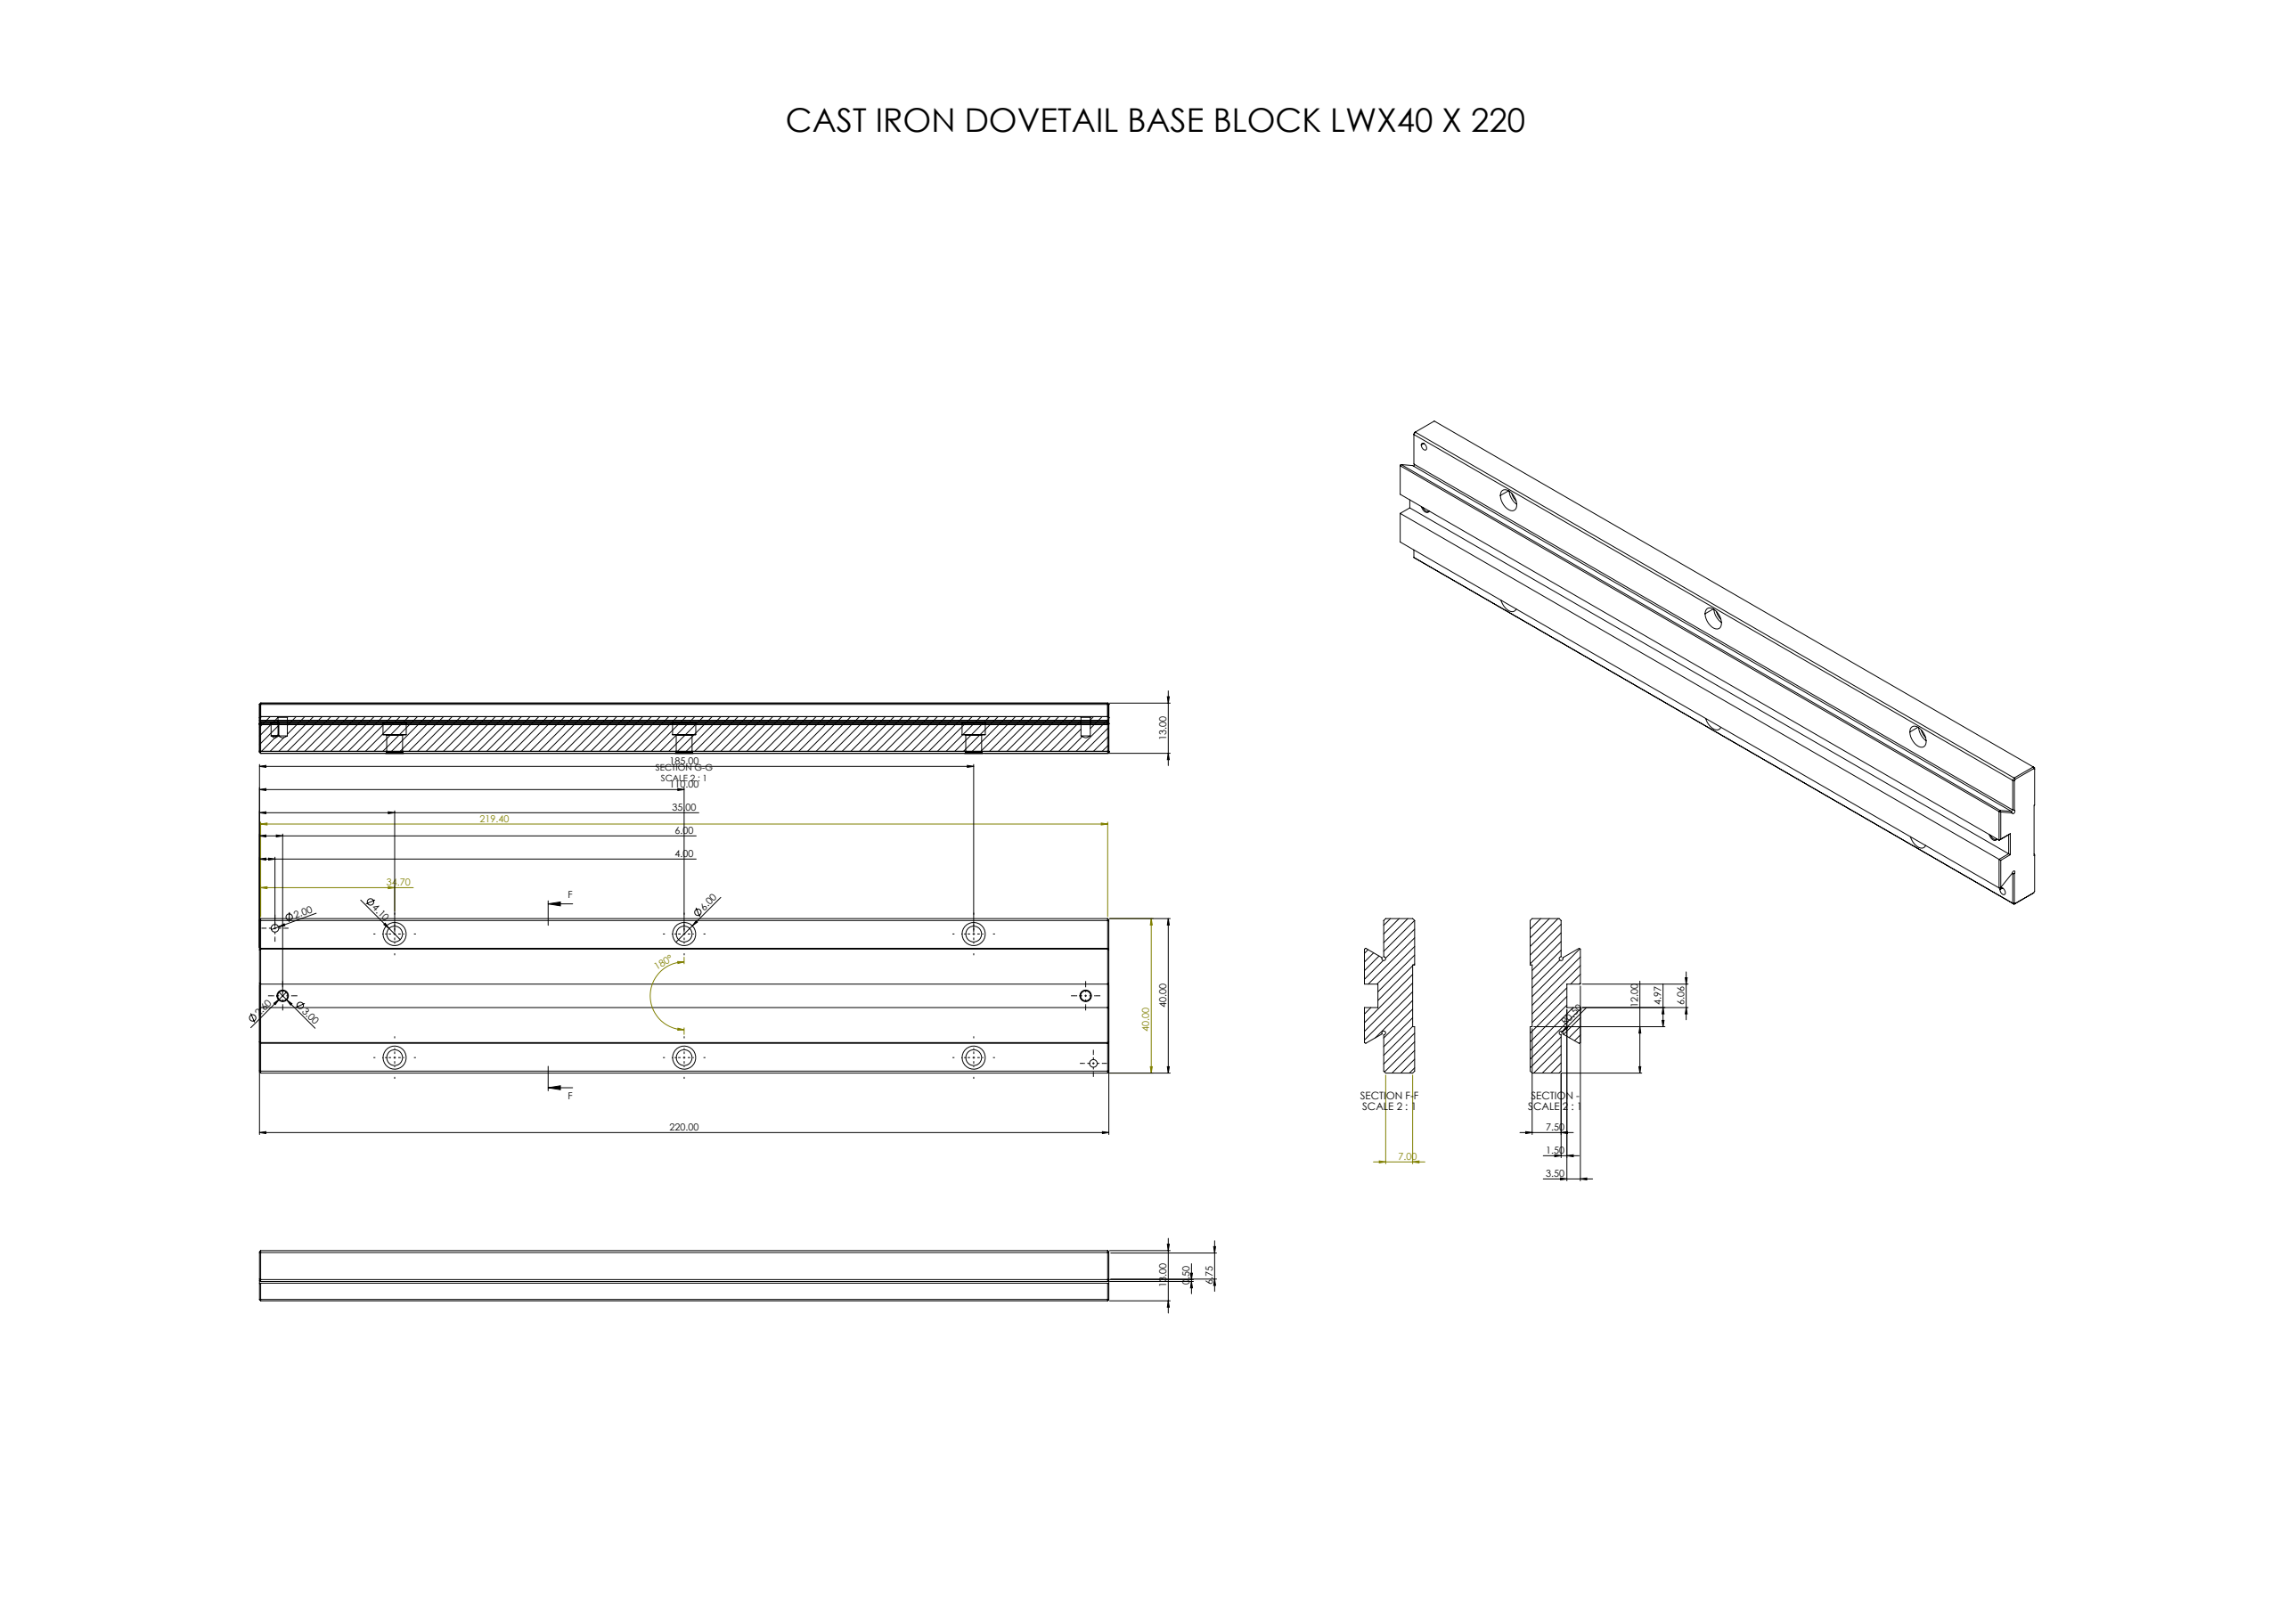
ISO-10303-21;
HEADER;
/* Generated by software containing ST-Developer
 * from STEP Tools, Inc. (www.steptools.com) 
 */

FILE_DESCRIPTION(
/* description */ (''),
/* implementation_level */ '2;1');

FILE_NAME(
/* name */ 'Cast Iron Dovetail Base Block LWX40 x 220.step',
/* time_stamp */ '2026-10-05T09:57:53+05:00',
/* author */ (''),
/* organization */ (''),
/* preprocessor_version */ 'ST-DEVELOPER v20.2',
/* originating_system */ 'Autodesk Translation Framework v15.15.0.0',
/* authorisation */ '');

FILE_SCHEMA (('AUTOMOTIVE_DESIGN { 1 0 10303 214 3 1 1 }'));
ENDSEC;

DATA;
#10=MECHANICAL_DESIGN_GEOMETRIC_PRESENTATION_REPRESENTATION('',(#551),#113984);
#515=SHAPE_REPRESENTATION_RELATIONSHIP('SRR','None',#114052,#533);
#533=ADVANCED_BREP_SHAPE_REPRESENTATION('',(#569),#113966);
#551=STYLED_ITEM('',(#114289),#569);
#569=MANIFOLD_SOLID_BREP('Cast Iron Dovetail Base Block LWX40 x 220',#60392);
#587=ELLIPSE('',#61749,0.707106781186562,0.499999999999998);
#588=ELLIPSE('',#61756,0.70710678118656,0.5);
#589=ELLIPSE('',#61760,0.707106781186549,0.499999999999998);
#590=ELLIPSE('',#61761,0.707106781186545,0.499999999999998);
#591=ELLIPSE('',#61762,0.707106781186558,0.499999999999998);
#592=ELLIPSE('',#61770,0.707106781186561,0.5);
#593=ELLIPSE('',#61787,0.707106781186547,0.5);
#594=ELLIPSE('',#61805,0.707106781186548,0.5);
#603=CYLINDRICAL_SURFACE('',#61679,1.);
#604=CYLINDRICAL_SURFACE('',#61681,1.00000000000001);
#605=CYLINDRICAL_SURFACE('',#61686,1.29999999999999);
#606=CYLINDRICAL_SURFACE('',#61693,1.3);
#607=CYLINDRICAL_SURFACE('',#61696,3.00000000000001);
#608=CYLINDRICAL_SURFACE('',#61701,3.);
#609=CYLINDRICAL_SURFACE('',#61706,3.);
#610=CYLINDRICAL_SURFACE('',#61711,3.00000000000001);
#611=CYLINDRICAL_SURFACE('',#61716,3.00000000000001);
#612=CYLINDRICAL_SURFACE('',#61721,3.00000000000001);
#613=CYLINDRICAL_SURFACE('',#61732,2.04999999999998);
#614=CYLINDRICAL_SURFACE('',#61735,2.05);
#615=CYLINDRICAL_SURFACE('',#61738,2.05);
#616=CYLINDRICAL_SURFACE('',#61741,2.05);
#617=CYLINDRICAL_SURFACE('',#61744,2.05);
#618=CYLINDRICAL_SURFACE('',#61747,2.04999999999998);
#619=CYLINDRICAL_SURFACE('',#61759,0.499999999999998);
#620=CYLINDRICAL_SURFACE('',#61809,0.5);
#875=CONICAL_SURFACE('',#61675,0.999999999999979,1.02974425867664);
#876=CONICAL_SURFACE('',#61677,1.,1.02974425867665);
#877=CONICAL_SURFACE('',#61683,1.39999999999999,0.785398163397437);
#878=CONICAL_SURFACE('',#61690,1.30000000000003,1.02974425867666);
#879=CONICAL_SURFACE('',#61691,1.4,0.785398163397448);
#880=CONICAL_SURFACE('',#61695,1.3,1.02974425867665);
#881=CONICAL_SURFACE('',#61726,2.19999999999999,0.785398163397467);
#882=CONICAL_SURFACE('',#61733,2.2,0.785398163397438);
#883=CONICAL_SURFACE('',#61736,2.2,0.785398163397438);
#884=CONICAL_SURFACE('',#61739,2.2,0.785398163397445);
#885=CONICAL_SURFACE('',#61742,2.2,0.785398163397445);
#886=CONICAL_SURFACE('',#61745,2.19999999999999,0.785398163397467);
#957=CIRCLE('',#61666,0.499999999999998);
#958=CIRCLE('',#61667,0.5);
#959=CIRCLE('',#61672,2.34999999999999);
#960=CIRCLE('',#61673,2.35);
#961=CIRCLE('',#61674,2.34999999999999);
#962=CIRCLE('',#61676,1.00000000000001);
#963=CIRCLE('',#61678,1.);
#964=CIRCLE('',#61680,1.);
#965=CIRCLE('',#61682,1.00000000000001);
#966=CIRCLE('',#61684,1.49999999999999);
#967=CIRCLE('',#61685,1.29999999999999);
#968=CIRCLE('',#61687,1.29999999999999);
#969=CIRCLE('',#61689,1.5);
#970=CIRCLE('',#61692,1.3);
#971=CIRCLE('',#61694,1.3);
#972=CIRCLE('',#61697,3.00000000000001);
#973=CIRCLE('',#61698,3.00000000000001);
#974=CIRCLE('',#61700,2.04999999999998);
#975=CIRCLE('',#61702,3.);
#976=CIRCLE('',#61703,3.);
#977=CIRCLE('',#61705,2.05);
#978=CIRCLE('',#61707,3.);
#979=CIRCLE('',#61708,3.);
#980=CIRCLE('',#61710,2.05);
#981=CIRCLE('',#61712,3.00000000000001);
#982=CIRCLE('',#61713,3.00000000000001);
#983=CIRCLE('',#61715,2.05);
#984=CIRCLE('',#61717,3.00000000000001);
#985=CIRCLE('',#61718,3.00000000000001);
#986=CIRCLE('',#61720,2.05);
#987=CIRCLE('',#61722,3.00000000000001);
#988=CIRCLE('',#61723,3.00000000000001);
#989=CIRCLE('',#61725,2.04999999999998);
#990=CIRCLE('',#61727,2.04999999999998);
#991=CIRCLE('',#61729,2.34999999999999);
#992=CIRCLE('',#61730,2.35);
#993=CIRCLE('',#61731,2.34999999999999);
#994=CIRCLE('',#61734,2.05);
#995=CIRCLE('',#61737,2.05);
#996=CIRCLE('',#61740,2.05);
#997=CIRCLE('',#61743,2.05);
#998=CIRCLE('',#61746,2.04999999999998);
#999=CIRCLE('',#61763,0.499999999999998);
#1000=CIRCLE('',#61807,0.5);
#1542=FACE_BOUND('',#7313,.T.);
#1543=FACE_BOUND('',#7345,.T.);
#1544=FACE_BOUND('',#7369,.T.);
#1545=FACE_BOUND('',#7404,.T.);
#1546=FACE_BOUND('',#7405,.T.);
#1547=FACE_BOUND('',#7430,.T.);
#1548=FACE_BOUND('',#7465,.T.);
#1549=FACE_BOUND('',#7495,.T.);
#1550=FACE_BOUND('',#7519,.T.);
#1551=FACE_BOUND('',#7565,.T.);
#1552=FACE_BOUND('',#7581,.T.);
#1553=FACE_BOUND('',#7605,.T.);
#1554=FACE_BOUND('',#7659,.T.);
#1555=FACE_BOUND('',#7705,.T.);
#1556=FACE_BOUND('',#7738,.T.);
#1557=FACE_BOUND('',#7761,.T.);
#1558=FACE_BOUND('',#7794,.T.);
#1559=FACE_BOUND('',#7840,.T.);
#1560=FACE_BOUND('',#7894,.T.);
#1561=FACE_BOUND('',#7910,.T.);
#1562=FACE_BOUND('',#7934,.T.);
#1563=FACE_BOUND('',#7980,.T.);
#1564=FACE_BOUND('',#8010,.T.);
#1565=FACE_BOUND('',#8034,.T.);
#1566=FACE_BOUND('',#8069,.T.);
#1567=FACE_BOUND('',#8104,.T.);
#1568=FACE_BOUND('',#8105,.T.);
#1569=FACE_BOUND('',#8130,.T.);
#1570=FACE_BOUND('',#8162,.T.);
#1571=FACE_BOUND('',#9078,.T.);
#1572=FACE_BOUND('',#9079,.T.);
#1573=FACE_BOUND('',#9080,.T.);
#1574=FACE_BOUND('',#9088,.T.);
#1575=FACE_BOUND('',#9089,.T.);
#1576=FACE_BOUND('',#9096,.T.);
#1577=FACE_BOUND('',#9099,.T.);
#1578=FACE_BOUND('',#9102,.T.);
#1579=FACE_BOUND('',#9105,.T.);
#1580=FACE_BOUND('',#9108,.T.);
#1581=FACE_BOUND('',#9111,.T.);
#1582=FACE_BOUND('',#9114,.T.);
#1583=FACE_BOUND('',#9115,.T.);
#1584=FACE_BOUND('',#9116,.T.);
#1585=FACE_BOUND('',#9152,.T.);
#1586=FACE_BOUND('',#9153,.T.);
#1587=FACE_BOUND('',#9154,.T.);
#1588=FACE_BOUND('',#9155,.T.);
#1589=FACE_BOUND('',#9161,.T.);
#1590=FACE_BOUND('',#9162,.T.);
#1591=FACE_BOUND('',#9163,.T.);
#1592=FACE_BOUND('',#9164,.T.);
#1593=FACE_BOUND('',#9165,.T.);
#1594=FACE_BOUND('',#9166,.T.);
#1595=FACE_BOUND('',#9167,.T.);
#1596=FACE_BOUND('',#9168,.T.);
#1597=FACE_BOUND('',#9169,.T.);
#1598=FACE_BOUND('',#9170,.T.);
#1599=FACE_BOUND('',#9171,.T.);
#1600=FACE_BOUND('',#9172,.T.);
#1601=FACE_BOUND('',#9173,.T.);
#1602=FACE_BOUND('',#9174,.T.);
#1603=FACE_BOUND('',#9175,.T.);
#1604=FACE_BOUND('',#9176,.T.);
#1605=FACE_BOUND('',#9177,.T.);
#1606=FACE_BOUND('',#9178,.T.);
#1607=FACE_BOUND('',#9179,.T.);
#1608=FACE_BOUND('',#9180,.T.);
#1609=FACE_BOUND('',#9181,.T.);
#1610=FACE_BOUND('',#9182,.T.);
#1611=FACE_BOUND('',#9183,.T.);
#1612=FACE_BOUND('',#9184,.T.);
#1613=FACE_BOUND('',#9185,.T.);
#1614=FACE_BOUND('',#9186,.T.);
#1615=FACE_BOUND('',#9187,.T.);
#1616=FACE_BOUND('',#9188,.T.);
#1617=FACE_BOUND('',#9189,.T.);
#1618=FACE_BOUND('',#9190,.T.);
#1619=FACE_BOUND('',#9191,.T.);
#1620=FACE_BOUND('',#9192,.T.);
#1621=FACE_BOUND('',#9193,.T.);
#1622=FACE_BOUND('',#9194,.T.);
#1623=FACE_BOUND('',#9195,.T.);
#1624=FACE_BOUND('',#9196,.T.);
#1625=FACE_BOUND('',#9197,.T.);
#1626=FACE_BOUND('',#9198,.T.);
#1627=FACE_BOUND('',#9199,.T.);
#1628=FACE_BOUND('',#9200,.T.);
#1629=FACE_BOUND('',#9201,.T.);
#1630=FACE_BOUND('',#9202,.T.);
#1631=FACE_BOUND('',#9203,.T.);
#1632=FACE_BOUND('',#9204,.T.);
#1633=FACE_BOUND('',#9205,.T.);
#1634=FACE_BOUND('',#9206,.T.);
#1635=FACE_BOUND('',#9207,.T.);
#1636=FACE_BOUND('',#9208,.T.);
#1637=FACE_BOUND('',#9209,.T.);
#1638=FACE_BOUND('',#9210,.T.);
#1639=FACE_BOUND('',#9211,.T.);
#1640=FACE_BOUND('',#9212,.T.);
#1641=FACE_BOUND('',#9213,.T.);
#1642=FACE_BOUND('',#9214,.T.);
#1643=FACE_BOUND('',#9215,.T.);
#1644=FACE_BOUND('',#9216,.T.);
#1645=FACE_BOUND('',#9217,.T.);
#1646=FACE_BOUND('',#9218,.T.);
#1647=FACE_BOUND('',#9219,.T.);
#1648=FACE_BOUND('',#9220,.T.);
#1649=FACE_BOUND('',#9221,.T.);
#1650=FACE_BOUND('',#9222,.T.);
#1651=FACE_BOUND('',#9223,.T.);
#1652=FACE_BOUND('',#9224,.T.);
#1653=FACE_BOUND('',#9225,.T.);
#1654=FACE_BOUND('',#9226,.T.);
#1655=FACE_BOUND('',#9227,.T.);
#1656=FACE_BOUND('',#9228,.T.);
#1657=FACE_BOUND('',#9229,.T.);
#1658=FACE_BOUND('',#9230,.T.);
#1659=FACE_BOUND('',#9231,.T.);
#1660=FACE_BOUND('',#9232,.T.);
#1661=FACE_BOUND('',#9233,.T.);
#1662=FACE_BOUND('',#9234,.T.);
#1663=FACE_BOUND('',#9235,.T.);
#1664=FACE_BOUND('',#9236,.T.);
#1665=FACE_BOUND('',#9237,.T.);
#1666=FACE_BOUND('',#9238,.T.);
#1667=FACE_BOUND('',#9239,.T.);
#1668=FACE_BOUND('',#9240,.T.);
#1669=FACE_BOUND('',#9241,.T.);
#1670=FACE_BOUND('',#9242,.T.);
#1671=FACE_BOUND('',#9243,.T.);
#1672=FACE_BOUND('',#9244,.T.);
#1673=FACE_BOUND('',#9245,.T.);
#1674=FACE_BOUND('',#9246,.T.);
#1675=FACE_BOUND('',#9247,.T.);
#1676=FACE_BOUND('',#9248,.T.);
#1677=FACE_BOUND('',#9249,.T.);
#1678=FACE_BOUND('',#9250,.T.);
#1679=FACE_BOUND('',#9251,.T.);
#1680=FACE_BOUND('',#9252,.T.);
#1681=FACE_BOUND('',#9253,.T.);
#1682=FACE_BOUND('',#9254,.T.);
#1683=FACE_BOUND('',#9255,.T.);
#1684=FACE_BOUND('',#9256,.T.);
#1685=FACE_BOUND('',#9257,.T.);
#1686=FACE_BOUND('',#9258,.T.);
#1687=FACE_BOUND('',#9259,.T.);
#1688=FACE_BOUND('',#9260,.T.);
#1689=FACE_BOUND('',#9261,.T.);
#1690=FACE_BOUND('',#9262,.T.);
#1691=FACE_BOUND('',#9263,.T.);
#1692=FACE_BOUND('',#9264,.T.);
#1693=FACE_BOUND('',#9265,.T.);
#1694=FACE_BOUND('',#9266,.T.);
#1695=FACE_BOUND('',#9267,.T.);
#1696=FACE_BOUND('',#9268,.T.);
#1697=FACE_BOUND('',#9269,.T.);
#1698=FACE_BOUND('',#9270,.T.);
#1699=FACE_BOUND('',#9271,.T.);
#1700=FACE_BOUND('',#9272,.T.);
#1701=FACE_BOUND('',#9273,.T.);
#1702=FACE_BOUND('',#9274,.T.);
#1703=FACE_BOUND('',#9275,.T.);
#1704=FACE_BOUND('',#9276,.T.);
#1705=FACE_BOUND('',#9277,.T.);
#1706=FACE_BOUND('',#9278,.T.);
#1707=FACE_BOUND('',#9279,.T.);
#1708=FACE_BOUND('',#9280,.T.);
#1709=FACE_BOUND('',#9281,.T.);
#1710=FACE_BOUND('',#9282,.T.);
#1711=FACE_BOUND('',#9283,.T.);
#1712=FACE_BOUND('',#9284,.T.);
#1713=FACE_BOUND('',#9285,.T.);
#1714=FACE_BOUND('',#9286,.T.);
#1715=FACE_BOUND('',#9287,.T.);
#1716=FACE_BOUND('',#9288,.T.);
#1717=FACE_BOUND('',#9289,.T.);
#1718=FACE_BOUND('',#9290,.T.);
#1719=FACE_BOUND('',#9291,.T.);
#1720=FACE_BOUND('',#9292,.T.);
#1721=FACE_BOUND('',#9293,.T.);
#1722=FACE_BOUND('',#9294,.T.);
#1723=FACE_BOUND('',#9295,.T.);
#1724=FACE_BOUND('',#9296,.T.);
#1725=FACE_BOUND('',#9297,.T.);
#1726=FACE_BOUND('',#9298,.T.);
#1727=FACE_BOUND('',#9299,.T.);
#1728=FACE_BOUND('',#9300,.T.);
#1729=FACE_BOUND('',#9301,.T.);
#1730=FACE_BOUND('',#9302,.T.);
#1731=FACE_BOUND('',#9303,.T.);
#1732=FACE_BOUND('',#9304,.T.);
#1733=FACE_BOUND('',#9305,.T.);
#1734=FACE_BOUND('',#9306,.T.);
#1735=FACE_BOUND('',#9307,.T.);
#1736=FACE_BOUND('',#9308,.T.);
#1737=FACE_BOUND('',#9309,.T.);
#1738=FACE_BOUND('',#9310,.T.);
#1739=FACE_BOUND('',#9311,.T.);
#1740=FACE_BOUND('',#9312,.T.);
#1741=FACE_BOUND('',#9313,.T.);
#1742=FACE_BOUND('',#9314,.T.);
#1743=FACE_BOUND('',#9315,.T.);
#1744=FACE_BOUND('',#9316,.T.);
#1745=FACE_BOUND('',#9317,.T.);
#1746=FACE_BOUND('',#9318,.T.);
#1747=FACE_BOUND('',#9319,.T.);
#1748=FACE_BOUND('',#9320,.T.);
#1749=FACE_BOUND('',#9321,.T.);
#1750=FACE_BOUND('',#9322,.T.);
#1751=FACE_BOUND('',#9323,.T.);
#1752=FACE_BOUND('',#9324,.T.);
#1753=FACE_BOUND('',#9325,.T.);
#1754=FACE_BOUND('',#9326,.T.);
#1755=FACE_BOUND('',#9327,.T.);
#1756=FACE_BOUND('',#9328,.T.);
#1757=FACE_BOUND('',#9329,.T.);
#1758=FACE_BOUND('',#9330,.T.);
#1759=FACE_BOUND('',#9331,.T.);
#1760=FACE_BOUND('',#9332,.T.);
#1761=FACE_BOUND('',#9333,.T.);
#1762=FACE_BOUND('',#9334,.T.);
#1763=FACE_BOUND('',#9335,.T.);
#1764=FACE_BOUND('',#9336,.T.);
#1765=FACE_BOUND('',#9337,.T.);
#1766=FACE_BOUND('',#9338,.T.);
#1767=FACE_BOUND('',#9339,.T.);
#1768=FACE_BOUND('',#9340,.T.);
#1769=FACE_BOUND('',#9341,.T.);
#1770=FACE_BOUND('',#9342,.T.);
#1771=FACE_BOUND('',#9343,.T.);
#1772=FACE_BOUND('',#9344,.T.);
#1773=FACE_BOUND('',#9345,.T.);
#1774=FACE_BOUND('',#9346,.T.);
#1775=FACE_BOUND('',#9347,.T.);
#1776=FACE_BOUND('',#9348,.T.);
#1777=FACE_BOUND('',#9349,.T.);
#1778=FACE_BOUND('',#9350,.T.);
#1779=FACE_BOUND('',#9351,.T.);
#1780=FACE_BOUND('',#9352,.T.);
#1781=FACE_BOUND('',#9353,.T.);
#1782=FACE_BOUND('',#9354,.T.);
#1783=FACE_BOUND('',#9355,.T.);
#1784=FACE_BOUND('',#9356,.T.);
#1785=FACE_BOUND('',#9357,.T.);
#1786=FACE_BOUND('',#9358,.T.);
#1787=FACE_BOUND('',#9359,.T.);
#1788=FACE_BOUND('',#9360,.T.);
#1789=FACE_BOUND('',#9361,.T.);
#1790=FACE_BOUND('',#9362,.T.);
#1791=FACE_BOUND('',#9363,.T.);
#1792=FACE_BOUND('',#9364,.T.);
#1793=FACE_BOUND('',#9365,.T.);
#1794=FACE_BOUND('',#9366,.T.);
#1795=FACE_BOUND('',#9367,.T.);
#1796=FACE_BOUND('',#9368,.T.);
#1797=FACE_BOUND('',#9369,.T.);
#1798=FACE_BOUND('',#9370,.T.);
#1799=FACE_BOUND('',#9371,.T.);
#1800=FACE_BOUND('',#9372,.T.);
#1801=FACE_BOUND('',#9373,.T.);
#1802=FACE_BOUND('',#9374,.T.);
#1803=FACE_BOUND('',#9375,.T.);
#1804=FACE_BOUND('',#9376,.T.);
#1805=FACE_BOUND('',#9377,.T.);
#1806=FACE_BOUND('',#9378,.T.);
#1807=FACE_BOUND('',#9381,.T.);
#1808=FACE_BOUND('',#9382,.T.);
#1809=FACE_BOUND('',#9383,.T.);
#1810=FACE_BOUND('',#9384,.T.);
#1859=PLANE('',#60611);
#1860=PLANE('',#60612);
#1861=PLANE('',#60613);
#1862=PLANE('',#60614);
#1863=PLANE('',#60615);
#1864=PLANE('',#60616);
#1865=PLANE('',#60617);
#1866=PLANE('',#60618);
#1867=PLANE('',#60619);
#1868=PLANE('',#60620);
#1869=PLANE('',#60621);
#1870=PLANE('',#60622);
#1871=PLANE('',#60623);
#1872=PLANE('',#60624);
#1873=PLANE('',#60625);
#1874=PLANE('',#60626);
#1875=PLANE('',#60627);
#1876=PLANE('',#60628);
#1877=PLANE('',#60629);
#1878=PLANE('',#60630);
#1879=PLANE('',#60631);
#1880=PLANE('',#60632);
#1881=PLANE('',#60633);
#1882=PLANE('',#60634);
#1883=PLANE('',#60635);
#1884=PLANE('',#60636);
#1885=PLANE('',#60637);
#1886=PLANE('',#60638);
#1887=PLANE('',#60639);
#1888=PLANE('',#60640);
#1889=PLANE('',#60641);
#1890=PLANE('',#60642);
#1891=PLANE('',#60643);
#1892=PLANE('',#60644);
#1893=PLANE('',#60645);
#1894=PLANE('',#60646);
#1895=PLANE('',#60647);
#1896=PLANE('',#60648);
#1897=PLANE('',#60649);
#1898=PLANE('',#60650);
#1899=PLANE('',#60651);
#1900=PLANE('',#60652);
#1901=PLANE('',#60653);
#1902=PLANE('',#60654);
#1903=PLANE('',#60655);
#1904=PLANE('',#60656);
#1905=PLANE('',#60657);
#1906=PLANE('',#60658);
#1907=PLANE('',#60659);
#1908=PLANE('',#60660);
#1909=PLANE('',#60661);
#1910=PLANE('',#60662);
#1911=PLANE('',#60663);
#1912=PLANE('',#60664);
#1913=PLANE('',#60665);
#1914=PLANE('',#60666);
#1915=PLANE('',#60667);
#1916=PLANE('',#60668);
#1917=PLANE('',#60669);
#1918=PLANE('',#60670);
#1919=PLANE('',#60671);
#1920=PLANE('',#60672);
#1921=PLANE('',#60673);
#1922=PLANE('',#60674);
#1923=PLANE('',#60675);
#1924=PLANE('',#60676);
#1925=PLANE('',#60677);
#1926=PLANE('',#60678);
#1927=PLANE('',#60679);
#1928=PLANE('',#60680);
#1929=PLANE('',#60681);
#1930=PLANE('',#60682);
#1931=PLANE('',#60683);
#1932=PLANE('',#60684);
#1933=PLANE('',#60685);
#1934=PLANE('',#60686);
#1935=PLANE('',#60687);
#1936=PLANE('',#60688);
#1937=PLANE('',#60689);
#1938=PLANE('',#60690);
#1939=PLANE('',#60691);
#1940=PLANE('',#60692);
#1941=PLANE('',#60693);
#1942=PLANE('',#60694);
#1943=PLANE('',#60695);
#1944=PLANE('',#60696);
#1945=PLANE('',#60697);
#1946=PLANE('',#60698);
#1947=PLANE('',#60699);
#1948=PLANE('',#60700);
#1949=PLANE('',#60701);
#1950=PLANE('',#60702);
#1951=PLANE('',#60703);
#1952=PLANE('',#60704);
#1953=PLANE('',#60705);
#1954=PLANE('',#60706);
#1955=PLANE('',#60707);
#1956=PLANE('',#60708);
#1957=PLANE('',#60709);
#1958=PLANE('',#60710);
#1959=PLANE('',#60711);
#1960=PLANE('',#60712);
#1961=PLANE('',#60713);
#1962=PLANE('',#60714);
#1963=PLANE('',#60715);
#1964=PLANE('',#60716);
#1965=PLANE('',#60717);
#1966=PLANE('',#60718);
#1967=PLANE('',#60719);
#1968=PLANE('',#60720);
#1969=PLANE('',#60721);
#1970=PLANE('',#60722);
#1971=PLANE('',#60723);
#1972=PLANE('',#60724);
#1973=PLANE('',#60725);
#1974=PLANE('',#60726);
#1975=PLANE('',#60727);
#1976=PLANE('',#60728);
#1977=PLANE('',#60729);
#1978=PLANE('',#60730);
#1979=PLANE('',#60731);
#1980=PLANE('',#60732);
#1981=PLANE('',#60733);
#1982=PLANE('',#60734);
#1983=PLANE('',#60735);
#1984=PLANE('',#60736);
#1985=PLANE('',#60737);
#1986=PLANE('',#60738);
#1987=PLANE('',#60739);
#1988=PLANE('',#60740);
#1989=PLANE('',#60741);
#1990=PLANE('',#60742);
#1991=PLANE('',#60743);
#1992=PLANE('',#60744);
#1993=PLANE('',#60745);
#1994=PLANE('',#60746);
#1995=PLANE('',#60747);
#1996=PLANE('',#60748);
#1997=PLANE('',#60749);
#1998=PLANE('',#60750);
#1999=PLANE('',#60751);
#2000=PLANE('',#60752);
#2001=PLANE('',#60753);
#2002=PLANE('',#60754);
#2003=PLANE('',#60755);
#2004=PLANE('',#60756);
#2005=PLANE('',#60757);
#2006=PLANE('',#60758);
#2007=PLANE('',#60759);
#2008=PLANE('',#60760);
#2009=PLANE('',#60761);
#2010=PLANE('',#60762);
#2011=PLANE('',#60763);
#2012=PLANE('',#60764);
#2013=PLANE('',#60765);
#2014=PLANE('',#60766);
#2015=PLANE('',#60767);
#2016=PLANE('',#60768);
#2017=PLANE('',#60769);
#2018=PLANE('',#60770);
#2019=PLANE('',#60771);
#2020=PLANE('',#60772);
#2021=PLANE('',#60773);
#2022=PLANE('',#60774);
#2023=PLANE('',#60775);
#2024=PLANE('',#60776);
#2025=PLANE('',#60777);
#2026=PLANE('',#60778);
#2027=PLANE('',#60779);
#2028=PLANE('',#60780);
#2029=PLANE('',#60781);
#2030=PLANE('',#60782);
#2031=PLANE('',#60783);
#2032=PLANE('',#60784);
#2033=PLANE('',#60785);
#2034=PLANE('',#60786);
#2035=PLANE('',#60787);
#2036=PLANE('',#60788);
#2037=PLANE('',#60789);
#2038=PLANE('',#60790);
#2039=PLANE('',#60791);
#2040=PLANE('',#60792);
#2041=PLANE('',#60793);
#2042=PLANE('',#60794);
#2043=PLANE('',#60795);
#2044=PLANE('',#60796);
#2045=PLANE('',#60797);
#2046=PLANE('',#60798);
#2047=PLANE('',#60799);
#2048=PLANE('',#60800);
#2049=PLANE('',#60801);
#2050=PLANE('',#60802);
#2051=PLANE('',#60803);
#2052=PLANE('',#60804);
#2053=PLANE('',#60805);
#2054=PLANE('',#60806);
#2055=PLANE('',#60807);
#2056=PLANE('',#60808);
#2057=PLANE('',#60809);
#2058=PLANE('',#60810);
#2059=PLANE('',#60811);
#2060=PLANE('',#60812);
#2061=PLANE('',#60813);
#2062=PLANE('',#60814);
#2063=PLANE('',#60815);
#2064=PLANE('',#60816);
#2065=PLANE('',#60817);
#2066=PLANE('',#60818);
#2067=PLANE('',#60819);
#2068=PLANE('',#60820);
#2069=PLANE('',#60821);
#2070=PLANE('',#60822);
#2071=PLANE('',#60823);
#2072=PLANE('',#60824);
#2073=PLANE('',#60825);
#2074=PLANE('',#60826);
#2075=PLANE('',#60827);
#2076=PLANE('',#60828);
#2077=PLANE('',#60829);
#2078=PLANE('',#60830);
#2079=PLANE('',#60831);
#2080=PLANE('',#60832);
#2081=PLANE('',#60833);
#2082=PLANE('',#60834);
#2083=PLANE('',#60835);
#2084=PLANE('',#60836);
#2085=PLANE('',#60837);
#2086=PLANE('',#60838);
#2087=PLANE('',#60839);
#2088=PLANE('',#60840);
#2089=PLANE('',#60841);
#2090=PLANE('',#60842);
#2091=PLANE('',#60843);
#2092=PLANE('',#60844);
#2093=PLANE('',#60845);
#2094=PLANE('',#60846);
#2095=PLANE('',#60847);
#2096=PLANE('',#60848);
#2097=PLANE('',#60849);
#2098=PLANE('',#60850);
#2099=PLANE('',#60851);
#2100=PLANE('',#60852);
#2101=PLANE('',#60853);
#2102=PLANE('',#60854);
#2103=PLANE('',#60855);
#2104=PLANE('',#60856);
#2105=PLANE('',#60857);
#2106=PLANE('',#60858);
#2107=PLANE('',#60859);
#2108=PLANE('',#60860);
#2109=PLANE('',#60861);
#2110=PLANE('',#60862);
#2111=PLANE('',#60863);
#2112=PLANE('',#60864);
#2113=PLANE('',#60865);
#2114=PLANE('',#60866);
#2115=PLANE('',#60867);
#2116=PLANE('',#60868);
#2117=PLANE('',#60869);
#2118=PLANE('',#60870);
#2119=PLANE('',#60871);
#2120=PLANE('',#60872);
#2121=PLANE('',#60873);
#2122=PLANE('',#60874);
#2123=PLANE('',#60875);
#2124=PLANE('',#60876);
#2125=PLANE('',#60877);
#2126=PLANE('',#60878);
#2127=PLANE('',#60879);
#2128=PLANE('',#60880);
#2129=PLANE('',#60881);
#2130=PLANE('',#60882);
#2131=PLANE('',#60883);
#2132=PLANE('',#60884);
#2133=PLANE('',#60885);
#2134=PLANE('',#60886);
#2135=PLANE('',#60887);
#2136=PLANE('',#60888);
#2137=PLANE('',#60889);
#2138=PLANE('',#60890);
#2139=PLANE('',#60891);
#2140=PLANE('',#60892);
#2141=PLANE('',#60893);
#2142=PLANE('',#60894);
#2143=PLANE('',#60895);
#2144=PLANE('',#60896);
#2145=PLANE('',#60897);
#2146=PLANE('',#60898);
#2147=PLANE('',#60899);
#2148=PLANE('',#60900);
#2149=PLANE('',#60901);
#2150=PLANE('',#60902);
#2151=PLANE('',#60903);
#2152=PLANE('',#60904);
#2153=PLANE('',#60905);
#2154=PLANE('',#60906);
#2155=PLANE('',#60907);
#2156=PLANE('',#60908);
#2157=PLANE('',#60909);
#2158=PLANE('',#60910);
#2159=PLANE('',#60911);
#2160=PLANE('',#60912);
#2161=PLANE('',#60913);
#2162=PLANE('',#60914);
#2163=PLANE('',#60915);
#2164=PLANE('',#60916);
#2165=PLANE('',#60917);
#2166=PLANE('',#60918);
#2167=PLANE('',#60919);
#2168=PLANE('',#60920);
#2169=PLANE('',#60921);
#2170=PLANE('',#60922);
#2171=PLANE('',#60923);
#2172=PLANE('',#60924);
#2173=PLANE('',#60925);
#2174=PLANE('',#60926);
#2175=PLANE('',#60927);
#2176=PLANE('',#60928);
#2177=PLANE('',#60929);
#2178=PLANE('',#60930);
#2179=PLANE('',#60931);
#2180=PLANE('',#60932);
#2181=PLANE('',#60933);
#2182=PLANE('',#60934);
#2183=PLANE('',#60935);
#2184=PLANE('',#60936);
#2185=PLANE('',#60937);
#2186=PLANE('',#60938);
#2187=PLANE('',#60939);
#2188=PLANE('',#60940);
#2189=PLANE('',#60941);
#2190=PLANE('',#60942);
#2191=PLANE('',#60943);
#2192=PLANE('',#60944);
#2193=PLANE('',#60945);
#2194=PLANE('',#60946);
#2195=PLANE('',#60947);
#2196=PLANE('',#60948);
#2197=PLANE('',#60949);
#2198=PLANE('',#60950);
#2199=PLANE('',#60951);
#2200=PLANE('',#60952);
#2201=PLANE('',#60953);
#2202=PLANE('',#60954);
#2203=PLANE('',#60955);
#2204=PLANE('',#60956);
#2205=PLANE('',#60957);
#2206=PLANE('',#60958);
#2207=PLANE('',#60959);
#2208=PLANE('',#60960);
#2209=PLANE('',#60961);
#2210=PLANE('',#60962);
#2211=PLANE('',#60963);
#2212=PLANE('',#60964);
#2213=PLANE('',#60965);
#2214=PLANE('',#60966);
#2215=PLANE('',#60967);
#2216=PLANE('',#60968);
#2217=PLANE('',#60969);
#2218=PLANE('',#60970);
#2219=PLANE('',#60971);
#2220=PLANE('',#60972);
#2221=PLANE('',#60973);
#2222=PLANE('',#60974);
#2223=PLANE('',#60975);
#2224=PLANE('',#60976);
#2225=PLANE('',#60977);
#2226=PLANE('',#60978);
#2227=PLANE('',#60979);
#2228=PLANE('',#60980);
#2229=PLANE('',#60981);
#2230=PLANE('',#60982);
#2231=PLANE('',#60983);
#2232=PLANE('',#60984);
#2233=PLANE('',#60985);
#2234=PLANE('',#60986);
#2235=PLANE('',#60987);
#2236=PLANE('',#60988);
#2237=PLANE('',#60989);
#2238=PLANE('',#60990);
#2239=PLANE('',#60991);
#2240=PLANE('',#60992);
#2241=PLANE('',#60993);
#2242=PLANE('',#60994);
#2243=PLANE('',#60995);
#2244=PLANE('',#60996);
#2245=PLANE('',#60997);
#2246=PLANE('',#60998);
#2247=PLANE('',#60999);
#2248=PLANE('',#61000);
#2249=PLANE('',#61001);
#2250=PLANE('',#61002);
#2251=PLANE('',#61003);
#2252=PLANE('',#61004);
#2253=PLANE('',#61005);
#2254=PLANE('',#61006);
#2255=PLANE('',#61007);
#2256=PLANE('',#61008);
#2257=PLANE('',#61009);
#2258=PLANE('',#61010);
#2259=PLANE('',#61011);
#2260=PLANE('',#61012);
#2261=PLANE('',#61013);
#2262=PLANE('',#61014);
#2263=PLANE('',#61015);
#2264=PLANE('',#61016);
#2265=PLANE('',#61017);
#2266=PLANE('',#61018);
#2267=PLANE('',#61019);
#2268=PLANE('',#61020);
#2269=PLANE('',#61021);
#2270=PLANE('',#61022);
#2271=PLANE('',#61023);
#2272=PLANE('',#61024);
#2273=PLANE('',#61025);
#2274=PLANE('',#61026);
#2275=PLANE('',#61027);
#2276=PLANE('',#61028);
#2277=PLANE('',#61029);
#2278=PLANE('',#61030);
#2279=PLANE('',#61031);
#2280=PLANE('',#61032);
#2281=PLANE('',#61033);
#2282=PLANE('',#61034);
#2283=PLANE('',#61035);
#2284=PLANE('',#61036);
#2285=PLANE('',#61037);
#2286=PLANE('',#61038);
#2287=PLANE('',#61039);
#2288=PLANE('',#61040);
#2289=PLANE('',#61041);
#2290=PLANE('',#61042);
#2291=PLANE('',#61043);
#2292=PLANE('',#61044);
#2293=PLANE('',#61045);
#2294=PLANE('',#61046);
#2295=PLANE('',#61047);
#2296=PLANE('',#61048);
#2297=PLANE('',#61049);
#2298=PLANE('',#61050);
#2299=PLANE('',#61051);
#2300=PLANE('',#61052);
#2301=PLANE('',#61053);
#2302=PLANE('',#61054);
#2303=PLANE('',#61055);
#2304=PLANE('',#61056);
#2305=PLANE('',#61057);
#2306=PLANE('',#61058);
#2307=PLANE('',#61059);
#2308=PLANE('',#61060);
#2309=PLANE('',#61061);
#2310=PLANE('',#61062);
#2311=PLANE('',#61063);
#2312=PLANE('',#61064);
#2313=PLANE('',#61065);
#2314=PLANE('',#61066);
#2315=PLANE('',#61067);
#2316=PLANE('',#61068);
#2317=PLANE('',#61069);
#2318=PLANE('',#61070);
#2319=PLANE('',#61071);
#2320=PLANE('',#61072);
#2321=PLANE('',#61073);
#2322=PLANE('',#61074);
#2323=PLANE('',#61075);
#2324=PLANE('',#61076);
#2325=PLANE('',#61077);
#2326=PLANE('',#61078);
#2327=PLANE('',#61079);
#2328=PLANE('',#61080);
#2329=PLANE('',#61081);
#2330=PLANE('',#61082);
#2331=PLANE('',#61083);
#2332=PLANE('',#61084);
#2333=PLANE('',#61085);
#2334=PLANE('',#61086);
#2335=PLANE('',#61087);
#2336=PLANE('',#61088);
#2337=PLANE('',#61089);
#2338=PLANE('',#61090);
#2339=PLANE('',#61091);
#2340=PLANE('',#61092);
#2341=PLANE('',#61093);
#2342=PLANE('',#61094);
#2343=PLANE('',#61095);
#2344=PLANE('',#61096);
#2345=PLANE('',#61097);
#2346=PLANE('',#61098);
#2347=PLANE('',#61099);
#2348=PLANE('',#61100);
#2349=PLANE('',#61101);
#2350=PLANE('',#61102);
#2351=PLANE('',#61103);
#2352=PLANE('',#61104);
#2353=PLANE('',#61105);
#2354=PLANE('',#61106);
#2355=PLANE('',#61107);
#2356=PLANE('',#61108);
#2357=PLANE('',#61109);
#2358=PLANE('',#61110);
#2359=PLANE('',#61111);
#2360=PLANE('',#61112);
#2361=PLANE('',#61113);
#2362=PLANE('',#61114);
#2363=PLANE('',#61115);
#2364=PLANE('',#61116);
#2365=PLANE('',#61117);
#2366=PLANE('',#61118);
#2367=PLANE('',#61119);
#2368=PLANE('',#61120);
#2369=PLANE('',#61121);
#2370=PLANE('',#61122);
#2371=PLANE('',#61123);
#2372=PLANE('',#61124);
#2373=PLANE('',#61125);
#2374=PLANE('',#61126);
#2375=PLANE('',#61127);
#2376=PLANE('',#61128);
#2377=PLANE('',#61129);
#2378=PLANE('',#61130);
#2379=PLANE('',#61131);
#2380=PLANE('',#61132);
#2381=PLANE('',#61133);
#2382=PLANE('',#61134);
#2383=PLANE('',#61135);
#2384=PLANE('',#61136);
#2385=PLANE('',#61137);
#2386=PLANE('',#61138);
#2387=PLANE('',#61139);
#2388=PLANE('',#61140);
#2389=PLANE('',#61141);
#2390=PLANE('',#61142);
#2391=PLANE('',#61143);
#2392=PLANE('',#61144);
#2393=PLANE('',#61145);
#2394=PLANE('',#61146);
#2395=PLANE('',#61147);
#2396=PLANE('',#61148);
#2397=PLANE('',#61149);
#2398=PLANE('',#61150);
#2399=PLANE('',#61151);
#2400=PLANE('',#61152);
#2401=PLANE('',#61153);
#2402=PLANE('',#61154);
#2403=PLANE('',#61155);
#2404=PLANE('',#61156);
#2405=PLANE('',#61157);
#2406=PLANE('',#61158);
#2407=PLANE('',#61159);
#2408=PLANE('',#61160);
#2409=PLANE('',#61161);
#2410=PLANE('',#61162);
#2411=PLANE('',#61163);
#2412=PLANE('',#61164);
#2413=PLANE('',#61165);
#2414=PLANE('',#61166);
#2415=PLANE('',#61167);
#2416=PLANE('',#61168);
#2417=PLANE('',#61169);
#2418=PLANE('',#61170);
#2419=PLANE('',#61171);
#2420=PLANE('',#61172);
#2421=PLANE('',#61173);
#2422=PLANE('',#61174);
#2423=PLANE('',#61175);
#2424=PLANE('',#61176);
#2425=PLANE('',#61177);
#2426=PLANE('',#61178);
#2427=PLANE('',#61179);
#2428=PLANE('',#61180);
#2429=PLANE('',#61181);
#2430=PLANE('',#61182);
#2431=PLANE('',#61183);
#2432=PLANE('',#61184);
#2433=PLANE('',#61185);
#2434=PLANE('',#61186);
#2435=PLANE('',#61187);
#2436=PLANE('',#61188);
#2437=PLANE('',#61189);
#2438=PLANE('',#61190);
#2439=PLANE('',#61191);
#2440=PLANE('',#61192);
#2441=PLANE('',#61193);
#2442=PLANE('',#61194);
#2443=PLANE('',#61195);
#2444=PLANE('',#61196);
#2445=PLANE('',#61197);
#2446=PLANE('',#61198);
#2447=PLANE('',#61199);
#2448=PLANE('',#61200);
#2449=PLANE('',#61201);
#2450=PLANE('',#61202);
#2451=PLANE('',#61203);
#2452=PLANE('',#61204);
#2453=PLANE('',#61205);
#2454=PLANE('',#61206);
#2455=PLANE('',#61207);
#2456=PLANE('',#61208);
#2457=PLANE('',#61209);
#2458=PLANE('',#61210);
#2459=PLANE('',#61211);
#2460=PLANE('',#61212);
#2461=PLANE('',#61213);
#2462=PLANE('',#61214);
#2463=PLANE('',#61215);
#2464=PLANE('',#61216);
#2465=PLANE('',#61217);
#2466=PLANE('',#61218);
#2467=PLANE('',#61219);
#2468=PLANE('',#61220);
#2469=PLANE('',#61221);
#2470=PLANE('',#61222);
#2471=PLANE('',#61223);
#2472=PLANE('',#61224);
#2473=PLANE('',#61225);
#2474=PLANE('',#61226);
#2475=PLANE('',#61227);
#2476=PLANE('',#61228);
#2477=PLANE('',#61229);
#2478=PLANE('',#61230);
#2479=PLANE('',#61231);
#2480=PLANE('',#61232);
#2481=PLANE('',#61233);
#2482=PLANE('',#61234);
#2483=PLANE('',#61235);
#2484=PLANE('',#61236);
#2485=PLANE('',#61237);
#2486=PLANE('',#61238);
#2487=PLANE('',#61239);
#2488=PLANE('',#61240);
#2489=PLANE('',#61241);
#2490=PLANE('',#61242);
#2491=PLANE('',#61243);
#2492=PLANE('',#61244);
#2493=PLANE('',#61245);
#2494=PLANE('',#61246);
#2495=PLANE('',#61247);
#2496=PLANE('',#61248);
#2497=PLANE('',#61249);
#2498=PLANE('',#61250);
#2499=PLANE('',#61251);
#2500=PLANE('',#61252);
#2501=PLANE('',#61253);
#2502=PLANE('',#61254);
#2503=PLANE('',#61255);
#2504=PLANE('',#61256);
#2505=PLANE('',#61257);
#2506=PLANE('',#61258);
#2507=PLANE('',#61259);
#2508=PLANE('',#61260);
#2509=PLANE('',#61261);
#2510=PLANE('',#61262);
#2511=PLANE('',#61263);
#2512=PLANE('',#61264);
#2513=PLANE('',#61265);
#2514=PLANE('',#61266);
#2515=PLANE('',#61267);
#2516=PLANE('',#61268);
#2517=PLANE('',#61269);
#2518=PLANE('',#61270);
#2519=PLANE('',#61271);
#2520=PLANE('',#61272);
#2521=PLANE('',#61273);
#2522=PLANE('',#61274);
#2523=PLANE('',#61275);
#2524=PLANE('',#61276);
#2525=PLANE('',#61277);
#2526=PLANE('',#61278);
#2527=PLANE('',#61279);
#2528=PLANE('',#61280);
#2529=PLANE('',#61281);
#2530=PLANE('',#61282);
#2531=PLANE('',#61283);
#2532=PLANE('',#61284);
#2533=PLANE('',#61285);
#2534=PLANE('',#61286);
#2535=PLANE('',#61287);
#2536=PLANE('',#61288);
#2537=PLANE('',#61289);
#2538=PLANE('',#61290);
#2539=PLANE('',#61291);
#2540=PLANE('',#61292);
#2541=PLANE('',#61293);
#2542=PLANE('',#61294);
#2543=PLANE('',#61295);
#2544=PLANE('',#61296);
#2545=PLANE('',#61297);
#2546=PLANE('',#61298);
#2547=PLANE('',#61299);
#2548=PLANE('',#61300);
#2549=PLANE('',#61301);
#2550=PLANE('',#61302);
#2551=PLANE('',#61303);
#2552=PLANE('',#61304);
#2553=PLANE('',#61305);
#2554=PLANE('',#61306);
#2555=PLANE('',#61307);
#2556=PLANE('',#61308);
#2557=PLANE('',#61309);
#2558=PLANE('',#61310);
#2559=PLANE('',#61311);
#2560=PLANE('',#61312);
#2561=PLANE('',#61313);
#2562=PLANE('',#61314);
#2563=PLANE('',#61315);
#2564=PLANE('',#61316);
#2565=PLANE('',#61317);
#2566=PLANE('',#61318);
#2567=PLANE('',#61319);
#2568=PLANE('',#61320);
#2569=PLANE('',#61321);
#2570=PLANE('',#61322);
#2571=PLANE('',#61323);
#2572=PLANE('',#61324);
#2573=PLANE('',#61325);
#2574=PLANE('',#61326);
#2575=PLANE('',#61327);
#2576=PLANE('',#61328);
#2577=PLANE('',#61329);
#2578=PLANE('',#61330);
#2579=PLANE('',#61331);
#2580=PLANE('',#61332);
#2581=PLANE('',#61333);
#2582=PLANE('',#61334);
#2583=PLANE('',#61335);
#2584=PLANE('',#61336);
#2585=PLANE('',#61337);
#2586=PLANE('',#61338);
#2587=PLANE('',#61339);
#2588=PLANE('',#61340);
#2589=PLANE('',#61341);
#2590=PLANE('',#61342);
#2591=PLANE('',#61343);
#2592=PLANE('',#61344);
#2593=PLANE('',#61345);
#2594=PLANE('',#61346);
#2595=PLANE('',#61347);
#2596=PLANE('',#61348);
#2597=PLANE('',#61349);
#2598=PLANE('',#61350);
#2599=PLANE('',#61351);
#2600=PLANE('',#61352);
#2601=PLANE('',#61353);
#2602=PLANE('',#61354);
#2603=PLANE('',#61355);
#2604=PLANE('',#61356);
#2605=PLANE('',#61357);
#2606=PLANE('',#61358);
#2607=PLANE('',#61359);
#2608=PLANE('',#61360);
#2609=PLANE('',#61361);
#2610=PLANE('',#61362);
#2611=PLANE('',#61363);
#2612=PLANE('',#61364);
#2613=PLANE('',#61365);
#2614=PLANE('',#61366);
#2615=PLANE('',#61367);
#2616=PLANE('',#61368);
#2617=PLANE('',#61369);
#2618=PLANE('',#61370);
#2619=PLANE('',#61371);
#2620=PLANE('',#61372);
#2621=PLANE('',#61373);
#2622=PLANE('',#61374);
#2623=PLANE('',#61375);
#2624=PLANE('',#61376);
#2625=PLANE('',#61377);
#2626=PLANE('',#61378);
#2627=PLANE('',#61379);
#2628=PLANE('',#61380);
#2629=PLANE('',#61381);
#2630=PLANE('',#61382);
#2631=PLANE('',#61383);
#2632=PLANE('',#61384);
#2633=PLANE('',#61385);
#2634=PLANE('',#61386);
#2635=PLANE('',#61387);
#2636=PLANE('',#61388);
#2637=PLANE('',#61389);
#2638=PLANE('',#61390);
#2639=PLANE('',#61391);
#2640=PLANE('',#61392);
#2641=PLANE('',#61393);
#2642=PLANE('',#61394);
#2643=PLANE('',#61395);
#2644=PLANE('',#61396);
#2645=PLANE('',#61397);
#2646=PLANE('',#61398);
#2647=PLANE('',#61399);
#2648=PLANE('',#61400);
#2649=PLANE('',#61401);
#2650=PLANE('',#61402);
#2651=PLANE('',#61403);
#2652=PLANE('',#61404);
#2653=PLANE('',#61405);
#2654=PLANE('',#61406);
#2655=PLANE('',#61407);
#2656=PLANE('',#61408);
#2657=PLANE('',#61409);
#2658=PLANE('',#61410);
#2659=PLANE('',#61411);
#2660=PLANE('',#61412);
#2661=PLANE('',#61413);
#2662=PLANE('',#61414);
#2663=PLANE('',#61415);
#2664=PLANE('',#61416);
#2665=PLANE('',#61417);
#2666=PLANE('',#61418);
#2667=PLANE('',#61419);
#2668=PLANE('',#61420);
#2669=PLANE('',#61421);
#2670=PLANE('',#61422);
#2671=PLANE('',#61423);
#2672=PLANE('',#61424);
#2673=PLANE('',#61425);
#2674=PLANE('',#61426);
#2675=PLANE('',#61427);
#2676=PLANE('',#61428);
#2677=PLANE('',#61429);
#2678=PLANE('',#61430);
#2679=PLANE('',#61431);
#2680=PLANE('',#61432);
#2681=PLANE('',#61433);
#2682=PLANE('',#61434);
#2683=PLANE('',#61435);
#2684=PLANE('',#61436);
#2685=PLANE('',#61437);
#2686=PLANE('',#61438);
#2687=PLANE('',#61439);
#2688=PLANE('',#61440);
#2689=PLANE('',#61441);
#2690=PLANE('',#61442);
#2691=PLANE('',#61443);
#2692=PLANE('',#61444);
#2693=PLANE('',#61445);
#2694=PLANE('',#61446);
#2695=PLANE('',#61447);
#2696=PLANE('',#61448);
#2697=PLANE('',#61449);
#2698=PLANE('',#61450);
#2699=PLANE('',#61451);
#2700=PLANE('',#61452);
#2701=PLANE('',#61453);
#2702=PLANE('',#61454);
#2703=PLANE('',#61455);
#2704=PLANE('',#61456);
#2705=PLANE('',#61457);
#2706=PLANE('',#61458);
#2707=PLANE('',#61459);
#2708=PLANE('',#61460);
#2709=PLANE('',#61461);
#2710=PLANE('',#61462);
#2711=PLANE('',#61463);
#2712=PLANE('',#61464);
#2713=PLANE('',#61465);
#2714=PLANE('',#61466);
#2715=PLANE('',#61467);
#2716=PLANE('',#61468);
#2717=PLANE('',#61469);
#2718=PLANE('',#61470);
#2719=PLANE('',#61471);
#2720=PLANE('',#61472);
#2721=PLANE('',#61473);
#2722=PLANE('',#61474);
#2723=PLANE('',#61475);
#2724=PLANE('',#61476);
#2725=PLANE('',#61477);
#2726=PLANE('',#61478);
#2727=PLANE('',#61479);
#2728=PLANE('',#61480);
#2729=PLANE('',#61481);
#2730=PLANE('',#61482);
#2731=PLANE('',#61483);
#2732=PLANE('',#61484);
#2733=PLANE('',#61485);
#2734=PLANE('',#61486);
#2735=PLANE('',#61487);
#2736=PLANE('',#61488);
#2737=PLANE('',#61489);
#2738=PLANE('',#61490);
#2739=PLANE('',#61491);
#2740=PLANE('',#61492);
#2741=PLANE('',#61493);
#2742=PLANE('',#61494);
#2743=PLANE('',#61495);
#2744=PLANE('',#61496);
#2745=PLANE('',#61497);
#2746=PLANE('',#61498);
#2747=PLANE('',#61499);
#2748=PLANE('',#61500);
#2749=PLANE('',#61501);
#2750=PLANE('',#61502);
#2751=PLANE('',#61503);
#2752=PLANE('',#61504);
#2753=PLANE('',#61505);
#2754=PLANE('',#61506);
#2755=PLANE('',#61507);
#2756=PLANE('',#61508);
#2757=PLANE('',#61509);
#2758=PLANE('',#61510);
#2759=PLANE('',#61511);
#2760=PLANE('',#61512);
#2761=PLANE('',#61513);
#2762=PLANE('',#61514);
#2763=PLANE('',#61515);
#2764=PLANE('',#61516);
#2765=PLANE('',#61517);
#2766=PLANE('',#61518);
#2767=PLANE('',#61519);
#2768=PLANE('',#61520);
#2769=PLANE('',#61521);
#2770=PLANE('',#61522);
#2771=PLANE('',#61523);
#2772=PLANE('',#61524);
#2773=PLANE('',#61525);
#2774=PLANE('',#61526);
#2775=PLANE('',#61527);
#2776=PLANE('',#61528);
#2777=PLANE('',#61529);
#2778=PLANE('',#61530);
#2779=PLANE('',#61531);
#2780=PLANE('',#61532);
#2781=PLANE('',#61533);
#2782=PLANE('',#61534);
#2783=PLANE('',#61535);
#2784=PLANE('',#61536);
#2785=PLANE('',#61537);
#2786=PLANE('',#61538);
#2787=PLANE('',#61539);
#2788=PLANE('',#61540);
#2789=PLANE('',#61541);
#2790=PLANE('',#61542);
#2791=PLANE('',#61543);
#2792=PLANE('',#61544);
#2793=PLANE('',#61545);
#2794=PLANE('',#61546);
#2795=PLANE('',#61547);
#2796=PLANE('',#61548);
#2797=PLANE('',#61549);
#2798=PLANE('',#61550);
#2799=PLANE('',#61551);
#2800=PLANE('',#61552);
#2801=PLANE('',#61553);
#2802=PLANE('',#61554);
#2803=PLANE('',#61555);
#2804=PLANE('',#61556);
#2805=PLANE('',#61557);
#2806=PLANE('',#61558);
#2807=PLANE('',#61559);
#2808=PLANE('',#61560);
#2809=PLANE('',#61561);
#2810=PLANE('',#61562);
#2811=PLANE('',#61563);
#2812=PLANE('',#61564);
#2813=PLANE('',#61565);
#2814=PLANE('',#61566);
#2815=PLANE('',#61567);
#2816=PLANE('',#61568);
#2817=PLANE('',#61569);
#2818=PLANE('',#61570);
#2819=PLANE('',#61571);
#2820=PLANE('',#61572);
#2821=PLANE('',#61573);
#2822=PLANE('',#61574);
#2823=PLANE('',#61575);
#2824=PLANE('',#61576);
#2825=PLANE('',#61577);
#2826=PLANE('',#61578);
#2827=PLANE('',#61579);
#2828=PLANE('',#61580);
#2829=PLANE('',#61581);
#2830=PLANE('',#61582);
#2831=PLANE('',#61583);
#2832=PLANE('',#61584);
#2833=PLANE('',#61585);
#2834=PLANE('',#61586);
#2835=PLANE('',#61587);
#2836=PLANE('',#61588);
#2837=PLANE('',#61589);
#2838=PLANE('',#61590);
#2839=PLANE('',#61591);
#2840=PLANE('',#61592);
#2841=PLANE('',#61593);
#2842=PLANE('',#61594);
#2843=PLANE('',#61595);
#2844=PLANE('',#61596);
#2845=PLANE('',#61597);
#2846=PLANE('',#61598);
#2847=PLANE('',#61599);
#2848=PLANE('',#61600);
#2849=PLANE('',#61601);
#2850=PLANE('',#61602);
#2851=PLANE('',#61603);
#2852=PLANE('',#61604);
#2853=PLANE('',#61605);
#2854=PLANE('',#61606);
#2855=PLANE('',#61607);
#2856=PLANE('',#61608);
#2857=PLANE('',#61609);
#2858=PLANE('',#61610);
#2859=PLANE('',#61611);
#2860=PLANE('',#61612);
#2861=PLANE('',#61613);
#2862=PLANE('',#61614);
#2863=PLANE('',#61615);
#2864=PLANE('',#61616);
#2865=PLANE('',#61617);
#2866=PLANE('',#61618);
#2867=PLANE('',#61619);
#2868=PLANE('',#61620);
#2869=PLANE('',#61621);
#2870=PLANE('',#61622);
#2871=PLANE('',#61623);
#2872=PLANE('',#61624);
#2873=PLANE('',#61625);
#2874=PLANE('',#61626);
#2875=PLANE('',#61627);
#2876=PLANE('',#61628);
#2877=PLANE('',#61629);
#2878=PLANE('',#61630);
#2879=PLANE('',#61631);
#2880=PLANE('',#61632);
#2881=PLANE('',#61633);
#2882=PLANE('',#61634);
#2883=PLANE('',#61635);
#2884=PLANE('',#61636);
#2885=PLANE('',#61637);
#2886=PLANE('',#61638);
#2887=PLANE('',#61639);
#2888=PLANE('',#61640);
#2889=PLANE('',#61641);
#2890=PLANE('',#61642);
#2891=PLANE('',#61643);
#2892=PLANE('',#61644);
#2893=PLANE('',#61645);
#2894=PLANE('',#61646);
#2895=PLANE('',#61647);
#2896=PLANE('',#61648);
#2897=PLANE('',#61649);
#2898=PLANE('',#61650);
#2899=PLANE('',#61651);
#2900=PLANE('',#61652);
#2901=PLANE('',#61653);
#2902=PLANE('',#61654);
#2903=PLANE('',#61655);
#2904=PLANE('',#61656);
#2905=PLANE('',#61657);
#2906=PLANE('',#61658);
#2907=PLANE('',#61659);
#2908=PLANE('',#61660);
#2909=PLANE('',#61661);
#2910=PLANE('',#61662);
#2911=PLANE('',#61663);
#2912=PLANE('',#61664);
#2913=PLANE('',#61665);
#2914=PLANE('',#61668);
#2915=PLANE('',#61669);
#2916=PLANE('',#61670);
#2917=PLANE('',#61671);
#2918=PLANE('',#61688);
#2919=PLANE('',#61699);
#2920=PLANE('',#61704);
#2921=PLANE('',#61709);
#2922=PLANE('',#61714);
#2923=PLANE('',#61719);
#2924=PLANE('',#61724);
#2925=PLANE('',#61728);
#2926=PLANE('',#61748);
#2927=PLANE('',#61750);
#2928=PLANE('',#61751);
#2929=PLANE('',#61752);
#2930=PLANE('',#61753);
#2931=PLANE('',#61754);
#2932=PLANE('',#61755);
#2933=PLANE('',#61757);
#2934=PLANE('',#61758);
#2935=PLANE('',#61764);
#2936=PLANE('',#61765);
#2937=PLANE('',#61766);
#2938=PLANE('',#61767);
#2939=PLANE('',#61768);
#2940=PLANE('',#61769);
#2941=PLANE('',#61771);
#2942=PLANE('',#61772);
#2943=PLANE('',#61773);
#2944=PLANE('',#61774);
#2945=PLANE('',#61775);
#2946=PLANE('',#61776);
#2947=PLANE('',#61777);
#2948=PLANE('',#61778);
#2949=PLANE('',#61779);
#2950=PLANE('',#61780);
#2951=PLANE('',#61781);
#2952=PLANE('',#61782);
#2953=PLANE('',#61783);
#2954=PLANE('',#61784);
#2955=PLANE('',#61785);
#2956=PLANE('',#61786);
#2957=PLANE('',#61788);
#2958=PLANE('',#61789);
#2959=PLANE('',#61790);
#2960=PLANE('',#61791);
#2961=PLANE('',#61792);
#2962=PLANE('',#61793);
#2963=PLANE('',#61794);
#2964=PLANE('',#61795);
#2965=PLANE('',#61796);
#2966=PLANE('',#61797);
#2967=PLANE('',#61798);
#2968=PLANE('',#61799);
#2969=PLANE('',#61800);
#2970=PLANE('',#61801);
#2971=PLANE('',#61802);
#2972=PLANE('',#61803);
#2973=PLANE('',#61804);
#2974=PLANE('',#61806);
#2975=PLANE('',#61808);
#2976=PLANE('',#61810);
#2977=PLANE('',#61811);
#4025=FACE_OUTER_BOUND('',#7292,.T.);
#4026=FACE_OUTER_BOUND('',#7293,.T.);
#4027=FACE_OUTER_BOUND('',#7294,.T.);
#4028=FACE_OUTER_BOUND('',#7295,.T.);
#4029=FACE_OUTER_BOUND('',#7296,.T.);
#4030=FACE_OUTER_BOUND('',#7297,.T.);
#4031=FACE_OUTER_BOUND('',#7298,.T.);
#4032=FACE_OUTER_BOUND('',#7299,.T.);
#4033=FACE_OUTER_BOUND('',#7300,.T.);
#4034=FACE_OUTER_BOUND('',#7301,.T.);
#4035=FACE_OUTER_BOUND('',#7302,.T.);
#4036=FACE_OUTER_BOUND('',#7303,.T.);
#4037=FACE_OUTER_BOUND('',#7304,.T.);
#4038=FACE_OUTER_BOUND('',#7305,.T.);
#4039=FACE_OUTER_BOUND('',#7306,.T.);
#4040=FACE_OUTER_BOUND('',#7307,.T.);
#4041=FACE_OUTER_BOUND('',#7308,.T.);
#4042=FACE_OUTER_BOUND('',#7309,.T.);
#4043=FACE_OUTER_BOUND('',#7310,.T.);
#4044=FACE_OUTER_BOUND('',#7311,.T.);
#4045=FACE_OUTER_BOUND('',#7312,.T.);
#4046=FACE_OUTER_BOUND('',#7314,.T.);
#4047=FACE_OUTER_BOUND('',#7315,.T.);
#4048=FACE_OUTER_BOUND('',#7316,.T.);
#4049=FACE_OUTER_BOUND('',#7317,.T.);
#4050=FACE_OUTER_BOUND('',#7318,.T.);
#4051=FACE_OUTER_BOUND('',#7319,.T.);
#4052=FACE_OUTER_BOUND('',#7320,.T.);
#4053=FACE_OUTER_BOUND('',#7321,.T.);
#4054=FACE_OUTER_BOUND('',#7322,.T.);
#4055=FACE_OUTER_BOUND('',#7323,.T.);
#4056=FACE_OUTER_BOUND('',#7324,.T.);
#4057=FACE_OUTER_BOUND('',#7325,.T.);
#4058=FACE_OUTER_BOUND('',#7326,.T.);
#4059=FACE_OUTER_BOUND('',#7327,.T.);
#4060=FACE_OUTER_BOUND('',#7328,.T.);
#4061=FACE_OUTER_BOUND('',#7329,.T.);
#4062=FACE_OUTER_BOUND('',#7330,.T.);
#4063=FACE_OUTER_BOUND('',#7331,.T.);
#4064=FACE_OUTER_BOUND('',#7332,.T.);
#4065=FACE_OUTER_BOUND('',#7333,.T.);
#4066=FACE_OUTER_BOUND('',#7334,.T.);
#4067=FACE_OUTER_BOUND('',#7335,.T.);
#4068=FACE_OUTER_BOUND('',#7336,.T.);
#4069=FACE_OUTER_BOUND('',#7337,.T.);
#4070=FACE_OUTER_BOUND('',#7338,.T.);
#4071=FACE_OUTER_BOUND('',#7339,.T.);
#4072=FACE_OUTER_BOUND('',#7340,.T.);
#4073=FACE_OUTER_BOUND('',#7341,.T.);
#4074=FACE_OUTER_BOUND('',#7342,.T.);
#4075=FACE_OUTER_BOUND('',#7343,.T.);
#4076=FACE_OUTER_BOUND('',#7344,.T.);
#4077=FACE_OUTER_BOUND('',#7346,.T.);
#4078=FACE_OUTER_BOUND('',#7347,.T.);
#4079=FACE_OUTER_BOUND('',#7348,.T.);
#4080=FACE_OUTER_BOUND('',#7349,.T.);
#4081=FACE_OUTER_BOUND('',#7350,.T.);
#4082=FACE_OUTER_BOUND('',#7351,.T.);
#4083=FACE_OUTER_BOUND('',#7352,.T.);
#4084=FACE_OUTER_BOUND('',#7353,.T.);
#4085=FACE_OUTER_BOUND('',#7354,.T.);
#4086=FACE_OUTER_BOUND('',#7355,.T.);
#4087=FACE_OUTER_BOUND('',#7356,.T.);
#4088=FACE_OUTER_BOUND('',#7357,.T.);
#4089=FACE_OUTER_BOUND('',#7358,.T.);
#4090=FACE_OUTER_BOUND('',#7359,.T.);
#4091=FACE_OUTER_BOUND('',#7360,.T.);
#4092=FACE_OUTER_BOUND('',#7361,.T.);
#4093=FACE_OUTER_BOUND('',#7362,.T.);
#4094=FACE_OUTER_BOUND('',#7363,.T.);
#4095=FACE_OUTER_BOUND('',#7364,.T.);
#4096=FACE_OUTER_BOUND('',#7365,.T.);
#4097=FACE_OUTER_BOUND('',#7366,.T.);
#4098=FACE_OUTER_BOUND('',#7367,.T.);
#4099=FACE_OUTER_BOUND('',#7368,.T.);
#4100=FACE_OUTER_BOUND('',#7370,.T.);
#4101=FACE_OUTER_BOUND('',#7371,.T.);
#4102=FACE_OUTER_BOUND('',#7372,.T.);
#4103=FACE_OUTER_BOUND('',#7373,.T.);
#4104=FACE_OUTER_BOUND('',#7374,.T.);
#4105=FACE_OUTER_BOUND('',#7375,.T.);
#4106=FACE_OUTER_BOUND('',#7376,.T.);
#4107=FACE_OUTER_BOUND('',#7377,.T.);
#4108=FACE_OUTER_BOUND('',#7378,.T.);
#4109=FACE_OUTER_BOUND('',#7379,.T.);
#4110=FACE_OUTER_BOUND('',#7380,.T.);
#4111=FACE_OUTER_BOUND('',#7381,.T.);
#4112=FACE_OUTER_BOUND('',#7382,.T.);
#4113=FACE_OUTER_BOUND('',#7383,.T.);
#4114=FACE_OUTER_BOUND('',#7384,.T.);
#4115=FACE_OUTER_BOUND('',#7385,.T.);
#4116=FACE_OUTER_BOUND('',#7386,.T.);
#4117=FACE_OUTER_BOUND('',#7387,.T.);
#4118=FACE_OUTER_BOUND('',#7388,.T.);
#4119=FACE_OUTER_BOUND('',#7389,.T.);
#4120=FACE_OUTER_BOUND('',#7390,.T.);
#4121=FACE_OUTER_BOUND('',#7391,.T.);
#4122=FACE_OUTER_BOUND('',#7392,.T.);
#4123=FACE_OUTER_BOUND('',#7393,.T.);
#4124=FACE_OUTER_BOUND('',#7394,.T.);
#4125=FACE_OUTER_BOUND('',#7395,.T.);
#4126=FACE_OUTER_BOUND('',#7396,.T.);
#4127=FACE_OUTER_BOUND('',#7397,.T.);
#4128=FACE_OUTER_BOUND('',#7398,.T.);
#4129=FACE_OUTER_BOUND('',#7399,.T.);
#4130=FACE_OUTER_BOUND('',#7400,.T.);
#4131=FACE_OUTER_BOUND('',#7401,.T.);
#4132=FACE_OUTER_BOUND('',#7402,.T.);
#4133=FACE_OUTER_BOUND('',#7403,.T.);
#4134=FACE_OUTER_BOUND('',#7406,.T.);
#4135=FACE_OUTER_BOUND('',#7407,.T.);
#4136=FACE_OUTER_BOUND('',#7408,.T.);
#4137=FACE_OUTER_BOUND('',#7409,.T.);
#4138=FACE_OUTER_BOUND('',#7410,.T.);
#4139=FACE_OUTER_BOUND('',#7411,.T.);
#4140=FACE_OUTER_BOUND('',#7412,.T.);
#4141=FACE_OUTER_BOUND('',#7413,.T.);
#4142=FACE_OUTER_BOUND('',#7414,.T.);
#4143=FACE_OUTER_BOUND('',#7415,.T.);
#4144=FACE_OUTER_BOUND('',#7416,.T.);
#4145=FACE_OUTER_BOUND('',#7417,.T.);
#4146=FACE_OUTER_BOUND('',#7418,.T.);
#4147=FACE_OUTER_BOUND('',#7419,.T.);
#4148=FACE_OUTER_BOUND('',#7420,.T.);
#4149=FACE_OUTER_BOUND('',#7421,.T.);
#4150=FACE_OUTER_BOUND('',#7422,.T.);
#4151=FACE_OUTER_BOUND('',#7423,.T.);
#4152=FACE_OUTER_BOUND('',#7424,.T.);
#4153=FACE_OUTER_BOUND('',#7425,.T.);
#4154=FACE_OUTER_BOUND('',#7426,.T.);
#4155=FACE_OUTER_BOUND('',#7427,.T.);
#4156=FACE_OUTER_BOUND('',#7428,.T.);
#4157=FACE_OUTER_BOUND('',#7429,.T.);
#4158=FACE_OUTER_BOUND('',#7431,.T.);
#4159=FACE_OUTER_BOUND('',#7432,.T.);
#4160=FACE_OUTER_BOUND('',#7433,.T.);
#4161=FACE_OUTER_BOUND('',#7434,.T.);
#4162=FACE_OUTER_BOUND('',#7435,.T.);
#4163=FACE_OUTER_BOUND('',#7436,.T.);
#4164=FACE_OUTER_BOUND('',#7437,.T.);
#4165=FACE_OUTER_BOUND('',#7438,.T.);
#4166=FACE_OUTER_BOUND('',#7439,.T.);
#4167=FACE_OUTER_BOUND('',#7440,.T.);
#4168=FACE_OUTER_BOUND('',#7441,.T.);
#4169=FACE_OUTER_BOUND('',#7442,.T.);
#4170=FACE_OUTER_BOUND('',#7443,.T.);
#4171=FACE_OUTER_BOUND('',#7444,.T.);
#4172=FACE_OUTER_BOUND('',#7445,.T.);
#4173=FACE_OUTER_BOUND('',#7446,.T.);
#4174=FACE_OUTER_BOUND('',#7447,.T.);
#4175=FACE_OUTER_BOUND('',#7448,.T.);
#4176=FACE_OUTER_BOUND('',#7449,.T.);
#4177=FACE_OUTER_BOUND('',#7450,.T.);
#4178=FACE_OUTER_BOUND('',#7451,.T.);
#4179=FACE_OUTER_BOUND('',#7452,.T.);
#4180=FACE_OUTER_BOUND('',#7453,.T.);
#4181=FACE_OUTER_BOUND('',#7454,.T.);
#4182=FACE_OUTER_BOUND('',#7455,.T.);
#4183=FACE_OUTER_BOUND('',#7456,.T.);
#4184=FACE_OUTER_BOUND('',#7457,.T.);
#4185=FACE_OUTER_BOUND('',#7458,.T.);
#4186=FACE_OUTER_BOUND('',#7459,.T.);
#4187=FACE_OUTER_BOUND('',#7460,.T.);
#4188=FACE_OUTER_BOUND('',#7461,.T.);
#4189=FACE_OUTER_BOUND('',#7462,.T.);
#4190=FACE_OUTER_BOUND('',#7463,.T.);
#4191=FACE_OUTER_BOUND('',#7464,.T.);
#4192=FACE_OUTER_BOUND('',#7466,.T.);
#4193=FACE_OUTER_BOUND('',#7467,.T.);
#4194=FACE_OUTER_BOUND('',#7468,.T.);
#4195=FACE_OUTER_BOUND('',#7469,.T.);
#4196=FACE_OUTER_BOUND('',#7470,.T.);
#4197=FACE_OUTER_BOUND('',#7471,.T.);
#4198=FACE_OUTER_BOUND('',#7472,.T.);
#4199=FACE_OUTER_BOUND('',#7473,.T.);
#4200=FACE_OUTER_BOUND('',#7474,.T.);
#4201=FACE_OUTER_BOUND('',#7475,.T.);
#4202=FACE_OUTER_BOUND('',#7476,.T.);
#4203=FACE_OUTER_BOUND('',#7477,.T.);
#4204=FACE_OUTER_BOUND('',#7478,.T.);
#4205=FACE_OUTER_BOUND('',#7479,.T.);
#4206=FACE_OUTER_BOUND('',#7480,.T.);
#4207=FACE_OUTER_BOUND('',#7481,.T.);
#4208=FACE_OUTER_BOUND('',#7482,.T.);
#4209=FACE_OUTER_BOUND('',#7483,.T.);
#4210=FACE_OUTER_BOUND('',#7484,.T.);
#4211=FACE_OUTER_BOUND('',#7485,.T.);
#4212=FACE_OUTER_BOUND('',#7486,.T.);
#4213=FACE_OUTER_BOUND('',#7487,.T.);
#4214=FACE_OUTER_BOUND('',#7488,.T.);
#4215=FACE_OUTER_BOUND('',#7489,.T.);
#4216=FACE_OUTER_BOUND('',#7490,.T.);
#4217=FACE_OUTER_BOUND('',#7491,.T.);
#4218=FACE_OUTER_BOUND('',#7492,.T.);
#4219=FACE_OUTER_BOUND('',#7493,.T.);
#4220=FACE_OUTER_BOUND('',#7494,.T.);
#4221=FACE_OUTER_BOUND('',#7496,.T.);
#4222=FACE_OUTER_BOUND('',#7497,.T.);
#4223=FACE_OUTER_BOUND('',#7498,.T.);
#4224=FACE_OUTER_BOUND('',#7499,.T.);
#4225=FACE_OUTER_BOUND('',#7500,.T.);
#4226=FACE_OUTER_BOUND('',#7501,.T.);
#4227=FACE_OUTER_BOUND('',#7502,.T.);
#4228=FACE_OUTER_BOUND('',#7503,.T.);
#4229=FACE_OUTER_BOUND('',#7504,.T.);
#4230=FACE_OUTER_BOUND('',#7505,.T.);
#4231=FACE_OUTER_BOUND('',#7506,.T.);
#4232=FACE_OUTER_BOUND('',#7507,.T.);
#4233=FACE_OUTER_BOUND('',#7508,.T.);
#4234=FACE_OUTER_BOUND('',#7509,.T.);
#4235=FACE_OUTER_BOUND('',#7510,.T.);
#4236=FACE_OUTER_BOUND('',#7511,.T.);
#4237=FACE_OUTER_BOUND('',#7512,.T.);
#4238=FACE_OUTER_BOUND('',#7513,.T.);
#4239=FACE_OUTER_BOUND('',#7514,.T.);
#4240=FACE_OUTER_BOUND('',#7515,.T.);
#4241=FACE_OUTER_BOUND('',#7516,.T.);
#4242=FACE_OUTER_BOUND('',#7517,.T.);
#4243=FACE_OUTER_BOUND('',#7518,.T.);
#4244=FACE_OUTER_BOUND('',#7520,.T.);
#4245=FACE_OUTER_BOUND('',#7521,.T.);
#4246=FACE_OUTER_BOUND('',#7522,.T.);
#4247=FACE_OUTER_BOUND('',#7523,.T.);
#4248=FACE_OUTER_BOUND('',#7524,.T.);
#4249=FACE_OUTER_BOUND('',#7525,.T.);
#4250=FACE_OUTER_BOUND('',#7526,.T.);
#4251=FACE_OUTER_BOUND('',#7527,.T.);
#4252=FACE_OUTER_BOUND('',#7528,.T.);
#4253=FACE_OUTER_BOUND('',#7529,.T.);
#4254=FACE_OUTER_BOUND('',#7530,.T.);
#4255=FACE_OUTER_BOUND('',#7531,.T.);
#4256=FACE_OUTER_BOUND('',#7532,.T.);
#4257=FACE_OUTER_BOUND('',#7533,.T.);
#4258=FACE_OUTER_BOUND('',#7534,.T.);
#4259=FACE_OUTER_BOUND('',#7535,.T.);
#4260=FACE_OUTER_BOUND('',#7536,.T.);
#4261=FACE_OUTER_BOUND('',#7537,.T.);
#4262=FACE_OUTER_BOUND('',#7538,.T.);
#4263=FACE_OUTER_BOUND('',#7539,.T.);
#4264=FACE_OUTER_BOUND('',#7540,.T.);
#4265=FACE_OUTER_BOUND('',#7541,.T.);
#4266=FACE_OUTER_BOUND('',#7542,.T.);
#4267=FACE_OUTER_BOUND('',#7543,.T.);
#4268=FACE_OUTER_BOUND('',#7544,.T.);
#4269=FACE_OUTER_BOUND('',#7545,.T.);
#4270=FACE_OUTER_BOUND('',#7546,.T.);
#4271=FACE_OUTER_BOUND('',#7547,.T.);
#4272=FACE_OUTER_BOUND('',#7548,.T.);
#4273=FACE_OUTER_BOUND('',#7549,.T.);
#4274=FACE_OUTER_BOUND('',#7550,.T.);
#4275=FACE_OUTER_BOUND('',#7551,.T.);
#4276=FACE_OUTER_BOUND('',#7552,.T.);
#4277=FACE_OUTER_BOUND('',#7553,.T.);
#4278=FACE_OUTER_BOUND('',#7554,.T.);
#4279=FACE_OUTER_BOUND('',#7555,.T.);
#4280=FACE_OUTER_BOUND('',#7556,.T.);
#4281=FACE_OUTER_BOUND('',#7557,.T.);
#4282=FACE_OUTER_BOUND('',#7558,.T.);
#4283=FACE_OUTER_BOUND('',#7559,.T.);
#4284=FACE_OUTER_BOUND('',#7560,.T.);
#4285=FACE_OUTER_BOUND('',#7561,.T.);
#4286=FACE_OUTER_BOUND('',#7562,.T.);
#4287=FACE_OUTER_BOUND('',#7563,.T.);
#4288=FACE_OUTER_BOUND('',#7564,.T.);
#4289=FACE_OUTER_BOUND('',#7566,.T.);
#4290=FACE_OUTER_BOUND('',#7567,.T.);
#4291=FACE_OUTER_BOUND('',#7568,.T.);
#4292=FACE_OUTER_BOUND('',#7569,.T.);
#4293=FACE_OUTER_BOUND('',#7570,.T.);
#4294=FACE_OUTER_BOUND('',#7571,.T.);
#4295=FACE_OUTER_BOUND('',#7572,.T.);
#4296=FACE_OUTER_BOUND('',#7573,.T.);
#4297=FACE_OUTER_BOUND('',#7574,.T.);
#4298=FACE_OUTER_BOUND('',#7575,.T.);
#4299=FACE_OUTER_BOUND('',#7576,.T.);
#4300=FACE_OUTER_BOUND('',#7577,.T.);
#4301=FACE_OUTER_BOUND('',#7578,.T.);
#4302=FACE_OUTER_BOUND('',#7579,.T.);
#4303=FACE_OUTER_BOUND('',#7580,.T.);
#4304=FACE_OUTER_BOUND('',#7582,.T.);
#4305=FACE_OUTER_BOUND('',#7583,.T.);
#4306=FACE_OUTER_BOUND('',#7584,.T.);
#4307=FACE_OUTER_BOUND('',#7585,.T.);
#4308=FACE_OUTER_BOUND('',#7586,.T.);
#4309=FACE_OUTER_BOUND('',#7587,.T.);
#4310=FACE_OUTER_BOUND('',#7588,.T.);
#4311=FACE_OUTER_BOUND('',#7589,.T.);
#4312=FACE_OUTER_BOUND('',#7590,.T.);
#4313=FACE_OUTER_BOUND('',#7591,.T.);
#4314=FACE_OUTER_BOUND('',#7592,.T.);
#4315=FACE_OUTER_BOUND('',#7593,.T.);
#4316=FACE_OUTER_BOUND('',#7594,.T.);
#4317=FACE_OUTER_BOUND('',#7595,.T.);
#4318=FACE_OUTER_BOUND('',#7596,.T.);
#4319=FACE_OUTER_BOUND('',#7597,.T.);
#4320=FACE_OUTER_BOUND('',#7598,.T.);
#4321=FACE_OUTER_BOUND('',#7599,.T.);
#4322=FACE_OUTER_BOUND('',#7600,.T.);
#4323=FACE_OUTER_BOUND('',#7601,.T.);
#4324=FACE_OUTER_BOUND('',#7602,.T.);
#4325=FACE_OUTER_BOUND('',#7603,.T.);
#4326=FACE_OUTER_BOUND('',#7604,.T.);
#4327=FACE_OUTER_BOUND('',#7606,.T.);
#4328=FACE_OUTER_BOUND('',#7607,.T.);
#4329=FACE_OUTER_BOUND('',#7608,.T.);
#4330=FACE_OUTER_BOUND('',#7609,.T.);
#4331=FACE_OUTER_BOUND('',#7610,.T.);
#4332=FACE_OUTER_BOUND('',#7611,.T.);
#4333=FACE_OUTER_BOUND('',#7612,.T.);
#4334=FACE_OUTER_BOUND('',#7613,.T.);
#4335=FACE_OUTER_BOUND('',#7614,.T.);
#4336=FACE_OUTER_BOUND('',#7615,.T.);
#4337=FACE_OUTER_BOUND('',#7616,.T.);
#4338=FACE_OUTER_BOUND('',#7617,.T.);
#4339=FACE_OUTER_BOUND('',#7618,.T.);
#4340=FACE_OUTER_BOUND('',#7619,.T.);
#4341=FACE_OUTER_BOUND('',#7620,.T.);
#4342=FACE_OUTER_BOUND('',#7621,.T.);
#4343=FACE_OUTER_BOUND('',#7622,.T.);
#4344=FACE_OUTER_BOUND('',#7623,.T.);
#4345=FACE_OUTER_BOUND('',#7624,.T.);
#4346=FACE_OUTER_BOUND('',#7625,.T.);
#4347=FACE_OUTER_BOUND('',#7626,.T.);
#4348=FACE_OUTER_BOUND('',#7627,.T.);
#4349=FACE_OUTER_BOUND('',#7628,.T.);
#4350=FACE_OUTER_BOUND('',#7629,.T.);
#4351=FACE_OUTER_BOUND('',#7630,.T.);
#4352=FACE_OUTER_BOUND('',#7631,.T.);
#4353=FACE_OUTER_BOUND('',#7632,.T.);
#4354=FACE_OUTER_BOUND('',#7633,.T.);
#4355=FACE_OUTER_BOUND('',#7634,.T.);
#4356=FACE_OUTER_BOUND('',#7635,.T.);
#4357=FACE_OUTER_BOUND('',#7636,.T.);
#4358=FACE_OUTER_BOUND('',#7637,.T.);
#4359=FACE_OUTER_BOUND('',#7638,.T.);
#4360=FACE_OUTER_BOUND('',#7639,.T.);
#4361=FACE_OUTER_BOUND('',#7640,.T.);
#4362=FACE_OUTER_BOUND('',#7641,.T.);
#4363=FACE_OUTER_BOUND('',#7642,.T.);
#4364=FACE_OUTER_BOUND('',#7643,.T.);
#4365=FACE_OUTER_BOUND('',#7644,.T.);
#4366=FACE_OUTER_BOUND('',#7645,.T.);
#4367=FACE_OUTER_BOUND('',#7646,.T.);
#4368=FACE_OUTER_BOUND('',#7647,.T.);
#4369=FACE_OUTER_BOUND('',#7648,.T.);
#4370=FACE_OUTER_BOUND('',#7649,.T.);
#4371=FACE_OUTER_BOUND('',#7650,.T.);
#4372=FACE_OUTER_BOUND('',#7651,.T.);
#4373=FACE_OUTER_BOUND('',#7652,.T.);
#4374=FACE_OUTER_BOUND('',#7653,.T.);
#4375=FACE_OUTER_BOUND('',#7654,.T.);
#4376=FACE_OUTER_BOUND('',#7655,.T.);
#4377=FACE_OUTER_BOUND('',#7656,.T.);
#4378=FACE_OUTER_BOUND('',#7657,.T.);
#4379=FACE_OUTER_BOUND('',#7658,.T.);
#4380=FACE_OUTER_BOUND('',#7660,.T.);
#4381=FACE_OUTER_BOUND('',#7661,.T.);
#4382=FACE_OUTER_BOUND('',#7662,.T.);
#4383=FACE_OUTER_BOUND('',#7663,.T.);
#4384=FACE_OUTER_BOUND('',#7664,.T.);
#4385=FACE_OUTER_BOUND('',#7665,.T.);
#4386=FACE_OUTER_BOUND('',#7666,.T.);
#4387=FACE_OUTER_BOUND('',#7667,.T.);
#4388=FACE_OUTER_BOUND('',#7668,.T.);
#4389=FACE_OUTER_BOUND('',#7669,.T.);
#4390=FACE_OUTER_BOUND('',#7670,.T.);
#4391=FACE_OUTER_BOUND('',#7671,.T.);
#4392=FACE_OUTER_BOUND('',#7672,.T.);
#4393=FACE_OUTER_BOUND('',#7673,.T.);
#4394=FACE_OUTER_BOUND('',#7674,.T.);
#4395=FACE_OUTER_BOUND('',#7675,.T.);
#4396=FACE_OUTER_BOUND('',#7676,.T.);
#4397=FACE_OUTER_BOUND('',#7677,.T.);
#4398=FACE_OUTER_BOUND('',#7678,.T.);
#4399=FACE_OUTER_BOUND('',#7679,.T.);
#4400=FACE_OUTER_BOUND('',#7680,.T.);
#4401=FACE_OUTER_BOUND('',#7681,.T.);
#4402=FACE_OUTER_BOUND('',#7682,.T.);
#4403=FACE_OUTER_BOUND('',#7683,.T.);
#4404=FACE_OUTER_BOUND('',#7684,.T.);
#4405=FACE_OUTER_BOUND('',#7685,.T.);
#4406=FACE_OUTER_BOUND('',#7686,.T.);
#4407=FACE_OUTER_BOUND('',#7687,.T.);
#4408=FACE_OUTER_BOUND('',#7688,.T.);
#4409=FACE_OUTER_BOUND('',#7689,.T.);
#4410=FACE_OUTER_BOUND('',#7690,.T.);
#4411=FACE_OUTER_BOUND('',#7691,.T.);
#4412=FACE_OUTER_BOUND('',#7692,.T.);
#4413=FACE_OUTER_BOUND('',#7693,.T.);
#4414=FACE_OUTER_BOUND('',#7694,.T.);
#4415=FACE_OUTER_BOUND('',#7695,.T.);
#4416=FACE_OUTER_BOUND('',#7696,.T.);
#4417=FACE_OUTER_BOUND('',#7697,.T.);
#4418=FACE_OUTER_BOUND('',#7698,.T.);
#4419=FACE_OUTER_BOUND('',#7699,.T.);
#4420=FACE_OUTER_BOUND('',#7700,.T.);
#4421=FACE_OUTER_BOUND('',#7701,.T.);
#4422=FACE_OUTER_BOUND('',#7702,.T.);
#4423=FACE_OUTER_BOUND('',#7703,.T.);
#4424=FACE_OUTER_BOUND('',#7704,.T.);
#4425=FACE_OUTER_BOUND('',#7706,.T.);
#4426=FACE_OUTER_BOUND('',#7707,.T.);
#4427=FACE_OUTER_BOUND('',#7708,.T.);
#4428=FACE_OUTER_BOUND('',#7709,.T.);
#4429=FACE_OUTER_BOUND('',#7710,.T.);
#4430=FACE_OUTER_BOUND('',#7711,.T.);
#4431=FACE_OUTER_BOUND('',#7712,.T.);
#4432=FACE_OUTER_BOUND('',#7713,.T.);
#4433=FACE_OUTER_BOUND('',#7714,.T.);
#4434=FACE_OUTER_BOUND('',#7715,.T.);
#4435=FACE_OUTER_BOUND('',#7716,.T.);
#4436=FACE_OUTER_BOUND('',#7717,.T.);
#4437=FACE_OUTER_BOUND('',#7718,.T.);
#4438=FACE_OUTER_BOUND('',#7719,.T.);
#4439=FACE_OUTER_BOUND('',#7720,.T.);
#4440=FACE_OUTER_BOUND('',#7721,.T.);
#4441=FACE_OUTER_BOUND('',#7722,.T.);
#4442=FACE_OUTER_BOUND('',#7723,.T.);
#4443=FACE_OUTER_BOUND('',#7724,.T.);
#4444=FACE_OUTER_BOUND('',#7725,.T.);
#4445=FACE_OUTER_BOUND('',#7726,.T.);
#4446=FACE_OUTER_BOUND('',#7727,.T.);
#4447=FACE_OUTER_BOUND('',#7728,.T.);
#4448=FACE_OUTER_BOUND('',#7729,.T.);
#4449=FACE_OUTER_BOUND('',#7730,.T.);
#4450=FACE_OUTER_BOUND('',#7731,.T.);
#4451=FACE_OUTER_BOUND('',#7732,.T.);
#4452=FACE_OUTER_BOUND('',#7733,.T.);
#4453=FACE_OUTER_BOUND('',#7734,.T.);
#4454=FACE_OUTER_BOUND('',#7735,.T.);
#4455=FACE_OUTER_BOUND('',#7736,.T.);
#4456=FACE_OUTER_BOUND('',#7737,.T.);
#4457=FACE_OUTER_BOUND('',#7739,.T.);
#4458=FACE_OUTER_BOUND('',#7740,.T.);
#4459=FACE_OUTER_BOUND('',#7741,.T.);
#4460=FACE_OUTER_BOUND('',#7742,.T.);
#4461=FACE_OUTER_BOUND('',#7743,.T.);
#4462=FACE_OUTER_BOUND('',#7744,.T.);
#4463=FACE_OUTER_BOUND('',#7745,.T.);
#4464=FACE_OUTER_BOUND('',#7746,.T.);
#4465=FACE_OUTER_BOUND('',#7747,.T.);
#4466=FACE_OUTER_BOUND('',#7748,.T.);
#4467=FACE_OUTER_BOUND('',#7749,.T.);
#4468=FACE_OUTER_BOUND('',#7750,.T.);
#4469=FACE_OUTER_BOUND('',#7751,.T.);
#4470=FACE_OUTER_BOUND('',#7752,.T.);
#4471=FACE_OUTER_BOUND('',#7753,.T.);
#4472=FACE_OUTER_BOUND('',#7754,.T.);
#4473=FACE_OUTER_BOUND('',#7755,.T.);
#4474=FACE_OUTER_BOUND('',#7756,.T.);
#4475=FACE_OUTER_BOUND('',#7757,.T.);
#4476=FACE_OUTER_BOUND('',#7758,.T.);
#4477=FACE_OUTER_BOUND('',#7759,.T.);
#4478=FACE_OUTER_BOUND('',#7760,.T.);
#4479=FACE_OUTER_BOUND('',#7762,.T.);
#4480=FACE_OUTER_BOUND('',#7763,.T.);
#4481=FACE_OUTER_BOUND('',#7764,.T.);
#4482=FACE_OUTER_BOUND('',#7765,.T.);
#4483=FACE_OUTER_BOUND('',#7766,.T.);
#4484=FACE_OUTER_BOUND('',#7767,.T.);
#4485=FACE_OUTER_BOUND('',#7768,.T.);
#4486=FACE_OUTER_BOUND('',#7769,.T.);
#4487=FACE_OUTER_BOUND('',#7770,.T.);
#4488=FACE_OUTER_BOUND('',#7771,.T.);
#4489=FACE_OUTER_BOUND('',#7772,.T.);
#4490=FACE_OUTER_BOUND('',#7773,.T.);
#4491=FACE_OUTER_BOUND('',#7774,.T.);
#4492=FACE_OUTER_BOUND('',#7775,.T.);
#4493=FACE_OUTER_BOUND('',#7776,.T.);
#4494=FACE_OUTER_BOUND('',#7777,.T.);
#4495=FACE_OUTER_BOUND('',#7778,.T.);
#4496=FACE_OUTER_BOUND('',#7779,.T.);
#4497=FACE_OUTER_BOUND('',#7780,.T.);
#4498=FACE_OUTER_BOUND('',#7781,.T.);
#4499=FACE_OUTER_BOUND('',#7782,.T.);
#4500=FACE_OUTER_BOUND('',#7783,.T.);
#4501=FACE_OUTER_BOUND('',#7784,.T.);
#4502=FACE_OUTER_BOUND('',#7785,.T.);
#4503=FACE_OUTER_BOUND('',#7786,.T.);
#4504=FACE_OUTER_BOUND('',#7787,.T.);
#4505=FACE_OUTER_BOUND('',#7788,.T.);
#4506=FACE_OUTER_BOUND('',#7789,.T.);
#4507=FACE_OUTER_BOUND('',#7790,.T.);
#4508=FACE_OUTER_BOUND('',#7791,.T.);
#4509=FACE_OUTER_BOUND('',#7792,.T.);
#4510=FACE_OUTER_BOUND('',#7793,.T.);
#4511=FACE_OUTER_BOUND('',#7795,.T.);
#4512=FACE_OUTER_BOUND('',#7796,.T.);
#4513=FACE_OUTER_BOUND('',#7797,.T.);
#4514=FACE_OUTER_BOUND('',#7798,.T.);
#4515=FACE_OUTER_BOUND('',#7799,.T.);
#4516=FACE_OUTER_BOUND('',#7800,.T.);
#4517=FACE_OUTER_BOUND('',#7801,.T.);
#4518=FACE_OUTER_BOUND('',#7802,.T.);
#4519=FACE_OUTER_BOUND('',#7803,.T.);
#4520=FACE_OUTER_BOUND('',#7804,.T.);
#4521=FACE_OUTER_BOUND('',#7805,.T.);
#4522=FACE_OUTER_BOUND('',#7806,.T.);
#4523=FACE_OUTER_BOUND('',#7807,.T.);
#4524=FACE_OUTER_BOUND('',#7808,.T.);
#4525=FACE_OUTER_BOUND('',#7809,.T.);
#4526=FACE_OUTER_BOUND('',#7810,.T.);
#4527=FACE_OUTER_BOUND('',#7811,.T.);
#4528=FACE_OUTER_BOUND('',#7812,.T.);
#4529=FACE_OUTER_BOUND('',#7813,.T.);
#4530=FACE_OUTER_BOUND('',#7814,.T.);
#4531=FACE_OUTER_BOUND('',#7815,.T.);
#4532=FACE_OUTER_BOUND('',#7816,.T.);
#4533=FACE_OUTER_BOUND('',#7817,.T.);
#4534=FACE_OUTER_BOUND('',#7818,.T.);
#4535=FACE_OUTER_BOUND('',#7819,.T.);
#4536=FACE_OUTER_BOUND('',#7820,.T.);
#4537=FACE_OUTER_BOUND('',#7821,.T.);
#4538=FACE_OUTER_BOUND('',#7822,.T.);
#4539=FACE_OUTER_BOUND('',#7823,.T.);
#4540=FACE_OUTER_BOUND('',#7824,.T.);
#4541=FACE_OUTER_BOUND('',#7825,.T.);
#4542=FACE_OUTER_BOUND('',#7826,.T.);
#4543=FACE_OUTER_BOUND('',#7827,.T.);
#4544=FACE_OUTER_BOUND('',#7828,.T.);
#4545=FACE_OUTER_BOUND('',#7829,.T.);
#4546=FACE_OUTER_BOUND('',#7830,.T.);
#4547=FACE_OUTER_BOUND('',#7831,.T.);
#4548=FACE_OUTER_BOUND('',#7832,.T.);
#4549=FACE_OUTER_BOUND('',#7833,.T.);
#4550=FACE_OUTER_BOUND('',#7834,.T.);
#4551=FACE_OUTER_BOUND('',#7835,.T.);
#4552=FACE_OUTER_BOUND('',#7836,.T.);
#4553=FACE_OUTER_BOUND('',#7837,.T.);
#4554=FACE_OUTER_BOUND('',#7838,.T.);
#4555=FACE_OUTER_BOUND('',#7839,.T.);
#4556=FACE_OUTER_BOUND('',#7841,.T.);
#4557=FACE_OUTER_BOUND('',#7842,.T.);
#4558=FACE_OUTER_BOUND('',#7843,.T.);
#4559=FACE_OUTER_BOUND('',#7844,.T.);
#4560=FACE_OUTER_BOUND('',#7845,.T.);
#4561=FACE_OUTER_BOUND('',#7846,.T.);
#4562=FACE_OUTER_BOUND('',#7847,.T.);
#4563=FACE_OUTER_BOUND('',#7848,.T.);
#4564=FACE_OUTER_BOUND('',#7849,.T.);
#4565=FACE_OUTER_BOUND('',#7850,.T.);
#4566=FACE_OUTER_BOUND('',#7851,.T.);
#4567=FACE_OUTER_BOUND('',#7852,.T.);
#4568=FACE_OUTER_BOUND('',#7853,.T.);
#4569=FACE_OUTER_BOUND('',#7854,.T.);
#4570=FACE_OUTER_BOUND('',#7855,.T.);
#4571=FACE_OUTER_BOUND('',#7856,.T.);
#4572=FACE_OUTER_BOUND('',#7857,.T.);
#4573=FACE_OUTER_BOUND('',#7858,.T.);
#4574=FACE_OUTER_BOUND('',#7859,.T.);
#4575=FACE_OUTER_BOUND('',#7860,.T.);
#4576=FACE_OUTER_BOUND('',#7861,.T.);
#4577=FACE_OUTER_BOUND('',#7862,.T.);
#4578=FACE_OUTER_BOUND('',#7863,.T.);
#4579=FACE_OUTER_BOUND('',#7864,.T.);
#4580=FACE_OUTER_BOUND('',#7865,.T.);
#4581=FACE_OUTER_BOUND('',#7866,.T.);
#4582=FACE_OUTER_BOUND('',#7867,.T.);
#4583=FACE_OUTER_BOUND('',#7868,.T.);
#4584=FACE_OUTER_BOUND('',#7869,.T.);
#4585=FACE_OUTER_BOUND('',#7870,.T.);
#4586=FACE_OUTER_BOUND('',#7871,.T.);
#4587=FACE_OUTER_BOUND('',#7872,.T.);
#4588=FACE_OUTER_BOUND('',#7873,.T.);
#4589=FACE_OUTER_BOUND('',#7874,.T.);
#4590=FACE_OUTER_BOUND('',#7875,.T.);
#4591=FACE_OUTER_BOUND('',#7876,.T.);
#4592=FACE_OUTER_BOUND('',#7877,.T.);
#4593=FACE_OUTER_BOUND('',#7878,.T.);
#4594=FACE_OUTER_BOUND('',#7879,.T.);
#4595=FACE_OUTER_BOUND('',#7880,.T.);
#4596=FACE_OUTER_BOUND('',#7881,.T.);
#4597=FACE_OUTER_BOUND('',#7882,.T.);
#4598=FACE_OUTER_BOUND('',#7883,.T.);
#4599=FACE_OUTER_BOUND('',#7884,.T.);
#4600=FACE_OUTER_BOUND('',#7885,.T.);
#4601=FACE_OUTER_BOUND('',#7886,.T.);
#4602=FACE_OUTER_BOUND('',#7887,.T.);
#4603=FACE_OUTER_BOUND('',#7888,.T.);
#4604=FACE_OUTER_BOUND('',#7889,.T.);
#4605=FACE_OUTER_BOUND('',#7890,.T.);
#4606=FACE_OUTER_BOUND('',#7891,.T.);
#4607=FACE_OUTER_BOUND('',#7892,.T.);
#4608=FACE_OUTER_BOUND('',#7893,.T.);
#4609=FACE_OUTER_BOUND('',#7895,.T.);
#4610=FACE_OUTER_BOUND('',#7896,.T.);
#4611=FACE_OUTER_BOUND('',#7897,.T.);
#4612=FACE_OUTER_BOUND('',#7898,.T.);
#4613=FACE_OUTER_BOUND('',#7899,.T.);
#4614=FACE_OUTER_BOUND('',#7900,.T.);
#4615=FACE_OUTER_BOUND('',#7901,.T.);
#4616=FACE_OUTER_BOUND('',#7902,.T.);
#4617=FACE_OUTER_BOUND('',#7903,.T.);
#4618=FACE_OUTER_BOUND('',#7904,.T.);
#4619=FACE_OUTER_BOUND('',#7905,.T.);
#4620=FACE_OUTER_BOUND('',#7906,.T.);
#4621=FACE_OUTER_BOUND('',#7907,.T.);
#4622=FACE_OUTER_BOUND('',#7908,.T.);
#4623=FACE_OUTER_BOUND('',#7909,.T.);
#4624=FACE_OUTER_BOUND('',#7911,.T.);
#4625=FACE_OUTER_BOUND('',#7912,.T.);
#4626=FACE_OUTER_BOUND('',#7913,.T.);
#4627=FACE_OUTER_BOUND('',#7914,.T.);
#4628=FACE_OUTER_BOUND('',#7915,.T.);
#4629=FACE_OUTER_BOUND('',#7916,.T.);
#4630=FACE_OUTER_BOUND('',#7917,.T.);
#4631=FACE_OUTER_BOUND('',#7918,.T.);
#4632=FACE_OUTER_BOUND('',#7919,.T.);
#4633=FACE_OUTER_BOUND('',#7920,.T.);
#4634=FACE_OUTER_BOUND('',#7921,.T.);
#4635=FACE_OUTER_BOUND('',#7922,.T.);
#4636=FACE_OUTER_BOUND('',#7923,.T.);
#4637=FACE_OUTER_BOUND('',#7924,.T.);
#4638=FACE_OUTER_BOUND('',#7925,.T.);
#4639=FACE_OUTER_BOUND('',#7926,.T.);
#4640=FACE_OUTER_BOUND('',#7927,.T.);
#4641=FACE_OUTER_BOUND('',#7928,.T.);
#4642=FACE_OUTER_BOUND('',#7929,.T.);
#4643=FACE_OUTER_BOUND('',#7930,.T.);
#4644=FACE_OUTER_BOUND('',#7931,.T.);
#4645=FACE_OUTER_BOUND('',#7932,.T.);
#4646=FACE_OUTER_BOUND('',#7933,.T.);
#4647=FACE_OUTER_BOUND('',#7935,.T.);
#4648=FACE_OUTER_BOUND('',#7936,.T.);
#4649=FACE_OUTER_BOUND('',#7937,.T.);
#4650=FACE_OUTER_BOUND('',#7938,.T.);
#4651=FACE_OUTER_BOUND('',#7939,.T.);
#4652=FACE_OUTER_BOUND('',#7940,.T.);
#4653=FACE_OUTER_BOUND('',#7941,.T.);
#4654=FACE_OUTER_BOUND('',#7942,.T.);
#4655=FACE_OUTER_BOUND('',#7943,.T.);
#4656=FACE_OUTER_BOUND('',#7944,.T.);
#4657=FACE_OUTER_BOUND('',#7945,.T.);
#4658=FACE_OUTER_BOUND('',#7946,.T.);
#4659=FACE_OUTER_BOUND('',#7947,.T.);
#4660=FACE_OUTER_BOUND('',#7948,.T.);
#4661=FACE_OUTER_BOUND('',#7949,.T.);
#4662=FACE_OUTER_BOUND('',#7950,.T.);
#4663=FACE_OUTER_BOUND('',#7951,.T.);
#4664=FACE_OUTER_BOUND('',#7952,.T.);
#4665=FACE_OUTER_BOUND('',#7953,.T.);
#4666=FACE_OUTER_BOUND('',#7954,.T.);
#4667=FACE_OUTER_BOUND('',#7955,.T.);
#4668=FACE_OUTER_BOUND('',#7956,.T.);
#4669=FACE_OUTER_BOUND('',#7957,.T.);
#4670=FACE_OUTER_BOUND('',#7958,.T.);
#4671=FACE_OUTER_BOUND('',#7959,.T.);
#4672=FACE_OUTER_BOUND('',#7960,.T.);
#4673=FACE_OUTER_BOUND('',#7961,.T.);
#4674=FACE_OUTER_BOUND('',#7962,.T.);
#4675=FACE_OUTER_BOUND('',#7963,.T.);
#4676=FACE_OUTER_BOUND('',#7964,.T.);
#4677=FACE_OUTER_BOUND('',#7965,.T.);
#4678=FACE_OUTER_BOUND('',#7966,.T.);
#4679=FACE_OUTER_BOUND('',#7967,.T.);
#4680=FACE_OUTER_BOUND('',#7968,.T.);
#4681=FACE_OUTER_BOUND('',#7969,.T.);
#4682=FACE_OUTER_BOUND('',#7970,.T.);
#4683=FACE_OUTER_BOUND('',#7971,.T.);
#4684=FACE_OUTER_BOUND('',#7972,.T.);
#4685=FACE_OUTER_BOUND('',#7973,.T.);
#4686=FACE_OUTER_BOUND('',#7974,.T.);
#4687=FACE_OUTER_BOUND('',#7975,.T.);
#4688=FACE_OUTER_BOUND('',#7976,.T.);
#4689=FACE_OUTER_BOUND('',#7977,.T.);
#4690=FACE_OUTER_BOUND('',#7978,.T.);
#4691=FACE_OUTER_BOUND('',#7979,.T.);
#4692=FACE_OUTER_BOUND('',#7981,.T.);
#4693=FACE_OUTER_BOUND('',#7982,.T.);
#4694=FACE_OUTER_BOUND('',#7983,.T.);
#4695=FACE_OUTER_BOUND('',#7984,.T.);
#4696=FACE_OUTER_BOUND('',#7985,.T.);
#4697=FACE_OUTER_BOUND('',#7986,.T.);
#4698=FACE_OUTER_BOUND('',#7987,.T.);
#4699=FACE_OUTER_BOUND('',#7988,.T.);
#4700=FACE_OUTER_BOUND('',#7989,.T.);
#4701=FACE_OUTER_BOUND('',#7990,.T.);
#4702=FACE_OUTER_BOUND('',#7991,.T.);
#4703=FACE_OUTER_BOUND('',#7992,.T.);
#4704=FACE_OUTER_BOUND('',#7993,.T.);
#4705=FACE_OUTER_BOUND('',#7994,.T.);
#4706=FACE_OUTER_BOUND('',#7995,.T.);
#4707=FACE_OUTER_BOUND('',#7996,.T.);
#4708=FACE_OUTER_BOUND('',#7997,.T.);
#4709=FACE_OUTER_BOUND('',#7998,.T.);
#4710=FACE_OUTER_BOUND('',#7999,.T.);
#4711=FACE_OUTER_BOUND('',#8000,.T.);
#4712=FACE_OUTER_BOUND('',#8001,.T.);
#4713=FACE_OUTER_BOUND('',#8002,.T.);
#4714=FACE_OUTER_BOUND('',#8003,.T.);
#4715=FACE_OUTER_BOUND('',#8004,.T.);
#4716=FACE_OUTER_BOUND('',#8005,.T.);
#4717=FACE_OUTER_BOUND('',#8006,.T.);
#4718=FACE_OUTER_BOUND('',#8007,.T.);
#4719=FACE_OUTER_BOUND('',#8008,.T.);
#4720=FACE_OUTER_BOUND('',#8009,.T.);
#4721=FACE_OUTER_BOUND('',#8011,.T.);
#4722=FACE_OUTER_BOUND('',#8012,.T.);
#4723=FACE_OUTER_BOUND('',#8013,.T.);
#4724=FACE_OUTER_BOUND('',#8014,.T.);
#4725=FACE_OUTER_BOUND('',#8015,.T.);
#4726=FACE_OUTER_BOUND('',#8016,.T.);
#4727=FACE_OUTER_BOUND('',#8017,.T.);
#4728=FACE_OUTER_BOUND('',#8018,.T.);
#4729=FACE_OUTER_BOUND('',#8019,.T.);
#4730=FACE_OUTER_BOUND('',#8020,.T.);
#4731=FACE_OUTER_BOUND('',#8021,.T.);
#4732=FACE_OUTER_BOUND('',#8022,.T.);
#4733=FACE_OUTER_BOUND('',#8023,.T.);
#4734=FACE_OUTER_BOUND('',#8024,.T.);
#4735=FACE_OUTER_BOUND('',#8025,.T.);
#4736=FACE_OUTER_BOUND('',#8026,.T.);
#4737=FACE_OUTER_BOUND('',#8027,.T.);
#4738=FACE_OUTER_BOUND('',#8028,.T.);
#4739=FACE_OUTER_BOUND('',#8029,.T.);
#4740=FACE_OUTER_BOUND('',#8030,.T.);
#4741=FACE_OUTER_BOUND('',#8031,.T.);
#4742=FACE_OUTER_BOUND('',#8032,.T.);
#4743=FACE_OUTER_BOUND('',#8033,.T.);
#4744=FACE_OUTER_BOUND('',#8035,.T.);
#4745=FACE_OUTER_BOUND('',#8036,.T.);
#4746=FACE_OUTER_BOUND('',#8037,.T.);
#4747=FACE_OUTER_BOUND('',#8038,.T.);
#4748=FACE_OUTER_BOUND('',#8039,.T.);
#4749=FACE_OUTER_BOUND('',#8040,.T.);
#4750=FACE_OUTER_BOUND('',#8041,.T.);
#4751=FACE_OUTER_BOUND('',#8042,.T.);
#4752=FACE_OUTER_BOUND('',#8043,.T.);
#4753=FACE_OUTER_BOUND('',#8044,.T.);
#4754=FACE_OUTER_BOUND('',#8045,.T.);
#4755=FACE_OUTER_BOUND('',#8046,.T.);
#4756=FACE_OUTER_BOUND('',#8047,.T.);
#4757=FACE_OUTER_BOUND('',#8048,.T.);
#4758=FACE_OUTER_BOUND('',#8049,.T.);
#4759=FACE_OUTER_BOUND('',#8050,.T.);
#4760=FACE_OUTER_BOUND('',#8051,.T.);
#4761=FACE_OUTER_BOUND('',#8052,.T.);
#4762=FACE_OUTER_BOUND('',#8053,.T.);
#4763=FACE_OUTER_BOUND('',#8054,.T.);
#4764=FACE_OUTER_BOUND('',#8055,.T.);
#4765=FACE_OUTER_BOUND('',#8056,.T.);
#4766=FACE_OUTER_BOUND('',#8057,.T.);
#4767=FACE_OUTER_BOUND('',#8058,.T.);
#4768=FACE_OUTER_BOUND('',#8059,.T.);
#4769=FACE_OUTER_BOUND('',#8060,.T.);
#4770=FACE_OUTER_BOUND('',#8061,.T.);
#4771=FACE_OUTER_BOUND('',#8062,.T.);
#4772=FACE_OUTER_BOUND('',#8063,.T.);
#4773=FACE_OUTER_BOUND('',#8064,.T.);
#4774=FACE_OUTER_BOUND('',#8065,.T.);
#4775=FACE_OUTER_BOUND('',#8066,.T.);
#4776=FACE_OUTER_BOUND('',#8067,.T.);
#4777=FACE_OUTER_BOUND('',#8068,.T.);
#4778=FACE_OUTER_BOUND('',#8070,.T.);
#4779=FACE_OUTER_BOUND('',#8071,.T.);
#4780=FACE_OUTER_BOUND('',#8072,.T.);
#4781=FACE_OUTER_BOUND('',#8073,.T.);
#4782=FACE_OUTER_BOUND('',#8074,.T.);
#4783=FACE_OUTER_BOUND('',#8075,.T.);
#4784=FACE_OUTER_BOUND('',#8076,.T.);
#4785=FACE_OUTER_BOUND('',#8077,.T.);
#4786=FACE_OUTER_BOUND('',#8078,.T.);
#4787=FACE_OUTER_BOUND('',#8079,.T.);
#4788=FACE_OUTER_BOUND('',#8080,.T.);
#4789=FACE_OUTER_BOUND('',#8081,.T.);
#4790=FACE_OUTER_BOUND('',#8082,.T.);
#4791=FACE_OUTER_BOUND('',#8083,.T.);
#4792=FACE_OUTER_BOUND('',#8084,.T.);
#4793=FACE_OUTER_BOUND('',#8085,.T.);
#4794=FACE_OUTER_BOUND('',#8086,.T.);
#4795=FACE_OUTER_BOUND('',#8087,.T.);
#4796=FACE_OUTER_BOUND('',#8088,.T.);
#4797=FACE_OUTER_BOUND('',#8089,.T.);
#4798=FACE_OUTER_BOUND('',#8090,.T.);
#4799=FACE_OUTER_BOUND('',#8091,.T.);
#4800=FACE_OUTER_BOUND('',#8092,.T.);
#4801=FACE_OUTER_BOUND('',#8093,.T.);
#4802=FACE_OUTER_BOUND('',#8094,.T.);
#4803=FACE_OUTER_BOUND('',#8095,.T.);
#4804=FACE_OUTER_BOUND('',#8096,.T.);
#4805=FACE_OUTER_BOUND('',#8097,.T.);
#4806=FACE_OUTER_BOUND('',#8098,.T.);
#4807=FACE_OUTER_BOUND('',#8099,.T.);
#4808=FACE_OUTER_BOUND('',#8100,.T.);
#4809=FACE_OUTER_BOUND('',#8101,.T.);
#4810=FACE_OUTER_BOUND('',#8102,.T.);
#4811=FACE_OUTER_BOUND('',#8103,.T.);
#4812=FACE_OUTER_BOUND('',#8106,.T.);
#4813=FACE_OUTER_BOUND('',#8107,.T.);
#4814=FACE_OUTER_BOUND('',#8108,.T.);
#4815=FACE_OUTER_BOUND('',#8109,.T.);
#4816=FACE_OUTER_BOUND('',#8110,.T.);
#4817=FACE_OUTER_BOUND('',#8111,.T.);
#4818=FACE_OUTER_BOUND('',#8112,.T.);
#4819=FACE_OUTER_BOUND('',#8113,.T.);
#4820=FACE_OUTER_BOUND('',#8114,.T.);
#4821=FACE_OUTER_BOUND('',#8115,.T.);
#4822=FACE_OUTER_BOUND('',#8116,.T.);
#4823=FACE_OUTER_BOUND('',#8117,.T.);
#4824=FACE_OUTER_BOUND('',#8118,.T.);
#4825=FACE_OUTER_BOUND('',#8119,.T.);
#4826=FACE_OUTER_BOUND('',#8120,.T.);
#4827=FACE_OUTER_BOUND('',#8121,.T.);
#4828=FACE_OUTER_BOUND('',#8122,.T.);
#4829=FACE_OUTER_BOUND('',#8123,.T.);
#4830=FACE_OUTER_BOUND('',#8124,.T.);
#4831=FACE_OUTER_BOUND('',#8125,.T.);
#4832=FACE_OUTER_BOUND('',#8126,.T.);
#4833=FACE_OUTER_BOUND('',#8127,.T.);
#4834=FACE_OUTER_BOUND('',#8128,.T.);
#4835=FACE_OUTER_BOUND('',#8129,.T.);
#4836=FACE_OUTER_BOUND('',#8131,.T.);
#4837=FACE_OUTER_BOUND('',#8132,.T.);
#4838=FACE_OUTER_BOUND('',#8133,.T.);
#4839=FACE_OUTER_BOUND('',#8134,.T.);
#4840=FACE_OUTER_BOUND('',#8135,.T.);
#4841=FACE_OUTER_BOUND('',#8136,.T.);
#4842=FACE_OUTER_BOUND('',#8137,.T.);
#4843=FACE_OUTER_BOUND('',#8138,.T.);
#4844=FACE_OUTER_BOUND('',#8139,.T.);
#4845=FACE_OUTER_BOUND('',#8140,.T.);
#4846=FACE_OUTER_BOUND('',#8141,.T.);
#4847=FACE_OUTER_BOUND('',#8142,.T.);
#4848=FACE_OUTER_BOUND('',#8143,.T.);
#4849=FACE_OUTER_BOUND('',#8144,.T.);
#4850=FACE_OUTER_BOUND('',#8145,.T.);
#4851=FACE_OUTER_BOUND('',#8146,.T.);
#4852=FACE_OUTER_BOUND('',#8147,.T.);
#4853=FACE_OUTER_BOUND('',#8148,.T.);
#4854=FACE_OUTER_BOUND('',#8149,.T.);
#4855=FACE_OUTER_BOUND('',#8150,.T.);
#4856=FACE_OUTER_BOUND('',#8151,.T.);
#4857=FACE_OUTER_BOUND('',#8152,.T.);
#4858=FACE_OUTER_BOUND('',#8153,.T.);
#4859=FACE_OUTER_BOUND('',#8154,.T.);
#4860=FACE_OUTER_BOUND('',#8155,.T.);
#4861=FACE_OUTER_BOUND('',#8156,.T.);
#4862=FACE_OUTER_BOUND('',#8157,.T.);
#4863=FACE_OUTER_BOUND('',#8158,.T.);
#4864=FACE_OUTER_BOUND('',#8159,.T.);
#4865=FACE_OUTER_BOUND('',#8160,.T.);
#4866=FACE_OUTER_BOUND('',#8161,.T.);
#4867=FACE_OUTER_BOUND('',#8163,.T.);
#4868=FACE_OUTER_BOUND('',#8164,.T.);
#4869=FACE_OUTER_BOUND('',#8165,.T.);
#4870=FACE_OUTER_BOUND('',#8166,.T.);
#4871=FACE_OUTER_BOUND('',#8167,.T.);
#4872=FACE_OUTER_BOUND('',#8168,.T.);
#4873=FACE_OUTER_BOUND('',#8169,.T.);
#4874=FACE_OUTER_BOUND('',#8170,.T.);
#4875=FACE_OUTER_BOUND('',#8171,.T.);
#4876=FACE_OUTER_BOUND('',#8172,.T.);
#4877=FACE_OUTER_BOUND('',#8173,.T.);
#4878=FACE_OUTER_BOUND('',#8174,.T.);
#4879=FACE_OUTER_BOUND('',#8175,.T.);
#4880=FACE_OUTER_BOUND('',#8176,.T.);
#4881=FACE_OUTER_BOUND('',#8177,.T.);
#4882=FACE_OUTER_BOUND('',#8178,.T.);
#4883=FACE_OUTER_BOUND('',#8179,.T.);
#4884=FACE_OUTER_BOUND('',#8180,.T.);
#4885=FACE_OUTER_BOUND('',#8181,.T.);
#4886=FACE_OUTER_BOUND('',#8182,.T.);
#4887=FACE_OUTER_BOUND('',#8183,.T.);
#4888=FACE_OUTER_BOUND('',#8184,.T.);
#4889=FACE_OUTER_BOUND('',#8185,.T.);
#4890=FACE_OUTER_BOUND('',#8186,.T.);
#4891=FACE_OUTER_BOUND('',#8187,.T.);
#4892=FACE_OUTER_BOUND('',#8188,.T.);
#4893=FACE_OUTER_BOUND('',#8189,.T.);
#4894=FACE_OUTER_BOUND('',#8190,.T.);
#4895=FACE_OUTER_BOUND('',#8191,.T.);
#4896=FACE_OUTER_BOUND('',#8192,.T.);
#4897=FACE_OUTER_BOUND('',#8193,.T.);
#4898=FACE_OUTER_BOUND('',#8194,.T.);
#4899=FACE_OUTER_BOUND('',#8195,.T.);
#4900=FACE_OUTER_BOUND('',#8196,.T.);
#4901=FACE_OUTER_BOUND('',#8197,.T.);
#4902=FACE_OUTER_BOUND('',#8198,.T.);
#4903=FACE_OUTER_BOUND('',#8199,.T.);
#4904=FACE_OUTER_BOUND('',#8200,.T.);
#4905=FACE_OUTER_BOUND('',#8201,.T.);
#4906=FACE_OUTER_BOUND('',#8202,.T.);
#4907=FACE_OUTER_BOUND('',#8203,.T.);
#4908=FACE_OUTER_BOUND('',#8204,.T.);
#4909=FACE_OUTER_BOUND('',#8205,.T.);
#4910=FACE_OUTER_BOUND('',#8206,.T.);
#4911=FACE_OUTER_BOUND('',#8207,.T.);
#4912=FACE_OUTER_BOUND('',#8208,.T.);
#4913=FACE_OUTER_BOUND('',#8209,.T.);
#4914=FACE_OUTER_BOUND('',#8210,.T.);
#4915=FACE_OUTER_BOUND('',#8211,.T.);
#4916=FACE_OUTER_BOUND('',#8212,.T.);
#4917=FACE_OUTER_BOUND('',#8213,.T.);
#4918=FACE_OUTER_BOUND('',#8214,.T.);
#4919=FACE_OUTER_BOUND('',#8215,.T.);
#4920=FACE_OUTER_BOUND('',#8216,.T.);
#4921=FACE_OUTER_BOUND('',#8217,.T.);
#4922=FACE_OUTER_BOUND('',#8218,.T.);
#4923=FACE_OUTER_BOUND('',#8219,.T.);
#4924=FACE_OUTER_BOUND('',#8220,.T.);
#4925=FACE_OUTER_BOUND('',#8221,.T.);
#4926=FACE_OUTER_BOUND('',#8222,.T.);
#4927=FACE_OUTER_BOUND('',#8223,.T.);
#4928=FACE_OUTER_BOUND('',#8224,.T.);
#4929=FACE_OUTER_BOUND('',#8225,.T.);
#4930=FACE_OUTER_BOUND('',#8226,.T.);
#4931=FACE_OUTER_BOUND('',#8227,.T.);
#4932=FACE_OUTER_BOUND('',#8228,.T.);
#4933=FACE_OUTER_BOUND('',#8229,.T.);
#4934=FACE_OUTER_BOUND('',#8230,.T.);
#4935=FACE_OUTER_BOUND('',#8231,.T.);
#4936=FACE_OUTER_BOUND('',#8232,.T.);
#4937=FACE_OUTER_BOUND('',#8233,.T.);
#4938=FACE_OUTER_BOUND('',#8234,.T.);
#4939=FACE_OUTER_BOUND('',#8235,.T.);
#4940=FACE_OUTER_BOUND('',#8236,.T.);
#4941=FACE_OUTER_BOUND('',#8237,.T.);
#4942=FACE_OUTER_BOUND('',#8238,.T.);
#4943=FACE_OUTER_BOUND('',#8239,.T.);
#4944=FACE_OUTER_BOUND('',#8240,.T.);
#4945=FACE_OUTER_BOUND('',#8241,.T.);
#4946=FACE_OUTER_BOUND('',#8242,.T.);
#4947=FACE_OUTER_BOUND('',#8243,.T.);
#4948=FACE_OUTER_BOUND('',#8244,.T.);
#4949=FACE_OUTER_BOUND('',#8245,.T.);
#4950=FACE_OUTER_BOUND('',#8246,.T.);
#4951=FACE_OUTER_BOUND('',#8247,.T.);
#4952=FACE_OUTER_BOUND('',#8248,.T.);
#4953=FACE_OUTER_BOUND('',#8249,.T.);
#4954=FACE_OUTER_BOUND('',#8250,.T.);
#4955=FACE_OUTER_BOUND('',#8251,.T.);
#4956=FACE_OUTER_BOUND('',#8252,.T.);
#4957=FACE_OUTER_BOUND('',#8253,.T.);
#4958=FACE_OUTER_BOUND('',#8254,.T.);
#4959=FACE_OUTER_BOUND('',#8255,.T.);
#4960=FACE_OUTER_BOUND('',#8256,.T.);
#4961=FACE_OUTER_BOUND('',#8257,.T.);
#4962=FACE_OUTER_BOUND('',#8258,.T.);
#4963=FACE_OUTER_BOUND('',#8259,.T.);
#4964=FACE_OUTER_BOUND('',#8260,.T.);
#4965=FACE_OUTER_BOUND('',#8261,.T.);
#4966=FACE_OUTER_BOUND('',#8262,.T.);
#4967=FACE_OUTER_BOUND('',#8263,.T.);
#4968=FACE_OUTER_BOUND('',#8264,.T.);
#4969=FACE_OUTER_BOUND('',#8265,.T.);
#4970=FACE_OUTER_BOUND('',#8266,.T.);
#4971=FACE_OUTER_BOUND('',#8267,.T.);
#4972=FACE_OUTER_BOUND('',#8268,.T.);
#4973=FACE_OUTER_BOUND('',#8269,.T.);
#4974=FACE_OUTER_BOUND('',#8270,.T.);
#4975=FACE_OUTER_BOUND('',#8271,.T.);
#4976=FACE_OUTER_BOUND('',#8272,.T.);
#4977=FACE_OUTER_BOUND('',#8273,.T.);
#4978=FACE_OUTER_BOUND('',#8274,.T.);
#4979=FACE_OUTER_BOUND('',#8275,.T.);
#4980=FACE_OUTER_BOUND('',#8276,.T.);
#4981=FACE_OUTER_BOUND('',#8277,.T.);
#4982=FACE_OUTER_BOUND('',#8278,.T.);
#4983=FACE_OUTER_BOUND('',#8279,.T.);
#4984=FACE_OUTER_BOUND('',#8280,.T.);
#4985=FACE_OUTER_BOUND('',#8281,.T.);
#4986=FACE_OUTER_BOUND('',#8282,.T.);
#4987=FACE_OUTER_BOUND('',#8283,.T.);
#4988=FACE_OUTER_BOUND('',#8284,.T.);
#4989=FACE_OUTER_BOUND('',#8285,.T.);
#4990=FACE_OUTER_BOUND('',#8286,.T.);
#4991=FACE_OUTER_BOUND('',#8287,.T.);
#4992=FACE_OUTER_BOUND('',#8288,.T.);
#4993=FACE_OUTER_BOUND('',#8289,.T.);
#4994=FACE_OUTER_BOUND('',#8290,.T.);
#4995=FACE_OUTER_BOUND('',#8291,.T.);
#4996=FACE_OUTER_BOUND('',#8292,.T.);
#4997=FACE_OUTER_BOUND('',#8293,.T.);
#4998=FACE_OUTER_BOUND('',#8294,.T.);
#4999=FACE_OUTER_BOUND('',#8295,.T.);
#5000=FACE_OUTER_BOUND('',#8296,.T.);
#5001=FACE_OUTER_BOUND('',#8297,.T.);
#5002=FACE_OUTER_BOUND('',#8298,.T.);
#5003=FACE_OUTER_BOUND('',#8299,.T.);
#5004=FACE_OUTER_BOUND('',#8300,.T.);
#5005=FACE_OUTER_BOUND('',#8301,.T.);
#5006=FACE_OUTER_BOUND('',#8302,.T.);
#5007=FACE_OUTER_BOUND('',#8303,.T.);
#5008=FACE_OUTER_BOUND('',#8304,.T.);
#5009=FACE_OUTER_BOUND('',#8305,.T.);
#5010=FACE_OUTER_BOUND('',#8306,.T.);
#5011=FACE_OUTER_BOUND('',#8307,.T.);
#5012=FACE_OUTER_BOUND('',#8308,.T.);
#5013=FACE_OUTER_BOUND('',#8309,.T.);
#5014=FACE_OUTER_BOUND('',#8310,.T.);
#5015=FACE_OUTER_BOUND('',#8311,.T.);
#5016=FACE_OUTER_BOUND('',#8312,.T.);
#5017=FACE_OUTER_BOUND('',#8313,.T.);
#5018=FACE_OUTER_BOUND('',#8314,.T.);
#5019=FACE_OUTER_BOUND('',#8315,.T.);
#5020=FACE_OUTER_BOUND('',#8316,.T.);
#5021=FACE_OUTER_BOUND('',#8317,.T.);
#5022=FACE_OUTER_BOUND('',#8318,.T.);
#5023=FACE_OUTER_BOUND('',#8319,.T.);
#5024=FACE_OUTER_BOUND('',#8320,.T.);
#5025=FACE_OUTER_BOUND('',#8321,.T.);
#5026=FACE_OUTER_BOUND('',#8322,.T.);
#5027=FACE_OUTER_BOUND('',#8323,.T.);
#5028=FACE_OUTER_BOUND('',#8324,.T.);
#5029=FACE_OUTER_BOUND('',#8325,.T.);
#5030=FACE_OUTER_BOUND('',#8326,.T.);
#5031=FACE_OUTER_BOUND('',#8327,.T.);
#5032=FACE_OUTER_BOUND('',#8328,.T.);
#5033=FACE_OUTER_BOUND('',#8329,.T.);
#5034=FACE_OUTER_BOUND('',#8330,.T.);
#5035=FACE_OUTER_BOUND('',#8331,.T.);
#5036=FACE_OUTER_BOUND('',#8332,.T.);
#5037=FACE_OUTER_BOUND('',#8333,.T.);
#5038=FACE_OUTER_BOUND('',#8334,.T.);
#5039=FACE_OUTER_BOUND('',#8335,.T.);
#5040=FACE_OUTER_BOUND('',#8336,.T.);
#5041=FACE_OUTER_BOUND('',#8337,.T.);
#5042=FACE_OUTER_BOUND('',#8338,.T.);
#5043=FACE_OUTER_BOUND('',#8339,.T.);
#5044=FACE_OUTER_BOUND('',#8340,.T.);
#5045=FACE_OUTER_BOUND('',#8341,.T.);
#5046=FACE_OUTER_BOUND('',#8342,.T.);
#5047=FACE_OUTER_BOUND('',#8343,.T.);
#5048=FACE_OUTER_BOUND('',#8344,.T.);
#5049=FACE_OUTER_BOUND('',#8345,.T.);
#5050=FACE_OUTER_BOUND('',#8346,.T.);
#5051=FACE_OUTER_BOUND('',#8347,.T.);
#5052=FACE_OUTER_BOUND('',#8348,.T.);
#5053=FACE_OUTER_BOUND('',#8349,.T.);
#5054=FACE_OUTER_BOUND('',#8350,.T.);
#5055=FACE_OUTER_BOUND('',#8351,.T.);
#5056=FACE_OUTER_BOUND('',#8352,.T.);
#5057=FACE_OUTER_BOUND('',#8353,.T.);
#5058=FACE_OUTER_BOUND('',#8354,.T.);
#5059=FACE_OUTER_BOUND('',#8355,.T.);
#5060=FACE_OUTER_BOUND('',#8356,.T.);
#5061=FACE_OUTER_BOUND('',#8357,.T.);
#5062=FACE_OUTER_BOUND('',#8358,.T.);
#5063=FACE_OUTER_BOUND('',#8359,.T.);
#5064=FACE_OUTER_BOUND('',#8360,.T.);
#5065=FACE_OUTER_BOUND('',#8361,.T.);
#5066=FACE_OUTER_BOUND('',#8362,.T.);
#5067=FACE_OUTER_BOUND('',#8363,.T.);
#5068=FACE_OUTER_BOUND('',#8364,.T.);
#5069=FACE_OUTER_BOUND('',#8365,.T.);
#5070=FACE_OUTER_BOUND('',#8366,.T.);
#5071=FACE_OUTER_BOUND('',#8367,.T.);
#5072=FACE_OUTER_BOUND('',#8368,.T.);
#5073=FACE_OUTER_BOUND('',#8369,.T.);
#5074=FACE_OUTER_BOUND('',#8370,.T.);
#5075=FACE_OUTER_BOUND('',#8371,.T.);
#5076=FACE_OUTER_BOUND('',#8372,.T.);
#5077=FACE_OUTER_BOUND('',#8373,.T.);
#5078=FACE_OUTER_BOUND('',#8374,.T.);
#5079=FACE_OUTER_BOUND('',#8375,.T.);
#5080=FACE_OUTER_BOUND('',#8376,.T.);
#5081=FACE_OUTER_BOUND('',#8377,.T.);
#5082=FACE_OUTER_BOUND('',#8378,.T.);
#5083=FACE_OUTER_BOUND('',#8379,.T.);
#5084=FACE_OUTER_BOUND('',#8380,.T.);
#5085=FACE_OUTER_BOUND('',#8381,.T.);
#5086=FACE_OUTER_BOUND('',#8382,.T.);
#5087=FACE_OUTER_BOUND('',#8383,.T.);
#5088=FACE_OUTER_BOUND('',#8384,.T.);
#5089=FACE_OUTER_BOUND('',#8385,.T.);
#5090=FACE_OUTER_BOUND('',#8386,.T.);
#5091=FACE_OUTER_BOUND('',#8387,.T.);
#5092=FACE_OUTER_BOUND('',#8388,.T.);
#5093=FACE_OUTER_BOUND('',#8389,.T.);
#5094=FACE_OUTER_BOUND('',#8390,.T.);
#5095=FACE_OUTER_BOUND('',#8391,.T.);
#5096=FACE_OUTER_BOUND('',#8392,.T.);
#5097=FACE_OUTER_BOUND('',#8393,.T.);
#5098=FACE_OUTER_BOUND('',#8394,.T.);
#5099=FACE_OUTER_BOUND('',#8395,.T.);
#5100=FACE_OUTER_BOUND('',#8396,.T.);
#5101=FACE_OUTER_BOUND('',#8397,.T.);
#5102=FACE_OUTER_BOUND('',#8398,.T.);
#5103=FACE_OUTER_BOUND('',#8399,.T.);
#5104=FACE_OUTER_BOUND('',#8400,.T.);
#5105=FACE_OUTER_BOUND('',#8401,.T.);
#5106=FACE_OUTER_BOUND('',#8402,.T.);
#5107=FACE_OUTER_BOUND('',#8403,.T.);
#5108=FACE_OUTER_BOUND('',#8404,.T.);
#5109=FACE_OUTER_BOUND('',#8405,.T.);
#5110=FACE_OUTER_BOUND('',#8406,.T.);
#5111=FACE_OUTER_BOUND('',#8407,.T.);
#5112=FACE_OUTER_BOUND('',#8408,.T.);
#5113=FACE_OUTER_BOUND('',#8409,.T.);
#5114=FACE_OUTER_BOUND('',#8410,.T.);
#5115=FACE_OUTER_BOUND('',#8411,.T.);
#5116=FACE_OUTER_BOUND('',#8412,.T.);
#5117=FACE_OUTER_BOUND('',#8413,.T.);
#5118=FACE_OUTER_BOUND('',#8414,.T.);
#5119=FACE_OUTER_BOUND('',#8415,.T.);
#5120=FACE_OUTER_BOUND('',#8416,.T.);
#5121=FACE_OUTER_BOUND('',#8417,.T.);
#5122=FACE_OUTER_BOUND('',#8418,.T.);
#5123=FACE_OUTER_BOUND('',#8419,.T.);
#5124=FACE_OUTER_BOUND('',#8420,.T.);
#5125=FACE_OUTER_BOUND('',#8421,.T.);
#5126=FACE_OUTER_BOUND('',#8422,.T.);
#5127=FACE_OUTER_BOUND('',#8423,.T.);
#5128=FACE_OUTER_BOUND('',#8424,.T.);
#5129=FACE_OUTER_BOUND('',#8425,.T.);
#5130=FACE_OUTER_BOUND('',#8426,.T.);
#5131=FACE_OUTER_BOUND('',#8427,.T.);
#5132=FACE_OUTER_BOUND('',#8428,.T.);
#5133=FACE_OUTER_BOUND('',#8429,.T.);
#5134=FACE_OUTER_BOUND('',#8430,.T.);
#5135=FACE_OUTER_BOUND('',#8431,.T.);
#5136=FACE_OUTER_BOUND('',#8432,.T.);
#5137=FACE_OUTER_BOUND('',#8433,.T.);
#5138=FACE_OUTER_BOUND('',#8434,.T.);
#5139=FACE_OUTER_BOUND('',#8435,.T.);
#5140=FACE_OUTER_BOUND('',#8436,.T.);
#5141=FACE_OUTER_BOUND('',#8437,.T.);
#5142=FACE_OUTER_BOUND('',#8438,.T.);
#5143=FACE_OUTER_BOUND('',#8439,.T.);
#5144=FACE_OUTER_BOUND('',#8440,.T.);
#5145=FACE_OUTER_BOUND('',#8441,.T.);
#5146=FACE_OUTER_BOUND('',#8442,.T.);
#5147=FACE_OUTER_BOUND('',#8443,.T.);
#5148=FACE_OUTER_BOUND('',#8444,.T.);
#5149=FACE_OUTER_BOUND('',#8445,.T.);
#5150=FACE_OUTER_BOUND('',#8446,.T.);
#5151=FACE_OUTER_BOUND('',#8447,.T.);
#5152=FACE_OUTER_BOUND('',#8448,.T.);
#5153=FACE_OUTER_BOUND('',#8449,.T.);
#5154=FACE_OUTER_BOUND('',#8450,.T.);
#5155=FACE_OUTER_BOUND('',#8451,.T.);
#5156=FACE_OUTER_BOUND('',#8452,.T.);
#5157=FACE_OUTER_BOUND('',#8453,.T.);
#5158=FACE_OUTER_BOUND('',#8454,.T.);
#5159=FACE_OUTER_BOUND('',#8455,.T.);
#5160=FACE_OUTER_BOUND('',#8456,.T.);
#5161=FACE_OUTER_BOUND('',#8457,.T.);
#5162=FACE_OUTER_BOUND('',#8458,.T.);
#5163=FACE_OUTER_BOUND('',#8459,.T.);
#5164=FACE_OUTER_BOUND('',#8460,.T.);
#5165=FACE_OUTER_BOUND('',#8461,.T.);
#5166=FACE_OUTER_BOUND('',#8462,.T.);
#5167=FACE_OUTER_BOUND('',#8463,.T.);
#5168=FACE_OUTER_BOUND('',#8464,.T.);
#5169=FACE_OUTER_BOUND('',#8465,.T.);
#5170=FACE_OUTER_BOUND('',#8466,.T.);
#5171=FACE_OUTER_BOUND('',#8467,.T.);
#5172=FACE_OUTER_BOUND('',#8468,.T.);
#5173=FACE_OUTER_BOUND('',#8469,.T.);
#5174=FACE_OUTER_BOUND('',#8470,.T.);
#5175=FACE_OUTER_BOUND('',#8471,.T.);
#5176=FACE_OUTER_BOUND('',#8472,.T.);
#5177=FACE_OUTER_BOUND('',#8473,.T.);
#5178=FACE_OUTER_BOUND('',#8474,.T.);
#5179=FACE_OUTER_BOUND('',#8475,.T.);
#5180=FACE_OUTER_BOUND('',#8476,.T.);
#5181=FACE_OUTER_BOUND('',#8477,.T.);
#5182=FACE_OUTER_BOUND('',#8478,.T.);
#5183=FACE_OUTER_BOUND('',#8479,.T.);
#5184=FACE_OUTER_BOUND('',#8480,.T.);
#5185=FACE_OUTER_BOUND('',#8481,.T.);
#5186=FACE_OUTER_BOUND('',#8482,.T.);
#5187=FACE_OUTER_BOUND('',#8483,.T.);
#5188=FACE_OUTER_BOUND('',#8484,.T.);
#5189=FACE_OUTER_BOUND('',#8485,.T.);
#5190=FACE_OUTER_BOUND('',#8486,.T.);
#5191=FACE_OUTER_BOUND('',#8487,.T.);
#5192=FACE_OUTER_BOUND('',#8488,.T.);
#5193=FACE_OUTER_BOUND('',#8489,.T.);
#5194=FACE_OUTER_BOUND('',#8490,.T.);
#5195=FACE_OUTER_BOUND('',#8491,.T.);
#5196=FACE_OUTER_BOUND('',#8492,.T.);
#5197=FACE_OUTER_BOUND('',#8493,.T.);
#5198=FACE_OUTER_BOUND('',#8494,.T.);
#5199=FACE_OUTER_BOUND('',#8495,.T.);
#5200=FACE_OUTER_BOUND('',#8496,.T.);
#5201=FACE_OUTER_BOUND('',#8497,.T.);
#5202=FACE_OUTER_BOUND('',#8498,.T.);
#5203=FACE_OUTER_BOUND('',#8499,.T.);
#5204=FACE_OUTER_BOUND('',#8500,.T.);
#5205=FACE_OUTER_BOUND('',#8501,.T.);
#5206=FACE_OUTER_BOUND('',#8502,.T.);
#5207=FACE_OUTER_BOUND('',#8503,.T.);
#5208=FACE_OUTER_BOUND('',#8504,.T.);
#5209=FACE_OUTER_BOUND('',#8505,.T.);
#5210=FACE_OUTER_BOUND('',#8506,.T.);
#5211=FACE_OUTER_BOUND('',#8507,.T.);
#5212=FACE_OUTER_BOUND('',#8508,.T.);
#5213=FACE_OUTER_BOUND('',#8509,.T.);
#5214=FACE_OUTER_BOUND('',#8510,.T.);
#5215=FACE_OUTER_BOUND('',#8511,.T.);
#5216=FACE_OUTER_BOUND('',#8512,.T.);
#5217=FACE_OUTER_BOUND('',#8513,.T.);
#5218=FACE_OUTER_BOUND('',#8514,.T.);
#5219=FACE_OUTER_BOUND('',#8515,.T.);
#5220=FACE_OUTER_BOUND('',#8516,.T.);
#5221=FACE_OUTER_BOUND('',#8517,.T.);
#5222=FACE_OUTER_BOUND('',#8518,.T.);
#5223=FACE_OUTER_BOUND('',#8519,.T.);
#5224=FACE_OUTER_BOUND('',#8520,.T.);
#5225=FACE_OUTER_BOUND('',#8521,.T.);
#5226=FACE_OUTER_BOUND('',#8522,.T.);
#5227=FACE_OUTER_BOUND('',#8523,.T.);
#5228=FACE_OUTER_BOUND('',#8524,.T.);
#5229=FACE_OUTER_BOUND('',#8525,.T.);
#5230=FACE_OUTER_BOUND('',#8526,.T.);
#5231=FACE_OUTER_BOUND('',#8527,.T.);
#5232=FACE_OUTER_BOUND('',#8528,.T.);
#5233=FACE_OUTER_BOUND('',#8529,.T.);
#5234=FACE_OUTER_BOUND('',#8530,.T.);
#5235=FACE_OUTER_BOUND('',#8531,.T.);
#5236=FACE_OUTER_BOUND('',#8532,.T.);
#5237=FACE_OUTER_BOUND('',#8533,.T.);
#5238=FACE_OUTER_BOUND('',#8534,.T.);
#5239=FACE_OUTER_BOUND('',#8535,.T.);
#5240=FACE_OUTER_BOUND('',#8536,.T.);
#5241=FACE_OUTER_BOUND('',#8537,.T.);
#5242=FACE_OUTER_BOUND('',#8538,.T.);
#5243=FACE_OUTER_BOUND('',#8539,.T.);
#5244=FACE_OUTER_BOUND('',#8540,.T.);
#5245=FACE_OUTER_BOUND('',#8541,.T.);
#5246=FACE_OUTER_BOUND('',#8542,.T.);
#5247=FACE_OUTER_BOUND('',#8543,.T.);
#5248=FACE_OUTER_BOUND('',#8544,.T.);
#5249=FACE_OUTER_BOUND('',#8545,.T.);
#5250=FACE_OUTER_BOUND('',#8546,.T.);
#5251=FACE_OUTER_BOUND('',#8547,.T.);
#5252=FACE_OUTER_BOUND('',#8548,.T.);
#5253=FACE_OUTER_BOUND('',#8549,.T.);
#5254=FACE_OUTER_BOUND('',#8550,.T.);
#5255=FACE_OUTER_BOUND('',#8551,.T.);
#5256=FACE_OUTER_BOUND('',#8552,.T.);
#5257=FACE_OUTER_BOUND('',#8553,.T.);
#5258=FACE_OUTER_BOUND('',#8554,.T.);
#5259=FACE_OUTER_BOUND('',#8555,.T.);
#5260=FACE_OUTER_BOUND('',#8556,.T.);
#5261=FACE_OUTER_BOUND('',#8557,.T.);
#5262=FACE_OUTER_BOUND('',#8558,.T.);
#5263=FACE_OUTER_BOUND('',#8559,.T.);
#5264=FACE_OUTER_BOUND('',#8560,.T.);
#5265=FACE_OUTER_BOUND('',#8561,.T.);
#5266=FACE_OUTER_BOUND('',#8562,.T.);
#5267=FACE_OUTER_BOUND('',#8563,.T.);
#5268=FACE_OUTER_BOUND('',#8564,.T.);
#5269=FACE_OUTER_BOUND('',#8565,.T.);
#5270=FACE_OUTER_BOUND('',#8566,.T.);
#5271=FACE_OUTER_BOUND('',#8567,.T.);
#5272=FACE_OUTER_BOUND('',#8568,.T.);
#5273=FACE_OUTER_BOUND('',#8569,.T.);
#5274=FACE_OUTER_BOUND('',#8570,.T.);
#5275=FACE_OUTER_BOUND('',#8571,.T.);
#5276=FACE_OUTER_BOUND('',#8572,.T.);
#5277=FACE_OUTER_BOUND('',#8573,.T.);
#5278=FACE_OUTER_BOUND('',#8574,.T.);
#5279=FACE_OUTER_BOUND('',#8575,.T.);
#5280=FACE_OUTER_BOUND('',#8576,.T.);
#5281=FACE_OUTER_BOUND('',#8577,.T.);
#5282=FACE_OUTER_BOUND('',#8578,.T.);
#5283=FACE_OUTER_BOUND('',#8579,.T.);
#5284=FACE_OUTER_BOUND('',#8580,.T.);
#5285=FACE_OUTER_BOUND('',#8581,.T.);
#5286=FACE_OUTER_BOUND('',#8582,.T.);
#5287=FACE_OUTER_BOUND('',#8583,.T.);
#5288=FACE_OUTER_BOUND('',#8584,.T.);
#5289=FACE_OUTER_BOUND('',#8585,.T.);
#5290=FACE_OUTER_BOUND('',#8586,.T.);
#5291=FACE_OUTER_BOUND('',#8587,.T.);
#5292=FACE_OUTER_BOUND('',#8588,.T.);
#5293=FACE_OUTER_BOUND('',#8589,.T.);
#5294=FACE_OUTER_BOUND('',#8590,.T.);
#5295=FACE_OUTER_BOUND('',#8591,.T.);
#5296=FACE_OUTER_BOUND('',#8592,.T.);
#5297=FACE_OUTER_BOUND('',#8593,.T.);
#5298=FACE_OUTER_BOUND('',#8594,.T.);
#5299=FACE_OUTER_BOUND('',#8595,.T.);
#5300=FACE_OUTER_BOUND('',#8596,.T.);
#5301=FACE_OUTER_BOUND('',#8597,.T.);
#5302=FACE_OUTER_BOUND('',#8598,.T.);
#5303=FACE_OUTER_BOUND('',#8599,.T.);
#5304=FACE_OUTER_BOUND('',#8600,.T.);
#5305=FACE_OUTER_BOUND('',#8601,.T.);
#5306=FACE_OUTER_BOUND('',#8602,.T.);
#5307=FACE_OUTER_BOUND('',#8603,.T.);
#5308=FACE_OUTER_BOUND('',#8604,.T.);
#5309=FACE_OUTER_BOUND('',#8605,.T.);
#5310=FACE_OUTER_BOUND('',#8606,.T.);
#5311=FACE_OUTER_BOUND('',#8607,.T.);
#5312=FACE_OUTER_BOUND('',#8608,.T.);
#5313=FACE_OUTER_BOUND('',#8609,.T.);
#5314=FACE_OUTER_BOUND('',#8610,.T.);
#5315=FACE_OUTER_BOUND('',#8611,.T.);
#5316=FACE_OUTER_BOUND('',#8612,.T.);
#5317=FACE_OUTER_BOUND('',#8613,.T.);
#5318=FACE_OUTER_BOUND('',#8614,.T.);
#5319=FACE_OUTER_BOUND('',#8615,.T.);
#5320=FACE_OUTER_BOUND('',#8616,.T.);
#5321=FACE_OUTER_BOUND('',#8617,.T.);
#5322=FACE_OUTER_BOUND('',#8618,.T.);
#5323=FACE_OUTER_BOUND('',#8619,.T.);
#5324=FACE_OUTER_BOUND('',#8620,.T.);
#5325=FACE_OUTER_BOUND('',#8621,.T.);
#5326=FACE_OUTER_BOUND('',#8622,.T.);
#5327=FACE_OUTER_BOUND('',#8623,.T.);
#5328=FACE_OUTER_BOUND('',#8624,.T.);
#5329=FACE_OUTER_BOUND('',#8625,.T.);
#5330=FACE_OUTER_BOUND('',#8626,.T.);
#5331=FACE_OUTER_BOUND('',#8627,.T.);
#5332=FACE_OUTER_BOUND('',#8628,.T.);
#5333=FACE_OUTER_BOUND('',#8629,.T.);
#5334=FACE_OUTER_BOUND('',#8630,.T.);
#5335=FACE_OUTER_BOUND('',#8631,.T.);
#5336=FACE_OUTER_BOUND('',#8632,.T.);
#5337=FACE_OUTER_BOUND('',#8633,.T.);
#5338=FACE_OUTER_BOUND('',#8634,.T.);
#5339=FACE_OUTER_BOUND('',#8635,.T.);
#5340=FACE_OUTER_BOUND('',#8636,.T.);
#5341=FACE_OUTER_BOUND('',#8637,.T.);
#5342=FACE_OUTER_BOUND('',#8638,.T.);
#5343=FACE_OUTER_BOUND('',#8639,.T.);
#5344=FACE_OUTER_BOUND('',#8640,.T.);
#5345=FACE_OUTER_BOUND('',#8641,.T.);
#5346=FACE_OUTER_BOUND('',#8642,.T.);
#5347=FACE_OUTER_BOUND('',#8643,.T.);
#5348=FACE_OUTER_BOUND('',#8644,.T.);
#5349=FACE_OUTER_BOUND('',#8645,.T.);
#5350=FACE_OUTER_BOUND('',#8646,.T.);
#5351=FACE_OUTER_BOUND('',#8647,.T.);
#5352=FACE_OUTER_BOUND('',#8648,.T.);
#5353=FACE_OUTER_BOUND('',#8649,.T.);
#5354=FACE_OUTER_BOUND('',#8650,.T.);
#5355=FACE_OUTER_BOUND('',#8651,.T.);
#5356=FACE_OUTER_BOUND('',#8652,.T.);
#5357=FACE_OUTER_BOUND('',#8653,.T.);
#5358=FACE_OUTER_BOUND('',#8654,.T.);
#5359=FACE_OUTER_BOUND('',#8655,.T.);
#5360=FACE_OUTER_BOUND('',#8656,.T.);
#5361=FACE_OUTER_BOUND('',#8657,.T.);
#5362=FACE_OUTER_BOUND('',#8658,.T.);
#5363=FACE_OUTER_BOUND('',#8659,.T.);
#5364=FACE_OUTER_BOUND('',#8660,.T.);
#5365=FACE_OUTER_BOUND('',#8661,.T.);
#5366=FACE_OUTER_BOUND('',#8662,.T.);
#5367=FACE_OUTER_BOUND('',#8663,.T.);
#5368=FACE_OUTER_BOUND('',#8664,.T.);
#5369=FACE_OUTER_BOUND('',#8665,.T.);
#5370=FACE_OUTER_BOUND('',#8666,.T.);
#5371=FACE_OUTER_BOUND('',#8667,.T.);
#5372=FACE_OUTER_BOUND('',#8668,.T.);
#5373=FACE_OUTER_BOUND('',#8669,.T.);
#5374=FACE_OUTER_BOUND('',#8670,.T.);
#5375=FACE_OUTER_BOUND('',#8671,.T.);
#5376=FACE_OUTER_BOUND('',#8672,.T.);
#5377=FACE_OUTER_BOUND('',#8673,.T.);
#5378=FACE_OUTER_BOUND('',#8674,.T.);
#5379=FACE_OUTER_BOUND('',#8675,.T.);
#5380=FACE_OUTER_BOUND('',#8676,.T.);
#5381=FACE_OUTER_BOUND('',#8677,.T.);
#5382=FACE_OUTER_BOUND('',#8678,.T.);
#5383=FACE_OUTER_BOUND('',#8679,.T.);
#5384=FACE_OUTER_BOUND('',#8680,.T.);
#5385=FACE_OUTER_BOUND('',#8681,.T.);
#5386=FACE_OUTER_BOUND('',#8682,.T.);
#5387=FACE_OUTER_BOUND('',#8683,.T.);
#5388=FACE_OUTER_BOUND('',#8684,.T.);
#5389=FACE_OUTER_BOUND('',#8685,.T.);
#5390=FACE_OUTER_BOUND('',#8686,.T.);
#5391=FACE_OUTER_BOUND('',#8687,.T.);
#5392=FACE_OUTER_BOUND('',#8688,.T.);
#5393=FACE_OUTER_BOUND('',#8689,.T.);
#5394=FACE_OUTER_BOUND('',#8690,.T.);
#5395=FACE_OUTER_BOUND('',#8691,.T.);
#5396=FACE_OUTER_BOUND('',#8692,.T.);
#5397=FACE_OUTER_BOUND('',#8693,.T.);
#5398=FACE_OUTER_BOUND('',#8694,.T.);
#5399=FACE_OUTER_BOUND('',#8695,.T.);
#5400=FACE_OUTER_BOUND('',#8696,.T.);
#5401=FACE_OUTER_BOUND('',#8697,.T.);
#5402=FACE_OUTER_BOUND('',#8698,.T.);
#5403=FACE_OUTER_BOUND('',#8699,.T.);
#5404=FACE_OUTER_BOUND('',#8700,.T.);
#5405=FACE_OUTER_BOUND('',#8701,.T.);
#5406=FACE_OUTER_BOUND('',#8702,.T.);
#5407=FACE_OUTER_BOUND('',#8703,.T.);
#5408=FACE_OUTER_BOUND('',#8704,.T.);
#5409=FACE_OUTER_BOUND('',#8705,.T.);
#5410=FACE_OUTER_BOUND('',#8706,.T.);
#5411=FACE_OUTER_BOUND('',#8707,.T.);
#5412=FACE_OUTER_BOUND('',#8708,.T.);
#5413=FACE_OUTER_BOUND('',#8709,.T.);
#5414=FACE_OUTER_BOUND('',#8710,.T.);
#5415=FACE_OUTER_BOUND('',#8711,.T.);
#5416=FACE_OUTER_BOUND('',#8712,.T.);
#5417=FACE_OUTER_BOUND('',#8713,.T.);
#5418=FACE_OUTER_BOUND('',#8714,.T.);
#5419=FACE_OUTER_BOUND('',#8715,.T.);
#5420=FACE_OUTER_BOUND('',#8716,.T.);
#5421=FACE_OUTER_BOUND('',#8717,.T.);
#5422=FACE_OUTER_BOUND('',#8718,.T.);
#5423=FACE_OUTER_BOUND('',#8719,.T.);
#5424=FACE_OUTER_BOUND('',#8720,.T.);
#5425=FACE_OUTER_BOUND('',#8721,.T.);
#5426=FACE_OUTER_BOUND('',#8722,.T.);
#5427=FACE_OUTER_BOUND('',#8723,.T.);
#5428=FACE_OUTER_BOUND('',#8724,.T.);
#5429=FACE_OUTER_BOUND('',#8725,.T.);
#5430=FACE_OUTER_BOUND('',#8726,.T.);
#5431=FACE_OUTER_BOUND('',#8727,.T.);
#5432=FACE_OUTER_BOUND('',#8728,.T.);
#5433=FACE_OUTER_BOUND('',#8729,.T.);
#5434=FACE_OUTER_BOUND('',#8730,.T.);
#5435=FACE_OUTER_BOUND('',#8731,.T.);
#5436=FACE_OUTER_BOUND('',#8732,.T.);
#5437=FACE_OUTER_BOUND('',#8733,.T.);
#5438=FACE_OUTER_BOUND('',#8734,.T.);
#5439=FACE_OUTER_BOUND('',#8735,.T.);
#5440=FACE_OUTER_BOUND('',#8736,.T.);
#5441=FACE_OUTER_BOUND('',#8737,.T.);
#5442=FACE_OUTER_BOUND('',#8738,.T.);
#5443=FACE_OUTER_BOUND('',#8739,.T.);
#5444=FACE_OUTER_BOUND('',#8740,.T.);
#5445=FACE_OUTER_BOUND('',#8741,.T.);
#5446=FACE_OUTER_BOUND('',#8742,.T.);
#5447=FACE_OUTER_BOUND('',#8743,.T.);
#5448=FACE_OUTER_BOUND('',#8744,.T.);
#5449=FACE_OUTER_BOUND('',#8745,.T.);
#5450=FACE_OUTER_BOUND('',#8746,.T.);
#5451=FACE_OUTER_BOUND('',#8747,.T.);
#5452=FACE_OUTER_BOUND('',#8748,.T.);
#5453=FACE_OUTER_BOUND('',#8749,.T.);
#5454=FACE_OUTER_BOUND('',#8750,.T.);
#5455=FACE_OUTER_BOUND('',#8751,.T.);
#5456=FACE_OUTER_BOUND('',#8752,.T.);
#5457=FACE_OUTER_BOUND('',#8753,.T.);
#5458=FACE_OUTER_BOUND('',#8754,.T.);
#5459=FACE_OUTER_BOUND('',#8755,.T.);
#5460=FACE_OUTER_BOUND('',#8756,.T.);
#5461=FACE_OUTER_BOUND('',#8757,.T.);
#5462=FACE_OUTER_BOUND('',#8758,.T.);
#5463=FACE_OUTER_BOUND('',#8759,.T.);
#5464=FACE_OUTER_BOUND('',#8760,.T.);
#5465=FACE_OUTER_BOUND('',#8761,.T.);
#5466=FACE_OUTER_BOUND('',#8762,.T.);
#5467=FACE_OUTER_BOUND('',#8763,.T.);
#5468=FACE_OUTER_BOUND('',#8764,.T.);
#5469=FACE_OUTER_BOUND('',#8765,.T.);
#5470=FACE_OUTER_BOUND('',#8766,.T.);
#5471=FACE_OUTER_BOUND('',#8767,.T.);
#5472=FACE_OUTER_BOUND('',#8768,.T.);
#5473=FACE_OUTER_BOUND('',#8769,.T.);
#5474=FACE_OUTER_BOUND('',#8770,.T.);
#5475=FACE_OUTER_BOUND('',#8771,.T.);
#5476=FACE_OUTER_BOUND('',#8772,.T.);
#5477=FACE_OUTER_BOUND('',#8773,.T.);
#5478=FACE_OUTER_BOUND('',#8774,.T.);
#5479=FACE_OUTER_BOUND('',#8775,.T.);
#5480=FACE_OUTER_BOUND('',#8776,.T.);
#5481=FACE_OUTER_BOUND('',#8777,.T.);
#5482=FACE_OUTER_BOUND('',#8778,.T.);
#5483=FACE_OUTER_BOUND('',#8779,.T.);
#5484=FACE_OUTER_BOUND('',#8780,.T.);
#5485=FACE_OUTER_BOUND('',#8781,.T.);
#5486=FACE_OUTER_BOUND('',#8782,.T.);
#5487=FACE_OUTER_BOUND('',#8783,.T.);
#5488=FACE_OUTER_BOUND('',#8784,.T.);
#5489=FACE_OUTER_BOUND('',#8785,.T.);
#5490=FACE_OUTER_BOUND('',#8786,.T.);
#5491=FACE_OUTER_BOUND('',#8787,.T.);
#5492=FACE_OUTER_BOUND('',#8788,.T.);
#5493=FACE_OUTER_BOUND('',#8789,.T.);
#5494=FACE_OUTER_BOUND('',#8790,.T.);
#5495=FACE_OUTER_BOUND('',#8791,.T.);
#5496=FACE_OUTER_BOUND('',#8792,.T.);
#5497=FACE_OUTER_BOUND('',#8793,.T.);
#5498=FACE_OUTER_BOUND('',#8794,.T.);
#5499=FACE_OUTER_BOUND('',#8795,.T.);
#5500=FACE_OUTER_BOUND('',#8796,.T.);
#5501=FACE_OUTER_BOUND('',#8797,.T.);
#5502=FACE_OUTER_BOUND('',#8798,.T.);
#5503=FACE_OUTER_BOUND('',#8799,.T.);
#5504=FACE_OUTER_BOUND('',#8800,.T.);
#5505=FACE_OUTER_BOUND('',#8801,.T.);
#5506=FACE_OUTER_BOUND('',#8802,.T.);
#5507=FACE_OUTER_BOUND('',#8803,.T.);
#5508=FACE_OUTER_BOUND('',#8804,.T.);
#5509=FACE_OUTER_BOUND('',#8805,.T.);
#5510=FACE_OUTER_BOUND('',#8806,.T.);
#5511=FACE_OUTER_BOUND('',#8807,.T.);
#5512=FACE_OUTER_BOUND('',#8808,.T.);
#5513=FACE_OUTER_BOUND('',#8809,.T.);
#5514=FACE_OUTER_BOUND('',#8810,.T.);
#5515=FACE_OUTER_BOUND('',#8811,.T.);
#5516=FACE_OUTER_BOUND('',#8812,.T.);
#5517=FACE_OUTER_BOUND('',#8813,.T.);
#5518=FACE_OUTER_BOUND('',#8814,.T.);
#5519=FACE_OUTER_BOUND('',#8815,.T.);
#5520=FACE_OUTER_BOUND('',#8816,.T.);
#5521=FACE_OUTER_BOUND('',#8817,.T.);
#5522=FACE_OUTER_BOUND('',#8818,.T.);
#5523=FACE_OUTER_BOUND('',#8819,.T.);
#5524=FACE_OUTER_BOUND('',#8820,.T.);
#5525=FACE_OUTER_BOUND('',#8821,.T.);
#5526=FACE_OUTER_BOUND('',#8822,.T.);
#5527=FACE_OUTER_BOUND('',#8823,.T.);
#5528=FACE_OUTER_BOUND('',#8824,.T.);
#5529=FACE_OUTER_BOUND('',#8825,.T.);
#5530=FACE_OUTER_BOUND('',#8826,.T.);
#5531=FACE_OUTER_BOUND('',#8827,.T.);
#5532=FACE_OUTER_BOUND('',#8828,.T.);
#5533=FACE_OUTER_BOUND('',#8829,.T.);
#5534=FACE_OUTER_BOUND('',#8830,.T.);
#5535=FACE_OUTER_BOUND('',#8831,.T.);
#5536=FACE_OUTER_BOUND('',#8832,.T.);
#5537=FACE_OUTER_BOUND('',#8833,.T.);
#5538=FACE_OUTER_BOUND('',#8834,.T.);
#5539=FACE_OUTER_BOUND('',#8835,.T.);
#5540=FACE_OUTER_BOUND('',#8836,.T.);
#5541=FACE_OUTER_BOUND('',#8837,.T.);
#5542=FACE_OUTER_BOUND('',#8838,.T.);
#5543=FACE_OUTER_BOUND('',#8839,.T.);
#5544=FACE_OUTER_BOUND('',#8840,.T.);
#5545=FACE_OUTER_BOUND('',#8841,.T.);
#5546=FACE_OUTER_BOUND('',#8842,.T.);
#5547=FACE_OUTER_BOUND('',#8843,.T.);
#5548=FACE_OUTER_BOUND('',#8844,.T.);
#5549=FACE_OUTER_BOUND('',#8845,.T.);
#5550=FACE_OUTER_BOUND('',#8846,.T.);
#5551=FACE_OUTER_BOUND('',#8847,.T.);
#5552=FACE_OUTER_BOUND('',#8848,.T.);
#5553=FACE_OUTER_BOUND('',#8849,.T.);
#5554=FACE_OUTER_BOUND('',#8850,.T.);
#5555=FACE_OUTER_BOUND('',#8851,.T.);
#5556=FACE_OUTER_BOUND('',#8852,.T.);
#5557=FACE_OUTER_BOUND('',#8853,.T.);
#5558=FACE_OUTER_BOUND('',#8854,.T.);
#5559=FACE_OUTER_BOUND('',#8855,.T.);
#5560=FACE_OUTER_BOUND('',#8856,.T.);
#5561=FACE_OUTER_BOUND('',#8857,.T.);
#5562=FACE_OUTER_BOUND('',#8858,.T.);
#5563=FACE_OUTER_BOUND('',#8859,.T.);
#5564=FACE_OUTER_BOUND('',#8860,.T.);
#5565=FACE_OUTER_BOUND('',#8861,.T.);
#5566=FACE_OUTER_BOUND('',#8862,.T.);
#5567=FACE_OUTER_BOUND('',#8863,.T.);
#5568=FACE_OUTER_BOUND('',#8864,.T.);
#5569=FACE_OUTER_BOUND('',#8865,.T.);
#5570=FACE_OUTER_BOUND('',#8866,.T.);
#5571=FACE_OUTER_BOUND('',#8867,.T.);
#5572=FACE_OUTER_BOUND('',#8868,.T.);
#5573=FACE_OUTER_BOUND('',#8869,.T.);
#5574=FACE_OUTER_BOUND('',#8870,.T.);
#5575=FACE_OUTER_BOUND('',#8871,.T.);
#5576=FACE_OUTER_BOUND('',#8872,.T.);
#5577=FACE_OUTER_BOUND('',#8873,.T.);
#5578=FACE_OUTER_BOUND('',#8874,.T.);
#5579=FACE_OUTER_BOUND('',#8875,.T.);
#5580=FACE_OUTER_BOUND('',#8876,.T.);
#5581=FACE_OUTER_BOUND('',#8877,.T.);
#5582=FACE_OUTER_BOUND('',#8878,.T.);
#5583=FACE_OUTER_BOUND('',#8879,.T.);
#5584=FACE_OUTER_BOUND('',#8880,.T.);
#5585=FACE_OUTER_BOUND('',#8881,.T.);
#5586=FACE_OUTER_BOUND('',#8882,.T.);
#5587=FACE_OUTER_BOUND('',#8883,.T.);
#5588=FACE_OUTER_BOUND('',#8884,.T.);
#5589=FACE_OUTER_BOUND('',#8885,.T.);
#5590=FACE_OUTER_BOUND('',#8886,.T.);
#5591=FACE_OUTER_BOUND('',#8887,.T.);
#5592=FACE_OUTER_BOUND('',#8888,.T.);
#5593=FACE_OUTER_BOUND('',#8889,.T.);
#5594=FACE_OUTER_BOUND('',#8890,.T.);
#5595=FACE_OUTER_BOUND('',#8891,.T.);
#5596=FACE_OUTER_BOUND('',#8892,.T.);
#5597=FACE_OUTER_BOUND('',#8893,.T.);
#5598=FACE_OUTER_BOUND('',#8894,.T.);
#5599=FACE_OUTER_BOUND('',#8895,.T.);
#5600=FACE_OUTER_BOUND('',#8896,.T.);
#5601=FACE_OUTER_BOUND('',#8897,.T.);
#5602=FACE_OUTER_BOUND('',#8898,.T.);
#5603=FACE_OUTER_BOUND('',#8899,.T.);
#5604=FACE_OUTER_BOUND('',#8900,.T.);
#5605=FACE_OUTER_BOUND('',#8901,.T.);
#5606=FACE_OUTER_BOUND('',#8902,.T.);
#5607=FACE_OUTER_BOUND('',#8903,.T.);
#5608=FACE_OUTER_BOUND('',#8904,.T.);
#5609=FACE_OUTER_BOUND('',#8905,.T.);
#5610=FACE_OUTER_BOUND('',#8906,.T.);
#5611=FACE_OUTER_BOUND('',#8907,.T.);
#5612=FACE_OUTER_BOUND('',#8908,.T.);
#5613=FACE_OUTER_BOUND('',#8909,.T.);
#5614=FACE_OUTER_BOUND('',#8910,.T.);
#5615=FACE_OUTER_BOUND('',#8911,.T.);
#5616=FACE_OUTER_BOUND('',#8912,.T.);
#5617=FACE_OUTER_BOUND('',#8913,.T.);
#5618=FACE_OUTER_BOUND('',#8914,.T.);
#5619=FACE_OUTER_BOUND('',#8915,.T.);
#5620=FACE_OUTER_BOUND('',#8916,.T.);
#5621=FACE_OUTER_BOUND('',#8917,.T.);
#5622=FACE_OUTER_BOUND('',#8918,.T.);
#5623=FACE_OUTER_BOUND('',#8919,.T.);
#5624=FACE_OUTER_BOUND('',#8920,.T.);
#5625=FACE_OUTER_BOUND('',#8921,.T.);
#5626=FACE_OUTER_BOUND('',#8922,.T.);
#5627=FACE_OUTER_BOUND('',#8923,.T.);
#5628=FACE_OUTER_BOUND('',#8924,.T.);
#5629=FACE_OUTER_BOUND('',#8925,.T.);
#5630=FACE_OUTER_BOUND('',#8926,.T.);
#5631=FACE_OUTER_BOUND('',#8927,.T.);
#5632=FACE_OUTER_BOUND('',#8928,.T.);
#5633=FACE_OUTER_BOUND('',#8929,.T.);
#5634=FACE_OUTER_BOUND('',#8930,.T.);
#5635=FACE_OUTER_BOUND('',#8931,.T.);
#5636=FACE_OUTER_BOUND('',#8932,.T.);
#5637=FACE_OUTER_BOUND('',#8933,.T.);
#5638=FACE_OUTER_BOUND('',#8934,.T.);
#5639=FACE_OUTER_BOUND('',#8935,.T.);
#5640=FACE_OUTER_BOUND('',#8936,.T.);
#5641=FACE_OUTER_BOUND('',#8937,.T.);
#5642=FACE_OUTER_BOUND('',#8938,.T.);
#5643=FACE_OUTER_BOUND('',#8939,.T.);
#5644=FACE_OUTER_BOUND('',#8940,.T.);
#5645=FACE_OUTER_BOUND('',#8941,.T.);
#5646=FACE_OUTER_BOUND('',#8942,.T.);
#5647=FACE_OUTER_BOUND('',#8943,.T.);
#5648=FACE_OUTER_BOUND('',#8944,.T.);
#5649=FACE_OUTER_BOUND('',#8945,.T.);
#5650=FACE_OUTER_BOUND('',#8946,.T.);
#5651=FACE_OUTER_BOUND('',#8947,.T.);
#5652=FACE_OUTER_BOUND('',#8948,.T.);
#5653=FACE_OUTER_BOUND('',#8949,.T.);
#5654=FACE_OUTER_BOUND('',#8950,.T.);
#5655=FACE_OUTER_BOUND('',#8951,.T.);
#5656=FACE_OUTER_BOUND('',#8952,.T.);
#5657=FACE_OUTER_BOUND('',#8953,.T.);
#5658=FACE_OUTER_BOUND('',#8954,.T.);
#5659=FACE_OUTER_BOUND('',#8955,.T.);
#5660=FACE_OUTER_BOUND('',#8956,.T.);
#5661=FACE_OUTER_BOUND('',#8957,.T.);
#5662=FACE_OUTER_BOUND('',#8958,.T.);
#5663=FACE_OUTER_BOUND('',#8959,.T.);
#5664=FACE_OUTER_BOUND('',#8960,.T.);
#5665=FACE_OUTER_BOUND('',#8961,.T.);
#5666=FACE_OUTER_BOUND('',#8962,.T.);
#5667=FACE_OUTER_BOUND('',#8963,.T.);
#5668=FACE_OUTER_BOUND('',#8964,.T.);
#5669=FACE_OUTER_BOUND('',#8965,.T.);
#5670=FACE_OUTER_BOUND('',#8966,.T.);
#5671=FACE_OUTER_BOUND('',#8967,.T.);
#5672=FACE_OUTER_BOUND('',#8968,.T.);
#5673=FACE_OUTER_BOUND('',#8969,.T.);
#5674=FACE_OUTER_BOUND('',#8970,.T.);
#5675=FACE_OUTER_BOUND('',#8971,.T.);
#5676=FACE_OUTER_BOUND('',#8972,.T.);
#5677=FACE_OUTER_BOUND('',#8973,.T.);
#5678=FACE_OUTER_BOUND('',#8974,.T.);
#5679=FACE_OUTER_BOUND('',#8975,.T.);
#5680=FACE_OUTER_BOUND('',#8976,.T.);
#5681=FACE_OUTER_BOUND('',#8977,.T.);
#5682=FACE_OUTER_BOUND('',#8978,.T.);
#5683=FACE_OUTER_BOUND('',#8979,.T.);
#5684=FACE_OUTER_BOUND('',#8980,.T.);
#5685=FACE_OUTER_BOUND('',#8981,.T.);
#5686=FACE_OUTER_BOUND('',#8982,.T.);
#5687=FACE_OUTER_BOUND('',#8983,.T.);
#5688=FACE_OUTER_BOUND('',#8984,.T.);
#5689=FACE_OUTER_BOUND('',#8985,.T.);
#5690=FACE_OUTER_BOUND('',#8986,.T.);
#5691=FACE_OUTER_BOUND('',#8987,.T.);
#5692=FACE_OUTER_BOUND('',#8988,.T.);
#5693=FACE_OUTER_BOUND('',#8989,.T.);
#5694=FACE_OUTER_BOUND('',#8990,.T.);
#5695=FACE_OUTER_BOUND('',#8991,.T.);
#5696=FACE_OUTER_BOUND('',#8992,.T.);
#5697=FACE_OUTER_BOUND('',#8993,.T.);
#5698=FACE_OUTER_BOUND('',#8994,.T.);
#5699=FACE_OUTER_BOUND('',#8995,.T.);
#5700=FACE_OUTER_BOUND('',#8996,.T.);
#5701=FACE_OUTER_BOUND('',#8997,.T.);
#5702=FACE_OUTER_BOUND('',#8998,.T.);
#5703=FACE_OUTER_BOUND('',#8999,.T.);
#5704=FACE_OUTER_BOUND('',#9000,.T.);
#5705=FACE_OUTER_BOUND('',#9001,.T.);
#5706=FACE_OUTER_BOUND('',#9002,.T.);
#5707=FACE_OUTER_BOUND('',#9003,.T.);
#5708=FACE_OUTER_BOUND('',#9004,.T.);
#5709=FACE_OUTER_BOUND('',#9005,.T.);
#5710=FACE_OUTER_BOUND('',#9006,.T.);
#5711=FACE_OUTER_BOUND('',#9007,.T.);
#5712=FACE_OUTER_BOUND('',#9008,.T.);
#5713=FACE_OUTER_BOUND('',#9009,.T.);
#5714=FACE_OUTER_BOUND('',#9010,.T.);
#5715=FACE_OUTER_BOUND('',#9011,.T.);
#5716=FACE_OUTER_BOUND('',#9012,.T.);
#5717=FACE_OUTER_BOUND('',#9013,.T.);
#5718=FACE_OUTER_BOUND('',#9014,.T.);
#5719=FACE_OUTER_BOUND('',#9015,.T.);
#5720=FACE_OUTER_BOUND('',#9016,.T.);
#5721=FACE_OUTER_BOUND('',#9017,.T.);
#5722=FACE_OUTER_BOUND('',#9018,.T.);
#5723=FACE_OUTER_BOUND('',#9019,.T.);
#5724=FACE_OUTER_BOUND('',#9020,.T.);
#5725=FACE_OUTER_BOUND('',#9021,.T.);
#5726=FACE_OUTER_BOUND('',#9022,.T.);
#5727=FACE_OUTER_BOUND('',#9023,.T.);
#5728=FACE_OUTER_BOUND('',#9024,.T.);
#5729=FACE_OUTER_BOUND('',#9025,.T.);
#5730=FACE_OUTER_BOUND('',#9026,.T.);
#5731=FACE_OUTER_BOUND('',#9027,.T.);
#5732=FACE_OUTER_BOUND('',#9028,.T.);
#5733=FACE_OUTER_BOUND('',#9029,.T.);
#5734=FACE_OUTER_BOUND('',#9030,.T.);
#5735=FACE_OUTER_BOUND('',#9031,.T.);
#5736=FACE_OUTER_BOUND('',#9032,.T.);
#5737=FACE_OUTER_BOUND('',#9033,.T.);
#5738=FACE_OUTER_BOUND('',#9034,.T.);
#5739=FACE_OUTER_BOUND('',#9035,.T.);
#5740=FACE_OUTER_BOUND('',#9036,.T.);
#5741=FACE_OUTER_BOUND('',#9037,.T.);
#5742=FACE_OUTER_BOUND('',#9038,.T.);
#5743=FACE_OUTER_BOUND('',#9039,.T.);
#5744=FACE_OUTER_BOUND('',#9040,.T.);
#5745=FACE_OUTER_BOUND('',#9041,.T.);
#5746=FACE_OUTER_BOUND('',#9042,.T.);
#5747=FACE_OUTER_BOUND('',#9043,.T.);
#5748=FACE_OUTER_BOUND('',#9044,.T.);
#5749=FACE_OUTER_BOUND('',#9045,.T.);
#5750=FACE_OUTER_BOUND('',#9046,.T.);
#5751=FACE_OUTER_BOUND('',#9047,.T.);
#5752=FACE_OUTER_BOUND('',#9048,.T.);
#5753=FACE_OUTER_BOUND('',#9049,.T.);
#5754=FACE_OUTER_BOUND('',#9050,.T.);
#5755=FACE_OUTER_BOUND('',#9051,.T.);
#5756=FACE_OUTER_BOUND('',#9052,.T.);
#5757=FACE_OUTER_BOUND('',#9053,.T.);
#5758=FACE_OUTER_BOUND('',#9054,.T.);
#5759=FACE_OUTER_BOUND('',#9055,.T.);
#5760=FACE_OUTER_BOUND('',#9056,.T.);
#5761=FACE_OUTER_BOUND('',#9057,.T.);
#5762=FACE_OUTER_BOUND('',#9058,.T.);
#5763=FACE_OUTER_BOUND('',#9059,.T.);
#5764=FACE_OUTER_BOUND('',#9060,.T.);
#5765=FACE_OUTER_BOUND('',#9061,.T.);
#5766=FACE_OUTER_BOUND('',#9062,.T.);
#5767=FACE_OUTER_BOUND('',#9063,.T.);
#5768=FACE_OUTER_BOUND('',#9064,.T.);
#5769=FACE_OUTER_BOUND('',#9065,.T.);
#5770=FACE_OUTER_BOUND('',#9066,.T.);
#5771=FACE_OUTER_BOUND('',#9067,.T.);
#5772=FACE_OUTER_BOUND('',#9068,.T.);
#5773=FACE_OUTER_BOUND('',#9069,.T.);
#5774=FACE_OUTER_BOUND('',#9070,.T.);
#5775=FACE_OUTER_BOUND('',#9071,.T.);
#5776=FACE_OUTER_BOUND('',#9072,.T.);
#5777=FACE_OUTER_BOUND('',#9073,.T.);
#5778=FACE_OUTER_BOUND('',#9074,.T.);
#5779=FACE_OUTER_BOUND('',#9075,.T.);
#5780=FACE_OUTER_BOUND('',#9076,.T.);
#5781=FACE_OUTER_BOUND('',#9077,.T.);
#5782=FACE_OUTER_BOUND('',#9081,.T.);
#5783=FACE_OUTER_BOUND('',#9082,.T.);
#5784=FACE_OUTER_BOUND('',#9083,.T.);
#5785=FACE_OUTER_BOUND('',#9084,.T.);
#5786=FACE_OUTER_BOUND('',#9085,.T.);
#5787=FACE_OUTER_BOUND('',#9086,.T.);
#5788=FACE_OUTER_BOUND('',#9087,.T.);
#5789=FACE_OUTER_BOUND('',#9090,.T.);
#5790=FACE_OUTER_BOUND('',#9091,.T.);
#5791=FACE_OUTER_BOUND('',#9092,.T.);
#5792=FACE_OUTER_BOUND('',#9093,.T.);
#5793=FACE_OUTER_BOUND('',#9094,.T.);
#5794=FACE_OUTER_BOUND('',#9095,.T.);
#5795=FACE_OUTER_BOUND('',#9097,.T.);
#5796=FACE_OUTER_BOUND('',#9098,.T.);
#5797=FACE_OUTER_BOUND('',#9100,.T.);
#5798=FACE_OUTER_BOUND('',#9101,.T.);
#5799=FACE_OUTER_BOUND('',#9103,.T.);
#5800=FACE_OUTER_BOUND('',#9104,.T.);
#5801=FACE_OUTER_BOUND('',#9106,.T.);
#5802=FACE_OUTER_BOUND('',#9107,.T.);
#5803=FACE_OUTER_BOUND('',#9109,.T.);
#5804=FACE_OUTER_BOUND('',#9110,.T.);
#5805=FACE_OUTER_BOUND('',#9112,.T.);
#5806=FACE_OUTER_BOUND('',#9113,.T.);
#5807=FACE_OUTER_BOUND('',#9117,.T.);
#5808=FACE_OUTER_BOUND('',#9118,.T.);
#5809=FACE_OUTER_BOUND('',#9119,.T.);
#5810=FACE_OUTER_BOUND('',#9120,.T.);
#5811=FACE_OUTER_BOUND('',#9121,.T.);
#5812=FACE_OUTER_BOUND('',#9122,.T.);
#5813=FACE_OUTER_BOUND('',#9123,.T.);
#5814=FACE_OUTER_BOUND('',#9124,.T.);
#5815=FACE_OUTER_BOUND('',#9125,.T.);
#5816=FACE_OUTER_BOUND('',#9126,.T.);
#5817=FACE_OUTER_BOUND('',#9127,.T.);
#5818=FACE_OUTER_BOUND('',#9128,.T.);
#5819=FACE_OUTER_BOUND('',#9129,.T.);
#5820=FACE_OUTER_BOUND('',#9130,.T.);
#5821=FACE_OUTER_BOUND('',#9131,.T.);
#5822=FACE_OUTER_BOUND('',#9132,.T.);
#5823=FACE_OUTER_BOUND('',#9133,.T.);
#5824=FACE_OUTER_BOUND('',#9134,.T.);
#5825=FACE_OUTER_BOUND('',#9135,.T.);
#5826=FACE_OUTER_BOUND('',#9136,.T.);
#5827=FACE_OUTER_BOUND('',#9137,.T.);
#5828=FACE_OUTER_BOUND('',#9138,.T.);
#5829=FACE_OUTER_BOUND('',#9139,.T.);
#5830=FACE_OUTER_BOUND('',#9140,.T.);
#5831=FACE_OUTER_BOUND('',#9141,.T.);
#5832=FACE_OUTER_BOUND('',#9142,.T.);
#5833=FACE_OUTER_BOUND('',#9143,.T.);
#5834=FACE_OUTER_BOUND('',#9144,.T.);
#5835=FACE_OUTER_BOUND('',#9145,.T.);
#5836=FACE_OUTER_BOUND('',#9146,.T.);
#5837=FACE_OUTER_BOUND('',#9147,.T.);
#5838=FACE_OUTER_BOUND('',#9148,.T.);
#5839=FACE_OUTER_BOUND('',#9149,.T.);
#5840=FACE_OUTER_BOUND('',#9150,.T.);
#5841=FACE_OUTER_BOUND('',#9151,.T.);
#5842=FACE_OUTER_BOUND('',#9156,.T.);
#5843=FACE_OUTER_BOUND('',#9157,.T.);
#5844=FACE_OUTER_BOUND('',#9158,.T.);
#5845=FACE_OUTER_BOUND('',#9159,.T.);
#5846=FACE_OUTER_BOUND('',#9160,.T.);
#5847=FACE_OUTER_BOUND('',#9379,.T.);
#5848=FACE_OUTER_BOUND('',#9380,.T.);
#5849=FACE_OUTER_BOUND('',#9385,.T.);
#5850=FACE_OUTER_BOUND('',#9386,.T.);
#5851=FACE_OUTER_BOUND('',#9387,.T.);
#5852=FACE_OUTER_BOUND('',#9388,.T.);
#5853=FACE_OUTER_BOUND('',#9389,.T.);
#5854=FACE_OUTER_BOUND('',#9390,.T.);
#5855=FACE_OUTER_BOUND('',#9391,.T.);
#5856=FACE_OUTER_BOUND('',#9392,.T.);
#5857=FACE_OUTER_BOUND('',#9393,.T.);
#5858=FACE_OUTER_BOUND('',#9394,.T.);
#5859=FACE_OUTER_BOUND('',#9395,.T.);
#5860=FACE_OUTER_BOUND('',#9396,.T.);
#5861=FACE_OUTER_BOUND('',#9397,.T.);
#5862=FACE_OUTER_BOUND('',#9398,.T.);
#5863=FACE_OUTER_BOUND('',#9399,.T.);
#5864=FACE_OUTER_BOUND('',#9400,.T.);
#5865=FACE_OUTER_BOUND('',#9401,.T.);
#5866=FACE_OUTER_BOUND('',#9402,.T.);
#5867=FACE_OUTER_BOUND('',#9403,.T.);
#5868=FACE_OUTER_BOUND('',#9404,.T.);
#5869=FACE_OUTER_BOUND('',#9405,.T.);
#5870=FACE_OUTER_BOUND('',#9406,.T.);
#5871=FACE_OUTER_BOUND('',#9407,.T.);
#7292=EDGE_LOOP('',(#39039,#39040,#39041,#39042));
#7293=EDGE_LOOP('',(#39043,#39044,#39045,#39046));
#7294=EDGE_LOOP('',(#39047,#39048,#39049,#39050));
#7295=EDGE_LOOP('',(#39051,#39052,#39053,#39054));
#7296=EDGE_LOOP('',(#39055,#39056,#39057,#39058));
#7297=EDGE_LOOP('',(#39059,#39060,#39061,#39062));
#7298=EDGE_LOOP('',(#39063,#39064,#39065,#39066));
#7299=EDGE_LOOP('',(#39067,#39068,#39069,#39070));
#7300=EDGE_LOOP('',(#39071,#39072,#39073,#39074));
#7301=EDGE_LOOP('',(#39075,#39076,#39077,#39078));
#7302=EDGE_LOOP('',(#39079,#39080,#39081,#39082));
#7303=EDGE_LOOP('',(#39083,#39084,#39085,#39086));
#7304=EDGE_LOOP('',(#39087,#39088,#39089,#39090));
#7305=EDGE_LOOP('',(#39091,#39092,#39093,#39094));
#7306=EDGE_LOOP('',(#39095,#39096,#39097,#39098));
#7307=EDGE_LOOP('',(#39099,#39100,#39101,#39102));
#7308=EDGE_LOOP('',(#39103,#39104,#39105,#39106));
#7309=EDGE_LOOP('',(#39107,#39108,#39109,#39110));
#7310=EDGE_LOOP('',(#39111,#39112,#39113,#39114));
#7311=EDGE_LOOP('',(#39115,#39116,#39117,#39118));
#7312=EDGE_LOOP('',(#39119,#39120,#39121,#39122,#39123,#39124,#39125,#39126,
#39127,#39128,#39129,#39130));
#7313=EDGE_LOOP('',(#39131,#39132,#39133,#39134,#39135,#39136,#39137,#39138));
#7314=EDGE_LOOP('',(#39139,#39140,#39141,#39142));
#7315=EDGE_LOOP('',(#39143,#39144,#39145,#39146));
#7316=EDGE_LOOP('',(#39147,#39148,#39149,#39150));
#7317=EDGE_LOOP('',(#39151,#39152,#39153,#39154));
#7318=EDGE_LOOP('',(#39155,#39156,#39157,#39158));
#7319=EDGE_LOOP('',(#39159,#39160,#39161,#39162));
#7320=EDGE_LOOP('',(#39163,#39164,#39165,#39166));
#7321=EDGE_LOOP('',(#39167,#39168,#39169,#39170));
#7322=EDGE_LOOP('',(#39171,#39172,#39173,#39174));
#7323=EDGE_LOOP('',(#39175,#39176,#39177,#39178));
#7324=EDGE_LOOP('',(#39179,#39180,#39181,#39182));
#7325=EDGE_LOOP('',(#39183,#39184,#39185,#39186));
#7326=EDGE_LOOP('',(#39187,#39188,#39189,#39190));
#7327=EDGE_LOOP('',(#39191,#39192,#39193,#39194));
#7328=EDGE_LOOP('',(#39195,#39196,#39197,#39198));
#7329=EDGE_LOOP('',(#39199,#39200,#39201,#39202));
#7330=EDGE_LOOP('',(#39203,#39204,#39205,#39206));
#7331=EDGE_LOOP('',(#39207,#39208,#39209,#39210));
#7332=EDGE_LOOP('',(#39211,#39212,#39213,#39214));
#7333=EDGE_LOOP('',(#39215,#39216,#39217,#39218));
#7334=EDGE_LOOP('',(#39219,#39220,#39221,#39222));
#7335=EDGE_LOOP('',(#39223,#39224,#39225,#39226));
#7336=EDGE_LOOP('',(#39227,#39228,#39229,#39230));
#7337=EDGE_LOOP('',(#39231,#39232,#39233,#39234));
#7338=EDGE_LOOP('',(#39235,#39236,#39237,#39238));
#7339=EDGE_LOOP('',(#39239,#39240,#39241,#39242));
#7340=EDGE_LOOP('',(#39243,#39244,#39245,#39246));
#7341=EDGE_LOOP('',(#39247,#39248,#39249,#39250));
#7342=EDGE_LOOP('',(#39251,#39252,#39253,#39254));
#7343=EDGE_LOOP('',(#39255,#39256,#39257,#39258));
#7344=EDGE_LOOP('',(#39259,#39260,#39261,#39262,#39263,#39264,#39265,#39266,
#39267,#39268,#39269,#39270,#39271,#39272,#39273,#39274,#39275,#39276,#39277,
#39278,#39279,#39280));
#7345=EDGE_LOOP('',(#39281,#39282,#39283,#39284,#39285,#39286,#39287,#39288));
#7346=EDGE_LOOP('',(#39289,#39290,#39291,#39292,#39293,#39294,#39295,#39296));
#7347=EDGE_LOOP('',(#39297,#39298,#39299,#39300,#39301,#39302,#39303,#39304));
#7348=EDGE_LOOP('',(#39305,#39306,#39307,#39308));
#7349=EDGE_LOOP('',(#39309,#39310,#39311,#39312));
#7350=EDGE_LOOP('',(#39313,#39314,#39315,#39316));
#7351=EDGE_LOOP('',(#39317,#39318,#39319,#39320));
#7352=EDGE_LOOP('',(#39321,#39322,#39323,#39324));
#7353=EDGE_LOOP('',(#39325,#39326,#39327,#39328));
#7354=EDGE_LOOP('',(#39329,#39330,#39331,#39332));
#7355=EDGE_LOOP('',(#39333,#39334,#39335,#39336));
#7356=EDGE_LOOP('',(#39337,#39338,#39339,#39340));
#7357=EDGE_LOOP('',(#39341,#39342,#39343,#39344));
#7358=EDGE_LOOP('',(#39345,#39346,#39347,#39348));
#7359=EDGE_LOOP('',(#39349,#39350,#39351,#39352));
#7360=EDGE_LOOP('',(#39353,#39354,#39355,#39356));
#7361=EDGE_LOOP('',(#39357,#39358,#39359,#39360));
#7362=EDGE_LOOP('',(#39361,#39362,#39363,#39364));
#7363=EDGE_LOOP('',(#39365,#39366,#39367,#39368));
#7364=EDGE_LOOP('',(#39369,#39370,#39371,#39372));
#7365=EDGE_LOOP('',(#39373,#39374,#39375,#39376));
#7366=EDGE_LOOP('',(#39377,#39378,#39379,#39380));
#7367=EDGE_LOOP('',(#39381,#39382,#39383,#39384));
#7368=EDGE_LOOP('',(#39385,#39386,#39387,#39388,#39389,#39390,#39391,#39392,
#39393,#39394,#39395,#39396));
#7369=EDGE_LOOP('',(#39397,#39398,#39399,#39400,#39401,#39402,#39403,#39404));
#7370=EDGE_LOOP('',(#39405,#39406,#39407,#39408));
#7371=EDGE_LOOP('',(#39409,#39410,#39411,#39412));
#7372=EDGE_LOOP('',(#39413,#39414,#39415,#39416));
#7373=EDGE_LOOP('',(#39417,#39418,#39419,#39420));
#7374=EDGE_LOOP('',(#39421,#39422,#39423,#39424));
#7375=EDGE_LOOP('',(#39425,#39426,#39427,#39428));
#7376=EDGE_LOOP('',(#39429,#39430,#39431,#39432));
#7377=EDGE_LOOP('',(#39433,#39434,#39435,#39436));
#7378=EDGE_LOOP('',(#39437,#39438,#39439,#39440));
#7379=EDGE_LOOP('',(#39441,#39442,#39443,#39444));
#7380=EDGE_LOOP('',(#39445,#39446,#39447,#39448));
#7381=EDGE_LOOP('',(#39449,#39450,#39451,#39452));
#7382=EDGE_LOOP('',(#39453,#39454,#39455,#39456));
#7383=EDGE_LOOP('',(#39457,#39458,#39459,#39460));
#7384=EDGE_LOOP('',(#39461,#39462,#39463,#39464));
#7385=EDGE_LOOP('',(#39465,#39466,#39467,#39468));
#7386=EDGE_LOOP('',(#39469,#39470,#39471,#39472));
#7387=EDGE_LOOP('',(#39473,#39474,#39475,#39476));
#7388=EDGE_LOOP('',(#39477,#39478,#39479,#39480));
#7389=EDGE_LOOP('',(#39481,#39482,#39483,#39484));
#7390=EDGE_LOOP('',(#39485,#39486,#39487,#39488));
#7391=EDGE_LOOP('',(#39489,#39490,#39491,#39492));
#7392=EDGE_LOOP('',(#39493,#39494,#39495,#39496));
#7393=EDGE_LOOP('',(#39497,#39498,#39499,#39500));
#7394=EDGE_LOOP('',(#39501,#39502,#39503,#39504));
#7395=EDGE_LOOP('',(#39505,#39506,#39507,#39508));
#7396=EDGE_LOOP('',(#39509,#39510,#39511,#39512));
#7397=EDGE_LOOP('',(#39513,#39514,#39515,#39516));
#7398=EDGE_LOOP('',(#39517,#39518,#39519,#39520));
#7399=EDGE_LOOP('',(#39521,#39522,#39523,#39524));
#7400=EDGE_LOOP('',(#39525,#39526,#39527,#39528));
#7401=EDGE_LOOP('',(#39529,#39530,#39531,#39532));
#7402=EDGE_LOOP('',(#39533,#39534,#39535,#39536));
#7403=EDGE_LOOP('',(#39537,#39538,#39539,#39540,#39541,#39542,#39543,#39544,
#39545,#39546,#39547,#39548,#39549,#39550,#39551,#39552));
#7404=EDGE_LOOP('',(#39553,#39554,#39555,#39556,#39557,#39558,#39559,#39560,
#39561));
#7405=EDGE_LOOP('',(#39562,#39563,#39564,#39565,#39566,#39567,#39568,#39569));
#7406=EDGE_LOOP('',(#39570,#39571,#39572,#39573,#39574,#39575,#39576,#39577,
#39578));
#7407=EDGE_LOOP('',(#39579,#39580,#39581,#39582,#39583,#39584,#39585,#39586));
#7408=EDGE_LOOP('',(#39587,#39588,#39589,#39590,#39591,#39592,#39593,#39594));
#7409=EDGE_LOOP('',(#39595,#39596,#39597,#39598));
#7410=EDGE_LOOP('',(#39599,#39600,#39601,#39602));
#7411=EDGE_LOOP('',(#39603,#39604,#39605,#39606));
#7412=EDGE_LOOP('',(#39607,#39608,#39609,#39610));
#7413=EDGE_LOOP('',(#39611,#39612,#39613,#39614));
#7414=EDGE_LOOP('',(#39615,#39616,#39617,#39618));
#7415=EDGE_LOOP('',(#39619,#39620,#39621,#39622));
#7416=EDGE_LOOP('',(#39623,#39624,#39625,#39626));
#7417=EDGE_LOOP('',(#39627,#39628,#39629,#39630));
#7418=EDGE_LOOP('',(#39631,#39632,#39633,#39634));
#7419=EDGE_LOOP('',(#39635,#39636,#39637,#39638));
#7420=EDGE_LOOP('',(#39639,#39640,#39641,#39642));
#7421=EDGE_LOOP('',(#39643,#39644,#39645,#39646));
#7422=EDGE_LOOP('',(#39647,#39648,#39649,#39650));
#7423=EDGE_LOOP('',(#39651,#39652,#39653,#39654));
#7424=EDGE_LOOP('',(#39655,#39656,#39657,#39658));
#7425=EDGE_LOOP('',(#39659,#39660,#39661,#39662));
#7426=EDGE_LOOP('',(#39663,#39664,#39665,#39666));
#7427=EDGE_LOOP('',(#39667,#39668,#39669,#39670));
#7428=EDGE_LOOP('',(#39671,#39672,#39673,#39674));
#7429=EDGE_LOOP('',(#39675,#39676,#39677,#39678,#39679,#39680,#39681,#39682,
#39683,#39684,#39685,#39686));
#7430=EDGE_LOOP('',(#39687,#39688,#39689,#39690,#39691,#39692,#39693,#39694));
#7431=EDGE_LOOP('',(#39695,#39696,#39697,#39698));
#7432=EDGE_LOOP('',(#39699,#39700,#39701,#39702));
#7433=EDGE_LOOP('',(#39703,#39704,#39705,#39706));
#7434=EDGE_LOOP('',(#39707,#39708,#39709,#39710));
#7435=EDGE_LOOP('',(#39711,#39712,#39713,#39714));
#7436=EDGE_LOOP('',(#39715,#39716,#39717,#39718));
#7437=EDGE_LOOP('',(#39719,#39720,#39721,#39722));
#7438=EDGE_LOOP('',(#39723,#39724,#39725,#39726));
#7439=EDGE_LOOP('',(#39727,#39728,#39729,#39730));
#7440=EDGE_LOOP('',(#39731,#39732,#39733,#39734));
#7441=EDGE_LOOP('',(#39735,#39736,#39737,#39738));
#7442=EDGE_LOOP('',(#39739,#39740,#39741,#39742,#39743,#39744,#39745,#39746,
#39747,#39748,#39749));
#7443=EDGE_LOOP('',(#39750,#39751,#39752,#39753,#39754,#39755,#39756,#39757));
#7444=EDGE_LOOP('',(#39758,#39759,#39760,#39761));
#7445=EDGE_LOOP('',(#39762,#39763,#39764,#39765));
#7446=EDGE_LOOP('',(#39766,#39767,#39768,#39769));
#7447=EDGE_LOOP('',(#39770,#39771,#39772,#39773));
#7448=EDGE_LOOP('',(#39774,#39775,#39776,#39777));
#7449=EDGE_LOOP('',(#39778,#39779,#39780,#39781));
#7450=EDGE_LOOP('',(#39782,#39783,#39784,#39785));
#7451=EDGE_LOOP('',(#39786,#39787,#39788,#39789));
#7452=EDGE_LOOP('',(#39790,#39791,#39792,#39793));
#7453=EDGE_LOOP('',(#39794,#39795,#39796,#39797));
#7454=EDGE_LOOP('',(#39798,#39799,#39800,#39801));
#7455=EDGE_LOOP('',(#39802,#39803,#39804,#39805));
#7456=EDGE_LOOP('',(#39806,#39807,#39808,#39809));
#7457=EDGE_LOOP('',(#39810,#39811,#39812,#39813));
#7458=EDGE_LOOP('',(#39814,#39815,#39816,#39817));
#7459=EDGE_LOOP('',(#39818,#39819,#39820,#39821));
#7460=EDGE_LOOP('',(#39822,#39823,#39824,#39825));
#7461=EDGE_LOOP('',(#39826,#39827,#39828,#39829));
#7462=EDGE_LOOP('',(#39830,#39831,#39832,#39833));
#7463=EDGE_LOOP('',(#39834,#39835,#39836,#39837));
#7464=EDGE_LOOP('',(#39838,#39839,#39840,#39841,#39842,#39843,#39844,#39845,
#39846,#39847,#39848,#39849));
#7465=EDGE_LOOP('',(#39850,#39851,#39852,#39853,#39854,#39855,#39856,#39857));
#7466=EDGE_LOOP('',(#39858,#39859,#39860,#39861));
#7467=EDGE_LOOP('',(#39862,#39863,#39864,#39865));
#7468=EDGE_LOOP('',(#39866,#39867,#39868,#39869));
#7469=EDGE_LOOP('',(#39870,#39871,#39872,#39873));
#7470=EDGE_LOOP('',(#39874,#39875,#39876,#39877));
#7471=EDGE_LOOP('',(#39878,#39879,#39880,#39881));
#7472=EDGE_LOOP('',(#39882,#39883,#39884,#39885));
#7473=EDGE_LOOP('',(#39886,#39887,#39888,#39889));
#7474=EDGE_LOOP('',(#39890,#39891,#39892,#39893));
#7475=EDGE_LOOP('',(#39894,#39895,#39896,#39897));
#7476=EDGE_LOOP('',(#39898,#39899,#39900,#39901));
#7477=EDGE_LOOP('',(#39902,#39903,#39904,#39905));
#7478=EDGE_LOOP('',(#39906,#39907,#39908,#39909));
#7479=EDGE_LOOP('',(#39910,#39911,#39912,#39913));
#7480=EDGE_LOOP('',(#39914,#39915,#39916,#39917));
#7481=EDGE_LOOP('',(#39918,#39919,#39920,#39921));
#7482=EDGE_LOOP('',(#39922,#39923,#39924,#39925));
#7483=EDGE_LOOP('',(#39926,#39927,#39928,#39929));
#7484=EDGE_LOOP('',(#39930,#39931,#39932,#39933));
#7485=EDGE_LOOP('',(#39934,#39935,#39936,#39937));
#7486=EDGE_LOOP('',(#39938,#39939,#39940,#39941));
#7487=EDGE_LOOP('',(#39942,#39943,#39944,#39945));
#7488=EDGE_LOOP('',(#39946,#39947,#39948,#39949));
#7489=EDGE_LOOP('',(#39950,#39951,#39952,#39953));
#7490=EDGE_LOOP('',(#39954,#39955,#39956,#39957));
#7491=EDGE_LOOP('',(#39958,#39959,#39960,#39961));
#7492=EDGE_LOOP('',(#39962,#39963,#39964,#39965));
#7493=EDGE_LOOP('',(#39966,#39967,#39968,#39969));
#7494=EDGE_LOOP('',(#39970,#39971,#39972,#39973,#39974,#39975,#39976,#39977,
#39978,#39979,#39980,#39981,#39982,#39983,#39984,#39985,#39986,#39987,#39988));
#7495=EDGE_LOOP('',(#39989,#39990,#39991,#39992,#39993,#39994,#39995,#39996,
#39997));
#7496=EDGE_LOOP('',(#39998,#39999,#40000,#40001,#40002,#40003,#40004,#40005,
#40006));
#7497=EDGE_LOOP('',(#40007,#40008,#40009,#40010,#40011,#40012,#40013,#40014));
#7498=EDGE_LOOP('',(#40015,#40016,#40017,#40018));
#7499=EDGE_LOOP('',(#40019,#40020,#40021,#40022));
#7500=EDGE_LOOP('',(#40023,#40024,#40025,#40026));
#7501=EDGE_LOOP('',(#40027,#40028,#40029,#40030));
#7502=EDGE_LOOP('',(#40031,#40032,#40033,#40034));
#7503=EDGE_LOOP('',(#40035,#40036,#40037,#40038));
#7504=EDGE_LOOP('',(#40039,#40040,#40041,#40042));
#7505=EDGE_LOOP('',(#40043,#40044,#40045,#40046));
#7506=EDGE_LOOP('',(#40047,#40048,#40049,#40050));
#7507=EDGE_LOOP('',(#40051,#40052,#40053,#40054));
#7508=EDGE_LOOP('',(#40055,#40056,#40057,#40058));
#7509=EDGE_LOOP('',(#40059,#40060,#40061,#40062));
#7510=EDGE_LOOP('',(#40063,#40064,#40065,#40066));
#7511=EDGE_LOOP('',(#40067,#40068,#40069,#40070));
#7512=EDGE_LOOP('',(#40071,#40072,#40073,#40074));
#7513=EDGE_LOOP('',(#40075,#40076,#40077,#40078));
#7514=EDGE_LOOP('',(#40079,#40080,#40081,#40082));
#7515=EDGE_LOOP('',(#40083,#40084,#40085,#40086));
#7516=EDGE_LOOP('',(#40087,#40088,#40089,#40090));
#7517=EDGE_LOOP('',(#40091,#40092,#40093,#40094));
#7518=EDGE_LOOP('',(#40095,#40096,#40097,#40098,#40099,#40100,#40101,#40102,
#40103,#40104,#40105,#40106));
#7519=EDGE_LOOP('',(#40107,#40108,#40109,#40110,#40111,#40112,#40113,#40114));
#7520=EDGE_LOOP('',(#40115,#40116,#40117,#40118));
#7521=EDGE_LOOP('',(#40119,#40120,#40121,#40122));
#7522=EDGE_LOOP('',(#40123,#40124,#40125,#40126));
#7523=EDGE_LOOP('',(#40127,#40128,#40129,#40130));
#7524=EDGE_LOOP('',(#40131,#40132,#40133,#40134));
#7525=EDGE_LOOP('',(#40135,#40136,#40137,#40138));
#7526=EDGE_LOOP('',(#40139,#40140,#40141,#40142));
#7527=EDGE_LOOP('',(#40143,#40144,#40145,#40146));
#7528=EDGE_LOOP('',(#40147,#40148,#40149,#40150));
#7529=EDGE_LOOP('',(#40151,#40152,#40153,#40154));
#7530=EDGE_LOOP('',(#40155,#40156,#40157,#40158));
#7531=EDGE_LOOP('',(#40159,#40160,#40161,#40162));
#7532=EDGE_LOOP('',(#40163,#40164,#40165,#40166));
#7533=EDGE_LOOP('',(#40167,#40168,#40169,#40170));
#7534=EDGE_LOOP('',(#40171,#40172,#40173,#40174));
#7535=EDGE_LOOP('',(#40175,#40176,#40177,#40178));
#7536=EDGE_LOOP('',(#40179,#40180,#40181,#40182));
#7537=EDGE_LOOP('',(#40183,#40184,#40185,#40186));
#7538=EDGE_LOOP('',(#40187,#40188,#40189,#40190));
#7539=EDGE_LOOP('',(#40191,#40192,#40193,#40194));
#7540=EDGE_LOOP('',(#40195,#40196,#40197,#40198));
#7541=EDGE_LOOP('',(#40199,#40200,#40201,#40202));
#7542=EDGE_LOOP('',(#40203,#40204,#40205,#40206,#40207,#40208,#40209,#40210,
#40211,#40212,#40213,#40214,#40215,#40216,#40217,#40218,#40219,#40220,#40221,
#40222,#40223,#40224));
#7543=EDGE_LOOP('',(#40225,#40226,#40227,#40228,#40229,#40230,#40231,#40232));
#7544=EDGE_LOOP('',(#40233,#40234,#40235,#40236));
#7545=EDGE_LOOP('',(#40237,#40238,#40239,#40240));
#7546=EDGE_LOOP('',(#40241,#40242,#40243,#40244));
#7547=EDGE_LOOP('',(#40245,#40246,#40247,#40248));
#7548=EDGE_LOOP('',(#40249,#40250,#40251,#40252));
#7549=EDGE_LOOP('',(#40253,#40254,#40255,#40256));
#7550=EDGE_LOOP('',(#40257,#40258,#40259,#40260));
#7551=EDGE_LOOP('',(#40261,#40262,#40263,#40264));
#7552=EDGE_LOOP('',(#40265,#40266,#40267,#40268));
#7553=EDGE_LOOP('',(#40269,#40270,#40271,#40272));
#7554=EDGE_LOOP('',(#40273,#40274,#40275,#40276));
#7555=EDGE_LOOP('',(#40277,#40278,#40279,#40280));
#7556=EDGE_LOOP('',(#40281,#40282,#40283,#40284));
#7557=EDGE_LOOP('',(#40285,#40286,#40287,#40288));
#7558=EDGE_LOOP('',(#40289,#40290,#40291,#40292));
#7559=EDGE_LOOP('',(#40293,#40294,#40295,#40296));
#7560=EDGE_LOOP('',(#40297,#40298,#40299,#40300));
#7561=EDGE_LOOP('',(#40301,#40302,#40303,#40304));
#7562=EDGE_LOOP('',(#40305,#40306,#40307,#40308));
#7563=EDGE_LOOP('',(#40309,#40310,#40311,#40312));
#7564=EDGE_LOOP('',(#40313,#40314,#40315,#40316,#40317,#40318,#40319,#40320,
#40321,#40322,#40323,#40324));
#7565=EDGE_LOOP('',(#40325,#40326,#40327,#40328,#40329,#40330,#40331,#40332));
#7566=EDGE_LOOP('',(#40333,#40334,#40335,#40336));
#7567=EDGE_LOOP('',(#40337,#40338,#40339,#40340));
#7568=EDGE_LOOP('',(#40341,#40342,#40343,#40344));
#7569=EDGE_LOOP('',(#40345,#40346,#40347,#40348));
#7570=EDGE_LOOP('',(#40349,#40350,#40351,#40352));
#7571=EDGE_LOOP('',(#40353,#40354,#40355,#40356));
#7572=EDGE_LOOP('',(#40357,#40358,#40359,#40360));
#7573=EDGE_LOOP('',(#40361,#40362,#40363,#40364));
#7574=EDGE_LOOP('',(#40365,#40366,#40367,#40368));
#7575=EDGE_LOOP('',(#40369,#40370,#40371,#40372));
#7576=EDGE_LOOP('',(#40373,#40374,#40375,#40376));
#7577=EDGE_LOOP('',(#40377,#40378,#40379,#40380));
#7578=EDGE_LOOP('',(#40381,#40382,#40383,#40384));
#7579=EDGE_LOOP('',(#40385,#40386,#40387,#40388));
#7580=EDGE_LOOP('',(#40389,#40390,#40391,#40392,#40393,#40394,#40395,#40396,
#40397,#40398,#40399));
#7581=EDGE_LOOP('',(#40400,#40401,#40402));
#7582=EDGE_LOOP('',(#40403,#40404,#40405));
#7583=EDGE_LOOP('',(#40406,#40407,#40408,#40409,#40410,#40411,#40412,#40413));
#7584=EDGE_LOOP('',(#40414,#40415,#40416,#40417));
#7585=EDGE_LOOP('',(#40418,#40419,#40420,#40421));
#7586=EDGE_LOOP('',(#40422,#40423,#40424,#40425));
#7587=EDGE_LOOP('',(#40426,#40427,#40428,#40429));
#7588=EDGE_LOOP('',(#40430,#40431,#40432,#40433));
#7589=EDGE_LOOP('',(#40434,#40435,#40436,#40437));
#7590=EDGE_LOOP('',(#40438,#40439,#40440,#40441));
#7591=EDGE_LOOP('',(#40442,#40443,#40444,#40445));
#7592=EDGE_LOOP('',(#40446,#40447,#40448,#40449));
#7593=EDGE_LOOP('',(#40450,#40451,#40452,#40453));
#7594=EDGE_LOOP('',(#40454,#40455,#40456,#40457));
#7595=EDGE_LOOP('',(#40458,#40459,#40460,#40461));
#7596=EDGE_LOOP('',(#40462,#40463,#40464,#40465));
#7597=EDGE_LOOP('',(#40466,#40467,#40468,#40469));
#7598=EDGE_LOOP('',(#40470,#40471,#40472,#40473));
#7599=EDGE_LOOP('',(#40474,#40475,#40476,#40477));
#7600=EDGE_LOOP('',(#40478,#40479,#40480,#40481));
#7601=EDGE_LOOP('',(#40482,#40483,#40484,#40485));
#7602=EDGE_LOOP('',(#40486,#40487,#40488,#40489));
#7603=EDGE_LOOP('',(#40490,#40491,#40492,#40493));
#7604=EDGE_LOOP('',(#40494,#40495,#40496,#40497,#40498,#40499,#40500,#40501,
#40502,#40503,#40504,#40505));
#7605=EDGE_LOOP('',(#40506,#40507,#40508,#40509,#40510,#40511,#40512,#40513));
#7606=EDGE_LOOP('',(#40514,#40515,#40516,#40517));
#7607=EDGE_LOOP('',(#40518,#40519,#40520,#40521));
#7608=EDGE_LOOP('',(#40522,#40523,#40524,#40525));
#7609=EDGE_LOOP('',(#40526,#40527,#40528,#40529));
#7610=EDGE_LOOP('',(#40530,#40531,#40532,#40533));
#7611=EDGE_LOOP('',(#40534,#40535,#40536,#40537));
#7612=EDGE_LOOP('',(#40538,#40539,#40540,#40541));
#7613=EDGE_LOOP('',(#40542,#40543,#40544,#40545));
#7614=EDGE_LOOP('',(#40546,#40547,#40548,#40549));
#7615=EDGE_LOOP('',(#40550,#40551,#40552,#40553));
#7616=EDGE_LOOP('',(#40554,#40555,#40556,#40557));
#7617=EDGE_LOOP('',(#40558,#40559,#40560,#40561));
#7618=EDGE_LOOP('',(#40562,#40563,#40564,#40565));
#7619=EDGE_LOOP('',(#40566,#40567,#40568,#40569));
#7620=EDGE_LOOP('',(#40570,#40571,#40572,#40573));
#7621=EDGE_LOOP('',(#40574,#40575,#40576,#40577));
#7622=EDGE_LOOP('',(#40578,#40579,#40580,#40581));
#7623=EDGE_LOOP('',(#40582,#40583,#40584,#40585));
#7624=EDGE_LOOP('',(#40586,#40587,#40588,#40589));
#7625=EDGE_LOOP('',(#40590,#40591,#40592,#40593));
#7626=EDGE_LOOP('',(#40594,#40595,#40596,#40597));
#7627=EDGE_LOOP('',(#40598,#40599,#40600,#40601));
#7628=EDGE_LOOP('',(#40602,#40603,#40604,#40605));
#7629=EDGE_LOOP('',(#40606,#40607,#40608,#40609));
#7630=EDGE_LOOP('',(#40610,#40611,#40612,#40613));
#7631=EDGE_LOOP('',(#40614,#40615,#40616,#40617));
#7632=EDGE_LOOP('',(#40618,#40619,#40620,#40621));
#7633=EDGE_LOOP('',(#40622,#40623,#40624,#40625));
#7634=EDGE_LOOP('',(#40626,#40627,#40628,#40629));
#7635=EDGE_LOOP('',(#40630,#40631,#40632,#40633));
#7636=EDGE_LOOP('',(#40634,#40635,#40636,#40637,#40638,#40639,#40640,#40641,
#40642,#40643,#40644,#40645,#40646,#40647,#40648,#40649,#40650,#40651,#40652,
#40653,#40654,#40655,#40656,#40657,#40658,#40659,#40660,#40661,#40662,#40663));
#7637=EDGE_LOOP('',(#40664,#40665,#40666,#40667,#40668,#40669,#40670,#40671));
#7638=EDGE_LOOP('',(#40672,#40673,#40674,#40675));
#7639=EDGE_LOOP('',(#40676,#40677,#40678,#40679));
#7640=EDGE_LOOP('',(#40680,#40681,#40682,#40683));
#7641=EDGE_LOOP('',(#40684,#40685,#40686,#40687));
#7642=EDGE_LOOP('',(#40688,#40689,#40690,#40691));
#7643=EDGE_LOOP('',(#40692,#40693,#40694,#40695));
#7644=EDGE_LOOP('',(#40696,#40697,#40698,#40699));
#7645=EDGE_LOOP('',(#40700,#40701,#40702,#40703));
#7646=EDGE_LOOP('',(#40704,#40705,#40706,#40707));
#7647=EDGE_LOOP('',(#40708,#40709,#40710,#40711));
#7648=EDGE_LOOP('',(#40712,#40713,#40714,#40715));
#7649=EDGE_LOOP('',(#40716,#40717,#40718,#40719));
#7650=EDGE_LOOP('',(#40720,#40721,#40722,#40723));
#7651=EDGE_LOOP('',(#40724,#40725,#40726,#40727));
#7652=EDGE_LOOP('',(#40728,#40729,#40730,#40731));
#7653=EDGE_LOOP('',(#40732,#40733,#40734,#40735));
#7654=EDGE_LOOP('',(#40736,#40737,#40738,#40739));
#7655=EDGE_LOOP('',(#40740,#40741,#40742,#40743));
#7656=EDGE_LOOP('',(#40744,#40745,#40746,#40747));
#7657=EDGE_LOOP('',(#40748,#40749,#40750,#40751));
#7658=EDGE_LOOP('',(#40752,#40753,#40754,#40755,#40756,#40757,#40758,#40759,
#40760,#40761,#40762,#40763));
#7659=EDGE_LOOP('',(#40764,#40765,#40766,#40767,#40768,#40769,#40770,#40771));
#7660=EDGE_LOOP('',(#40772,#40773,#40774,#40775));
#7661=EDGE_LOOP('',(#40776,#40777,#40778,#40779));
#7662=EDGE_LOOP('',(#40780,#40781,#40782,#40783));
#7663=EDGE_LOOP('',(#40784,#40785,#40786,#40787));
#7664=EDGE_LOOP('',(#40788,#40789,#40790,#40791));
#7665=EDGE_LOOP('',(#40792,#40793,#40794,#40795));
#7666=EDGE_LOOP('',(#40796,#40797,#40798,#40799));
#7667=EDGE_LOOP('',(#40800,#40801,#40802,#40803));
#7668=EDGE_LOOP('',(#40804,#40805,#40806,#40807));
#7669=EDGE_LOOP('',(#40808,#40809,#40810,#40811));
#7670=EDGE_LOOP('',(#40812,#40813,#40814,#40815));
#7671=EDGE_LOOP('',(#40816,#40817,#40818,#40819));
#7672=EDGE_LOOP('',(#40820,#40821,#40822,#40823));
#7673=EDGE_LOOP('',(#40824,#40825,#40826,#40827));
#7674=EDGE_LOOP('',(#40828,#40829,#40830,#40831));
#7675=EDGE_LOOP('',(#40832,#40833,#40834,#40835));
#7676=EDGE_LOOP('',(#40836,#40837,#40838,#40839));
#7677=EDGE_LOOP('',(#40840,#40841,#40842,#40843));
#7678=EDGE_LOOP('',(#40844,#40845,#40846,#40847));
#7679=EDGE_LOOP('',(#40848,#40849,#40850,#40851));
#7680=EDGE_LOOP('',(#40852,#40853,#40854,#40855));
#7681=EDGE_LOOP('',(#40856,#40857,#40858,#40859));
#7682=EDGE_LOOP('',(#40860,#40861,#40862,#40863,#40864,#40865,#40866,#40867,
#40868,#40869,#40870,#40871,#40872,#40873,#40874,#40875,#40876,#40877,#40878,
#40879,#40880,#40881));
#7683=EDGE_LOOP('',(#40882,#40883,#40884,#40885,#40886,#40887,#40888,#40889));
#7684=EDGE_LOOP('',(#40890,#40891,#40892,#40893));
#7685=EDGE_LOOP('',(#40894,#40895,#40896,#40897));
#7686=EDGE_LOOP('',(#40898,#40899,#40900,#40901));
#7687=EDGE_LOOP('',(#40902,#40903,#40904,#40905));
#7688=EDGE_LOOP('',(#40906,#40907,#40908,#40909));
#7689=EDGE_LOOP('',(#40910,#40911,#40912,#40913));
#7690=EDGE_LOOP('',(#40914,#40915,#40916,#40917));
#7691=EDGE_LOOP('',(#40918,#40919,#40920,#40921));
#7692=EDGE_LOOP('',(#40922,#40923,#40924,#40925));
#7693=EDGE_LOOP('',(#40926,#40927,#40928,#40929));
#7694=EDGE_LOOP('',(#40930,#40931,#40932,#40933));
#7695=EDGE_LOOP('',(#40934,#40935,#40936,#40937));
#7696=EDGE_LOOP('',(#40938,#40939,#40940,#40941));
#7697=EDGE_LOOP('',(#40942,#40943,#40944,#40945));
#7698=EDGE_LOOP('',(#40946,#40947,#40948,#40949));
#7699=EDGE_LOOP('',(#40950,#40951,#40952,#40953));
#7700=EDGE_LOOP('',(#40954,#40955,#40956,#40957));
#7701=EDGE_LOOP('',(#40958,#40959,#40960,#40961));
#7702=EDGE_LOOP('',(#40962,#40963,#40964,#40965));
#7703=EDGE_LOOP('',(#40966,#40967,#40968,#40969));
#7704=EDGE_LOOP('',(#40970,#40971,#40972,#40973,#40974,#40975,#40976,#40977,
#40978,#40979,#40980,#40981));
#7705=EDGE_LOOP('',(#40982,#40983,#40984,#40985,#40986,#40987,#40988,#40989));
#7706=EDGE_LOOP('',(#40990,#40991,#40992,#40993));
#7707=EDGE_LOOP('',(#40994,#40995,#40996,#40997));
#7708=EDGE_LOOP('',(#40998,#40999,#41000,#41001));
#7709=EDGE_LOOP('',(#41002,#41003,#41004,#41005));
#7710=EDGE_LOOP('',(#41006,#41007,#41008,#41009));
#7711=EDGE_LOOP('',(#41010,#41011,#41012,#41013));
#7712=EDGE_LOOP('',(#41014,#41015,#41016,#41017));
#7713=EDGE_LOOP('',(#41018,#41019,#41020,#41021));
#7714=EDGE_LOOP('',(#41022,#41023,#41024,#41025));
#7715=EDGE_LOOP('',(#41026,#41027,#41028,#41029,#41030,#41031,#41032,#41033,
#41034));
#7716=EDGE_LOOP('',(#41035,#41036,#41037,#41038,#41039,#41040,#41041,#41042));
#7717=EDGE_LOOP('',(#41043,#41044,#41045,#41046));
#7718=EDGE_LOOP('',(#41047,#41048,#41049,#41050));
#7719=EDGE_LOOP('',(#41051,#41052,#41053,#41054));
#7720=EDGE_LOOP('',(#41055,#41056,#41057,#41058));
#7721=EDGE_LOOP('',(#41059,#41060,#41061,#41062));
#7722=EDGE_LOOP('',(#41063,#41064,#41065,#41066));
#7723=EDGE_LOOP('',(#41067,#41068,#41069,#41070));
#7724=EDGE_LOOP('',(#41071,#41072,#41073,#41074));
#7725=EDGE_LOOP('',(#41075,#41076,#41077,#41078));
#7726=EDGE_LOOP('',(#41079,#41080,#41081,#41082));
#7727=EDGE_LOOP('',(#41083,#41084,#41085,#41086));
#7728=EDGE_LOOP('',(#41087,#41088,#41089,#41090));
#7729=EDGE_LOOP('',(#41091,#41092,#41093,#41094));
#7730=EDGE_LOOP('',(#41095,#41096,#41097,#41098));
#7731=EDGE_LOOP('',(#41099,#41100,#41101,#41102));
#7732=EDGE_LOOP('',(#41103,#41104,#41105,#41106));
#7733=EDGE_LOOP('',(#41107,#41108,#41109,#41110));
#7734=EDGE_LOOP('',(#41111,#41112,#41113,#41114));
#7735=EDGE_LOOP('',(#41115,#41116,#41117,#41118));
#7736=EDGE_LOOP('',(#41119,#41120,#41121,#41122));
#7737=EDGE_LOOP('',(#41123,#41124,#41125,#41126,#41127,#41128,#41129,#41130,
#41131,#41132,#41133,#41134));
#7738=EDGE_LOOP('',(#41135,#41136,#41137,#41138,#41139,#41140,#41141,#41142));
#7739=EDGE_LOOP('',(#41143,#41144,#41145,#41146,#41147,#41148,#41149,#41150));
#7740=EDGE_LOOP('',(#41151,#41152,#41153,#41154));
#7741=EDGE_LOOP('',(#41155,#41156,#41157,#41158));
#7742=EDGE_LOOP('',(#41159,#41160,#41161,#41162));
#7743=EDGE_LOOP('',(#41163,#41164,#41165,#41166));
#7744=EDGE_LOOP('',(#41167,#41168,#41169,#41170));
#7745=EDGE_LOOP('',(#41171,#41172,#41173,#41174));
#7746=EDGE_LOOP('',(#41175,#41176,#41177,#41178));
#7747=EDGE_LOOP('',(#41179,#41180,#41181,#41182));
#7748=EDGE_LOOP('',(#41183,#41184,#41185,#41186));
#7749=EDGE_LOOP('',(#41187,#41188,#41189,#41190));
#7750=EDGE_LOOP('',(#41191,#41192,#41193,#41194));
#7751=EDGE_LOOP('',(#41195,#41196,#41197,#41198));
#7752=EDGE_LOOP('',(#41199,#41200,#41201,#41202));
#7753=EDGE_LOOP('',(#41203,#41204,#41205,#41206));
#7754=EDGE_LOOP('',(#41207,#41208,#41209,#41210));
#7755=EDGE_LOOP('',(#41211,#41212,#41213,#41214));
#7756=EDGE_LOOP('',(#41215,#41216,#41217,#41218));
#7757=EDGE_LOOP('',(#41219,#41220,#41221,#41222));
#7758=EDGE_LOOP('',(#41223,#41224,#41225,#41226));
#7759=EDGE_LOOP('',(#41227,#41228,#41229,#41230));
#7760=EDGE_LOOP('',(#41231,#41232,#41233,#41234,#41235,#41236,#41237,#41238,
#41239,#41240,#41241,#41242));
#7761=EDGE_LOOP('',(#41243,#41244,#41245,#41246,#41247,#41248,#41249,#41250));
#7762=EDGE_LOOP('',(#41251,#41252,#41253,#41254));
#7763=EDGE_LOOP('',(#41255,#41256,#41257,#41258));
#7764=EDGE_LOOP('',(#41259,#41260,#41261,#41262));
#7765=EDGE_LOOP('',(#41263,#41264,#41265,#41266));
#7766=EDGE_LOOP('',(#41267,#41268,#41269,#41270));
#7767=EDGE_LOOP('',(#41271,#41272,#41273,#41274));
#7768=EDGE_LOOP('',(#41275,#41276,#41277,#41278));
#7769=EDGE_LOOP('',(#41279,#41280,#41281,#41282));
#7770=EDGE_LOOP('',(#41283,#41284,#41285,#41286));
#7771=EDGE_LOOP('',(#41287,#41288,#41289,#41290,#41291,#41292,#41293,#41294,
#41295));
#7772=EDGE_LOOP('',(#41296,#41297,#41298,#41299,#41300,#41301,#41302,#41303));
#7773=EDGE_LOOP('',(#41304,#41305,#41306,#41307));
#7774=EDGE_LOOP('',(#41308,#41309,#41310,#41311));
#7775=EDGE_LOOP('',(#41312,#41313,#41314,#41315));
#7776=EDGE_LOOP('',(#41316,#41317,#41318,#41319));
#7777=EDGE_LOOP('',(#41320,#41321,#41322,#41323));
#7778=EDGE_LOOP('',(#41324,#41325,#41326,#41327));
#7779=EDGE_LOOP('',(#41328,#41329,#41330,#41331));
#7780=EDGE_LOOP('',(#41332,#41333,#41334,#41335));
#7781=EDGE_LOOP('',(#41336,#41337,#41338,#41339));
#7782=EDGE_LOOP('',(#41340,#41341,#41342,#41343));
#7783=EDGE_LOOP('',(#41344,#41345,#41346,#41347));
#7784=EDGE_LOOP('',(#41348,#41349,#41350,#41351));
#7785=EDGE_LOOP('',(#41352,#41353,#41354,#41355));
#7786=EDGE_LOOP('',(#41356,#41357,#41358,#41359));
#7787=EDGE_LOOP('',(#41360,#41361,#41362,#41363));
#7788=EDGE_LOOP('',(#41364,#41365,#41366,#41367));
#7789=EDGE_LOOP('',(#41368,#41369,#41370,#41371));
#7790=EDGE_LOOP('',(#41372,#41373,#41374,#41375));
#7791=EDGE_LOOP('',(#41376,#41377,#41378,#41379));
#7792=EDGE_LOOP('',(#41380,#41381,#41382,#41383));
#7793=EDGE_LOOP('',(#41384,#41385,#41386,#41387,#41388,#41389,#41390,#41391,
#41392,#41393,#41394,#41395));
#7794=EDGE_LOOP('',(#41396,#41397,#41398,#41399,#41400,#41401,#41402,#41403));
#7795=EDGE_LOOP('',(#41404,#41405,#41406,#41407));
#7796=EDGE_LOOP('',(#41408,#41409,#41410,#41411));
#7797=EDGE_LOOP('',(#41412,#41413,#41414,#41415));
#7798=EDGE_LOOP('',(#41416,#41417,#41418,#41419));
#7799=EDGE_LOOP('',(#41420,#41421,#41422,#41423));
#7800=EDGE_LOOP('',(#41424,#41425,#41426,#41427));
#7801=EDGE_LOOP('',(#41428,#41429,#41430,#41431));
#7802=EDGE_LOOP('',(#41432,#41433,#41434,#41435));
#7803=EDGE_LOOP('',(#41436,#41437,#41438,#41439));
#7804=EDGE_LOOP('',(#41440,#41441,#41442,#41443));
#7805=EDGE_LOOP('',(#41444,#41445,#41446,#41447));
#7806=EDGE_LOOP('',(#41448,#41449,#41450,#41451));
#7807=EDGE_LOOP('',(#41452,#41453,#41454,#41455));
#7808=EDGE_LOOP('',(#41456,#41457,#41458,#41459));
#7809=EDGE_LOOP('',(#41460,#41461,#41462,#41463));
#7810=EDGE_LOOP('',(#41464,#41465,#41466,#41467));
#7811=EDGE_LOOP('',(#41468,#41469,#41470,#41471));
#7812=EDGE_LOOP('',(#41472,#41473,#41474,#41475));
#7813=EDGE_LOOP('',(#41476,#41477,#41478,#41479));
#7814=EDGE_LOOP('',(#41480,#41481,#41482,#41483));
#7815=EDGE_LOOP('',(#41484,#41485,#41486,#41487));
#7816=EDGE_LOOP('',(#41488,#41489,#41490,#41491));
#7817=EDGE_LOOP('',(#41492,#41493,#41494,#41495,#41496,#41497,#41498,#41499,
#41500,#41501,#41502,#41503,#41504,#41505,#41506,#41507,#41508,#41509,#41510,
#41511,#41512,#41513));
#7818=EDGE_LOOP('',(#41514,#41515,#41516,#41517,#41518,#41519,#41520,#41521));
#7819=EDGE_LOOP('',(#41522,#41523,#41524,#41525));
#7820=EDGE_LOOP('',(#41526,#41527,#41528,#41529));
#7821=EDGE_LOOP('',(#41530,#41531,#41532,#41533));
#7822=EDGE_LOOP('',(#41534,#41535,#41536,#41537));
#7823=EDGE_LOOP('',(#41538,#41539,#41540,#41541));
#7824=EDGE_LOOP('',(#41542,#41543,#41544,#41545));
#7825=EDGE_LOOP('',(#41546,#41547,#41548,#41549));
#7826=EDGE_LOOP('',(#41550,#41551,#41552,#41553));
#7827=EDGE_LOOP('',(#41554,#41555,#41556,#41557));
#7828=EDGE_LOOP('',(#41558,#41559,#41560,#41561));
#7829=EDGE_LOOP('',(#41562,#41563,#41564,#41565));
#7830=EDGE_LOOP('',(#41566,#41567,#41568,#41569));
#7831=EDGE_LOOP('',(#41570,#41571,#41572,#41573));
#7832=EDGE_LOOP('',(#41574,#41575,#41576,#41577));
#7833=EDGE_LOOP('',(#41578,#41579,#41580,#41581));
#7834=EDGE_LOOP('',(#41582,#41583,#41584,#41585));
#7835=EDGE_LOOP('',(#41586,#41587,#41588,#41589));
#7836=EDGE_LOOP('',(#41590,#41591,#41592,#41593));
#7837=EDGE_LOOP('',(#41594,#41595,#41596,#41597));
#7838=EDGE_LOOP('',(#41598,#41599,#41600,#41601));
#7839=EDGE_LOOP('',(#41602,#41603,#41604,#41605,#41606,#41607,#41608,#41609,
#41610,#41611,#41612,#41613));
#7840=EDGE_LOOP('',(#41614,#41615,#41616,#41617,#41618,#41619,#41620,#41621));
#7841=EDGE_LOOP('',(#41622,#41623,#41624,#41625));
#7842=EDGE_LOOP('',(#41626,#41627,#41628,#41629));
#7843=EDGE_LOOP('',(#41630,#41631,#41632,#41633));
#7844=EDGE_LOOP('',(#41634,#41635,#41636,#41637));
#7845=EDGE_LOOP('',(#41638,#41639,#41640,#41641));
#7846=EDGE_LOOP('',(#41642,#41643,#41644,#41645));
#7847=EDGE_LOOP('',(#41646,#41647,#41648,#41649));
#7848=EDGE_LOOP('',(#41650,#41651,#41652,#41653));
#7849=EDGE_LOOP('',(#41654,#41655,#41656,#41657));
#7850=EDGE_LOOP('',(#41658,#41659,#41660,#41661));
#7851=EDGE_LOOP('',(#41662,#41663,#41664,#41665));
#7852=EDGE_LOOP('',(#41666,#41667,#41668,#41669));
#7853=EDGE_LOOP('',(#41670,#41671,#41672,#41673));
#7854=EDGE_LOOP('',(#41674,#41675,#41676,#41677));
#7855=EDGE_LOOP('',(#41678,#41679,#41680,#41681));
#7856=EDGE_LOOP('',(#41682,#41683,#41684,#41685));
#7857=EDGE_LOOP('',(#41686,#41687,#41688,#41689));
#7858=EDGE_LOOP('',(#41690,#41691,#41692,#41693));
#7859=EDGE_LOOP('',(#41694,#41695,#41696,#41697));
#7860=EDGE_LOOP('',(#41698,#41699,#41700,#41701));
#7861=EDGE_LOOP('',(#41702,#41703,#41704,#41705));
#7862=EDGE_LOOP('',(#41706,#41707,#41708,#41709));
#7863=EDGE_LOOP('',(#41710,#41711,#41712,#41713));
#7864=EDGE_LOOP('',(#41714,#41715,#41716,#41717));
#7865=EDGE_LOOP('',(#41718,#41719,#41720,#41721));
#7866=EDGE_LOOP('',(#41722,#41723,#41724,#41725));
#7867=EDGE_LOOP('',(#41726,#41727,#41728,#41729));
#7868=EDGE_LOOP('',(#41730,#41731,#41732,#41733));
#7869=EDGE_LOOP('',(#41734,#41735,#41736,#41737));
#7870=EDGE_LOOP('',(#41738,#41739,#41740,#41741));
#7871=EDGE_LOOP('',(#41742,#41743,#41744,#41745,#41746,#41747,#41748,#41749,
#41750,#41751,#41752,#41753,#41754,#41755,#41756,#41757,#41758,#41759,#41760,
#41761,#41762,#41763,#41764,#41765,#41766,#41767,#41768,#41769,#41770,#41771));
#7872=EDGE_LOOP('',(#41772,#41773,#41774,#41775,#41776,#41777,#41778,#41779));
#7873=EDGE_LOOP('',(#41780,#41781,#41782,#41783));
#7874=EDGE_LOOP('',(#41784,#41785,#41786,#41787));
#7875=EDGE_LOOP('',(#41788,#41789,#41790,#41791));
#7876=EDGE_LOOP('',(#41792,#41793,#41794,#41795));
#7877=EDGE_LOOP('',(#41796,#41797,#41798,#41799));
#7878=EDGE_LOOP('',(#41800,#41801,#41802,#41803));
#7879=EDGE_LOOP('',(#41804,#41805,#41806,#41807));
#7880=EDGE_LOOP('',(#41808,#41809,#41810,#41811));
#7881=EDGE_LOOP('',(#41812,#41813,#41814,#41815));
#7882=EDGE_LOOP('',(#41816,#41817,#41818,#41819));
#7883=EDGE_LOOP('',(#41820,#41821,#41822,#41823));
#7884=EDGE_LOOP('',(#41824,#41825,#41826,#41827));
#7885=EDGE_LOOP('',(#41828,#41829,#41830,#41831));
#7886=EDGE_LOOP('',(#41832,#41833,#41834,#41835));
#7887=EDGE_LOOP('',(#41836,#41837,#41838,#41839));
#7888=EDGE_LOOP('',(#41840,#41841,#41842,#41843));
#7889=EDGE_LOOP('',(#41844,#41845,#41846,#41847));
#7890=EDGE_LOOP('',(#41848,#41849,#41850,#41851));
#7891=EDGE_LOOP('',(#41852,#41853,#41854,#41855));
#7892=EDGE_LOOP('',(#41856,#41857,#41858,#41859));
#7893=EDGE_LOOP('',(#41860,#41861,#41862,#41863,#41864,#41865,#41866,#41867,
#41868,#41869,#41870,#41871));
#7894=EDGE_LOOP('',(#41872,#41873,#41874,#41875,#41876,#41877,#41878,#41879));
#7895=EDGE_LOOP('',(#41880,#41881,#41882,#41883));
#7896=EDGE_LOOP('',(#41884,#41885,#41886,#41887));
#7897=EDGE_LOOP('',(#41888,#41889,#41890,#41891));
#7898=EDGE_LOOP('',(#41892,#41893,#41894,#41895));
#7899=EDGE_LOOP('',(#41896,#41897,#41898,#41899));
#7900=EDGE_LOOP('',(#41900,#41901,#41902,#41903));
#7901=EDGE_LOOP('',(#41904,#41905,#41906,#41907));
#7902=EDGE_LOOP('',(#41908,#41909,#41910,#41911));
#7903=EDGE_LOOP('',(#41912,#41913,#41914,#41915));
#7904=EDGE_LOOP('',(#41916,#41917,#41918,#41919));
#7905=EDGE_LOOP('',(#41920,#41921,#41922,#41923));
#7906=EDGE_LOOP('',(#41924,#41925,#41926,#41927));
#7907=EDGE_LOOP('',(#41928,#41929,#41930,#41931));
#7908=EDGE_LOOP('',(#41932,#41933,#41934,#41935));
#7909=EDGE_LOOP('',(#41936,#41937,#41938,#41939,#41940,#41941,#41942,#41943,
#41944,#41945,#41946));
#7910=EDGE_LOOP('',(#41947,#41948,#41949));
#7911=EDGE_LOOP('',(#41950,#41951,#41952));
#7912=EDGE_LOOP('',(#41953,#41954,#41955,#41956,#41957,#41958,#41959,#41960));
#7913=EDGE_LOOP('',(#41961,#41962,#41963,#41964));
#7914=EDGE_LOOP('',(#41965,#41966,#41967,#41968));
#7915=EDGE_LOOP('',(#41969,#41970,#41971,#41972));
#7916=EDGE_LOOP('',(#41973,#41974,#41975,#41976));
#7917=EDGE_LOOP('',(#41977,#41978,#41979,#41980));
#7918=EDGE_LOOP('',(#41981,#41982,#41983,#41984));
#7919=EDGE_LOOP('',(#41985,#41986,#41987,#41988));
#7920=EDGE_LOOP('',(#41989,#41990,#41991,#41992));
#7921=EDGE_LOOP('',(#41993,#41994,#41995,#41996));
#7922=EDGE_LOOP('',(#41997,#41998,#41999,#42000));
#7923=EDGE_LOOP('',(#42001,#42002,#42003,#42004));
#7924=EDGE_LOOP('',(#42005,#42006,#42007,#42008));
#7925=EDGE_LOOP('',(#42009,#42010,#42011,#42012));
#7926=EDGE_LOOP('',(#42013,#42014,#42015,#42016));
#7927=EDGE_LOOP('',(#42017,#42018,#42019,#42020));
#7928=EDGE_LOOP('',(#42021,#42022,#42023,#42024));
#7929=EDGE_LOOP('',(#42025,#42026,#42027,#42028));
#7930=EDGE_LOOP('',(#42029,#42030,#42031,#42032));
#7931=EDGE_LOOP('',(#42033,#42034,#42035,#42036));
#7932=EDGE_LOOP('',(#42037,#42038,#42039,#42040));
#7933=EDGE_LOOP('',(#42041,#42042,#42043,#42044,#42045,#42046,#42047,#42048,
#42049,#42050,#42051,#42052));
#7934=EDGE_LOOP('',(#42053,#42054,#42055,#42056,#42057,#42058,#42059,#42060));
#7935=EDGE_LOOP('',(#42061,#42062,#42063,#42064));
#7936=EDGE_LOOP('',(#42065,#42066,#42067,#42068));
#7937=EDGE_LOOP('',(#42069,#42070,#42071,#42072));
#7938=EDGE_LOOP('',(#42073,#42074,#42075,#42076));
#7939=EDGE_LOOP('',(#42077,#42078,#42079,#42080));
#7940=EDGE_LOOP('',(#42081,#42082,#42083,#42084));
#7941=EDGE_LOOP('',(#42085,#42086,#42087,#42088));
#7942=EDGE_LOOP('',(#42089,#42090,#42091,#42092));
#7943=EDGE_LOOP('',(#42093,#42094,#42095,#42096));
#7944=EDGE_LOOP('',(#42097,#42098,#42099,#42100));
#7945=EDGE_LOOP('',(#42101,#42102,#42103,#42104));
#7946=EDGE_LOOP('',(#42105,#42106,#42107,#42108));
#7947=EDGE_LOOP('',(#42109,#42110,#42111,#42112));
#7948=EDGE_LOOP('',(#42113,#42114,#42115,#42116));
#7949=EDGE_LOOP('',(#42117,#42118,#42119,#42120));
#7950=EDGE_LOOP('',(#42121,#42122,#42123,#42124));
#7951=EDGE_LOOP('',(#42125,#42126,#42127,#42128));
#7952=EDGE_LOOP('',(#42129,#42130,#42131,#42132));
#7953=EDGE_LOOP('',(#42133,#42134,#42135,#42136));
#7954=EDGE_LOOP('',(#42137,#42138,#42139,#42140));
#7955=EDGE_LOOP('',(#42141,#42142,#42143,#42144));
#7956=EDGE_LOOP('',(#42145,#42146,#42147,#42148));
#7957=EDGE_LOOP('',(#42149,#42150,#42151,#42152,#42153,#42154,#42155,#42156,
#42157,#42158,#42159,#42160,#42161,#42162,#42163,#42164,#42165,#42166,#42167,
#42168,#42169,#42170));
#7958=EDGE_LOOP('',(#42171,#42172,#42173,#42174,#42175,#42176,#42177,#42178));
#7959=EDGE_LOOP('',(#42179,#42180,#42181,#42182));
#7960=EDGE_LOOP('',(#42183,#42184,#42185,#42186));
#7961=EDGE_LOOP('',(#42187,#42188,#42189,#42190));
#7962=EDGE_LOOP('',(#42191,#42192,#42193,#42194));
#7963=EDGE_LOOP('',(#42195,#42196,#42197,#42198));
#7964=EDGE_LOOP('',(#42199,#42200,#42201,#42202));
#7965=EDGE_LOOP('',(#42203,#42204,#42205,#42206));
#7966=EDGE_LOOP('',(#42207,#42208,#42209,#42210));
#7967=EDGE_LOOP('',(#42211,#42212,#42213,#42214));
#7968=EDGE_LOOP('',(#42215,#42216,#42217,#42218));
#7969=EDGE_LOOP('',(#42219,#42220,#42221,#42222));
#7970=EDGE_LOOP('',(#42223,#42224,#42225,#42226));
#7971=EDGE_LOOP('',(#42227,#42228,#42229,#42230));
#7972=EDGE_LOOP('',(#42231,#42232,#42233,#42234));
#7973=EDGE_LOOP('',(#42235,#42236,#42237,#42238));
#7974=EDGE_LOOP('',(#42239,#42240,#42241,#42242));
#7975=EDGE_LOOP('',(#42243,#42244,#42245,#42246));
#7976=EDGE_LOOP('',(#42247,#42248,#42249,#42250));
#7977=EDGE_LOOP('',(#42251,#42252,#42253,#42254));
#7978=EDGE_LOOP('',(#42255,#42256,#42257,#42258));
#7979=EDGE_LOOP('',(#42259,#42260,#42261,#42262,#42263,#42264,#42265,#42266,
#42267,#42268,#42269,#42270));
#7980=EDGE_LOOP('',(#42271,#42272,#42273,#42274,#42275,#42276,#42277,#42278));
#7981=EDGE_LOOP('',(#42279,#42280,#42281,#42282));
#7982=EDGE_LOOP('',(#42283,#42284,#42285,#42286));
#7983=EDGE_LOOP('',(#42287,#42288,#42289,#42290));
#7984=EDGE_LOOP('',(#42291,#42292,#42293,#42294));
#7985=EDGE_LOOP('',(#42295,#42296,#42297,#42298));
#7986=EDGE_LOOP('',(#42299,#42300,#42301,#42302));
#7987=EDGE_LOOP('',(#42303,#42304,#42305,#42306));
#7988=EDGE_LOOP('',(#42307,#42308,#42309,#42310));
#7989=EDGE_LOOP('',(#42311,#42312,#42313,#42314));
#7990=EDGE_LOOP('',(#42315,#42316,#42317,#42318));
#7991=EDGE_LOOP('',(#42319,#42320,#42321,#42322));
#7992=EDGE_LOOP('',(#42323,#42324,#42325,#42326));
#7993=EDGE_LOOP('',(#42327,#42328,#42329,#42330));
#7994=EDGE_LOOP('',(#42331,#42332,#42333,#42334));
#7995=EDGE_LOOP('',(#42335,#42336,#42337,#42338));
#7996=EDGE_LOOP('',(#42339,#42340,#42341,#42342));
#7997=EDGE_LOOP('',(#42343,#42344,#42345,#42346));
#7998=EDGE_LOOP('',(#42347,#42348,#42349,#42350));
#7999=EDGE_LOOP('',(#42351,#42352,#42353,#42354));
#8000=EDGE_LOOP('',(#42355,#42356,#42357,#42358));
#8001=EDGE_LOOP('',(#42359,#42360,#42361,#42362));
#8002=EDGE_LOOP('',(#42363,#42364,#42365,#42366));
#8003=EDGE_LOOP('',(#42367,#42368,#42369,#42370));
#8004=EDGE_LOOP('',(#42371,#42372,#42373,#42374));
#8005=EDGE_LOOP('',(#42375,#42376,#42377,#42378));
#8006=EDGE_LOOP('',(#42379,#42380,#42381,#42382));
#8007=EDGE_LOOP('',(#42383,#42384,#42385,#42386));
#8008=EDGE_LOOP('',(#42387,#42388,#42389,#42390));
#8009=EDGE_LOOP('',(#42391,#42392,#42393,#42394,#42395,#42396,#42397,#42398,
#42399,#42400,#42401,#42402,#42403,#42404,#42405,#42406,#42407,#42408,#42409));
#8010=EDGE_LOOP('',(#42410,#42411,#42412,#42413,#42414,#42415,#42416,#42417,
#42418));
#8011=EDGE_LOOP('',(#42419,#42420,#42421,#42422,#42423,#42424,#42425,#42426,
#42427));
#8012=EDGE_LOOP('',(#42428,#42429,#42430,#42431,#42432,#42433,#42434,#42435));
#8013=EDGE_LOOP('',(#42436,#42437,#42438,#42439));
#8014=EDGE_LOOP('',(#42440,#42441,#42442,#42443));
#8015=EDGE_LOOP('',(#42444,#42445,#42446,#42447));
#8016=EDGE_LOOP('',(#42448,#42449,#42450,#42451));
#8017=EDGE_LOOP('',(#42452,#42453,#42454,#42455));
#8018=EDGE_LOOP('',(#42456,#42457,#42458,#42459));
#8019=EDGE_LOOP('',(#42460,#42461,#42462,#42463));
#8020=EDGE_LOOP('',(#42464,#42465,#42466,#42467));
#8021=EDGE_LOOP('',(#42468,#42469,#42470,#42471));
#8022=EDGE_LOOP('',(#42472,#42473,#42474,#42475));
#8023=EDGE_LOOP('',(#42476,#42477,#42478,#42479));
#8024=EDGE_LOOP('',(#42480,#42481,#42482,#42483));
#8025=EDGE_LOOP('',(#42484,#42485,#42486,#42487));
#8026=EDGE_LOOP('',(#42488,#42489,#42490,#42491));
#8027=EDGE_LOOP('',(#42492,#42493,#42494,#42495));
#8028=EDGE_LOOP('',(#42496,#42497,#42498,#42499));
#8029=EDGE_LOOP('',(#42500,#42501,#42502,#42503));
#8030=EDGE_LOOP('',(#42504,#42505,#42506,#42507));
#8031=EDGE_LOOP('',(#42508,#42509,#42510,#42511));
#8032=EDGE_LOOP('',(#42512,#42513,#42514,#42515));
#8033=EDGE_LOOP('',(#42516,#42517,#42518,#42519,#42520,#42521,#42522,#42523,
#42524,#42525,#42526,#42527));
#8034=EDGE_LOOP('',(#42528,#42529,#42530,#42531,#42532,#42533,#42534,#42535));
#8035=EDGE_LOOP('',(#42536,#42537,#42538,#42539));
#8036=EDGE_LOOP('',(#42540,#42541,#42542,#42543));
#8037=EDGE_LOOP('',(#42544,#42545,#42546,#42547));
#8038=EDGE_LOOP('',(#42548,#42549,#42550,#42551));
#8039=EDGE_LOOP('',(#42552,#42553,#42554,#42555));
#8040=EDGE_LOOP('',(#42556,#42557,#42558,#42559));
#8041=EDGE_LOOP('',(#42560,#42561,#42562,#42563));
#8042=EDGE_LOOP('',(#42564,#42565,#42566,#42567));
#8043=EDGE_LOOP('',(#42568,#42569,#42570,#42571));
#8044=EDGE_LOOP('',(#42572,#42573,#42574,#42575));
#8045=EDGE_LOOP('',(#42576,#42577,#42578,#42579));
#8046=EDGE_LOOP('',(#42580,#42581,#42582,#42583,#42584,#42585,#42586,#42587,
#42588,#42589,#42590));
#8047=EDGE_LOOP('',(#42591,#42592,#42593,#42594,#42595,#42596,#42597,#42598));
#8048=EDGE_LOOP('',(#42599,#42600,#42601,#42602));
#8049=EDGE_LOOP('',(#42603,#42604,#42605,#42606));
#8050=EDGE_LOOP('',(#42607,#42608,#42609,#42610));
#8051=EDGE_LOOP('',(#42611,#42612,#42613,#42614));
#8052=EDGE_LOOP('',(#42615,#42616,#42617,#42618));
#8053=EDGE_LOOP('',(#42619,#42620,#42621,#42622));
#8054=EDGE_LOOP('',(#42623,#42624,#42625,#42626));
#8055=EDGE_LOOP('',(#42627,#42628,#42629,#42630));
#8056=EDGE_LOOP('',(#42631,#42632,#42633,#42634));
#8057=EDGE_LOOP('',(#42635,#42636,#42637,#42638));
#8058=EDGE_LOOP('',(#42639,#42640,#42641,#42642));
#8059=EDGE_LOOP('',(#42643,#42644,#42645,#42646));
#8060=EDGE_LOOP('',(#42647,#42648,#42649,#42650));
#8061=EDGE_LOOP('',(#42651,#42652,#42653,#42654));
#8062=EDGE_LOOP('',(#42655,#42656,#42657,#42658));
#8063=EDGE_LOOP('',(#42659,#42660,#42661,#42662));
#8064=EDGE_LOOP('',(#42663,#42664,#42665,#42666));
#8065=EDGE_LOOP('',(#42667,#42668,#42669,#42670));
#8066=EDGE_LOOP('',(#42671,#42672,#42673,#42674));
#8067=EDGE_LOOP('',(#42675,#42676,#42677,#42678));
#8068=EDGE_LOOP('',(#42679,#42680,#42681,#42682,#42683,#42684,#42685,#42686,
#42687,#42688,#42689,#42690));
#8069=EDGE_LOOP('',(#42691,#42692,#42693,#42694,#42695,#42696,#42697,#42698));
#8070=EDGE_LOOP('',(#42699,#42700,#42701,#42702));
#8071=EDGE_LOOP('',(#42703,#42704,#42705,#42706));
#8072=EDGE_LOOP('',(#42707,#42708,#42709,#42710));
#8073=EDGE_LOOP('',(#42711,#42712,#42713,#42714));
#8074=EDGE_LOOP('',(#42715,#42716,#42717,#42718));
#8075=EDGE_LOOP('',(#42719,#42720,#42721,#42722));
#8076=EDGE_LOOP('',(#42723,#42724,#42725,#42726));
#8077=EDGE_LOOP('',(#42727,#42728,#42729,#42730));
#8078=EDGE_LOOP('',(#42731,#42732,#42733,#42734));
#8079=EDGE_LOOP('',(#42735,#42736,#42737,#42738));
#8080=EDGE_LOOP('',(#42739,#42740,#42741,#42742));
#8081=EDGE_LOOP('',(#42743,#42744,#42745,#42746));
#8082=EDGE_LOOP('',(#42747,#42748,#42749,#42750));
#8083=EDGE_LOOP('',(#42751,#42752,#42753,#42754));
#8084=EDGE_LOOP('',(#42755,#42756,#42757,#42758));
#8085=EDGE_LOOP('',(#42759,#42760,#42761,#42762));
#8086=EDGE_LOOP('',(#42763,#42764,#42765,#42766));
#8087=EDGE_LOOP('',(#42767,#42768,#42769,#42770));
#8088=EDGE_LOOP('',(#42771,#42772,#42773,#42774));
#8089=EDGE_LOOP('',(#42775,#42776,#42777,#42778));
#8090=EDGE_LOOP('',(#42779,#42780,#42781,#42782));
#8091=EDGE_LOOP('',(#42783,#42784,#42785,#42786));
#8092=EDGE_LOOP('',(#42787,#42788,#42789,#42790));
#8093=EDGE_LOOP('',(#42791,#42792,#42793,#42794));
#8094=EDGE_LOOP('',(#42795,#42796,#42797,#42798));
#8095=EDGE_LOOP('',(#42799,#42800,#42801,#42802));
#8096=EDGE_LOOP('',(#42803,#42804,#42805,#42806));
#8097=EDGE_LOOP('',(#42807,#42808,#42809,#42810));
#8098=EDGE_LOOP('',(#42811,#42812,#42813,#42814));
#8099=EDGE_LOOP('',(#42815,#42816,#42817,#42818));
#8100=EDGE_LOOP('',(#42819,#42820,#42821,#42822));
#8101=EDGE_LOOP('',(#42823,#42824,#42825,#42826));
#8102=EDGE_LOOP('',(#42827,#42828,#42829,#42830));
#8103=EDGE_LOOP('',(#42831,#42832,#42833,#42834,#42835,#42836,#42837,#42838,
#42839,#42840,#42841,#42842,#42843,#42844,#42845,#42846));
#8104=EDGE_LOOP('',(#42847,#42848,#42849,#42850,#42851,#42852,#42853,#42854,
#42855));
#8105=EDGE_LOOP('',(#42856,#42857,#42858,#42859,#42860,#42861,#42862,#42863));
#8106=EDGE_LOOP('',(#42864,#42865,#42866,#42867,#42868,#42869,#42870,#42871,
#42872));
#8107=EDGE_LOOP('',(#42873,#42874,#42875,#42876,#42877,#42878,#42879,#42880));
#8108=EDGE_LOOP('',(#42881,#42882,#42883,#42884,#42885,#42886,#42887,#42888));
#8109=EDGE_LOOP('',(#42889,#42890,#42891,#42892));
#8110=EDGE_LOOP('',(#42893,#42894,#42895,#42896));
#8111=EDGE_LOOP('',(#42897,#42898,#42899,#42900));
#8112=EDGE_LOOP('',(#42901,#42902,#42903,#42904));
#8113=EDGE_LOOP('',(#42905,#42906,#42907,#42908));
#8114=EDGE_LOOP('',(#42909,#42910,#42911,#42912));
#8115=EDGE_LOOP('',(#42913,#42914,#42915,#42916));
#8116=EDGE_LOOP('',(#42917,#42918,#42919,#42920));
#8117=EDGE_LOOP('',(#42921,#42922,#42923,#42924));
#8118=EDGE_LOOP('',(#42925,#42926,#42927,#42928));
#8119=EDGE_LOOP('',(#42929,#42930,#42931,#42932));
#8120=EDGE_LOOP('',(#42933,#42934,#42935,#42936));
#8121=EDGE_LOOP('',(#42937,#42938,#42939,#42940));
#8122=EDGE_LOOP('',(#42941,#42942,#42943,#42944));
#8123=EDGE_LOOP('',(#42945,#42946,#42947,#42948));
#8124=EDGE_LOOP('',(#42949,#42950,#42951,#42952));
#8125=EDGE_LOOP('',(#42953,#42954,#42955,#42956));
#8126=EDGE_LOOP('',(#42957,#42958,#42959,#42960));
#8127=EDGE_LOOP('',(#42961,#42962,#42963,#42964));
#8128=EDGE_LOOP('',(#42965,#42966,#42967,#42968));
#8129=EDGE_LOOP('',(#42969,#42970,#42971,#42972,#42973,#42974,#42975,#42976,
#42977,#42978,#42979,#42980));
#8130=EDGE_LOOP('',(#42981,#42982,#42983,#42984,#42985,#42986,#42987,#42988));
#8131=EDGE_LOOP('',(#42989,#42990,#42991,#42992));
#8132=EDGE_LOOP('',(#42993,#42994,#42995,#42996));
#8133=EDGE_LOOP('',(#42997,#42998,#42999,#43000));
#8134=EDGE_LOOP('',(#43001,#43002,#43003,#43004));
#8135=EDGE_LOOP('',(#43005,#43006,#43007,#43008));
#8136=EDGE_LOOP('',(#43009,#43010,#43011,#43012));
#8137=EDGE_LOOP('',(#43013,#43014,#43015,#43016));
#8138=EDGE_LOOP('',(#43017,#43018,#43019,#43020));
#8139=EDGE_LOOP('',(#43021,#43022,#43023,#43024));
#8140=EDGE_LOOP('',(#43025,#43026,#43027,#43028));
#8141=EDGE_LOOP('',(#43029,#43030,#43031,#43032));
#8142=EDGE_LOOP('',(#43033,#43034,#43035,#43036));
#8143=EDGE_LOOP('',(#43037,#43038,#43039,#43040));
#8144=EDGE_LOOP('',(#43041,#43042,#43043,#43044));
#8145=EDGE_LOOP('',(#43045,#43046,#43047,#43048));
#8146=EDGE_LOOP('',(#43049,#43050,#43051,#43052));
#8147=EDGE_LOOP('',(#43053,#43054,#43055,#43056));
#8148=EDGE_LOOP('',(#43057,#43058,#43059,#43060));
#8149=EDGE_LOOP('',(#43061,#43062,#43063,#43064));
#8150=EDGE_LOOP('',(#43065,#43066,#43067,#43068));
#8151=EDGE_LOOP('',(#43069,#43070,#43071,#43072));
#8152=EDGE_LOOP('',(#43073,#43074,#43075,#43076));
#8153=EDGE_LOOP('',(#43077,#43078,#43079,#43080));
#8154=EDGE_LOOP('',(#43081,#43082,#43083,#43084));
#8155=EDGE_LOOP('',(#43085,#43086,#43087,#43088));
#8156=EDGE_LOOP('',(#43089,#43090,#43091,#43092));
#8157=EDGE_LOOP('',(#43093,#43094,#43095,#43096));
#8158=EDGE_LOOP('',(#43097,#43098,#43099,#43100));
#8159=EDGE_LOOP('',(#43101,#43102,#43103,#43104));
#8160=EDGE_LOOP('',(#43105,#43106,#43107,#43108));
#8161=EDGE_LOOP('',(#43109,#43110,#43111,#43112,#43113,#43114,#43115,#43116,
#43117,#43118,#43119,#43120,#43121,#43122,#43123,#43124,#43125,#43126,#43127,
#43128,#43129,#43130));
#8162=EDGE_LOOP('',(#43131,#43132,#43133,#43134,#43135,#43136,#43137,#43138));
#8163=EDGE_LOOP('',(#43139,#43140,#43141,#43142,#43143,#43144,#43145,#43146));
#8164=EDGE_LOOP('',(#43147,#43148,#43149,#43150,#43151,#43152,#43153,#43154));
#8165=EDGE_LOOP('',(#43155,#43156,#43157,#43158));
#8166=EDGE_LOOP('',(#43159,#43160,#43161,#43162));
#8167=EDGE_LOOP('',(#43163,#43164,#43165,#43166));
#8168=EDGE_LOOP('',(#43167,#43168,#43169,#43170));
#8169=EDGE_LOOP('',(#43171,#43172,#43173,#43174));
#8170=EDGE_LOOP('',(#43175,#43176,#43177,#43178));
#8171=EDGE_LOOP('',(#43179,#43180,#43181,#43182));
#8172=EDGE_LOOP('',(#43183,#43184,#43185,#43186));
#8173=EDGE_LOOP('',(#43187,#43188,#43189,#43190));
#8174=EDGE_LOOP('',(#43191,#43192,#43193,#43194));
#8175=EDGE_LOOP('',(#43195,#43196,#43197,#43198));
#8176=EDGE_LOOP('',(#43199,#43200,#43201,#43202));
#8177=EDGE_LOOP('',(#43203,#43204,#43205,#43206));
#8178=EDGE_LOOP('',(#43207,#43208,#43209,#43210));
#8179=EDGE_LOOP('',(#43211,#43212,#43213,#43214));
#8180=EDGE_LOOP('',(#43215,#43216,#43217,#43218));
#8181=EDGE_LOOP('',(#43219,#43220,#43221,#43222));
#8182=EDGE_LOOP('',(#43223,#43224,#43225,#43226));
#8183=EDGE_LOOP('',(#43227,#43228,#43229,#43230));
#8184=EDGE_LOOP('',(#43231,#43232,#43233,#43234));
#8185=EDGE_LOOP('',(#43235,#43236,#43237,#43238));
#8186=EDGE_LOOP('',(#43239,#43240,#43241,#43242));
#8187=EDGE_LOOP('',(#43243,#43244,#43245,#43246));
#8188=EDGE_LOOP('',(#43247,#43248,#43249,#43250));
#8189=EDGE_LOOP('',(#43251,#43252,#43253,#43254));
#8190=EDGE_LOOP('',(#43255,#43256,#43257,#43258));
#8191=EDGE_LOOP('',(#43259,#43260,#43261,#43262));
#8192=EDGE_LOOP('',(#43263,#43264,#43265,#43266));
#8193=EDGE_LOOP('',(#43267,#43268,#43269,#43270));
#8194=EDGE_LOOP('',(#43271,#43272,#43273,#43274));
#8195=EDGE_LOOP('',(#43275,#43276,#43277,#43278));
#8196=EDGE_LOOP('',(#43279,#43280,#43281,#43282));
#8197=EDGE_LOOP('',(#43283,#43284,#43285,#43286));
#8198=EDGE_LOOP('',(#43287,#43288,#43289,#43290));
#8199=EDGE_LOOP('',(#43291,#43292,#43293,#43294));
#8200=EDGE_LOOP('',(#43295,#43296,#43297,#43298));
#8201=EDGE_LOOP('',(#43299,#43300,#43301,#43302));
#8202=EDGE_LOOP('',(#43303,#43304,#43305,#43306));
#8203=EDGE_LOOP('',(#43307,#43308,#43309,#43310));
#8204=EDGE_LOOP('',(#43311,#43312,#43313,#43314));
#8205=EDGE_LOOP('',(#43315,#43316,#43317,#43318));
#8206=EDGE_LOOP('',(#43319,#43320,#43321,#43322));
#8207=EDGE_LOOP('',(#43323,#43324,#43325,#43326));
#8208=EDGE_LOOP('',(#43327,#43328,#43329,#43330));
#8209=EDGE_LOOP('',(#43331,#43332,#43333,#43334));
#8210=EDGE_LOOP('',(#43335,#43336,#43337,#43338));
#8211=EDGE_LOOP('',(#43339,#43340,#43341,#43342));
#8212=EDGE_LOOP('',(#43343,#43344,#43345,#43346));
#8213=EDGE_LOOP('',(#43347,#43348,#43349,#43350));
#8214=EDGE_LOOP('',(#43351,#43352,#43353,#43354));
#8215=EDGE_LOOP('',(#43355,#43356,#43357,#43358));
#8216=EDGE_LOOP('',(#43359,#43360,#43361,#43362));
#8217=EDGE_LOOP('',(#43363,#43364,#43365,#43366));
#8218=EDGE_LOOP('',(#43367,#43368,#43369,#43370));
#8219=EDGE_LOOP('',(#43371,#43372,#43373,#43374));
#8220=EDGE_LOOP('',(#43375,#43376,#43377,#43378));
#8221=EDGE_LOOP('',(#43379,#43380,#43381,#43382));
#8222=EDGE_LOOP('',(#43383,#43384,#43385,#43386));
#8223=EDGE_LOOP('',(#43387,#43388,#43389,#43390));
#8224=EDGE_LOOP('',(#43391,#43392,#43393,#43394));
#8225=EDGE_LOOP('',(#43395,#43396,#43397,#43398));
#8226=EDGE_LOOP('',(#43399,#43400,#43401,#43402));
#8227=EDGE_LOOP('',(#43403,#43404,#43405,#43406));
#8228=EDGE_LOOP('',(#43407,#43408,#43409,#43410));
#8229=EDGE_LOOP('',(#43411,#43412,#43413,#43414));
#8230=EDGE_LOOP('',(#43415,#43416,#43417,#43418));
#8231=EDGE_LOOP('',(#43419,#43420,#43421,#43422));
#8232=EDGE_LOOP('',(#43423,#43424,#43425,#43426));
#8233=EDGE_LOOP('',(#43427,#43428,#43429,#43430));
#8234=EDGE_LOOP('',(#43431,#43432,#43433,#43434));
#8235=EDGE_LOOP('',(#43435,#43436,#43437,#43438));
#8236=EDGE_LOOP('',(#43439,#43440,#43441,#43442));
#8237=EDGE_LOOP('',(#43443,#43444,#43445,#43446));
#8238=EDGE_LOOP('',(#43447,#43448,#43449,#43450));
#8239=EDGE_LOOP('',(#43451,#43452,#43453,#43454));
#8240=EDGE_LOOP('',(#43455,#43456,#43457,#43458));
#8241=EDGE_LOOP('',(#43459,#43460,#43461,#43462));
#8242=EDGE_LOOP('',(#43463,#43464,#43465,#43466));
#8243=EDGE_LOOP('',(#43467,#43468,#43469,#43470));
#8244=EDGE_LOOP('',(#43471,#43472,#43473,#43474));
#8245=EDGE_LOOP('',(#43475,#43476,#43477,#43478));
#8246=EDGE_LOOP('',(#43479,#43480,#43481,#43482));
#8247=EDGE_LOOP('',(#43483,#43484,#43485,#43486));
#8248=EDGE_LOOP('',(#43487,#43488,#43489,#43490));
#8249=EDGE_LOOP('',(#43491,#43492,#43493,#43494));
#8250=EDGE_LOOP('',(#43495,#43496,#43497,#43498));
#8251=EDGE_LOOP('',(#43499,#43500,#43501,#43502));
#8252=EDGE_LOOP('',(#43503,#43504,#43505,#43506));
#8253=EDGE_LOOP('',(#43507,#43508,#43509,#43510));
#8254=EDGE_LOOP('',(#43511,#43512,#43513,#43514));
#8255=EDGE_LOOP('',(#43515,#43516,#43517,#43518));
#8256=EDGE_LOOP('',(#43519,#43520,#43521,#43522));
#8257=EDGE_LOOP('',(#43523,#43524,#43525,#43526));
#8258=EDGE_LOOP('',(#43527,#43528,#43529,#43530));
#8259=EDGE_LOOP('',(#43531,#43532,#43533,#43534));
#8260=EDGE_LOOP('',(#43535,#43536,#43537,#43538));
#8261=EDGE_LOOP('',(#43539,#43540,#43541,#43542));
#8262=EDGE_LOOP('',(#43543,#43544,#43545,#43546));
#8263=EDGE_LOOP('',(#43547,#43548,#43549,#43550));
#8264=EDGE_LOOP('',(#43551,#43552,#43553,#43554));
#8265=EDGE_LOOP('',(#43555,#43556,#43557,#43558));
#8266=EDGE_LOOP('',(#43559,#43560,#43561,#43562));
#8267=EDGE_LOOP('',(#43563,#43564,#43565,#43566));
#8268=EDGE_LOOP('',(#43567,#43568,#43569,#43570));
#8269=EDGE_LOOP('',(#43571,#43572,#43573,#43574));
#8270=EDGE_LOOP('',(#43575,#43576,#43577,#43578));
#8271=EDGE_LOOP('',(#43579,#43580,#43581,#43582));
#8272=EDGE_LOOP('',(#43583,#43584,#43585,#43586));
#8273=EDGE_LOOP('',(#43587,#43588,#43589,#43590));
#8274=EDGE_LOOP('',(#43591,#43592,#43593,#43594));
#8275=EDGE_LOOP('',(#43595,#43596,#43597,#43598));
#8276=EDGE_LOOP('',(#43599,#43600,#43601,#43602));
#8277=EDGE_LOOP('',(#43603,#43604,#43605,#43606));
#8278=EDGE_LOOP('',(#43607,#43608,#43609,#43610));
#8279=EDGE_LOOP('',(#43611,#43612,#43613,#43614));
#8280=EDGE_LOOP('',(#43615,#43616,#43617,#43618));
#8281=EDGE_LOOP('',(#43619,#43620,#43621,#43622));
#8282=EDGE_LOOP('',(#43623,#43624,#43625,#43626));
#8283=EDGE_LOOP('',(#43627,#43628,#43629,#43630));
#8284=EDGE_LOOP('',(#43631,#43632,#43633,#43634));
#8285=EDGE_LOOP('',(#43635,#43636,#43637,#43638));
#8286=EDGE_LOOP('',(#43639,#43640,#43641,#43642));
#8287=EDGE_LOOP('',(#43643,#43644,#43645,#43646));
#8288=EDGE_LOOP('',(#43647,#43648,#43649,#43650));
#8289=EDGE_LOOP('',(#43651,#43652,#43653,#43654));
#8290=EDGE_LOOP('',(#43655,#43656,#43657,#43658));
#8291=EDGE_LOOP('',(#43659,#43660,#43661,#43662));
#8292=EDGE_LOOP('',(#43663,#43664,#43665,#43666));
#8293=EDGE_LOOP('',(#43667,#43668,#43669,#43670));
#8294=EDGE_LOOP('',(#43671,#43672,#43673,#43674));
#8295=EDGE_LOOP('',(#43675,#43676,#43677,#43678));
#8296=EDGE_LOOP('',(#43679,#43680,#43681,#43682));
#8297=EDGE_LOOP('',(#43683,#43684,#43685,#43686));
#8298=EDGE_LOOP('',(#43687,#43688,#43689,#43690));
#8299=EDGE_LOOP('',(#43691,#43692,#43693,#43694));
#8300=EDGE_LOOP('',(#43695,#43696,#43697,#43698));
#8301=EDGE_LOOP('',(#43699,#43700,#43701,#43702));
#8302=EDGE_LOOP('',(#43703,#43704,#43705,#43706));
#8303=EDGE_LOOP('',(#43707,#43708,#43709,#43710));
#8304=EDGE_LOOP('',(#43711,#43712,#43713,#43714));
#8305=EDGE_LOOP('',(#43715,#43716,#43717,#43718));
#8306=EDGE_LOOP('',(#43719,#43720,#43721,#43722));
#8307=EDGE_LOOP('',(#43723,#43724,#43725,#43726));
#8308=EDGE_LOOP('',(#43727,#43728,#43729,#43730));
#8309=EDGE_LOOP('',(#43731,#43732,#43733,#43734));
#8310=EDGE_LOOP('',(#43735,#43736,#43737,#43738));
#8311=EDGE_LOOP('',(#43739,#43740,#43741,#43742));
#8312=EDGE_LOOP('',(#43743,#43744,#43745,#43746));
#8313=EDGE_LOOP('',(#43747,#43748,#43749,#43750));
#8314=EDGE_LOOP('',(#43751,#43752,#43753,#43754));
#8315=EDGE_LOOP('',(#43755,#43756,#43757,#43758));
#8316=EDGE_LOOP('',(#43759,#43760,#43761,#43762));
#8317=EDGE_LOOP('',(#43763,#43764,#43765,#43766));
#8318=EDGE_LOOP('',(#43767,#43768,#43769,#43770));
#8319=EDGE_LOOP('',(#43771,#43772,#43773,#43774));
#8320=EDGE_LOOP('',(#43775,#43776,#43777,#43778));
#8321=EDGE_LOOP('',(#43779,#43780,#43781,#43782));
#8322=EDGE_LOOP('',(#43783,#43784,#43785,#43786));
#8323=EDGE_LOOP('',(#43787,#43788,#43789,#43790));
#8324=EDGE_LOOP('',(#43791,#43792,#43793,#43794));
#8325=EDGE_LOOP('',(#43795,#43796,#43797,#43798));
#8326=EDGE_LOOP('',(#43799,#43800,#43801,#43802));
#8327=EDGE_LOOP('',(#43803,#43804,#43805,#43806));
#8328=EDGE_LOOP('',(#43807,#43808,#43809,#43810));
#8329=EDGE_LOOP('',(#43811,#43812,#43813,#43814));
#8330=EDGE_LOOP('',(#43815,#43816,#43817,#43818));
#8331=EDGE_LOOP('',(#43819,#43820,#43821,#43822));
#8332=EDGE_LOOP('',(#43823,#43824,#43825,#43826));
#8333=EDGE_LOOP('',(#43827,#43828,#43829,#43830));
#8334=EDGE_LOOP('',(#43831,#43832,#43833,#43834));
#8335=EDGE_LOOP('',(#43835,#43836,#43837,#43838));
#8336=EDGE_LOOP('',(#43839,#43840,#43841,#43842));
#8337=EDGE_LOOP('',(#43843,#43844,#43845,#43846));
#8338=EDGE_LOOP('',(#43847,#43848,#43849,#43850));
#8339=EDGE_LOOP('',(#43851,#43852,#43853,#43854));
#8340=EDGE_LOOP('',(#43855,#43856,#43857,#43858));
#8341=EDGE_LOOP('',(#43859,#43860,#43861,#43862));
#8342=EDGE_LOOP('',(#43863,#43864,#43865,#43866));
#8343=EDGE_LOOP('',(#43867,#43868,#43869,#43870));
#8344=EDGE_LOOP('',(#43871,#43872,#43873,#43874));
#8345=EDGE_LOOP('',(#43875,#43876,#43877,#43878));
#8346=EDGE_LOOP('',(#43879,#43880,#43881,#43882));
#8347=EDGE_LOOP('',(#43883,#43884,#43885,#43886));
#8348=EDGE_LOOP('',(#43887,#43888,#43889,#43890));
#8349=EDGE_LOOP('',(#43891,#43892,#43893,#43894));
#8350=EDGE_LOOP('',(#43895,#43896,#43897,#43898));
#8351=EDGE_LOOP('',(#43899,#43900,#43901,#43902));
#8352=EDGE_LOOP('',(#43903,#43904,#43905,#43906));
#8353=EDGE_LOOP('',(#43907,#43908,#43909,#43910));
#8354=EDGE_LOOP('',(#43911,#43912,#43913,#43914));
#8355=EDGE_LOOP('',(#43915,#43916,#43917,#43918));
#8356=EDGE_LOOP('',(#43919,#43920,#43921,#43922));
#8357=EDGE_LOOP('',(#43923,#43924,#43925,#43926));
#8358=EDGE_LOOP('',(#43927,#43928,#43929,#43930));
#8359=EDGE_LOOP('',(#43931,#43932,#43933,#43934));
#8360=EDGE_LOOP('',(#43935,#43936,#43937,#43938));
#8361=EDGE_LOOP('',(#43939,#43940,#43941,#43942));
#8362=EDGE_LOOP('',(#43943,#43944,#43945,#43946));
#8363=EDGE_LOOP('',(#43947,#43948,#43949,#43950));
#8364=EDGE_LOOP('',(#43951,#43952,#43953,#43954));
#8365=EDGE_LOOP('',(#43955,#43956,#43957,#43958));
#8366=EDGE_LOOP('',(#43959,#43960,#43961,#43962));
#8367=EDGE_LOOP('',(#43963,#43964,#43965,#43966));
#8368=EDGE_LOOP('',(#43967,#43968,#43969,#43970));
#8369=EDGE_LOOP('',(#43971,#43972,#43973,#43974));
#8370=EDGE_LOOP('',(#43975,#43976,#43977,#43978));
#8371=EDGE_LOOP('',(#43979,#43980,#43981,#43982));
#8372=EDGE_LOOP('',(#43983,#43984,#43985,#43986));
#8373=EDGE_LOOP('',(#43987,#43988,#43989,#43990));
#8374=EDGE_LOOP('',(#43991,#43992,#43993,#43994));
#8375=EDGE_LOOP('',(#43995,#43996,#43997,#43998));
#8376=EDGE_LOOP('',(#43999,#44000,#44001,#44002));
#8377=EDGE_LOOP('',(#44003,#44004,#44005,#44006));
#8378=EDGE_LOOP('',(#44007,#44008,#44009,#44010));
#8379=EDGE_LOOP('',(#44011,#44012,#44013,#44014));
#8380=EDGE_LOOP('',(#44015,#44016,#44017,#44018));
#8381=EDGE_LOOP('',(#44019,#44020,#44021,#44022));
#8382=EDGE_LOOP('',(#44023,#44024,#44025,#44026));
#8383=EDGE_LOOP('',(#44027,#44028,#44029,#44030));
#8384=EDGE_LOOP('',(#44031,#44032,#44033,#44034));
#8385=EDGE_LOOP('',(#44035,#44036,#44037,#44038));
#8386=EDGE_LOOP('',(#44039,#44040,#44041,#44042));
#8387=EDGE_LOOP('',(#44043,#44044,#44045,#44046));
#8388=EDGE_LOOP('',(#44047,#44048,#44049,#44050));
#8389=EDGE_LOOP('',(#44051,#44052,#44053,#44054));
#8390=EDGE_LOOP('',(#44055,#44056,#44057,#44058));
#8391=EDGE_LOOP('',(#44059,#44060,#44061,#44062));
#8392=EDGE_LOOP('',(#44063,#44064,#44065,#44066));
#8393=EDGE_LOOP('',(#44067,#44068,#44069,#44070));
#8394=EDGE_LOOP('',(#44071,#44072,#44073,#44074));
#8395=EDGE_LOOP('',(#44075,#44076,#44077,#44078));
#8396=EDGE_LOOP('',(#44079,#44080,#44081,#44082));
#8397=EDGE_LOOP('',(#44083,#44084,#44085,#44086));
#8398=EDGE_LOOP('',(#44087,#44088,#44089,#44090));
#8399=EDGE_LOOP('',(#44091,#44092,#44093,#44094));
#8400=EDGE_LOOP('',(#44095,#44096,#44097,#44098));
#8401=EDGE_LOOP('',(#44099,#44100,#44101,#44102));
#8402=EDGE_LOOP('',(#44103,#44104,#44105,#44106));
#8403=EDGE_LOOP('',(#44107,#44108,#44109,#44110));
#8404=EDGE_LOOP('',(#44111,#44112,#44113,#44114));
#8405=EDGE_LOOP('',(#44115,#44116,#44117,#44118));
#8406=EDGE_LOOP('',(#44119,#44120,#44121,#44122));
#8407=EDGE_LOOP('',(#44123,#44124,#44125,#44126));
#8408=EDGE_LOOP('',(#44127,#44128,#44129,#44130));
#8409=EDGE_LOOP('',(#44131,#44132,#44133,#44134));
#8410=EDGE_LOOP('',(#44135,#44136,#44137,#44138));
#8411=EDGE_LOOP('',(#44139,#44140,#44141,#44142));
#8412=EDGE_LOOP('',(#44143,#44144,#44145,#44146));
#8413=EDGE_LOOP('',(#44147,#44148,#44149,#44150));
#8414=EDGE_LOOP('',(#44151,#44152,#44153,#44154));
#8415=EDGE_LOOP('',(#44155,#44156,#44157,#44158));
#8416=EDGE_LOOP('',(#44159,#44160,#44161,#44162));
#8417=EDGE_LOOP('',(#44163,#44164,#44165,#44166));
#8418=EDGE_LOOP('',(#44167,#44168,#44169,#44170));
#8419=EDGE_LOOP('',(#44171,#44172,#44173,#44174));
#8420=EDGE_LOOP('',(#44175,#44176,#44177,#44178));
#8421=EDGE_LOOP('',(#44179,#44180,#44181,#44182));
#8422=EDGE_LOOP('',(#44183,#44184,#44185,#44186));
#8423=EDGE_LOOP('',(#44187,#44188,#44189,#44190));
#8424=EDGE_LOOP('',(#44191,#44192,#44193,#44194));
#8425=EDGE_LOOP('',(#44195,#44196,#44197,#44198));
#8426=EDGE_LOOP('',(#44199,#44200,#44201,#44202));
#8427=EDGE_LOOP('',(#44203,#44204,#44205,#44206));
#8428=EDGE_LOOP('',(#44207,#44208,#44209,#44210));
#8429=EDGE_LOOP('',(#44211,#44212,#44213,#44214));
#8430=EDGE_LOOP('',(#44215,#44216,#44217,#44218));
#8431=EDGE_LOOP('',(#44219,#44220,#44221,#44222));
#8432=EDGE_LOOP('',(#44223,#44224,#44225,#44226));
#8433=EDGE_LOOP('',(#44227,#44228,#44229,#44230));
#8434=EDGE_LOOP('',(#44231,#44232,#44233,#44234));
#8435=EDGE_LOOP('',(#44235,#44236,#44237,#44238));
#8436=EDGE_LOOP('',(#44239,#44240,#44241,#44242));
#8437=EDGE_LOOP('',(#44243,#44244,#44245,#44246));
#8438=EDGE_LOOP('',(#44247,#44248,#44249,#44250));
#8439=EDGE_LOOP('',(#44251,#44252,#44253,#44254));
#8440=EDGE_LOOP('',(#44255,#44256,#44257,#44258));
#8441=EDGE_LOOP('',(#44259,#44260,#44261,#44262));
#8442=EDGE_LOOP('',(#44263,#44264,#44265,#44266));
#8443=EDGE_LOOP('',(#44267,#44268,#44269,#44270));
#8444=EDGE_LOOP('',(#44271,#44272,#44273,#44274));
#8445=EDGE_LOOP('',(#44275,#44276,#44277,#44278));
#8446=EDGE_LOOP('',(#44279,#44280,#44281,#44282));
#8447=EDGE_LOOP('',(#44283,#44284,#44285,#44286));
#8448=EDGE_LOOP('',(#44287,#44288,#44289,#44290));
#8449=EDGE_LOOP('',(#44291,#44292,#44293,#44294));
#8450=EDGE_LOOP('',(#44295,#44296,#44297,#44298));
#8451=EDGE_LOOP('',(#44299,#44300,#44301,#44302));
#8452=EDGE_LOOP('',(#44303,#44304,#44305,#44306));
#8453=EDGE_LOOP('',(#44307,#44308,#44309,#44310));
#8454=EDGE_LOOP('',(#44311,#44312,#44313,#44314));
#8455=EDGE_LOOP('',(#44315,#44316,#44317,#44318));
#8456=EDGE_LOOP('',(#44319,#44320,#44321,#44322));
#8457=EDGE_LOOP('',(#44323,#44324,#44325,#44326));
#8458=EDGE_LOOP('',(#44327,#44328,#44329,#44330));
#8459=EDGE_LOOP('',(#44331,#44332,#44333,#44334));
#8460=EDGE_LOOP('',(#44335,#44336,#44337,#44338));
#8461=EDGE_LOOP('',(#44339,#44340,#44341,#44342));
#8462=EDGE_LOOP('',(#44343,#44344,#44345,#44346));
#8463=EDGE_LOOP('',(#44347,#44348,#44349,#44350));
#8464=EDGE_LOOP('',(#44351,#44352,#44353,#44354));
#8465=EDGE_LOOP('',(#44355,#44356,#44357,#44358));
#8466=EDGE_LOOP('',(#44359,#44360,#44361,#44362));
#8467=EDGE_LOOP('',(#44363,#44364,#44365,#44366));
#8468=EDGE_LOOP('',(#44367,#44368,#44369,#44370));
#8469=EDGE_LOOP('',(#44371,#44372,#44373,#44374));
#8470=EDGE_LOOP('',(#44375,#44376,#44377,#44378));
#8471=EDGE_LOOP('',(#44379,#44380,#44381,#44382));
#8472=EDGE_LOOP('',(#44383,#44384,#44385,#44386));
#8473=EDGE_LOOP('',(#44387,#44388,#44389,#44390));
#8474=EDGE_LOOP('',(#44391,#44392,#44393,#44394));
#8475=EDGE_LOOP('',(#44395,#44396,#44397,#44398));
#8476=EDGE_LOOP('',(#44399,#44400,#44401,#44402));
#8477=EDGE_LOOP('',(#44403,#44404,#44405,#44406));
#8478=EDGE_LOOP('',(#44407,#44408,#44409,#44410));
#8479=EDGE_LOOP('',(#44411,#44412,#44413,#44414));
#8480=EDGE_LOOP('',(#44415,#44416,#44417,#44418));
#8481=EDGE_LOOP('',(#44419,#44420,#44421,#44422));
#8482=EDGE_LOOP('',(#44423,#44424,#44425,#44426));
#8483=EDGE_LOOP('',(#44427,#44428,#44429,#44430));
#8484=EDGE_LOOP('',(#44431,#44432,#44433,#44434));
#8485=EDGE_LOOP('',(#44435,#44436,#44437,#44438));
#8486=EDGE_LOOP('',(#44439,#44440,#44441,#44442));
#8487=EDGE_LOOP('',(#44443,#44444,#44445,#44446));
#8488=EDGE_LOOP('',(#44447,#44448,#44449,#44450));
#8489=EDGE_LOOP('',(#44451,#44452,#44453,#44454));
#8490=EDGE_LOOP('',(#44455,#44456,#44457,#44458));
#8491=EDGE_LOOP('',(#44459,#44460,#44461,#44462));
#8492=EDGE_LOOP('',(#44463,#44464,#44465,#44466));
#8493=EDGE_LOOP('',(#44467,#44468,#44469,#44470));
#8494=EDGE_LOOP('',(#44471,#44472,#44473,#44474));
#8495=EDGE_LOOP('',(#44475,#44476,#44477,#44478));
#8496=EDGE_LOOP('',(#44479,#44480,#44481,#44482));
#8497=EDGE_LOOP('',(#44483,#44484,#44485,#44486));
#8498=EDGE_LOOP('',(#44487,#44488,#44489,#44490));
#8499=EDGE_LOOP('',(#44491,#44492,#44493,#44494));
#8500=EDGE_LOOP('',(#44495,#44496,#44497,#44498));
#8501=EDGE_LOOP('',(#44499,#44500,#44501,#44502));
#8502=EDGE_LOOP('',(#44503,#44504,#44505,#44506));
#8503=EDGE_LOOP('',(#44507,#44508,#44509,#44510));
#8504=EDGE_LOOP('',(#44511,#44512,#44513,#44514));
#8505=EDGE_LOOP('',(#44515,#44516,#44517,#44518));
#8506=EDGE_LOOP('',(#44519,#44520,#44521,#44522));
#8507=EDGE_LOOP('',(#44523,#44524,#44525,#44526));
#8508=EDGE_LOOP('',(#44527,#44528,#44529,#44530));
#8509=EDGE_LOOP('',(#44531,#44532,#44533,#44534));
#8510=EDGE_LOOP('',(#44535,#44536,#44537,#44538));
#8511=EDGE_LOOP('',(#44539,#44540,#44541,#44542));
#8512=EDGE_LOOP('',(#44543,#44544,#44545,#44546));
#8513=EDGE_LOOP('',(#44547,#44548,#44549,#44550));
#8514=EDGE_LOOP('',(#44551,#44552,#44553,#44554));
#8515=EDGE_LOOP('',(#44555,#44556,#44557,#44558));
#8516=EDGE_LOOP('',(#44559,#44560,#44561,#44562));
#8517=EDGE_LOOP('',(#44563,#44564,#44565,#44566));
#8518=EDGE_LOOP('',(#44567,#44568,#44569,#44570));
#8519=EDGE_LOOP('',(#44571,#44572,#44573,#44574));
#8520=EDGE_LOOP('',(#44575,#44576,#44577,#44578));
#8521=EDGE_LOOP('',(#44579,#44580,#44581,#44582));
#8522=EDGE_LOOP('',(#44583,#44584,#44585,#44586));
#8523=EDGE_LOOP('',(#44587,#44588,#44589,#44590));
#8524=EDGE_LOOP('',(#44591,#44592,#44593,#44594));
#8525=EDGE_LOOP('',(#44595,#44596,#44597,#44598));
#8526=EDGE_LOOP('',(#44599,#44600,#44601,#44602));
#8527=EDGE_LOOP('',(#44603,#44604,#44605,#44606));
#8528=EDGE_LOOP('',(#44607,#44608,#44609,#44610));
#8529=EDGE_LOOP('',(#44611,#44612,#44613,#44614));
#8530=EDGE_LOOP('',(#44615,#44616,#44617,#44618));
#8531=EDGE_LOOP('',(#44619,#44620,#44621,#44622));
#8532=EDGE_LOOP('',(#44623,#44624,#44625,#44626));
#8533=EDGE_LOOP('',(#44627,#44628,#44629,#44630));
#8534=EDGE_LOOP('',(#44631,#44632,#44633,#44634));
#8535=EDGE_LOOP('',(#44635,#44636,#44637,#44638));
#8536=EDGE_LOOP('',(#44639,#44640,#44641,#44642));
#8537=EDGE_LOOP('',(#44643,#44644,#44645,#44646));
#8538=EDGE_LOOP('',(#44647,#44648,#44649,#44650));
#8539=EDGE_LOOP('',(#44651,#44652,#44653,#44654));
#8540=EDGE_LOOP('',(#44655,#44656,#44657,#44658));
#8541=EDGE_LOOP('',(#44659,#44660,#44661,#44662));
#8542=EDGE_LOOP('',(#44663,#44664,#44665,#44666));
#8543=EDGE_LOOP('',(#44667,#44668,#44669,#44670));
#8544=EDGE_LOOP('',(#44671,#44672,#44673,#44674));
#8545=EDGE_LOOP('',(#44675,#44676,#44677,#44678));
#8546=EDGE_LOOP('',(#44679,#44680,#44681,#44682));
#8547=EDGE_LOOP('',(#44683,#44684,#44685,#44686));
#8548=EDGE_LOOP('',(#44687,#44688,#44689,#44690));
#8549=EDGE_LOOP('',(#44691,#44692,#44693,#44694));
#8550=EDGE_LOOP('',(#44695,#44696,#44697,#44698));
#8551=EDGE_LOOP('',(#44699,#44700,#44701,#44702));
#8552=EDGE_LOOP('',(#44703,#44704,#44705,#44706));
#8553=EDGE_LOOP('',(#44707,#44708,#44709,#44710));
#8554=EDGE_LOOP('',(#44711,#44712,#44713,#44714));
#8555=EDGE_LOOP('',(#44715,#44716,#44717,#44718));
#8556=EDGE_LOOP('',(#44719,#44720,#44721,#44722));
#8557=EDGE_LOOP('',(#44723,#44724,#44725,#44726));
#8558=EDGE_LOOP('',(#44727,#44728,#44729,#44730));
#8559=EDGE_LOOP('',(#44731,#44732,#44733,#44734));
#8560=EDGE_LOOP('',(#44735,#44736,#44737,#44738));
#8561=EDGE_LOOP('',(#44739,#44740,#44741,#44742));
#8562=EDGE_LOOP('',(#44743,#44744,#44745,#44746));
#8563=EDGE_LOOP('',(#44747,#44748,#44749,#44750));
#8564=EDGE_LOOP('',(#44751,#44752,#44753,#44754));
#8565=EDGE_LOOP('',(#44755,#44756,#44757,#44758));
#8566=EDGE_LOOP('',(#44759,#44760,#44761,#44762));
#8567=EDGE_LOOP('',(#44763,#44764,#44765,#44766));
#8568=EDGE_LOOP('',(#44767,#44768,#44769,#44770));
#8569=EDGE_LOOP('',(#44771,#44772,#44773,#44774));
#8570=EDGE_LOOP('',(#44775,#44776,#44777,#44778));
#8571=EDGE_LOOP('',(#44779,#44780,#44781,#44782));
#8572=EDGE_LOOP('',(#44783,#44784,#44785,#44786));
#8573=EDGE_LOOP('',(#44787,#44788,#44789,#44790));
#8574=EDGE_LOOP('',(#44791,#44792,#44793,#44794));
#8575=EDGE_LOOP('',(#44795,#44796,#44797,#44798));
#8576=EDGE_LOOP('',(#44799,#44800,#44801,#44802));
#8577=EDGE_LOOP('',(#44803,#44804,#44805,#44806));
#8578=EDGE_LOOP('',(#44807,#44808,#44809,#44810));
#8579=EDGE_LOOP('',(#44811,#44812,#44813,#44814));
#8580=EDGE_LOOP('',(#44815,#44816,#44817,#44818));
#8581=EDGE_LOOP('',(#44819,#44820,#44821,#44822));
#8582=EDGE_LOOP('',(#44823,#44824,#44825,#44826));
#8583=EDGE_LOOP('',(#44827,#44828,#44829,#44830));
#8584=EDGE_LOOP('',(#44831,#44832,#44833,#44834));
#8585=EDGE_LOOP('',(#44835,#44836,#44837,#44838));
#8586=EDGE_LOOP('',(#44839,#44840,#44841,#44842));
#8587=EDGE_LOOP('',(#44843,#44844,#44845,#44846));
#8588=EDGE_LOOP('',(#44847,#44848,#44849,#44850));
#8589=EDGE_LOOP('',(#44851,#44852,#44853,#44854));
#8590=EDGE_LOOP('',(#44855,#44856,#44857,#44858));
#8591=EDGE_LOOP('',(#44859,#44860,#44861,#44862));
#8592=EDGE_LOOP('',(#44863,#44864,#44865,#44866));
#8593=EDGE_LOOP('',(#44867,#44868,#44869,#44870));
#8594=EDGE_LOOP('',(#44871,#44872,#44873,#44874));
#8595=EDGE_LOOP('',(#44875,#44876,#44877,#44878));
#8596=EDGE_LOOP('',(#44879,#44880,#44881,#44882));
#8597=EDGE_LOOP('',(#44883,#44884,#44885,#44886));
#8598=EDGE_LOOP('',(#44887,#44888,#44889,#44890));
#8599=EDGE_LOOP('',(#44891,#44892,#44893,#44894));
#8600=EDGE_LOOP('',(#44895,#44896,#44897,#44898));
#8601=EDGE_LOOP('',(#44899,#44900,#44901,#44902));
#8602=EDGE_LOOP('',(#44903,#44904,#44905,#44906));
#8603=EDGE_LOOP('',(#44907,#44908,#44909,#44910));
#8604=EDGE_LOOP('',(#44911,#44912,#44913,#44914));
#8605=EDGE_LOOP('',(#44915,#44916,#44917,#44918));
#8606=EDGE_LOOP('',(#44919,#44920,#44921,#44922));
#8607=EDGE_LOOP('',(#44923,#44924,#44925,#44926));
#8608=EDGE_LOOP('',(#44927,#44928,#44929,#44930));
#8609=EDGE_LOOP('',(#44931,#44932,#44933,#44934));
#8610=EDGE_LOOP('',(#44935,#44936,#44937,#44938));
#8611=EDGE_LOOP('',(#44939,#44940,#44941,#44942));
#8612=EDGE_LOOP('',(#44943,#44944,#44945,#44946));
#8613=EDGE_LOOP('',(#44947,#44948,#44949,#44950));
#8614=EDGE_LOOP('',(#44951,#44952,#44953,#44954));
#8615=EDGE_LOOP('',(#44955,#44956,#44957,#44958));
#8616=EDGE_LOOP('',(#44959,#44960,#44961,#44962));
#8617=EDGE_LOOP('',(#44963,#44964,#44965,#44966));
#8618=EDGE_LOOP('',(#44967,#44968,#44969,#44970));
#8619=EDGE_LOOP('',(#44971,#44972,#44973,#44974));
#8620=EDGE_LOOP('',(#44975,#44976,#44977,#44978));
#8621=EDGE_LOOP('',(#44979,#44980,#44981,#44982));
#8622=EDGE_LOOP('',(#44983,#44984,#44985,#44986));
#8623=EDGE_LOOP('',(#44987,#44988,#44989,#44990));
#8624=EDGE_LOOP('',(#44991,#44992,#44993,#44994));
#8625=EDGE_LOOP('',(#44995,#44996,#44997,#44998));
#8626=EDGE_LOOP('',(#44999,#45000,#45001,#45002));
#8627=EDGE_LOOP('',(#45003,#45004,#45005,#45006));
#8628=EDGE_LOOP('',(#45007,#45008,#45009,#45010));
#8629=EDGE_LOOP('',(#45011,#45012,#45013,#45014));
#8630=EDGE_LOOP('',(#45015,#45016,#45017,#45018));
#8631=EDGE_LOOP('',(#45019,#45020,#45021,#45022));
#8632=EDGE_LOOP('',(#45023,#45024,#45025,#45026));
#8633=EDGE_LOOP('',(#45027,#45028,#45029,#45030));
#8634=EDGE_LOOP('',(#45031,#45032,#45033,#45034));
#8635=EDGE_LOOP('',(#45035,#45036,#45037,#45038));
#8636=EDGE_LOOP('',(#45039,#45040,#45041,#45042));
#8637=EDGE_LOOP('',(#45043,#45044,#45045,#45046));
#8638=EDGE_LOOP('',(#45047,#45048,#45049,#45050));
#8639=EDGE_LOOP('',(#45051,#45052,#45053,#45054));
#8640=EDGE_LOOP('',(#45055,#45056,#45057,#45058));
#8641=EDGE_LOOP('',(#45059,#45060,#45061,#45062));
#8642=EDGE_LOOP('',(#45063,#45064,#45065,#45066));
#8643=EDGE_LOOP('',(#45067,#45068,#45069,#45070));
#8644=EDGE_LOOP('',(#45071,#45072,#45073,#45074));
#8645=EDGE_LOOP('',(#45075,#45076,#45077,#45078));
#8646=EDGE_LOOP('',(#45079,#45080,#45081,#45082));
#8647=EDGE_LOOP('',(#45083,#45084,#45085,#45086));
#8648=EDGE_LOOP('',(#45087,#45088,#45089,#45090));
#8649=EDGE_LOOP('',(#45091,#45092,#45093,#45094));
#8650=EDGE_LOOP('',(#45095,#45096,#45097,#45098));
#8651=EDGE_LOOP('',(#45099,#45100,#45101,#45102));
#8652=EDGE_LOOP('',(#45103,#45104,#45105,#45106));
#8653=EDGE_LOOP('',(#45107,#45108,#45109,#45110));
#8654=EDGE_LOOP('',(#45111,#45112,#45113,#45114));
#8655=EDGE_LOOP('',(#45115,#45116,#45117,#45118));
#8656=EDGE_LOOP('',(#45119,#45120,#45121,#45122));
#8657=EDGE_LOOP('',(#45123,#45124,#45125,#45126));
#8658=EDGE_LOOP('',(#45127,#45128,#45129,#45130));
#8659=EDGE_LOOP('',(#45131,#45132,#45133,#45134));
#8660=EDGE_LOOP('',(#45135,#45136,#45137,#45138));
#8661=EDGE_LOOP('',(#45139,#45140,#45141,#45142));
#8662=EDGE_LOOP('',(#45143,#45144,#45145,#45146));
#8663=EDGE_LOOP('',(#45147,#45148,#45149,#45150));
#8664=EDGE_LOOP('',(#45151,#45152,#45153,#45154));
#8665=EDGE_LOOP('',(#45155,#45156,#45157,#45158));
#8666=EDGE_LOOP('',(#45159,#45160,#45161,#45162));
#8667=EDGE_LOOP('',(#45163,#45164,#45165,#45166));
#8668=EDGE_LOOP('',(#45167,#45168,#45169,#45170));
#8669=EDGE_LOOP('',(#45171,#45172,#45173,#45174));
#8670=EDGE_LOOP('',(#45175,#45176,#45177,#45178));
#8671=EDGE_LOOP('',(#45179,#45180,#45181,#45182));
#8672=EDGE_LOOP('',(#45183,#45184,#45185,#45186));
#8673=EDGE_LOOP('',(#45187,#45188,#45189,#45190));
#8674=EDGE_LOOP('',(#45191,#45192,#45193,#45194));
#8675=EDGE_LOOP('',(#45195,#45196,#45197,#45198));
#8676=EDGE_LOOP('',(#45199,#45200,#45201,#45202));
#8677=EDGE_LOOP('',(#45203,#45204,#45205,#45206));
#8678=EDGE_LOOP('',(#45207,#45208,#45209,#45210));
#8679=EDGE_LOOP('',(#45211,#45212,#45213,#45214));
#8680=EDGE_LOOP('',(#45215,#45216,#45217,#45218));
#8681=EDGE_LOOP('',(#45219,#45220,#45221,#45222));
#8682=EDGE_LOOP('',(#45223,#45224,#45225,#45226));
#8683=EDGE_LOOP('',(#45227,#45228,#45229,#45230));
#8684=EDGE_LOOP('',(#45231,#45232,#45233,#45234));
#8685=EDGE_LOOP('',(#45235,#45236,#45237,#45238));
#8686=EDGE_LOOP('',(#45239,#45240,#45241,#45242));
#8687=EDGE_LOOP('',(#45243,#45244,#45245,#45246));
#8688=EDGE_LOOP('',(#45247,#45248,#45249,#45250));
#8689=EDGE_LOOP('',(#45251,#45252,#45253,#45254));
#8690=EDGE_LOOP('',(#45255,#45256,#45257,#45258));
#8691=EDGE_LOOP('',(#45259,#45260,#45261,#45262));
#8692=EDGE_LOOP('',(#45263,#45264,#45265,#45266));
#8693=EDGE_LOOP('',(#45267,#45268,#45269,#45270));
#8694=EDGE_LOOP('',(#45271,#45272,#45273,#45274));
#8695=EDGE_LOOP('',(#45275,#45276,#45277,#45278));
#8696=EDGE_LOOP('',(#45279,#45280,#45281,#45282));
#8697=EDGE_LOOP('',(#45283,#45284,#45285,#45286));
#8698=EDGE_LOOP('',(#45287,#45288,#45289,#45290));
#8699=EDGE_LOOP('',(#45291,#45292,#45293,#45294));
#8700=EDGE_LOOP('',(#45295,#45296,#45297,#45298));
#8701=EDGE_LOOP('',(#45299,#45300,#45301,#45302));
#8702=EDGE_LOOP('',(#45303,#45304,#45305,#45306));
#8703=EDGE_LOOP('',(#45307,#45308,#45309,#45310));
#8704=EDGE_LOOP('',(#45311,#45312,#45313,#45314));
#8705=EDGE_LOOP('',(#45315,#45316,#45317,#45318));
#8706=EDGE_LOOP('',(#45319,#45320,#45321,#45322));
#8707=EDGE_LOOP('',(#45323,#45324,#45325,#45326));
#8708=EDGE_LOOP('',(#45327,#45328,#45329,#45330));
#8709=EDGE_LOOP('',(#45331,#45332,#45333,#45334));
#8710=EDGE_LOOP('',(#45335,#45336,#45337,#45338));
#8711=EDGE_LOOP('',(#45339,#45340,#45341,#45342));
#8712=EDGE_LOOP('',(#45343,#45344,#45345,#45346));
#8713=EDGE_LOOP('',(#45347,#45348,#45349,#45350));
#8714=EDGE_LOOP('',(#45351,#45352,#45353,#45354));
#8715=EDGE_LOOP('',(#45355,#45356,#45357,#45358));
#8716=EDGE_LOOP('',(#45359,#45360,#45361,#45362));
#8717=EDGE_LOOP('',(#45363,#45364,#45365,#45366));
#8718=EDGE_LOOP('',(#45367,#45368,#45369,#45370));
#8719=EDGE_LOOP('',(#45371,#45372,#45373,#45374));
#8720=EDGE_LOOP('',(#45375,#45376,#45377,#45378));
#8721=EDGE_LOOP('',(#45379,#45380,#45381,#45382));
#8722=EDGE_LOOP('',(#45383,#45384,#45385,#45386));
#8723=EDGE_LOOP('',(#45387,#45388,#45389,#45390));
#8724=EDGE_LOOP('',(#45391,#45392,#45393,#45394));
#8725=EDGE_LOOP('',(#45395,#45396,#45397,#45398));
#8726=EDGE_LOOP('',(#45399,#45400,#45401,#45402));
#8727=EDGE_LOOP('',(#45403,#45404,#45405,#45406));
#8728=EDGE_LOOP('',(#45407,#45408,#45409,#45410));
#8729=EDGE_LOOP('',(#45411,#45412,#45413,#45414));
#8730=EDGE_LOOP('',(#45415,#45416,#45417,#45418));
#8731=EDGE_LOOP('',(#45419,#45420,#45421,#45422));
#8732=EDGE_LOOP('',(#45423,#45424,#45425,#45426));
#8733=EDGE_LOOP('',(#45427,#45428,#45429,#45430));
#8734=EDGE_LOOP('',(#45431,#45432,#45433,#45434));
#8735=EDGE_LOOP('',(#45435,#45436,#45437,#45438));
#8736=EDGE_LOOP('',(#45439,#45440,#45441,#45442));
#8737=EDGE_LOOP('',(#45443,#45444,#45445,#45446));
#8738=EDGE_LOOP('',(#45447,#45448,#45449,#45450));
#8739=EDGE_LOOP('',(#45451,#45452,#45453,#45454));
#8740=EDGE_LOOP('',(#45455,#45456,#45457,#45458));
#8741=EDGE_LOOP('',(#45459,#45460,#45461,#45462));
#8742=EDGE_LOOP('',(#45463,#45464,#45465,#45466));
#8743=EDGE_LOOP('',(#45467,#45468,#45469,#45470));
#8744=EDGE_LOOP('',(#45471,#45472,#45473,#45474));
#8745=EDGE_LOOP('',(#45475,#45476,#45477,#45478));
#8746=EDGE_LOOP('',(#45479,#45480,#45481,#45482));
#8747=EDGE_LOOP('',(#45483,#45484,#45485,#45486));
#8748=EDGE_LOOP('',(#45487,#45488,#45489,#45490));
#8749=EDGE_LOOP('',(#45491,#45492,#45493,#45494));
#8750=EDGE_LOOP('',(#45495,#45496,#45497,#45498));
#8751=EDGE_LOOP('',(#45499,#45500,#45501,#45502));
#8752=EDGE_LOOP('',(#45503,#45504,#45505,#45506));
#8753=EDGE_LOOP('',(#45507,#45508,#45509,#45510));
#8754=EDGE_LOOP('',(#45511,#45512,#45513,#45514));
#8755=EDGE_LOOP('',(#45515,#45516,#45517,#45518));
#8756=EDGE_LOOP('',(#45519,#45520,#45521,#45522));
#8757=EDGE_LOOP('',(#45523,#45524,#45525,#45526));
#8758=EDGE_LOOP('',(#45527,#45528,#45529,#45530));
#8759=EDGE_LOOP('',(#45531,#45532,#45533,#45534));
#8760=EDGE_LOOP('',(#45535,#45536,#45537,#45538));
#8761=EDGE_LOOP('',(#45539,#45540,#45541,#45542));
#8762=EDGE_LOOP('',(#45543,#45544,#45545,#45546));
#8763=EDGE_LOOP('',(#45547,#45548,#45549,#45550));
#8764=EDGE_LOOP('',(#45551,#45552,#45553,#45554));
#8765=EDGE_LOOP('',(#45555,#45556,#45557,#45558));
#8766=EDGE_LOOP('',(#45559,#45560,#45561,#45562));
#8767=EDGE_LOOP('',(#45563,#45564,#45565,#45566));
#8768=EDGE_LOOP('',(#45567,#45568,#45569,#45570));
#8769=EDGE_LOOP('',(#45571,#45572,#45573,#45574));
#8770=EDGE_LOOP('',(#45575,#45576,#45577,#45578));
#8771=EDGE_LOOP('',(#45579,#45580,#45581,#45582));
#8772=EDGE_LOOP('',(#45583,#45584,#45585,#45586));
#8773=EDGE_LOOP('',(#45587,#45588,#45589,#45590));
#8774=EDGE_LOOP('',(#45591,#45592,#45593,#45594));
#8775=EDGE_LOOP('',(#45595,#45596,#45597,#45598));
#8776=EDGE_LOOP('',(#45599,#45600,#45601,#45602));
#8777=EDGE_LOOP('',(#45603,#45604,#45605,#45606));
#8778=EDGE_LOOP('',(#45607,#45608,#45609,#45610));
#8779=EDGE_LOOP('',(#45611,#45612,#45613,#45614));
#8780=EDGE_LOOP('',(#45615,#45616,#45617,#45618));
#8781=EDGE_LOOP('',(#45619,#45620,#45621,#45622));
#8782=EDGE_LOOP('',(#45623,#45624,#45625,#45626));
#8783=EDGE_LOOP('',(#45627,#45628,#45629,#45630));
#8784=EDGE_LOOP('',(#45631,#45632,#45633,#45634));
#8785=EDGE_LOOP('',(#45635,#45636,#45637,#45638));
#8786=EDGE_LOOP('',(#45639,#45640,#45641,#45642));
#8787=EDGE_LOOP('',(#45643,#45644,#45645,#45646));
#8788=EDGE_LOOP('',(#45647,#45648,#45649,#45650));
#8789=EDGE_LOOP('',(#45651,#45652,#45653,#45654));
#8790=EDGE_LOOP('',(#45655,#45656,#45657,#45658));
#8791=EDGE_LOOP('',(#45659,#45660,#45661,#45662));
#8792=EDGE_LOOP('',(#45663,#45664,#45665,#45666));
#8793=EDGE_LOOP('',(#45667,#45668,#45669,#45670));
#8794=EDGE_LOOP('',(#45671,#45672,#45673,#45674));
#8795=EDGE_LOOP('',(#45675,#45676,#45677,#45678));
#8796=EDGE_LOOP('',(#45679,#45680,#45681,#45682));
#8797=EDGE_LOOP('',(#45683,#45684,#45685,#45686));
#8798=EDGE_LOOP('',(#45687,#45688,#45689,#45690));
#8799=EDGE_LOOP('',(#45691,#45692,#45693,#45694));
#8800=EDGE_LOOP('',(#45695,#45696,#45697,#45698));
#8801=EDGE_LOOP('',(#45699,#45700,#45701,#45702));
#8802=EDGE_LOOP('',(#45703,#45704,#45705,#45706));
#8803=EDGE_LOOP('',(#45707,#45708,#45709,#45710));
#8804=EDGE_LOOP('',(#45711,#45712,#45713,#45714));
#8805=EDGE_LOOP('',(#45715,#45716,#45717,#45718));
#8806=EDGE_LOOP('',(#45719,#45720,#45721,#45722));
#8807=EDGE_LOOP('',(#45723,#45724,#45725,#45726));
#8808=EDGE_LOOP('',(#45727,#45728,#45729,#45730));
#8809=EDGE_LOOP('',(#45731,#45732,#45733,#45734));
#8810=EDGE_LOOP('',(#45735,#45736,#45737,#45738));
#8811=EDGE_LOOP('',(#45739,#45740,#45741,#45742));
#8812=EDGE_LOOP('',(#45743,#45744,#45745,#45746));
#8813=EDGE_LOOP('',(#45747,#45748,#45749,#45750));
#8814=EDGE_LOOP('',(#45751,#45752,#45753,#45754));
#8815=EDGE_LOOP('',(#45755,#45756,#45757,#45758));
#8816=EDGE_LOOP('',(#45759,#45760,#45761,#45762));
#8817=EDGE_LOOP('',(#45763,#45764,#45765,#45766));
#8818=EDGE_LOOP('',(#45767,#45768,#45769,#45770));
#8819=EDGE_LOOP('',(#45771,#45772,#45773,#45774));
#8820=EDGE_LOOP('',(#45775,#45776,#45777,#45778));
#8821=EDGE_LOOP('',(#45779,#45780,#45781,#45782));
#8822=EDGE_LOOP('',(#45783,#45784,#45785,#45786));
#8823=EDGE_LOOP('',(#45787,#45788,#45789,#45790));
#8824=EDGE_LOOP('',(#45791,#45792,#45793,#45794));
#8825=EDGE_LOOP('',(#45795,#45796,#45797,#45798));
#8826=EDGE_LOOP('',(#45799,#45800,#45801,#45802));
#8827=EDGE_LOOP('',(#45803,#45804,#45805,#45806));
#8828=EDGE_LOOP('',(#45807,#45808,#45809,#45810));
#8829=EDGE_LOOP('',(#45811,#45812,#45813,#45814));
#8830=EDGE_LOOP('',(#45815,#45816,#45817,#45818));
#8831=EDGE_LOOP('',(#45819,#45820,#45821,#45822));
#8832=EDGE_LOOP('',(#45823,#45824,#45825,#45826));
#8833=EDGE_LOOP('',(#45827,#45828,#45829,#45830));
#8834=EDGE_LOOP('',(#45831,#45832,#45833,#45834));
#8835=EDGE_LOOP('',(#45835,#45836,#45837,#45838));
#8836=EDGE_LOOP('',(#45839,#45840,#45841,#45842));
#8837=EDGE_LOOP('',(#45843,#45844,#45845,#45846));
#8838=EDGE_LOOP('',(#45847,#45848,#45849,#45850));
#8839=EDGE_LOOP('',(#45851,#45852,#45853,#45854));
#8840=EDGE_LOOP('',(#45855,#45856,#45857,#45858));
#8841=EDGE_LOOP('',(#45859,#45860,#45861,#45862));
#8842=EDGE_LOOP('',(#45863,#45864,#45865,#45866));
#8843=EDGE_LOOP('',(#45867,#45868,#45869,#45870));
#8844=EDGE_LOOP('',(#45871,#45872,#45873,#45874));
#8845=EDGE_LOOP('',(#45875,#45876,#45877,#45878));
#8846=EDGE_LOOP('',(#45879,#45880,#45881,#45882));
#8847=EDGE_LOOP('',(#45883,#45884,#45885,#45886));
#8848=EDGE_LOOP('',(#45887,#45888,#45889,#45890));
#8849=EDGE_LOOP('',(#45891,#45892,#45893,#45894));
#8850=EDGE_LOOP('',(#45895,#45896,#45897,#45898));
#8851=EDGE_LOOP('',(#45899,#45900,#45901,#45902));
#8852=EDGE_LOOP('',(#45903,#45904,#45905,#45906));
#8853=EDGE_LOOP('',(#45907,#45908,#45909,#45910));
#8854=EDGE_LOOP('',(#45911,#45912,#45913,#45914));
#8855=EDGE_LOOP('',(#45915,#45916,#45917,#45918));
#8856=EDGE_LOOP('',(#45919,#45920,#45921,#45922));
#8857=EDGE_LOOP('',(#45923,#45924,#45925,#45926));
#8858=EDGE_LOOP('',(#45927,#45928,#45929,#45930));
#8859=EDGE_LOOP('',(#45931,#45932,#45933,#45934));
#8860=EDGE_LOOP('',(#45935,#45936,#45937,#45938));
#8861=EDGE_LOOP('',(#45939,#45940,#45941,#45942));
#8862=EDGE_LOOP('',(#45943,#45944,#45945,#45946));
#8863=EDGE_LOOP('',(#45947,#45948,#45949,#45950));
#8864=EDGE_LOOP('',(#45951,#45952,#45953,#45954));
#8865=EDGE_LOOP('',(#45955,#45956,#45957,#45958));
#8866=EDGE_LOOP('',(#45959,#45960,#45961,#45962));
#8867=EDGE_LOOP('',(#45963,#45964,#45965,#45966));
#8868=EDGE_LOOP('',(#45967,#45968,#45969,#45970));
#8869=EDGE_LOOP('',(#45971,#45972,#45973,#45974));
#8870=EDGE_LOOP('',(#45975,#45976,#45977,#45978));
#8871=EDGE_LOOP('',(#45979,#45980,#45981,#45982));
#8872=EDGE_LOOP('',(#45983,#45984,#45985,#45986));
#8873=EDGE_LOOP('',(#45987,#45988,#45989,#45990));
#8874=EDGE_LOOP('',(#45991,#45992,#45993,#45994));
#8875=EDGE_LOOP('',(#45995,#45996,#45997,#45998));
#8876=EDGE_LOOP('',(#45999,#46000,#46001,#46002));
#8877=EDGE_LOOP('',(#46003,#46004,#46005,#46006));
#8878=EDGE_LOOP('',(#46007,#46008,#46009,#46010));
#8879=EDGE_LOOP('',(#46011,#46012,#46013,#46014));
#8880=EDGE_LOOP('',(#46015,#46016,#46017,#46018));
#8881=EDGE_LOOP('',(#46019,#46020,#46021,#46022));
#8882=EDGE_LOOP('',(#46023,#46024,#46025,#46026));
#8883=EDGE_LOOP('',(#46027,#46028,#46029,#46030));
#8884=EDGE_LOOP('',(#46031,#46032,#46033,#46034));
#8885=EDGE_LOOP('',(#46035,#46036,#46037,#46038));
#8886=EDGE_LOOP('',(#46039,#46040,#46041,#46042));
#8887=EDGE_LOOP('',(#46043,#46044,#46045,#46046));
#8888=EDGE_LOOP('',(#46047,#46048,#46049,#46050));
#8889=EDGE_LOOP('',(#46051,#46052,#46053,#46054));
#8890=EDGE_LOOP('',(#46055,#46056,#46057,#46058));
#8891=EDGE_LOOP('',(#46059,#46060,#46061,#46062));
#8892=EDGE_LOOP('',(#46063,#46064,#46065,#46066));
#8893=EDGE_LOOP('',(#46067,#46068,#46069,#46070));
#8894=EDGE_LOOP('',(#46071,#46072,#46073,#46074));
#8895=EDGE_LOOP('',(#46075,#46076,#46077,#46078));
#8896=EDGE_LOOP('',(#46079,#46080,#46081,#46082));
#8897=EDGE_LOOP('',(#46083,#46084,#46085,#46086));
#8898=EDGE_LOOP('',(#46087,#46088,#46089,#46090));
#8899=EDGE_LOOP('',(#46091,#46092,#46093,#46094));
#8900=EDGE_LOOP('',(#46095,#46096,#46097,#46098));
#8901=EDGE_LOOP('',(#46099,#46100,#46101,#46102));
#8902=EDGE_LOOP('',(#46103,#46104,#46105,#46106));
#8903=EDGE_LOOP('',(#46107,#46108,#46109,#46110));
#8904=EDGE_LOOP('',(#46111,#46112,#46113,#46114));
#8905=EDGE_LOOP('',(#46115,#46116,#46117,#46118));
#8906=EDGE_LOOP('',(#46119,#46120,#46121,#46122));
#8907=EDGE_LOOP('',(#46123,#46124,#46125,#46126));
#8908=EDGE_LOOP('',(#46127,#46128,#46129,#46130));
#8909=EDGE_LOOP('',(#46131,#46132,#46133,#46134));
#8910=EDGE_LOOP('',(#46135,#46136,#46137,#46138));
#8911=EDGE_LOOP('',(#46139,#46140,#46141,#46142));
#8912=EDGE_LOOP('',(#46143,#46144,#46145,#46146));
#8913=EDGE_LOOP('',(#46147,#46148,#46149,#46150));
#8914=EDGE_LOOP('',(#46151,#46152,#46153,#46154));
#8915=EDGE_LOOP('',(#46155,#46156,#46157,#46158));
#8916=EDGE_LOOP('',(#46159,#46160,#46161,#46162));
#8917=EDGE_LOOP('',(#46163,#46164,#46165,#46166));
#8918=EDGE_LOOP('',(#46167,#46168,#46169,#46170));
#8919=EDGE_LOOP('',(#46171,#46172,#46173,#46174));
#8920=EDGE_LOOP('',(#46175,#46176,#46177,#46178));
#8921=EDGE_LOOP('',(#46179,#46180,#46181,#46182));
#8922=EDGE_LOOP('',(#46183,#46184,#46185,#46186));
#8923=EDGE_LOOP('',(#46187,#46188,#46189,#46190));
#8924=EDGE_LOOP('',(#46191,#46192,#46193,#46194));
#8925=EDGE_LOOP('',(#46195,#46196,#46197,#46198));
#8926=EDGE_LOOP('',(#46199,#46200,#46201,#46202));
#8927=EDGE_LOOP('',(#46203,#46204,#46205,#46206));
#8928=EDGE_LOOP('',(#46207,#46208,#46209,#46210));
#8929=EDGE_LOOP('',(#46211,#46212,#46213,#46214));
#8930=EDGE_LOOP('',(#46215,#46216,#46217,#46218));
#8931=EDGE_LOOP('',(#46219,#46220,#46221,#46222));
#8932=EDGE_LOOP('',(#46223,#46224,#46225,#46226));
#8933=EDGE_LOOP('',(#46227,#46228,#46229,#46230));
#8934=EDGE_LOOP('',(#46231,#46232,#46233,#46234));
#8935=EDGE_LOOP('',(#46235,#46236,#46237,#46238));
#8936=EDGE_LOOP('',(#46239,#46240,#46241,#46242));
#8937=EDGE_LOOP('',(#46243,#46244,#46245,#46246));
#8938=EDGE_LOOP('',(#46247,#46248,#46249,#46250));
#8939=EDGE_LOOP('',(#46251,#46252,#46253,#46254));
#8940=EDGE_LOOP('',(#46255,#46256,#46257,#46258));
#8941=EDGE_LOOP('',(#46259,#46260,#46261,#46262));
#8942=EDGE_LOOP('',(#46263,#46264,#46265,#46266));
#8943=EDGE_LOOP('',(#46267,#46268,#46269,#46270));
#8944=EDGE_LOOP('',(#46271,#46272,#46273,#46274));
#8945=EDGE_LOOP('',(#46275,#46276,#46277,#46278));
#8946=EDGE_LOOP('',(#46279,#46280,#46281,#46282));
#8947=EDGE_LOOP('',(#46283,#46284,#46285,#46286));
#8948=EDGE_LOOP('',(#46287,#46288,#46289,#46290));
#8949=EDGE_LOOP('',(#46291,#46292,#46293,#46294));
#8950=EDGE_LOOP('',(#46295,#46296,#46297,#46298));
#8951=EDGE_LOOP('',(#46299,#46300,#46301,#46302));
#8952=EDGE_LOOP('',(#46303,#46304,#46305,#46306));
#8953=EDGE_LOOP('',(#46307,#46308,#46309,#46310));
#8954=EDGE_LOOP('',(#46311,#46312,#46313,#46314));
#8955=EDGE_LOOP('',(#46315,#46316,#46317,#46318));
#8956=EDGE_LOOP('',(#46319,#46320,#46321,#46322));
#8957=EDGE_LOOP('',(#46323,#46324,#46325,#46326));
#8958=EDGE_LOOP('',(#46327,#46328,#46329,#46330));
#8959=EDGE_LOOP('',(#46331,#46332,#46333,#46334));
#8960=EDGE_LOOP('',(#46335,#46336,#46337,#46338));
#8961=EDGE_LOOP('',(#46339,#46340,#46341,#46342));
#8962=EDGE_LOOP('',(#46343,#46344,#46345,#46346));
#8963=EDGE_LOOP('',(#46347,#46348,#46349,#46350));
#8964=EDGE_LOOP('',(#46351,#46352,#46353,#46354));
#8965=EDGE_LOOP('',(#46355,#46356,#46357,#46358));
#8966=EDGE_LOOP('',(#46359,#46360,#46361,#46362));
#8967=EDGE_LOOP('',(#46363,#46364,#46365,#46366));
#8968=EDGE_LOOP('',(#46367,#46368,#46369,#46370));
#8969=EDGE_LOOP('',(#46371,#46372,#46373,#46374));
#8970=EDGE_LOOP('',(#46375,#46376,#46377,#46378));
#8971=EDGE_LOOP('',(#46379,#46380,#46381,#46382));
#8972=EDGE_LOOP('',(#46383,#46384,#46385,#46386));
#8973=EDGE_LOOP('',(#46387,#46388,#46389,#46390));
#8974=EDGE_LOOP('',(#46391,#46392,#46393,#46394));
#8975=EDGE_LOOP('',(#46395,#46396,#46397,#46398));
#8976=EDGE_LOOP('',(#46399,#46400,#46401,#46402));
#8977=EDGE_LOOP('',(#46403,#46404,#46405,#46406));
#8978=EDGE_LOOP('',(#46407,#46408,#46409,#46410));
#8979=EDGE_LOOP('',(#46411,#46412,#46413,#46414));
#8980=EDGE_LOOP('',(#46415,#46416,#46417,#46418));
#8981=EDGE_LOOP('',(#46419,#46420,#46421,#46422));
#8982=EDGE_LOOP('',(#46423,#46424,#46425,#46426));
#8983=EDGE_LOOP('',(#46427,#46428,#46429,#46430));
#8984=EDGE_LOOP('',(#46431,#46432,#46433,#46434));
#8985=EDGE_LOOP('',(#46435,#46436,#46437,#46438));
#8986=EDGE_LOOP('',(#46439,#46440,#46441,#46442));
#8987=EDGE_LOOP('',(#46443,#46444,#46445,#46446));
#8988=EDGE_LOOP('',(#46447,#46448,#46449,#46450));
#8989=EDGE_LOOP('',(#46451,#46452,#46453,#46454));
#8990=EDGE_LOOP('',(#46455,#46456,#46457,#46458));
#8991=EDGE_LOOP('',(#46459,#46460,#46461,#46462));
#8992=EDGE_LOOP('',(#46463,#46464,#46465,#46466));
#8993=EDGE_LOOP('',(#46467,#46468,#46469,#46470));
#8994=EDGE_LOOP('',(#46471,#46472,#46473,#46474));
#8995=EDGE_LOOP('',(#46475,#46476,#46477,#46478));
#8996=EDGE_LOOP('',(#46479,#46480,#46481,#46482));
#8997=EDGE_LOOP('',(#46483,#46484,#46485,#46486));
#8998=EDGE_LOOP('',(#46487,#46488,#46489,#46490));
#8999=EDGE_LOOP('',(#46491,#46492,#46493,#46494));
#9000=EDGE_LOOP('',(#46495,#46496,#46497,#46498));
#9001=EDGE_LOOP('',(#46499,#46500,#46501,#46502));
#9002=EDGE_LOOP('',(#46503,#46504,#46505,#46506));
#9003=EDGE_LOOP('',(#46507,#46508,#46509,#46510));
#9004=EDGE_LOOP('',(#46511,#46512,#46513,#46514));
#9005=EDGE_LOOP('',(#46515,#46516,#46517,#46518));
#9006=EDGE_LOOP('',(#46519,#46520,#46521,#46522));
#9007=EDGE_LOOP('',(#46523,#46524,#46525,#46526));
#9008=EDGE_LOOP('',(#46527,#46528,#46529,#46530));
#9009=EDGE_LOOP('',(#46531,#46532,#46533,#46534));
#9010=EDGE_LOOP('',(#46535,#46536,#46537,#46538));
#9011=EDGE_LOOP('',(#46539,#46540,#46541,#46542));
#9012=EDGE_LOOP('',(#46543,#46544,#46545,#46546));
#9013=EDGE_LOOP('',(#46547,#46548,#46549,#46550));
#9014=EDGE_LOOP('',(#46551,#46552,#46553,#46554));
#9015=EDGE_LOOP('',(#46555,#46556,#46557,#46558));
#9016=EDGE_LOOP('',(#46559,#46560,#46561,#46562));
#9017=EDGE_LOOP('',(#46563,#46564,#46565,#46566));
#9018=EDGE_LOOP('',(#46567,#46568,#46569,#46570));
#9019=EDGE_LOOP('',(#46571,#46572,#46573,#46574));
#9020=EDGE_LOOP('',(#46575,#46576,#46577,#46578));
#9021=EDGE_LOOP('',(#46579,#46580,#46581,#46582));
#9022=EDGE_LOOP('',(#46583,#46584,#46585,#46586));
#9023=EDGE_LOOP('',(#46587,#46588,#46589,#46590));
#9024=EDGE_LOOP('',(#46591,#46592,#46593,#46594));
#9025=EDGE_LOOP('',(#46595,#46596,#46597,#46598));
#9026=EDGE_LOOP('',(#46599,#46600,#46601,#46602));
#9027=EDGE_LOOP('',(#46603,#46604,#46605,#46606));
#9028=EDGE_LOOP('',(#46607,#46608,#46609,#46610));
#9029=EDGE_LOOP('',(#46611,#46612,#46613,#46614));
#9030=EDGE_LOOP('',(#46615,#46616,#46617,#46618));
#9031=EDGE_LOOP('',(#46619,#46620,#46621,#46622));
#9032=EDGE_LOOP('',(#46623,#46624,#46625,#46626));
#9033=EDGE_LOOP('',(#46627,#46628,#46629,#46630));
#9034=EDGE_LOOP('',(#46631,#46632,#46633,#46634));
#9035=EDGE_LOOP('',(#46635,#46636,#46637,#46638));
#9036=EDGE_LOOP('',(#46639,#46640,#46641,#46642));
#9037=EDGE_LOOP('',(#46643,#46644,#46645,#46646));
#9038=EDGE_LOOP('',(#46647,#46648,#46649,#46650));
#9039=EDGE_LOOP('',(#46651,#46652,#46653,#46654));
#9040=EDGE_LOOP('',(#46655,#46656,#46657,#46658));
#9041=EDGE_LOOP('',(#46659,#46660,#46661,#46662));
#9042=EDGE_LOOP('',(#46663,#46664,#46665,#46666));
#9043=EDGE_LOOP('',(#46667,#46668,#46669,#46670));
#9044=EDGE_LOOP('',(#46671,#46672,#46673,#46674));
#9045=EDGE_LOOP('',(#46675,#46676,#46677,#46678));
#9046=EDGE_LOOP('',(#46679,#46680,#46681,#46682));
#9047=EDGE_LOOP('',(#46683,#46684,#46685,#46686));
#9048=EDGE_LOOP('',(#46687,#46688,#46689,#46690));
#9049=EDGE_LOOP('',(#46691,#46692,#46693,#46694));
#9050=EDGE_LOOP('',(#46695,#46696,#46697,#46698));
#9051=EDGE_LOOP('',(#46699,#46700,#46701,#46702));
#9052=EDGE_LOOP('',(#46703,#46704,#46705,#46706));
#9053=EDGE_LOOP('',(#46707,#46708,#46709,#46710));
#9054=EDGE_LOOP('',(#46711,#46712,#46713,#46714));
#9055=EDGE_LOOP('',(#46715,#46716,#46717,#46718));
#9056=EDGE_LOOP('',(#46719,#46720,#46721,#46722));
#9057=EDGE_LOOP('',(#46723,#46724,#46725,#46726));
#9058=EDGE_LOOP('',(#46727,#46728,#46729,#46730));
#9059=EDGE_LOOP('',(#46731,#46732,#46733,#46734));
#9060=EDGE_LOOP('',(#46735,#46736,#46737,#46738));
#9061=EDGE_LOOP('',(#46739,#46740,#46741,#46742));
#9062=EDGE_LOOP('',(#46743,#46744,#46745,#46746));
#9063=EDGE_LOOP('',(#46747,#46748,#46749,#46750));
#9064=EDGE_LOOP('',(#46751,#46752,#46753,#46754));
#9065=EDGE_LOOP('',(#46755,#46756,#46757,#46758));
#9066=EDGE_LOOP('',(#46759,#46760,#46761,#46762));
#9067=EDGE_LOOP('',(#46763,#46764,#46765,#46766));
#9068=EDGE_LOOP('',(#46767,#46768,#46769,#46770));
#9069=EDGE_LOOP('',(#46771,#46772,#46773,#46774));
#9070=EDGE_LOOP('',(#46775,#46776,#46777,#46778,#46779,#46780));
#9071=EDGE_LOOP('',(#46781,#46782,#46783,#46784,#46785,#46786));
#9072=EDGE_LOOP('',(#46787,#46788,#46789,#46790));
#9073=EDGE_LOOP('',(#46791,#46792,#46793,#46794,#46795,#46796,#46797,#46798,
#46799,#46800,#46801,#46802,#46803,#46804,#46805,#46806,#46807,#46808,#46809,
#46810,#46811,#46812,#46813,#46814));
#9074=EDGE_LOOP('',(#46815,#46816,#46817,#46818));
#9075=EDGE_LOOP('',(#46819,#46820,#46821,#46822));
#9076=EDGE_LOOP('',(#46823,#46824,#46825,#46826));
#9077=EDGE_LOOP('',(#46827,#46828,#46829,#46830));
#9078=EDGE_LOOP('',(#46831));
#9079=EDGE_LOOP('',(#46832));
#9080=EDGE_LOOP('',(#46833));
#9081=EDGE_LOOP('',(#46834,#46835,#46836));
#9082=EDGE_LOOP('',(#46837,#46838,#46839));
#9083=EDGE_LOOP('',(#46840,#46841,#46842,#46843));
#9084=EDGE_LOOP('',(#46844,#46845,#46846,#46847));
#9085=EDGE_LOOP('',(#46848,#46849,#46850,#46851));
#9086=EDGE_LOOP('',(#46852,#46853,#46854,#46855));
#9087=EDGE_LOOP('',(#46856,#46857,#46858,#46859));
#9088=EDGE_LOOP('',(#46860));
#9089=EDGE_LOOP('',(#46861));
#9090=EDGE_LOOP('',(#46862,#46863,#46864));
#9091=EDGE_LOOP('',(#46865,#46866,#46867,#46868));
#9092=EDGE_LOOP('',(#46869,#46870,#46871,#46872));
#9093=EDGE_LOOP('',(#46873,#46874,#46875));
#9094=EDGE_LOOP('',(#46876,#46877,#46878,#46879));
#9095=EDGE_LOOP('',(#46880));
#9096=EDGE_LOOP('',(#46881));
#9097=EDGE_LOOP('',(#46882,#46883,#46884,#46885));
#9098=EDGE_LOOP('',(#46886));
#9099=EDGE_LOOP('',(#46887));
#9100=EDGE_LOOP('',(#46888,#46889,#46890,#46891));
#9101=EDGE_LOOP('',(#46892));
#9102=EDGE_LOOP('',(#46893));
#9103=EDGE_LOOP('',(#46894,#46895,#46896,#46897));
#9104=EDGE_LOOP('',(#46898));
#9105=EDGE_LOOP('',(#46899));
#9106=EDGE_LOOP('',(#46900,#46901,#46902,#46903));
#9107=EDGE_LOOP('',(#46904));
#9108=EDGE_LOOP('',(#46905));
#9109=EDGE_LOOP('',(#46906,#46907,#46908,#46909));
#9110=EDGE_LOOP('',(#46910));
#9111=EDGE_LOOP('',(#46911));
#9112=EDGE_LOOP('',(#46912,#46913,#46914,#46915));
#9113=EDGE_LOOP('',(#46916,#46917,#46918,#46919));
#9114=EDGE_LOOP('',(#46920));
#9115=EDGE_LOOP('',(#46921));
#9116=EDGE_LOOP('',(#46922));
#9117=EDGE_LOOP('',(#46923,#46924,#46925,#46926));
#9118=EDGE_LOOP('',(#46927,#46928,#46929,#46930));
#9119=EDGE_LOOP('',(#46931,#46932,#46933,#46934));
#9120=EDGE_LOOP('',(#46935,#46936,#46937,#46938));
#9121=EDGE_LOOP('',(#46939,#46940,#46941,#46942));
#9122=EDGE_LOOP('',(#46943,#46944,#46945,#46946));
#9123=EDGE_LOOP('',(#46947,#46948,#46949,#46950));
#9124=EDGE_LOOP('',(#46951,#46952,#46953,#46954));
#9125=EDGE_LOOP('',(#46955,#46956,#46957,#46958));
#9126=EDGE_LOOP('',(#46959,#46960,#46961,#46962));
#9127=EDGE_LOOP('',(#46963,#46964,#46965,#46966));
#9128=EDGE_LOOP('',(#46967,#46968,#46969,#46970));
#9129=EDGE_LOOP('',(#46971,#46972,#46973,#46974));
#9130=EDGE_LOOP('',(#46975,#46976,#46977,#46978));
#9131=EDGE_LOOP('',(#46979,#46980,#46981,#46982));
#9132=EDGE_LOOP('',(#46983,#46984,#46985,#46986));
#9133=EDGE_LOOP('',(#46987,#46988,#46989,#46990));
#9134=EDGE_LOOP('',(#46991,#46992,#46993,#46994));
#9135=EDGE_LOOP('',(#46995,#46996,#46997,#46998));
#9136=EDGE_LOOP('',(#46999,#47000,#47001,#47002));
#9137=EDGE_LOOP('',(#47003,#47004,#47005,#47006,#47007,#47008,#47009,#47010));
#9138=EDGE_LOOP('',(#47011,#47012,#47013,#47014));
#9139=EDGE_LOOP('',(#47015,#47016,#47017,#47018));
#9140=EDGE_LOOP('',(#47019,#47020,#47021,#47022));
#9141=EDGE_LOOP('',(#47023,#47024,#47025,#47026));
#9142=EDGE_LOOP('',(#47027,#47028,#47029,#47030));
#9143=EDGE_LOOP('',(#47031,#47032,#47033,#47034));
#9144=EDGE_LOOP('',(#47035,#47036,#47037,#47038));
#9145=EDGE_LOOP('',(#47039,#47040,#47041,#47042));
#9146=EDGE_LOOP('',(#47043,#47044,#47045,#47046));
#9147=EDGE_LOOP('',(#47047,#47048,#47049,#47050));
#9148=EDGE_LOOP('',(#47051,#47052,#47053,#47054));
#9149=EDGE_LOOP('',(#47055,#47056,#47057,#47058));
#9150=EDGE_LOOP('',(#47059,#47060,#47061,#47062));
#9151=EDGE_LOOP('',(#47063,#47064,#47065,#47066));
#9152=EDGE_LOOP('',(#47067));
#9153=EDGE_LOOP('',(#47068));
#9154=EDGE_LOOP('',(#47069));
#9155=EDGE_LOOP('',(#47070));
#9156=EDGE_LOOP('',(#47071,#47072,#47073,#47074));
#9157=EDGE_LOOP('',(#47075,#47076,#47077,#47078));
#9158=EDGE_LOOP('',(#47079,#47080,#47081,#47082));
#9159=EDGE_LOOP('',(#47083,#47084,#47085,#47086));
#9160=EDGE_LOOP('',(#47087,#47088,#47089,#47090));
#9161=EDGE_LOOP('',(#47091,#47092,#47093,#47094,#47095,#47096,#47097,#47098,
#47099,#47100,#47101,#47102));
#9162=EDGE_LOOP('',(#47103,#47104,#47105,#47106,#47107,#47108,#47109,#47110,
#47111,#47112,#47113,#47114,#47115,#47116,#47117,#47118));
#9163=EDGE_LOOP('',(#47119,#47120,#47121,#47122,#47123,#47124,#47125,#47126,
#47127,#47128,#47129,#47130));
#9164=EDGE_LOOP('',(#47131,#47132,#47133,#47134,#47135,#47136,#47137,#47138,
#47139,#47140,#47141,#47142,#47143,#47144,#47145,#47146,#47147,#47148,#47149));
#9165=EDGE_LOOP('',(#47150,#47151,#47152,#47153,#47154,#47155,#47156,#47157,
#47158,#47159,#47160,#47161));
#9166=EDGE_LOOP('',(#47162,#47163,#47164,#47165,#47166,#47167,#47168,#47169,
#47170,#47171,#47172));
#9167=EDGE_LOOP('',(#47173,#47174,#47175,#47176,#47177,#47178,#47179,#47180,
#47181,#47182,#47183,#47184));
#9168=EDGE_LOOP('',(#47185,#47186,#47187,#47188,#47189,#47190,#47191,#47192,
#47193,#47194,#47195,#47196,#47197,#47198,#47199,#47200,#47201,#47202,#47203,
#47204,#47205,#47206));
#9169=EDGE_LOOP('',(#47207,#47208,#47209,#47210,#47211,#47212,#47213,#47214,
#47215,#47216,#47217,#47218));
#9170=EDGE_LOOP('',(#47219,#47220,#47221,#47222,#47223,#47224,#47225,#47226,
#47227,#47228,#47229,#47230));
#9171=EDGE_LOOP('',(#47231,#47232,#47233,#47234,#47235,#47236,#47237,#47238,
#47239,#47240,#47241,#47242,#47243,#47244,#47245,#47246,#47247,#47248,#47249,
#47250,#47251,#47252));
#9172=EDGE_LOOP('',(#47253,#47254,#47255,#47256,#47257,#47258,#47259,#47260,
#47261,#47262,#47263,#47264));
#9173=EDGE_LOOP('',(#47265,#47266,#47267,#47268,#47269,#47270,#47271,#47272,
#47273,#47274,#47275));
#9174=EDGE_LOOP('',(#47276,#47277,#47278,#47279,#47280,#47281,#47282,#47283,
#47284,#47285,#47286,#47287));
#9175=EDGE_LOOP('',(#47288,#47289,#47290,#47291,#47292,#47293,#47294,#47295,
#47296,#47297,#47298,#47299,#47300,#47301,#47302,#47303,#47304,#47305,#47306));
#9176=EDGE_LOOP('',(#47307,#47308,#47309,#47310,#47311,#47312,#47313,#47314,
#47315,#47316,#47317,#47318));
#9177=EDGE_LOOP('',(#47319,#47320,#47321,#47322,#47323,#47324,#47325,#47326,
#47327,#47328,#47329,#47330,#47331,#47332,#47333,#47334));
#9178=EDGE_LOOP('',(#47335,#47336,#47337,#47338));
#9179=EDGE_LOOP('',(#47339,#47340,#47341,#47342));
#9180=EDGE_LOOP('',(#47343,#47344,#47345,#47346));
#9181=EDGE_LOOP('',(#47347,#47348,#47349,#47350));
#9182=EDGE_LOOP('',(#47351,#47352,#47353,#47354));
#9183=EDGE_LOOP('',(#47355,#47356,#47357,#47358));
#9184=EDGE_LOOP('',(#47359,#47360,#47361,#47362));
#9185=EDGE_LOOP('',(#47363,#47364,#47365,#47366));
#9186=EDGE_LOOP('',(#47367,#47368,#47369,#47370));
#9187=EDGE_LOOP('',(#47371,#47372,#47373,#47374));
#9188=EDGE_LOOP('',(#47375,#47376,#47377,#47378));
#9189=EDGE_LOOP('',(#47379,#47380,#47381,#47382));
#9190=EDGE_LOOP('',(#47383,#47384,#47385,#47386));
#9191=EDGE_LOOP('',(#47387,#47388,#47389,#47390));
#9192=EDGE_LOOP('',(#47391,#47392,#47393,#47394));
#9193=EDGE_LOOP('',(#47395,#47396,#47397,#47398));
#9194=EDGE_LOOP('',(#47399,#47400,#47401,#47402));
#9195=EDGE_LOOP('',(#47403,#47404,#47405,#47406));
#9196=EDGE_LOOP('',(#47407,#47408,#47409,#47410));
#9197=EDGE_LOOP('',(#47411,#47412,#47413,#47414));
#9198=EDGE_LOOP('',(#47415,#47416,#47417,#47418));
#9199=EDGE_LOOP('',(#47419,#47420,#47421,#47422));
#9200=EDGE_LOOP('',(#47423,#47424,#47425,#47426));
#9201=EDGE_LOOP('',(#47427,#47428,#47429,#47430));
#9202=EDGE_LOOP('',(#47431,#47432,#47433,#47434));
#9203=EDGE_LOOP('',(#47435,#47436,#47437,#47438));
#9204=EDGE_LOOP('',(#47439,#47440,#47441,#47442));
#9205=EDGE_LOOP('',(#47443,#47444,#47445,#47446));
#9206=EDGE_LOOP('',(#47447,#47448,#47449,#47450));
#9207=EDGE_LOOP('',(#47451,#47452,#47453,#47454));
#9208=EDGE_LOOP('',(#47455,#47456,#47457,#47458));
#9209=EDGE_LOOP('',(#47459,#47460,#47461,#47462));
#9210=EDGE_LOOP('',(#47463,#47464,#47465,#47466));
#9211=EDGE_LOOP('',(#47467,#47468,#47469,#47470));
#9212=EDGE_LOOP('',(#47471,#47472,#47473,#47474));
#9213=EDGE_LOOP('',(#47475,#47476,#47477,#47478));
#9214=EDGE_LOOP('',(#47479,#47480,#47481,#47482));
#9215=EDGE_LOOP('',(#47483,#47484,#47485,#47486));
#9216=EDGE_LOOP('',(#47487,#47488,#47489,#47490));
#9217=EDGE_LOOP('',(#47491,#47492,#47493,#47494));
#9218=EDGE_LOOP('',(#47495,#47496,#47497,#47498));
#9219=EDGE_LOOP('',(#47499,#47500,#47501,#47502));
#9220=EDGE_LOOP('',(#47503,#47504,#47505,#47506));
#9221=EDGE_LOOP('',(#47507,#47508,#47509,#47510));
#9222=EDGE_LOOP('',(#47511,#47512,#47513,#47514));
#9223=EDGE_LOOP('',(#47515,#47516,#47517,#47518));
#9224=EDGE_LOOP('',(#47519,#47520,#47521,#47522));
#9225=EDGE_LOOP('',(#47523,#47524,#47525,#47526));
#9226=EDGE_LOOP('',(#47527,#47528,#47529,#47530));
#9227=EDGE_LOOP('',(#47531,#47532,#47533,#47534));
#9228=EDGE_LOOP('',(#47535,#47536,#47537,#47538));
#9229=EDGE_LOOP('',(#47539,#47540,#47541,#47542));
#9230=EDGE_LOOP('',(#47543,#47544,#47545,#47546));
#9231=EDGE_LOOP('',(#47547,#47548,#47549,#47550));
#9232=EDGE_LOOP('',(#47551,#47552,#47553,#47554));
#9233=EDGE_LOOP('',(#47555,#47556,#47557,#47558));
#9234=EDGE_LOOP('',(#47559,#47560,#47561,#47562));
#9235=EDGE_LOOP('',(#47563,#47564,#47565,#47566));
#9236=EDGE_LOOP('',(#47567,#47568,#47569,#47570));
#9237=EDGE_LOOP('',(#47571,#47572,#47573,#47574));
#9238=EDGE_LOOP('',(#47575,#47576,#47577,#47578));
#9239=EDGE_LOOP('',(#47579,#47580,#47581,#47582));
#9240=EDGE_LOOP('',(#47583,#47584,#47585,#47586));
#9241=EDGE_LOOP('',(#47587,#47588,#47589,#47590));
#9242=EDGE_LOOP('',(#47591,#47592,#47593,#47594));
#9243=EDGE_LOOP('',(#47595,#47596,#47597,#47598));
#9244=EDGE_LOOP('',(#47599,#47600,#47601,#47602));
#9245=EDGE_LOOP('',(#47603,#47604,#47605,#47606));
#9246=EDGE_LOOP('',(#47607,#47608,#47609,#47610));
#9247=EDGE_LOOP('',(#47611,#47612,#47613,#47614));
#9248=EDGE_LOOP('',(#47615,#47616,#47617,#47618));
#9249=EDGE_LOOP('',(#47619,#47620,#47621,#47622));
#9250=EDGE_LOOP('',(#47623,#47624,#47625,#47626));
#9251=EDGE_LOOP('',(#47627,#47628,#47629,#47630));
#9252=EDGE_LOOP('',(#47631,#47632,#47633,#47634));
#9253=EDGE_LOOP('',(#47635,#47636,#47637,#47638));
#9254=EDGE_LOOP('',(#47639,#47640,#47641,#47642));
#9255=EDGE_LOOP('',(#47643,#47644,#47645,#47646));
#9256=EDGE_LOOP('',(#47647,#47648,#47649,#47650));
#9257=EDGE_LOOP('',(#47651,#47652,#47653,#47654));
#9258=EDGE_LOOP('',(#47655,#47656,#47657,#47658));
#9259=EDGE_LOOP('',(#47659,#47660,#47661,#47662));
#9260=EDGE_LOOP('',(#47663,#47664,#47665,#47666));
#9261=EDGE_LOOP('',(#47667,#47668,#47669,#47670));
#9262=EDGE_LOOP('',(#47671,#47672,#47673,#47674));
#9263=EDGE_LOOP('',(#47675,#47676,#47677,#47678));
#9264=EDGE_LOOP('',(#47679,#47680,#47681,#47682));
#9265=EDGE_LOOP('',(#47683,#47684,#47685,#47686));
#9266=EDGE_LOOP('',(#47687,#47688,#47689,#47690));
#9267=EDGE_LOOP('',(#47691,#47692,#47693,#47694));
#9268=EDGE_LOOP('',(#47695,#47696,#47697,#47698));
#9269=EDGE_LOOP('',(#47699,#47700,#47701,#47702));
#9270=EDGE_LOOP('',(#47703,#47704,#47705,#47706));
#9271=EDGE_LOOP('',(#47707,#47708,#47709,#47710));
#9272=EDGE_LOOP('',(#47711,#47712,#47713,#47714));
#9273=EDGE_LOOP('',(#47715,#47716,#47717,#47718));
#9274=EDGE_LOOP('',(#47719,#47720,#47721,#47722));
#9275=EDGE_LOOP('',(#47723,#47724,#47725,#47726));
#9276=EDGE_LOOP('',(#47727,#47728,#47729,#47730));
#9277=EDGE_LOOP('',(#47731,#47732,#47733,#47734));
#9278=EDGE_LOOP('',(#47735,#47736,#47737,#47738));
#9279=EDGE_LOOP('',(#47739,#47740,#47741,#47742));
#9280=EDGE_LOOP('',(#47743,#47744,#47745,#47746));
#9281=EDGE_LOOP('',(#47747,#47748,#47749,#47750));
#9282=EDGE_LOOP('',(#47751,#47752,#47753,#47754));
#9283=EDGE_LOOP('',(#47755,#47756,#47757,#47758));
#9284=EDGE_LOOP('',(#47759,#47760,#47761,#47762));
#9285=EDGE_LOOP('',(#47763,#47764,#47765,#47766));
#9286=EDGE_LOOP('',(#47767,#47768,#47769,#47770));
#9287=EDGE_LOOP('',(#47771,#47772,#47773,#47774));
#9288=EDGE_LOOP('',(#47775,#47776,#47777,#47778));
#9289=EDGE_LOOP('',(#47779,#47780,#47781,#47782));
#9290=EDGE_LOOP('',(#47783,#47784,#47785,#47786));
#9291=EDGE_LOOP('',(#47787,#47788,#47789,#47790));
#9292=EDGE_LOOP('',(#47791,#47792,#47793,#47794));
#9293=EDGE_LOOP('',(#47795,#47796,#47797,#47798));
#9294=EDGE_LOOP('',(#47799,#47800,#47801,#47802));
#9295=EDGE_LOOP('',(#47803,#47804,#47805,#47806));
#9296=EDGE_LOOP('',(#47807,#47808,#47809,#47810));
#9297=EDGE_LOOP('',(#47811,#47812,#47813,#47814));
#9298=EDGE_LOOP('',(#47815,#47816,#47817,#47818));
#9299=EDGE_LOOP('',(#47819,#47820,#47821,#47822));
#9300=EDGE_LOOP('',(#47823,#47824,#47825,#47826));
#9301=EDGE_LOOP('',(#47827,#47828,#47829,#47830));
#9302=EDGE_LOOP('',(#47831,#47832,#47833,#47834));
#9303=EDGE_LOOP('',(#47835,#47836,#47837,#47838));
#9304=EDGE_LOOP('',(#47839,#47840,#47841,#47842));
#9305=EDGE_LOOP('',(#47843,#47844,#47845,#47846));
#9306=EDGE_LOOP('',(#47847,#47848,#47849,#47850));
#9307=EDGE_LOOP('',(#47851,#47852,#47853,#47854));
#9308=EDGE_LOOP('',(#47855,#47856,#47857,#47858));
#9309=EDGE_LOOP('',(#47859,#47860,#47861,#47862));
#9310=EDGE_LOOP('',(#47863,#47864,#47865,#47866));
#9311=EDGE_LOOP('',(#47867,#47868,#47869,#47870));
#9312=EDGE_LOOP('',(#47871,#47872,#47873,#47874));
#9313=EDGE_LOOP('',(#47875,#47876,#47877,#47878));
#9314=EDGE_LOOP('',(#47879,#47880,#47881,#47882));
#9315=EDGE_LOOP('',(#47883,#47884,#47885,#47886));
#9316=EDGE_LOOP('',(#47887,#47888,#47889,#47890));
#9317=EDGE_LOOP('',(#47891,#47892,#47893,#47894));
#9318=EDGE_LOOP('',(#47895,#47896,#47897,#47898));
#9319=EDGE_LOOP('',(#47899,#47900,#47901,#47902));
#9320=EDGE_LOOP('',(#47903,#47904,#47905,#47906));
#9321=EDGE_LOOP('',(#47907,#47908,#47909,#47910));
#9322=EDGE_LOOP('',(#47911,#47912,#47913,#47914));
#9323=EDGE_LOOP('',(#47915,#47916,#47917,#47918));
#9324=EDGE_LOOP('',(#47919,#47920,#47921,#47922));
#9325=EDGE_LOOP('',(#47923,#47924,#47925,#47926));
#9326=EDGE_LOOP('',(#47927,#47928,#47929,#47930));
#9327=EDGE_LOOP('',(#47931,#47932,#47933,#47934));
#9328=EDGE_LOOP('',(#47935,#47936,#47937,#47938));
#9329=EDGE_LOOP('',(#47939,#47940,#47941,#47942));
#9330=EDGE_LOOP('',(#47943,#47944,#47945,#47946));
#9331=EDGE_LOOP('',(#47947,#47948,#47949,#47950));
#9332=EDGE_LOOP('',(#47951,#47952,#47953,#47954));
#9333=EDGE_LOOP('',(#47955,#47956,#47957,#47958));
#9334=EDGE_LOOP('',(#47959,#47960,#47961,#47962));
#9335=EDGE_LOOP('',(#47963,#47964,#47965,#47966));
#9336=EDGE_LOOP('',(#47967,#47968,#47969,#47970));
#9337=EDGE_LOOP('',(#47971,#47972,#47973,#47974));
#9338=EDGE_LOOP('',(#47975,#47976,#47977,#47978));
#9339=EDGE_LOOP('',(#47979,#47980,#47981,#47982));
#9340=EDGE_LOOP('',(#47983,#47984,#47985,#47986));
#9341=EDGE_LOOP('',(#47987,#47988,#47989,#47990));
#9342=EDGE_LOOP('',(#47991,#47992,#47993,#47994));
#9343=EDGE_LOOP('',(#47995,#47996,#47997,#47998));
#9344=EDGE_LOOP('',(#47999,#48000,#48001,#48002));
#9345=EDGE_LOOP('',(#48003,#48004,#48005,#48006));
#9346=EDGE_LOOP('',(#48007,#48008,#48009,#48010));
#9347=EDGE_LOOP('',(#48011,#48012,#48013,#48014));
#9348=EDGE_LOOP('',(#48015,#48016,#48017,#48018));
#9349=EDGE_LOOP('',(#48019,#48020,#48021,#48022));
#9350=EDGE_LOOP('',(#48023,#48024,#48025,#48026));
#9351=EDGE_LOOP('',(#48027,#48028,#48029,#48030));
#9352=EDGE_LOOP('',(#48031,#48032,#48033,#48034));
#9353=EDGE_LOOP('',(#48035,#48036,#48037,#48038));
#9354=EDGE_LOOP('',(#48039,#48040,#48041,#48042));
#9355=EDGE_LOOP('',(#48043,#48044,#48045,#48046));
#9356=EDGE_LOOP('',(#48047,#48048,#48049,#48050));
#9357=EDGE_LOOP('',(#48051,#48052,#48053,#48054));
#9358=EDGE_LOOP('',(#48055,#48056,#48057,#48058));
#9359=EDGE_LOOP('',(#48059,#48060,#48061,#48062,#48063,#48064,#48065,#48066,
#48067,#48068,#48069,#48070,#48071,#48072,#48073,#48074,#48075,#48076,#48077,
#48078,#48079,#48080));
#9360=EDGE_LOOP('',(#48081,#48082,#48083,#48084,#48085,#48086,#48087,#48088,
#48089,#48090,#48091,#48092));
#9361=EDGE_LOOP('',(#48093,#48094,#48095,#48096,#48097,#48098,#48099,#48100,
#48101,#48102,#48103));
#9362=EDGE_LOOP('',(#48104,#48105,#48106,#48107,#48108,#48109,#48110,#48111,
#48112,#48113,#48114,#48115));
#9363=EDGE_LOOP('',(#48116,#48117,#48118,#48119,#48120,#48121,#48122,#48123,
#48124,#48125,#48126,#48127,#48128,#48129,#48130,#48131,#48132,#48133,#48134,
#48135,#48136,#48137));
#9364=EDGE_LOOP('',(#48138,#48139,#48140,#48141,#48142,#48143,#48144,#48145,
#48146,#48147,#48148,#48149));
#9365=EDGE_LOOP('',(#48150,#48151,#48152,#48153,#48154,#48155,#48156,#48157,
#48158,#48159,#48160,#48161,#48162,#48163,#48164,#48165,#48166,#48167,#48168,
#48169,#48170,#48171,#48172,#48173,#48174,#48175,#48176,#48177,#48178,#48179));
#9366=EDGE_LOOP('',(#48180,#48181,#48182,#48183,#48184,#48185,#48186,#48187,
#48188,#48189,#48190,#48191));
#9367=EDGE_LOOP('',(#48192,#48193,#48194,#48195,#48196,#48197,#48198,#48199,
#48200));
#9368=EDGE_LOOP('',(#48201,#48202,#48203,#48204,#48205,#48206,#48207,#48208,
#48209,#48210,#48211,#48212));
#9369=EDGE_LOOP('',(#48213,#48214,#48215,#48216,#48217,#48218,#48219,#48220,
#48221));
#9370=EDGE_LOOP('',(#48222,#48223,#48224,#48225,#48226,#48227,#48228,#48229,
#48230,#48231,#48232,#48233));
#9371=EDGE_LOOP('',(#48234,#48235,#48236,#48237,#48238,#48239,#48240,#48241,
#48242,#48243,#48244,#48245,#48246,#48247,#48248,#48249,#48250,#48251,#48252,
#48253,#48254,#48255,#48256,#48257,#48258,#48259,#48260,#48261,#48262,#48263));
#9372=EDGE_LOOP('',(#48264,#48265,#48266,#48267,#48268,#48269,#48270,#48271,
#48272,#48273,#48274,#48275));
#9373=EDGE_LOOP('',(#48276,#48277,#48278,#48279,#48280,#48281,#48282,#48283,
#48284,#48285,#48286,#48287,#48288,#48289,#48290,#48291,#48292,#48293,#48294,
#48295,#48296,#48297));
#9374=EDGE_LOOP('',(#48298,#48299,#48300,#48301,#48302,#48303,#48304,#48305,
#48306,#48307,#48308,#48309));
#9375=EDGE_LOOP('',(#48310,#48311,#48312,#48313,#48314,#48315,#48316,#48317,
#48318,#48319,#48320));
#9376=EDGE_LOOP('',(#48321,#48322,#48323,#48324,#48325,#48326,#48327,#48328,
#48329,#48330,#48331,#48332));
#9377=EDGE_LOOP('',(#48333,#48334,#48335,#48336,#48337,#48338,#48339,#48340,
#48341,#48342,#48343,#48344,#48345,#48346,#48347,#48348,#48349,#48350,#48351,
#48352,#48353,#48354));
#9378=EDGE_LOOP('',(#48355,#48356,#48357,#48358,#48359,#48360,#48361,#48362,
#48363,#48364,#48365,#48366));
#9379=EDGE_LOOP('',(#48367,#48368,#48369,#48370));
#9380=EDGE_LOOP('',(#48371,#48372,#48373,#48374));
#9381=EDGE_LOOP('',(#48375));
#9382=EDGE_LOOP('',(#48376));
#9383=EDGE_LOOP('',(#48377));
#9384=EDGE_LOOP('',(#48378));
#9385=EDGE_LOOP('',(#48379,#48380,#48381,#48382));
#9386=EDGE_LOOP('',(#48383,#48384,#48385,#48386));
#9387=EDGE_LOOP('',(#48387,#48388,#48389,#48390));
#9388=EDGE_LOOP('',(#48391,#48392,#48393,#48394));
#9389=EDGE_LOOP('',(#48395,#48396,#48397,#48398));
#9390=EDGE_LOOP('',(#48399,#48400,#48401,#48402));
#9391=EDGE_LOOP('',(#48403,#48404,#48405,#48406));
#9392=EDGE_LOOP('',(#48407,#48408,#48409,#48410));
#9393=EDGE_LOOP('',(#48411,#48412,#48413,#48414));
#9394=EDGE_LOOP('',(#48415,#48416,#48417,#48418));
#9395=EDGE_LOOP('',(#48419,#48420,#48421,#48422));
#9396=EDGE_LOOP('',(#48423,#48424,#48425,#48426));
#9397=EDGE_LOOP('',(#48427,#48428,#48429,#48430));
#9398=EDGE_LOOP('',(#48431,#48432,#48433,#48434));
#9399=EDGE_LOOP('',(#48435,#48436,#48437,#48438));
#9400=EDGE_LOOP('',(#48439,#48440,#48441,#48442));
#9401=EDGE_LOOP('',(#48443,#48444,#48445,#48446));
#9402=EDGE_LOOP('',(#48447,#48448,#48449,#48450));
#9403=EDGE_LOOP('',(#48451,#48452,#48453,#48454,#48455,#48456,#48457,#48458,
#48459,#48460,#48461,#48462,#48463,#48464,#48465,#48466,#48467,#48468,#48469,
#48470,#48471,#48472,#48473,#48474));
#9404=EDGE_LOOP('',(#48475,#48476,#48477,#48478));
#9405=EDGE_LOOP('',(#48479,#48480,#48481,#48482,#48483,#48484,#48485,#48486));
#9406=EDGE_LOOP('',(#48487,#48488,#48489,#48490));
#9407=EDGE_LOOP('',(#48491,#48492,#48493,#48494));
#10876=LINE('',#76158,#16910);
#10877=LINE('',#76163,#16911);
#10878=LINE('',#76175,#16912);
#10879=LINE('',#76190,#16913);
#10880=LINE('',#76205,#16914);
#10881=LINE('',#76220,#16915);
#10882=LINE('',#76235,#16916);
#10883=LINE('',#76250,#16917);
#10884=LINE('',#76278,#16918);
#10885=LINE('',#76283,#16919);
#10886=LINE('',#76295,#16920);
#10887=LINE('',#76310,#16921);
#10888=LINE('',#76325,#16922);
#10889=LINE('',#76340,#16923);
#10890=LINE('',#76355,#16924);
#10891=LINE('',#76370,#16925);
#10892=LINE('',#76385,#16926);
#10893=LINE('',#76400,#16927);
#10894=LINE('',#76415,#16928);
#10895=LINE('',#76430,#16929);
#10896=LINE('',#76459,#16930);
#10897=LINE('',#76464,#16931);
#10898=LINE('',#76476,#16932);
#10899=LINE('',#76491,#16933);
#10900=LINE('',#76506,#16934);
#10901=LINE('',#76521,#16935);
#10902=LINE('',#76536,#16936);
#10903=LINE('',#76551,#16937);
#10904=LINE('',#76579,#16938);
#10905=LINE('',#76584,#16939);
#10906=LINE('',#76596,#16940);
#10907=LINE('',#76611,#16941);
#10908=LINE('',#76626,#16942);
#10909=LINE('',#76641,#16943);
#10910=LINE('',#76656,#16944);
#10911=LINE('',#76671,#16945);
#10912=LINE('',#76686,#16946);
#10913=LINE('',#76701,#16947);
#10914=LINE('',#76716,#16948);
#10915=LINE('',#76731,#16949);
#10916=LINE('',#76746,#16950);
#10917=LINE('',#76761,#16951);
#10918=LINE('',#76776,#16952);
#10919=LINE('',#76791,#16953);
#10920=LINE('',#76806,#16954);
#10921=LINE('',#76821,#16955);
#10922=LINE('',#76836,#16956);
#10923=LINE('',#76851,#16957);
#10924=LINE('',#76866,#16958);
#10925=LINE('',#76872,#16959);
#10926=LINE('',#76874,#16960);
#10927=LINE('',#76875,#16961);
#10928=LINE('',#76903,#16962);
#10929=LINE('',#76908,#16963);
#10930=LINE('',#76920,#16964);
#10931=LINE('',#76935,#16965);
#10932=LINE('',#76950,#16966);
#10933=LINE('',#76965,#16967);
#10934=LINE('',#76980,#16968);
#10935=LINE('',#76995,#16969);
#10936=LINE('',#77023,#16970);
#10937=LINE('',#77028,#16971);
#10938=LINE('',#77040,#16972);
#10939=LINE('',#77055,#16973);
#10940=LINE('',#77070,#16974);
#10941=LINE('',#77085,#16975);
#10942=LINE('',#77100,#16976);
#10943=LINE('',#77115,#16977);
#10944=LINE('',#77130,#16978);
#10945=LINE('',#77145,#16979);
#10946=LINE('',#77160,#16980);
#10947=LINE('',#77175,#16981);
#10948=LINE('',#77204,#16982);
#10949=LINE('',#77209,#16983);
#10950=LINE('',#77221,#16984);
#10951=LINE('',#77236,#16985);
#10952=LINE('',#77251,#16986);
#10953=LINE('',#77266,#16987);
#10954=LINE('',#77281,#16988);
#10955=LINE('',#77296,#16989);
#10956=LINE('',#77324,#16990);
#10957=LINE('',#77329,#16991);
#10958=LINE('',#77341,#16992);
#10959=LINE('',#77356,#16993);
#10960=LINE('',#77371,#16994);
#10961=LINE('',#77386,#16995);
#10962=LINE('',#77401,#16996);
#10963=LINE('',#77416,#16997);
#10964=LINE('',#77431,#16998);
#10965=LINE('',#77459,#16999);
#10966=LINE('',#77464,#17000);
#10967=LINE('',#77476,#17001);
#10968=LINE('',#77491,#17002);
#10969=LINE('',#77506,#17003);
#10970=LINE('',#77521,#17004);
#10971=LINE('',#77536,#17005);
#10972=LINE('',#77551,#17006);
#10973=LINE('',#77566,#17007);
#10974=LINE('',#77581,#17008);
#10975=LINE('',#77596,#17009);
#10976=LINE('',#77611,#17010);
#10977=LINE('',#77626,#17011);
#10978=LINE('',#77641,#17012);
#10979=LINE('',#77656,#17013);
#10980=LINE('',#77671,#17014);
#10981=LINE('',#77703,#17015);
#10982=LINE('',#77708,#17016);
#10983=LINE('',#77720,#17017);
#10984=LINE('',#77735,#17018);
#10985=LINE('',#77750,#17019);
#10986=LINE('',#77765,#17020);
#10987=LINE('',#77780,#17021);
#10988=LINE('',#77795,#17022);
#10989=LINE('',#77823,#17023);
#10990=LINE('',#77828,#17024);
#10991=LINE('',#77840,#17025);
#10992=LINE('',#77855,#17026);
#10993=LINE('',#77870,#17027);
#10994=LINE('',#77885,#17028);
#10995=LINE('',#77900,#17029);
#10996=LINE('',#77915,#17030);
#10997=LINE('',#77930,#17031);
#10998=LINE('',#77945,#17032);
#10999=LINE('',#77960,#17033);
#11000=LINE('',#77975,#17034);
#11001=LINE('',#78004,#17035);
#11002=LINE('',#78009,#17036);
#11003=LINE('',#78021,#17037);
#11004=LINE('',#78036,#17038);
#11005=LINE('',#78042,#17039);
#11006=LINE('',#78044,#17040);
#11007=LINE('',#78045,#17041);
#11008=LINE('',#78057,#17042);
#11009=LINE('',#78072,#17043);
#11010=LINE('',#78087,#17044);
#11011=LINE('',#78093,#17045);
#11012=LINE('',#78095,#17046);
#11013=LINE('',#78096,#17047);
#11014=LINE('',#78099,#17048);
#11015=LINE('',#78101,#17049);
#11016=LINE('',#78102,#17050);
#11017=LINE('',#78105,#17051);
#11018=LINE('',#78107,#17052);
#11019=LINE('',#78108,#17053);
#11020=LINE('',#78110,#17054);
#11021=LINE('',#78111,#17055);
#11022=LINE('',#78126,#17056);
#11023=LINE('',#78131,#17057);
#11024=LINE('',#78143,#17058);
#11025=LINE('',#78158,#17059);
#11026=LINE('',#78173,#17060);
#11027=LINE('',#78188,#17061);
#11028=LINE('',#78203,#17062);
#11029=LINE('',#78218,#17063);
#11030=LINE('',#78246,#17064);
#11031=LINE('',#78251,#17065);
#11032=LINE('',#78263,#17066);
#11033=LINE('',#78278,#17067);
#11034=LINE('',#78293,#17068);
#11035=LINE('',#78308,#17069);
#11036=LINE('',#78323,#17070);
#11037=LINE('',#78338,#17071);
#11038=LINE('',#78353,#17072);
#11039=LINE('',#78368,#17073);
#11040=LINE('',#78383,#17074);
#11041=LINE('',#78398,#17075);
#11042=LINE('',#78427,#17076);
#11043=LINE('',#78432,#17077);
#11044=LINE('',#78444,#17078);
#11045=LINE('',#78459,#17079);
#11046=LINE('',#78474,#17080);
#11047=LINE('',#78489,#17081);
#11048=LINE('',#78504,#17082);
#11049=LINE('',#78519,#17083);
#11050=LINE('',#78534,#17084);
#11051=LINE('',#78562,#17085);
#11052=LINE('',#78567,#17086);
#11053=LINE('',#78579,#17087);
#11054=LINE('',#78594,#17088);
#11055=LINE('',#78609,#17089);
#11056=LINE('',#78624,#17090);
#11057=LINE('',#78639,#17091);
#11058=LINE('',#78654,#17092);
#11059=LINE('',#78669,#17093);
#11060=LINE('',#78684,#17094);
#11061=LINE('',#78699,#17095);
#11062=LINE('',#78714,#17096);
#11063=LINE('',#78729,#17097);
#11064=LINE('',#78744,#17098);
#11065=LINE('',#78759,#17099);
#11066=LINE('',#78774,#17100);
#11067=LINE('',#78789,#17101);
#11068=LINE('',#78804,#17102);
#11069=LINE('',#78810,#17103);
#11070=LINE('',#78812,#17104);
#11071=LINE('',#78813,#17105);
#11072=LINE('',#78841,#17106);
#11073=LINE('',#78846,#17107);
#11074=LINE('',#78858,#17108);
#11075=LINE('',#78873,#17109);
#11076=LINE('',#78888,#17110);
#11077=LINE('',#78903,#17111);
#11078=LINE('',#78918,#17112);
#11079=LINE('',#78933,#17113);
#11080=LINE('',#78961,#17114);
#11081=LINE('',#78966,#17115);
#11082=LINE('',#78978,#17116);
#11083=LINE('',#78993,#17117);
#11084=LINE('',#79008,#17118);
#11085=LINE('',#79023,#17119);
#11086=LINE('',#79038,#17120);
#11087=LINE('',#79053,#17121);
#11088=LINE('',#79068,#17122);
#11089=LINE('',#79083,#17123);
#11090=LINE('',#79098,#17124);
#11091=LINE('',#79113,#17125);
#11092=LINE('',#79142,#17126);
#11093=LINE('',#79147,#17127);
#11094=LINE('',#79159,#17128);
#11095=LINE('',#79174,#17129);
#11096=LINE('',#79189,#17130);
#11097=LINE('',#79204,#17131);
#11098=LINE('',#79219,#17132);
#11099=LINE('',#79225,#17133);
#11100=LINE('',#79227,#17134);
#11101=LINE('',#79228,#17135);
#11102=LINE('',#79231,#17136);
#11103=LINE('',#79233,#17137);
#11104=LINE('',#79234,#17138);
#11105=LINE('',#79237,#17139);
#11106=LINE('',#79239,#17140);
#11107=LINE('',#79240,#17141);
#11108=LINE('',#79243,#17142);
#11109=LINE('',#79245,#17143);
#11110=LINE('',#79246,#17144);
#11111=LINE('',#79249,#17145);
#11112=LINE('',#79251,#17146);
#11113=LINE('',#79252,#17147);
#11114=LINE('',#79255,#17148);
#11115=LINE('',#79257,#17149);
#11116=LINE('',#79258,#17150);
#11117=LINE('',#79270,#17151);
#11118=LINE('',#79285,#17152);
#11119=LINE('',#79300,#17153);
#11120=LINE('',#79315,#17154);
#11121=LINE('',#79330,#17155);
#11122=LINE('',#79345,#17156);
#11123=LINE('',#79360,#17157);
#11124=LINE('',#79375,#17158);
#11125=LINE('',#79381,#17159);
#11126=LINE('',#79383,#17160);
#11127=LINE('',#79384,#17161);
#11128=LINE('',#79411,#17162);
#11129=LINE('',#79416,#17163);
#11130=LINE('',#79428,#17164);
#11131=LINE('',#79443,#17165);
#11132=LINE('',#79458,#17166);
#11133=LINE('',#79473,#17167);
#11134=LINE('',#79488,#17168);
#11135=LINE('',#79503,#17169);
#11136=LINE('',#79531,#17170);
#11137=LINE('',#79536,#17171);
#11138=LINE('',#79548,#17172);
#11139=LINE('',#79563,#17173);
#11140=LINE('',#79578,#17174);
#11141=LINE('',#79593,#17175);
#11142=LINE('',#79608,#17176);
#11143=LINE('',#79623,#17177);
#11144=LINE('',#79638,#17178);
#11145=LINE('',#79653,#17179);
#11146=LINE('',#79668,#17180);
#11147=LINE('',#79683,#17181);
#11148=LINE('',#79703,#17182);
#11149=LINE('',#79705,#17183);
#11150=LINE('',#79707,#17184);
#11151=LINE('',#79708,#17185);
#11152=LINE('',#79711,#17186);
#11153=LINE('',#79713,#17187);
#11154=LINE('',#79714,#17188);
#11155=LINE('',#79716,#17189);
#11156=LINE('',#79717,#17190);
#11157=LINE('',#79721,#17191);
#11158=LINE('',#79723,#17192);
#11159=LINE('',#79725,#17193);
#11160=LINE('',#79726,#17194);
#11161=LINE('',#79729,#17195);
#11162=LINE('',#79731,#17196);
#11163=LINE('',#79732,#17197);
#11164=LINE('',#79735,#17198);
#11165=LINE('',#79737,#17199);
#11166=LINE('',#79738,#17200);
#11167=LINE('',#79741,#17201);
#11168=LINE('',#79743,#17202);
#11169=LINE('',#79744,#17203);
#11170=LINE('',#79747,#17204);
#11171=LINE('',#79749,#17205);
#11172=LINE('',#79750,#17206);
#11173=LINE('',#79753,#17207);
#11174=LINE('',#79755,#17208);
#11175=LINE('',#79756,#17209);
#11176=LINE('',#79759,#17210);
#11177=LINE('',#79761,#17211);
#11178=LINE('',#79762,#17212);
#11179=LINE('',#79765,#17213);
#11180=LINE('',#79767,#17214);
#11181=LINE('',#79768,#17215);
#11182=LINE('',#79771,#17216);
#11183=LINE('',#79773,#17217);
#11184=LINE('',#79774,#17218);
#11185=LINE('',#79777,#17219);
#11186=LINE('',#79779,#17220);
#11187=LINE('',#79780,#17221);
#11188=LINE('',#79782,#17222);
#11189=LINE('',#79783,#17223);
#11190=LINE('',#79799,#17224);
#11191=LINE('',#79804,#17225);
#11192=LINE('',#79816,#17226);
#11193=LINE('',#79831,#17227);
#11194=LINE('',#79846,#17228);
#11195=LINE('',#79861,#17229);
#11196=LINE('',#79876,#17230);
#11197=LINE('',#79891,#17231);
#11198=LINE('',#79919,#17232);
#11199=LINE('',#79924,#17233);
#11200=LINE('',#79936,#17234);
#11201=LINE('',#79951,#17235);
#11202=LINE('',#79966,#17236);
#11203=LINE('',#79981,#17237);
#11204=LINE('',#79996,#17238);
#11205=LINE('',#80011,#17239);
#11206=LINE('',#80026,#17240);
#11207=LINE('',#80041,#17241);
#11208=LINE('',#80056,#17242);
#11209=LINE('',#80071,#17243);
#11210=LINE('',#80100,#17244);
#11211=LINE('',#80105,#17245);
#11212=LINE('',#80117,#17246);
#11213=LINE('',#80132,#17247);
#11214=LINE('',#80147,#17248);
#11215=LINE('',#80162,#17249);
#11216=LINE('',#80177,#17250);
#11217=LINE('',#80192,#17251);
#11218=LINE('',#80207,#17252);
#11219=LINE('',#80222,#17253);
#11220=LINE('',#80237,#17254);
#11221=LINE('',#80252,#17255);
#11222=LINE('',#80267,#17256);
#11223=LINE('',#80273,#17257);
#11224=LINE('',#80275,#17258);
#11225=LINE('',#80276,#17259);
#11226=LINE('',#80288,#17260);
#11227=LINE('',#80303,#17261);
#11228=LINE('',#80318,#17262);
#11229=LINE('',#80333,#17263);
#11230=LINE('',#80348,#17264);
#11231=LINE('',#80363,#17265);
#11232=LINE('',#80378,#17266);
#11233=LINE('',#80384,#17267);
#11234=LINE('',#80386,#17268);
#11235=LINE('',#80387,#17269);
#11236=LINE('',#80399,#17270);
#11237=LINE('',#80414,#17271);
#11238=LINE('',#80429,#17272);
#11239=LINE('',#80444,#17273);
#11240=LINE('',#80459,#17274);
#11241=LINE('',#80474,#17275);
#11242=LINE('',#80489,#17276);
#11243=LINE('',#80495,#17277);
#11244=LINE('',#80497,#17278);
#11245=LINE('',#80498,#17279);
#11246=LINE('',#80525,#17280);
#11247=LINE('',#80530,#17281);
#11248=LINE('',#80542,#17282);
#11249=LINE('',#80557,#17283);
#11250=LINE('',#80572,#17284);
#11251=LINE('',#80587,#17285);
#11252=LINE('',#80602,#17286);
#11253=LINE('',#80617,#17287);
#11254=LINE('',#80645,#17288);
#11255=LINE('',#80650,#17289);
#11256=LINE('',#80662,#17290);
#11257=LINE('',#80677,#17291);
#11258=LINE('',#80692,#17292);
#11259=LINE('',#80707,#17293);
#11260=LINE('',#80722,#17294);
#11261=LINE('',#80737,#17295);
#11262=LINE('',#80752,#17296);
#11263=LINE('',#80767,#17297);
#11264=LINE('',#80782,#17298);
#11265=LINE('',#80797,#17299);
#11266=LINE('',#80826,#17300);
#11267=LINE('',#80831,#17301);
#11268=LINE('',#80843,#17302);
#11269=LINE('',#80858,#17303);
#11270=LINE('',#80873,#17304);
#11271=LINE('',#80888,#17305);
#11272=LINE('',#80903,#17306);
#11273=LINE('',#80918,#17307);
#11274=LINE('',#80933,#17308);
#11275=LINE('',#80948,#17309);
#11276=LINE('',#80954,#17310);
#11277=LINE('',#80956,#17311);
#11278=LINE('',#80957,#17312);
#11279=LINE('',#80969,#17313);
#11280=LINE('',#80984,#17314);
#11281=LINE('',#80999,#17315);
#11282=LINE('',#81014,#17316);
#11283=LINE('',#81029,#17317);
#11284=LINE('',#81044,#17318);
#11285=LINE('',#81059,#17319);
#11286=LINE('',#81074,#17320);
#11287=LINE('',#81089,#17321);
#11288=LINE('',#81095,#17322);
#11289=LINE('',#81097,#17323);
#11290=LINE('',#81098,#17324);
#11291=LINE('',#81101,#17325);
#11292=LINE('',#81103,#17326);
#11293=LINE('',#81104,#17327);
#11294=LINE('',#81106,#17328);
#11295=LINE('',#81107,#17329);
#11296=LINE('',#81122,#17330);
#11297=LINE('',#81127,#17331);
#11298=LINE('',#81139,#17332);
#11299=LINE('',#81154,#17333);
#11300=LINE('',#81169,#17334);
#11301=LINE('',#81184,#17335);
#11302=LINE('',#81199,#17336);
#11303=LINE('',#81214,#17337);
#11304=LINE('',#81242,#17338);
#11305=LINE('',#81247,#17339);
#11306=LINE('',#81259,#17340);
#11307=LINE('',#81274,#17341);
#11308=LINE('',#81289,#17342);
#11309=LINE('',#81304,#17343);
#11310=LINE('',#81319,#17344);
#11311=LINE('',#81334,#17345);
#11312=LINE('',#81349,#17346);
#11313=LINE('',#81364,#17347);
#11314=LINE('',#81379,#17348);
#11315=LINE('',#81394,#17349);
#11316=LINE('',#81414,#17350);
#11317=LINE('',#81416,#17351);
#11318=LINE('',#81418,#17352);
#11319=LINE('',#81419,#17353);
#11320=LINE('',#81431,#17354);
#11321=LINE('',#81446,#17355);
#11322=LINE('',#81452,#17356);
#11323=LINE('',#81454,#17357);
#11324=LINE('',#81455,#17358);
#11325=LINE('',#81467,#17359);
#11326=LINE('',#81482,#17360);
#11327=LINE('',#81488,#17361);
#11328=LINE('',#81490,#17362);
#11329=LINE('',#81491,#17363);
#11330=LINE('',#81494,#17364);
#11331=LINE('',#81496,#17365);
#11332=LINE('',#81497,#17366);
#11333=LINE('',#81499,#17367);
#11334=LINE('',#81500,#17368);
#11335=LINE('',#81515,#17369);
#11336=LINE('',#81520,#17370);
#11337=LINE('',#81532,#17371);
#11338=LINE('',#81547,#17372);
#11339=LINE('',#81562,#17373);
#11340=LINE('',#81577,#17374);
#11341=LINE('',#81592,#17375);
#11342=LINE('',#81607,#17376);
#11343=LINE('',#81635,#17377);
#11344=LINE('',#81640,#17378);
#11345=LINE('',#81652,#17379);
#11346=LINE('',#81667,#17380);
#11347=LINE('',#81682,#17381);
#11348=LINE('',#81697,#17382);
#11349=LINE('',#81712,#17383);
#11350=LINE('',#81727,#17384);
#11351=LINE('',#81742,#17385);
#11352=LINE('',#81757,#17386);
#11353=LINE('',#81772,#17387);
#11354=LINE('',#81787,#17388);
#11355=LINE('',#81817,#17389);
#11356=LINE('',#81822,#17390);
#11357=LINE('',#81834,#17391);
#11358=LINE('',#81849,#17392);
#11359=LINE('',#81864,#17393);
#11360=LINE('',#81879,#17394);
#11361=LINE('',#81894,#17395);
#11362=LINE('',#81909,#17396);
#11363=LINE('',#81937,#17397);
#11364=LINE('',#81942,#17398);
#11365=LINE('',#81954,#17399);
#11366=LINE('',#81969,#17400);
#11367=LINE('',#81984,#17401);
#11368=LINE('',#81999,#17402);
#11369=LINE('',#82014,#17403);
#11370=LINE('',#82029,#17404);
#11371=LINE('',#82044,#17405);
#11372=LINE('',#82059,#17406);
#11373=LINE('',#82074,#17407);
#11374=LINE('',#82089,#17408);
#11375=LINE('',#82109,#17409);
#11376=LINE('',#82111,#17410);
#11377=LINE('',#82113,#17411);
#11378=LINE('',#82114,#17412);
#11379=LINE('',#82126,#17413);
#11380=LINE('',#82141,#17414);
#11381=LINE('',#82147,#17415);
#11382=LINE('',#82149,#17416);
#11383=LINE('',#82150,#17417);
#11384=LINE('',#82162,#17418);
#11385=LINE('',#82177,#17419);
#11386=LINE('',#82183,#17420);
#11387=LINE('',#82185,#17421);
#11388=LINE('',#82186,#17422);
#11389=LINE('',#82189,#17423);
#11390=LINE('',#82191,#17424);
#11391=LINE('',#82192,#17425);
#11392=LINE('',#82194,#17426);
#11393=LINE('',#82195,#17427);
#11394=LINE('',#82210,#17428);
#11395=LINE('',#82215,#17429);
#11396=LINE('',#82227,#17430);
#11397=LINE('',#82242,#17431);
#11398=LINE('',#82257,#17432);
#11399=LINE('',#82272,#17433);
#11400=LINE('',#82287,#17434);
#11401=LINE('',#82302,#17435);
#11402=LINE('',#82330,#17436);
#11403=LINE('',#82335,#17437);
#11404=LINE('',#82347,#17438);
#11405=LINE('',#82362,#17439);
#11406=LINE('',#82377,#17440);
#11407=LINE('',#82392,#17441);
#11408=LINE('',#82407,#17442);
#11409=LINE('',#82422,#17443);
#11410=LINE('',#82437,#17444);
#11411=LINE('',#82452,#17445);
#11412=LINE('',#82467,#17446);
#11413=LINE('',#82482,#17447);
#11414=LINE('',#82511,#17448);
#11415=LINE('',#82516,#17449);
#11416=LINE('',#82528,#17450);
#11417=LINE('',#82543,#17451);
#11418=LINE('',#82558,#17452);
#11419=LINE('',#82573,#17453);
#11420=LINE('',#82588,#17454);
#11421=LINE('',#82603,#17455);
#11422=LINE('',#82618,#17456);
#11423=LINE('',#82633,#17457);
#11424=LINE('',#82639,#17458);
#11425=LINE('',#82641,#17459);
#11426=LINE('',#82642,#17460);
#11427=LINE('',#82654,#17461);
#11428=LINE('',#82669,#17462);
#11429=LINE('',#82684,#17463);
#11430=LINE('',#82699,#17464);
#11431=LINE('',#82714,#17465);
#11432=LINE('',#82729,#17466);
#11433=LINE('',#82744,#17467);
#11434=LINE('',#82759,#17468);
#11435=LINE('',#82774,#17469);
#11436=LINE('',#82780,#17470);
#11437=LINE('',#82782,#17471);
#11438=LINE('',#82783,#17472);
#11439=LINE('',#82786,#17473);
#11440=LINE('',#82788,#17474);
#11441=LINE('',#82789,#17475);
#11442=LINE('',#82791,#17476);
#11443=LINE('',#82792,#17477);
#11444=LINE('',#82807,#17478);
#11445=LINE('',#82812,#17479);
#11446=LINE('',#82824,#17480);
#11447=LINE('',#82839,#17481);
#11448=LINE('',#82854,#17482);
#11449=LINE('',#82869,#17483);
#11450=LINE('',#82884,#17484);
#11451=LINE('',#82899,#17485);
#11452=LINE('',#82927,#17486);
#11453=LINE('',#82932,#17487);
#11454=LINE('',#82944,#17488);
#11455=LINE('',#82959,#17489);
#11456=LINE('',#82974,#17490);
#11457=LINE('',#82989,#17491);
#11458=LINE('',#83004,#17492);
#11459=LINE('',#83019,#17493);
#11460=LINE('',#83034,#17494);
#11461=LINE('',#83049,#17495);
#11462=LINE('',#83064,#17496);
#11463=LINE('',#83079,#17497);
#11464=LINE('',#83108,#17498);
#11465=LINE('',#83113,#17499);
#11466=LINE('',#83125,#17500);
#11467=LINE('',#83140,#17501);
#11468=LINE('',#83155,#17502);
#11469=LINE('',#83170,#17503);
#11470=LINE('',#83185,#17504);
#11471=LINE('',#83200,#17505);
#11472=LINE('',#83215,#17506);
#11473=LINE('',#83230,#17507);
#11474=LINE('',#83245,#17508);
#11475=LINE('',#83260,#17509);
#11476=LINE('',#83275,#17510);
#11477=LINE('',#83281,#17511);
#11478=LINE('',#83283,#17512);
#11479=LINE('',#83284,#17513);
#11480=LINE('',#83296,#17514);
#11481=LINE('',#83311,#17515);
#11482=LINE('',#83326,#17516);
#11483=LINE('',#83341,#17517);
#11484=LINE('',#83356,#17518);
#11485=LINE('',#83371,#17519);
#11486=LINE('',#83386,#17520);
#11487=LINE('',#83392,#17521);
#11488=LINE('',#83394,#17522);
#11489=LINE('',#83395,#17523);
#11490=LINE('',#83407,#17524);
#11491=LINE('',#83422,#17525);
#11492=LINE('',#83437,#17526);
#11493=LINE('',#83452,#17527);
#11494=LINE('',#83467,#17528);
#11495=LINE('',#83482,#17529);
#11496=LINE('',#83497,#17530);
#11497=LINE('',#83503,#17531);
#11498=LINE('',#83505,#17532);
#11499=LINE('',#83506,#17533);
#11500=LINE('',#83533,#17534);
#11501=LINE('',#83538,#17535);
#11502=LINE('',#83550,#17536);
#11503=LINE('',#83565,#17537);
#11504=LINE('',#83580,#17538);
#11505=LINE('',#83595,#17539);
#11506=LINE('',#83610,#17540);
#11507=LINE('',#83625,#17541);
#11508=LINE('',#83653,#17542);
#11509=LINE('',#83658,#17543);
#11510=LINE('',#83670,#17544);
#11511=LINE('',#83685,#17545);
#11512=LINE('',#83700,#17546);
#11513=LINE('',#83715,#17547);
#11514=LINE('',#83730,#17548);
#11515=LINE('',#83745,#17549);
#11516=LINE('',#83760,#17550);
#11517=LINE('',#83775,#17551);
#11518=LINE('',#83790,#17552);
#11519=LINE('',#83805,#17553);
#11520=LINE('',#83825,#17554);
#11521=LINE('',#83827,#17555);
#11522=LINE('',#83829,#17556);
#11523=LINE('',#83830,#17557);
#11524=LINE('',#83833,#17558);
#11525=LINE('',#83835,#17559);
#11526=LINE('',#83836,#17560);
#11527=LINE('',#83838,#17561);
#11528=LINE('',#83839,#17562);
#11529=LINE('',#83843,#17563);
#11530=LINE('',#83845,#17564);
#11531=LINE('',#83847,#17565);
#11532=LINE('',#83848,#17566);
#11533=LINE('',#83851,#17567);
#11534=LINE('',#83853,#17568);
#11535=LINE('',#83854,#17569);
#11536=LINE('',#83857,#17570);
#11537=LINE('',#83859,#17571);
#11538=LINE('',#83860,#17572);
#11539=LINE('',#83863,#17573);
#11540=LINE('',#83865,#17574);
#11541=LINE('',#83866,#17575);
#11542=LINE('',#83869,#17576);
#11543=LINE('',#83871,#17577);
#11544=LINE('',#83872,#17578);
#11545=LINE('',#83875,#17579);
#11546=LINE('',#83877,#17580);
#11547=LINE('',#83878,#17581);
#11548=LINE('',#83881,#17582);
#11549=LINE('',#83883,#17583);
#11550=LINE('',#83884,#17584);
#11551=LINE('',#83887,#17585);
#11552=LINE('',#83889,#17586);
#11553=LINE('',#83890,#17587);
#11554=LINE('',#83893,#17588);
#11555=LINE('',#83895,#17589);
#11556=LINE('',#83896,#17590);
#11557=LINE('',#83899,#17591);
#11558=LINE('',#83901,#17592);
#11559=LINE('',#83902,#17593);
#11560=LINE('',#83904,#17594);
#11561=LINE('',#83905,#17595);
#11562=LINE('',#83921,#17596);
#11563=LINE('',#83926,#17597);
#11564=LINE('',#83938,#17598);
#11565=LINE('',#83953,#17599);
#11566=LINE('',#83968,#17600);
#11567=LINE('',#83983,#17601);
#11568=LINE('',#83998,#17602);
#11569=LINE('',#84013,#17603);
#11570=LINE('',#84041,#17604);
#11571=LINE('',#84046,#17605);
#11572=LINE('',#84058,#17606);
#11573=LINE('',#84073,#17607);
#11574=LINE('',#84088,#17608);
#11575=LINE('',#84103,#17609);
#11576=LINE('',#84118,#17610);
#11577=LINE('',#84133,#17611);
#11578=LINE('',#84148,#17612);
#11579=LINE('',#84163,#17613);
#11580=LINE('',#84178,#17614);
#11581=LINE('',#84193,#17615);
#11582=LINE('',#84222,#17616);
#11583=LINE('',#84227,#17617);
#11584=LINE('',#84239,#17618);
#11585=LINE('',#84254,#17619);
#11586=LINE('',#84269,#17620);
#11587=LINE('',#84284,#17621);
#11588=LINE('',#84299,#17622);
#11589=LINE('',#84305,#17623);
#11590=LINE('',#84307,#17624);
#11591=LINE('',#84308,#17625);
#11592=LINE('',#84311,#17626);
#11593=LINE('',#84313,#17627);
#11594=LINE('',#84314,#17628);
#11595=LINE('',#84317,#17629);
#11596=LINE('',#84319,#17630);
#11597=LINE('',#84320,#17631);
#11598=LINE('',#84323,#17632);
#11599=LINE('',#84325,#17633);
#11600=LINE('',#84326,#17634);
#11601=LINE('',#84329,#17635);
#11602=LINE('',#84331,#17636);
#11603=LINE('',#84332,#17637);
#11604=LINE('',#84335,#17638);
#11605=LINE('',#84337,#17639);
#11606=LINE('',#84338,#17640);
#11607=LINE('',#84350,#17641);
#11608=LINE('',#84365,#17642);
#11609=LINE('',#84380,#17643);
#11610=LINE('',#84395,#17644);
#11611=LINE('',#84410,#17645);
#11612=LINE('',#84425,#17646);
#11613=LINE('',#84440,#17647);
#11614=LINE('',#84455,#17648);
#11615=LINE('',#84461,#17649);
#11616=LINE('',#84463,#17650);
#11617=LINE('',#84464,#17651);
#11618=LINE('',#84491,#17652);
#11619=LINE('',#84496,#17653);
#11620=LINE('',#84508,#17654);
#11621=LINE('',#84523,#17655);
#11622=LINE('',#84538,#17656);
#11623=LINE('',#84553,#17657);
#11624=LINE('',#84568,#17658);
#11625=LINE('',#84583,#17659);
#11626=LINE('',#84611,#17660);
#11627=LINE('',#84616,#17661);
#11628=LINE('',#84628,#17662);
#11629=LINE('',#84643,#17663);
#11630=LINE('',#84658,#17664);
#11631=LINE('',#84673,#17665);
#11632=LINE('',#84688,#17666);
#11633=LINE('',#84703,#17667);
#11634=LINE('',#84718,#17668);
#11635=LINE('',#84733,#17669);
#11636=LINE('',#84748,#17670);
#11637=LINE('',#84763,#17671);
#11638=LINE('',#84792,#17672);
#11639=LINE('',#84797,#17673);
#11640=LINE('',#84809,#17674);
#11641=LINE('',#84824,#17675);
#11642=LINE('',#84839,#17676);
#11643=LINE('',#84854,#17677);
#11644=LINE('',#84869,#17678);
#11645=LINE('',#84884,#17679);
#11646=LINE('',#84899,#17680);
#11647=LINE('',#84927,#17681);
#11648=LINE('',#84932,#17682);
#11649=LINE('',#84944,#17683);
#11650=LINE('',#84959,#17684);
#11651=LINE('',#84974,#17685);
#11652=LINE('',#84989,#17686);
#11653=LINE('',#85004,#17687);
#11654=LINE('',#85019,#17688);
#11655=LINE('',#85034,#17689);
#11656=LINE('',#85049,#17690);
#11657=LINE('',#85064,#17691);
#11658=LINE('',#85079,#17692);
#11659=LINE('',#85094,#17693);
#11660=LINE('',#85109,#17694);
#11661=LINE('',#85124,#17695);
#11662=LINE('',#85139,#17696);
#11663=LINE('',#85154,#17697);
#11664=LINE('',#85169,#17698);
#11665=LINE('',#85175,#17699);
#11666=LINE('',#85177,#17700);
#11667=LINE('',#85178,#17701);
#11668=LINE('',#85206,#17702);
#11669=LINE('',#85211,#17703);
#11670=LINE('',#85223,#17704);
#11671=LINE('',#85238,#17705);
#11672=LINE('',#85253,#17706);
#11673=LINE('',#85268,#17707);
#11674=LINE('',#85283,#17708);
#11675=LINE('',#85298,#17709);
#11676=LINE('',#85326,#17710);
#11677=LINE('',#85331,#17711);
#11678=LINE('',#85343,#17712);
#11679=LINE('',#85358,#17713);
#11680=LINE('',#85373,#17714);
#11681=LINE('',#85388,#17715);
#11682=LINE('',#85403,#17716);
#11683=LINE('',#85418,#17717);
#11684=LINE('',#85433,#17718);
#11685=LINE('',#85448,#17719);
#11686=LINE('',#85463,#17720);
#11687=LINE('',#85478,#17721);
#11688=LINE('',#85507,#17722);
#11689=LINE('',#85512,#17723);
#11690=LINE('',#85524,#17724);
#11691=LINE('',#85539,#17725);
#11692=LINE('',#85545,#17726);
#11693=LINE('',#85547,#17727);
#11694=LINE('',#85548,#17728);
#11695=LINE('',#85560,#17729);
#11696=LINE('',#85575,#17730);
#11697=LINE('',#85590,#17731);
#11698=LINE('',#85596,#17732);
#11699=LINE('',#85598,#17733);
#11700=LINE('',#85599,#17734);
#11701=LINE('',#85602,#17735);
#11702=LINE('',#85604,#17736);
#11703=LINE('',#85605,#17737);
#11704=LINE('',#85608,#17738);
#11705=LINE('',#85610,#17739);
#11706=LINE('',#85611,#17740);
#11707=LINE('',#85613,#17741);
#11708=LINE('',#85614,#17742);
#11709=LINE('',#85629,#17743);
#11710=LINE('',#85634,#17744);
#11711=LINE('',#85646,#17745);
#11712=LINE('',#85661,#17746);
#11713=LINE('',#85676,#17747);
#11714=LINE('',#85691,#17748);
#11715=LINE('',#85706,#17749);
#11716=LINE('',#85721,#17750);
#11717=LINE('',#85749,#17751);
#11718=LINE('',#85754,#17752);
#11719=LINE('',#85766,#17753);
#11720=LINE('',#85781,#17754);
#11721=LINE('',#85796,#17755);
#11722=LINE('',#85811,#17756);
#11723=LINE('',#85826,#17757);
#11724=LINE('',#85841,#17758);
#11725=LINE('',#85856,#17759);
#11726=LINE('',#85871,#17760);
#11727=LINE('',#85886,#17761);
#11728=LINE('',#85901,#17762);
#11729=LINE('',#85930,#17763);
#11730=LINE('',#85935,#17764);
#11731=LINE('',#85947,#17765);
#11732=LINE('',#85962,#17766);
#11733=LINE('',#85977,#17767);
#11734=LINE('',#85992,#17768);
#11735=LINE('',#86007,#17769);
#11736=LINE('',#86022,#17770);
#11737=LINE('',#86050,#17771);
#11738=LINE('',#86055,#17772);
#11739=LINE('',#86067,#17773);
#11740=LINE('',#86082,#17774);
#11741=LINE('',#86097,#17775);
#11742=LINE('',#86112,#17776);
#11743=LINE('',#86127,#17777);
#11744=LINE('',#86142,#17778);
#11745=LINE('',#86157,#17779);
#11746=LINE('',#86185,#17780);
#11747=LINE('',#86190,#17781);
#11748=LINE('',#86202,#17782);
#11749=LINE('',#86217,#17783);
#11750=LINE('',#86232,#17784);
#11751=LINE('',#86247,#17785);
#11752=LINE('',#86262,#17786);
#11753=LINE('',#86277,#17787);
#11754=LINE('',#86292,#17788);
#11755=LINE('',#86307,#17789);
#11756=LINE('',#86322,#17790);
#11757=LINE('',#86337,#17791);
#11758=LINE('',#86352,#17792);
#11759=LINE('',#86367,#17793);
#11760=LINE('',#86382,#17794);
#11761=LINE('',#86397,#17795);
#11762=LINE('',#86429,#17796);
#11763=LINE('',#86434,#17797);
#11764=LINE('',#86446,#17798);
#11765=LINE('',#86461,#17799);
#11766=LINE('',#86476,#17800);
#11767=LINE('',#86491,#17801);
#11768=LINE('',#86506,#17802);
#11769=LINE('',#86521,#17803);
#11770=LINE('',#86549,#17804);
#11771=LINE('',#86554,#17805);
#11772=LINE('',#86566,#17806);
#11773=LINE('',#86581,#17807);
#11774=LINE('',#86596,#17808);
#11775=LINE('',#86611,#17809);
#11776=LINE('',#86626,#17810);
#11777=LINE('',#86641,#17811);
#11778=LINE('',#86656,#17812);
#11779=LINE('',#86671,#17813);
#11780=LINE('',#86686,#17814);
#11781=LINE('',#86701,#17815);
#11782=LINE('',#86730,#17816);
#11783=LINE('',#86735,#17817);
#11784=LINE('',#86747,#17818);
#11785=LINE('',#86762,#17819);
#11786=LINE('',#86777,#17820);
#11787=LINE('',#86792,#17821);
#11788=LINE('',#86807,#17822);
#11789=LINE('',#86822,#17823);
#11790=LINE('',#86850,#17824);
#11791=LINE('',#86855,#17825);
#11792=LINE('',#86867,#17826);
#11793=LINE('',#86882,#17827);
#11794=LINE('',#86897,#17828);
#11795=LINE('',#86912,#17829);
#11796=LINE('',#86927,#17830);
#11797=LINE('',#86942,#17831);
#11798=LINE('',#86957,#17832);
#11799=LINE('',#86972,#17833);
#11800=LINE('',#86987,#17834);
#11801=LINE('',#87002,#17835);
#11802=LINE('',#87017,#17836);
#11803=LINE('',#87032,#17837);
#11804=LINE('',#87047,#17838);
#11805=LINE('',#87062,#17839);
#11806=LINE('',#87077,#17840);
#11807=LINE('',#87092,#17841);
#11808=LINE('',#87107,#17842);
#11809=LINE('',#87122,#17843);
#11810=LINE('',#87137,#17844);
#11811=LINE('',#87143,#17845);
#11812=LINE('',#87145,#17846);
#11813=LINE('',#87146,#17847);
#11814=LINE('',#87165,#17848);
#11815=LINE('',#87167,#17849);
#11816=LINE('',#87169,#17850);
#11817=LINE('',#87170,#17851);
#11818=LINE('',#87173,#17852);
#11819=LINE('',#87175,#17853);
#11820=LINE('',#87176,#17854);
#11821=LINE('',#87179,#17855);
#11822=LINE('',#87181,#17856);
#11823=LINE('',#87182,#17857);
#11824=LINE('',#87184,#17858);
#11825=LINE('',#87185,#17859);
#11826=LINE('',#87190,#17860);
#11827=LINE('',#87192,#17861);
#11828=LINE('',#87194,#17862);
#11829=LINE('',#87195,#17863);
#11830=LINE('',#87198,#17864);
#11831=LINE('',#87200,#17865);
#11832=LINE('',#87201,#17866);
#11833=LINE('',#87204,#17867);
#11834=LINE('',#87206,#17868);
#11835=LINE('',#87207,#17869);
#11836=LINE('',#87209,#17870);
#11837=LINE('',#87210,#17871);
#11838=LINE('',#87215,#17872);
#11839=LINE('',#87217,#17873);
#11840=LINE('',#87219,#17874);
#11841=LINE('',#87220,#17875);
#11842=LINE('',#87223,#17876);
#11843=LINE('',#87225,#17877);
#11844=LINE('',#87226,#17878);
#11845=LINE('',#87229,#17879);
#11846=LINE('',#87231,#17880);
#11847=LINE('',#87232,#17881);
#11848=LINE('',#87234,#17882);
#11849=LINE('',#87235,#17883);
#11850=LINE('',#87240,#17884);
#11851=LINE('',#87242,#17885);
#11852=LINE('',#87244,#17886);
#11853=LINE('',#87245,#17887);
#11854=LINE('',#87248,#17888);
#11855=LINE('',#87250,#17889);
#11856=LINE('',#87251,#17890);
#11857=LINE('',#87254,#17891);
#11858=LINE('',#87256,#17892);
#11859=LINE('',#87257,#17893);
#11860=LINE('',#87259,#17894);
#11861=LINE('',#87260,#17895);
#11862=LINE('',#87265,#17896);
#11863=LINE('',#87267,#17897);
#11864=LINE('',#87269,#17898);
#11865=LINE('',#87270,#17899);
#11866=LINE('',#87273,#17900);
#11867=LINE('',#87275,#17901);
#11868=LINE('',#87276,#17902);
#11869=LINE('',#87279,#17903);
#11870=LINE('',#87281,#17904);
#11871=LINE('',#87282,#17905);
#11872=LINE('',#87284,#17906);
#11873=LINE('',#87285,#17907);
#11874=LINE('',#87290,#17908);
#11875=LINE('',#87292,#17909);
#11876=LINE('',#87294,#17910);
#11877=LINE('',#87295,#17911);
#11878=LINE('',#87298,#17912);
#11879=LINE('',#87300,#17913);
#11880=LINE('',#87301,#17914);
#11881=LINE('',#87304,#17915);
#11882=LINE('',#87306,#17916);
#11883=LINE('',#87307,#17917);
#11884=LINE('',#87309,#17918);
#11885=LINE('',#87310,#17919);
#11886=LINE('',#87315,#17920);
#11887=LINE('',#87317,#17921);
#11888=LINE('',#87319,#17922);
#11889=LINE('',#87320,#17923);
#11890=LINE('',#87323,#17924);
#11891=LINE('',#87325,#17925);
#11892=LINE('',#87326,#17926);
#11893=LINE('',#87329,#17927);
#11894=LINE('',#87331,#17928);
#11895=LINE('',#87332,#17929);
#11896=LINE('',#87334,#17930);
#11897=LINE('',#87335,#17931);
#11898=LINE('',#87340,#17932);
#11899=LINE('',#87342,#17933);
#11900=LINE('',#87344,#17934);
#11901=LINE('',#87345,#17935);
#11902=LINE('',#87348,#17936);
#11903=LINE('',#87350,#17937);
#11904=LINE('',#87351,#17938);
#11905=LINE('',#87354,#17939);
#11906=LINE('',#87356,#17940);
#11907=LINE('',#87357,#17941);
#11908=LINE('',#87359,#17942);
#11909=LINE('',#87360,#17943);
#11910=LINE('',#87365,#17944);
#11911=LINE('',#87367,#17945);
#11912=LINE('',#87369,#17946);
#11913=LINE('',#87370,#17947);
#11914=LINE('',#87373,#17948);
#11915=LINE('',#87375,#17949);
#11916=LINE('',#87376,#17950);
#11917=LINE('',#87379,#17951);
#11918=LINE('',#87381,#17952);
#11919=LINE('',#87382,#17953);
#11920=LINE('',#87384,#17954);
#11921=LINE('',#87385,#17955);
#11922=LINE('',#87390,#17956);
#11923=LINE('',#87392,#17957);
#11924=LINE('',#87394,#17958);
#11925=LINE('',#87395,#17959);
#11926=LINE('',#87398,#17960);
#11927=LINE('',#87400,#17961);
#11928=LINE('',#87401,#17962);
#11929=LINE('',#87404,#17963);
#11930=LINE('',#87406,#17964);
#11931=LINE('',#87407,#17965);
#11932=LINE('',#87409,#17966);
#11933=LINE('',#87410,#17967);
#11934=LINE('',#87415,#17968);
#11935=LINE('',#87417,#17969);
#11936=LINE('',#87419,#17970);
#11937=LINE('',#87420,#17971);
#11938=LINE('',#87423,#17972);
#11939=LINE('',#87425,#17973);
#11940=LINE('',#87426,#17974);
#11941=LINE('',#87429,#17975);
#11942=LINE('',#87431,#17976);
#11943=LINE('',#87432,#17977);
#11944=LINE('',#87434,#17978);
#11945=LINE('',#87435,#17979);
#11946=LINE('',#87440,#17980);
#11947=LINE('',#87442,#17981);
#11948=LINE('',#87444,#17982);
#11949=LINE('',#87445,#17983);
#11950=LINE('',#87448,#17984);
#11951=LINE('',#87450,#17985);
#11952=LINE('',#87451,#17986);
#11953=LINE('',#87454,#17987);
#11954=LINE('',#87456,#17988);
#11955=LINE('',#87457,#17989);
#11956=LINE('',#87459,#17990);
#11957=LINE('',#87460,#17991);
#11958=LINE('',#87465,#17992);
#11959=LINE('',#87467,#17993);
#11960=LINE('',#87469,#17994);
#11961=LINE('',#87470,#17995);
#11962=LINE('',#87473,#17996);
#11963=LINE('',#87475,#17997);
#11964=LINE('',#87476,#17998);
#11965=LINE('',#87479,#17999);
#11966=LINE('',#87481,#18000);
#11967=LINE('',#87482,#18001);
#11968=LINE('',#87484,#18002);
#11969=LINE('',#87485,#18003);
#11970=LINE('',#87490,#18004);
#11971=LINE('',#87492,#18005);
#11972=LINE('',#87494,#18006);
#11973=LINE('',#87495,#18007);
#11974=LINE('',#87498,#18008);
#11975=LINE('',#87500,#18009);
#11976=LINE('',#87501,#18010);
#11977=LINE('',#87504,#18011);
#11978=LINE('',#87506,#18012);
#11979=LINE('',#87507,#18013);
#11980=LINE('',#87509,#18014);
#11981=LINE('',#87510,#18015);
#11982=LINE('',#87515,#18016);
#11983=LINE('',#87517,#18017);
#11984=LINE('',#87519,#18018);
#11985=LINE('',#87520,#18019);
#11986=LINE('',#87523,#18020);
#11987=LINE('',#87525,#18021);
#11988=LINE('',#87526,#18022);
#11989=LINE('',#87529,#18023);
#11990=LINE('',#87531,#18024);
#11991=LINE('',#87532,#18025);
#11992=LINE('',#87534,#18026);
#11993=LINE('',#87535,#18027);
#11994=LINE('',#87540,#18028);
#11995=LINE('',#87542,#18029);
#11996=LINE('',#87544,#18030);
#11997=LINE('',#87545,#18031);
#11998=LINE('',#87548,#18032);
#11999=LINE('',#87550,#18033);
#12000=LINE('',#87551,#18034);
#12001=LINE('',#87554,#18035);
#12002=LINE('',#87556,#18036);
#12003=LINE('',#87557,#18037);
#12004=LINE('',#87559,#18038);
#12005=LINE('',#87560,#18039);
#12006=LINE('',#87565,#18040);
#12007=LINE('',#87567,#18041);
#12008=LINE('',#87569,#18042);
#12009=LINE('',#87570,#18043);
#12010=LINE('',#87573,#18044);
#12011=LINE('',#87575,#18045);
#12012=LINE('',#87576,#18046);
#12013=LINE('',#87579,#18047);
#12014=LINE('',#87581,#18048);
#12015=LINE('',#87582,#18049);
#12016=LINE('',#87584,#18050);
#12017=LINE('',#87585,#18051);
#12018=LINE('',#87590,#18052);
#12019=LINE('',#87592,#18053);
#12020=LINE('',#87594,#18054);
#12021=LINE('',#87595,#18055);
#12022=LINE('',#87598,#18056);
#12023=LINE('',#87600,#18057);
#12024=LINE('',#87601,#18058);
#12025=LINE('',#87604,#18059);
#12026=LINE('',#87606,#18060);
#12027=LINE('',#87607,#18061);
#12028=LINE('',#87609,#18062);
#12029=LINE('',#87610,#18063);
#12030=LINE('',#87615,#18064);
#12031=LINE('',#87617,#18065);
#12032=LINE('',#87619,#18066);
#12033=LINE('',#87620,#18067);
#12034=LINE('',#87623,#18068);
#12035=LINE('',#87625,#18069);
#12036=LINE('',#87626,#18070);
#12037=LINE('',#87629,#18071);
#12038=LINE('',#87631,#18072);
#12039=LINE('',#87632,#18073);
#12040=LINE('',#87634,#18074);
#12041=LINE('',#87635,#18075);
#12042=LINE('',#87640,#18076);
#12043=LINE('',#87642,#18077);
#12044=LINE('',#87644,#18078);
#12045=LINE('',#87645,#18079);
#12046=LINE('',#87648,#18080);
#12047=LINE('',#87650,#18081);
#12048=LINE('',#87651,#18082);
#12049=LINE('',#87654,#18083);
#12050=LINE('',#87656,#18084);
#12051=LINE('',#87657,#18085);
#12052=LINE('',#87659,#18086);
#12053=LINE('',#87660,#18087);
#12054=LINE('',#87665,#18088);
#12055=LINE('',#87667,#18089);
#12056=LINE('',#87669,#18090);
#12057=LINE('',#87670,#18091);
#12058=LINE('',#87673,#18092);
#12059=LINE('',#87675,#18093);
#12060=LINE('',#87676,#18094);
#12061=LINE('',#87679,#18095);
#12062=LINE('',#87681,#18096);
#12063=LINE('',#87682,#18097);
#12064=LINE('',#87684,#18098);
#12065=LINE('',#87685,#18099);
#12066=LINE('',#87690,#18100);
#12067=LINE('',#87692,#18101);
#12068=LINE('',#87694,#18102);
#12069=LINE('',#87695,#18103);
#12070=LINE('',#87698,#18104);
#12071=LINE('',#87700,#18105);
#12072=LINE('',#87701,#18106);
#12073=LINE('',#87704,#18107);
#12074=LINE('',#87706,#18108);
#12075=LINE('',#87707,#18109);
#12076=LINE('',#87709,#18110);
#12077=LINE('',#87710,#18111);
#12078=LINE('',#87715,#18112);
#12079=LINE('',#87717,#18113);
#12080=LINE('',#87719,#18114);
#12081=LINE('',#87720,#18115);
#12082=LINE('',#87723,#18116);
#12083=LINE('',#87725,#18117);
#12084=LINE('',#87726,#18118);
#12085=LINE('',#87729,#18119);
#12086=LINE('',#87731,#18120);
#12087=LINE('',#87732,#18121);
#12088=LINE('',#87734,#18122);
#12089=LINE('',#87735,#18123);
#12090=LINE('',#87740,#18124);
#12091=LINE('',#87742,#18125);
#12092=LINE('',#87744,#18126);
#12093=LINE('',#87745,#18127);
#12094=LINE('',#87748,#18128);
#12095=LINE('',#87750,#18129);
#12096=LINE('',#87751,#18130);
#12097=LINE('',#87754,#18131);
#12098=LINE('',#87756,#18132);
#12099=LINE('',#87757,#18133);
#12100=LINE('',#87759,#18134);
#12101=LINE('',#87760,#18135);
#12102=LINE('',#87765,#18136);
#12103=LINE('',#87767,#18137);
#12104=LINE('',#87769,#18138);
#12105=LINE('',#87770,#18139);
#12106=LINE('',#87773,#18140);
#12107=LINE('',#87775,#18141);
#12108=LINE('',#87776,#18142);
#12109=LINE('',#87779,#18143);
#12110=LINE('',#87781,#18144);
#12111=LINE('',#87782,#18145);
#12112=LINE('',#87784,#18146);
#12113=LINE('',#87785,#18147);
#12114=LINE('',#87790,#18148);
#12115=LINE('',#87792,#18149);
#12116=LINE('',#87794,#18150);
#12117=LINE('',#87795,#18151);
#12118=LINE('',#87798,#18152);
#12119=LINE('',#87800,#18153);
#12120=LINE('',#87801,#18154);
#12121=LINE('',#87804,#18155);
#12122=LINE('',#87806,#18156);
#12123=LINE('',#87807,#18157);
#12124=LINE('',#87809,#18158);
#12125=LINE('',#87810,#18159);
#12126=LINE('',#87815,#18160);
#12127=LINE('',#87817,#18161);
#12128=LINE('',#87819,#18162);
#12129=LINE('',#87820,#18163);
#12130=LINE('',#87823,#18164);
#12131=LINE('',#87825,#18165);
#12132=LINE('',#87826,#18166);
#12133=LINE('',#87829,#18167);
#12134=LINE('',#87831,#18168);
#12135=LINE('',#87832,#18169);
#12136=LINE('',#87834,#18170);
#12137=LINE('',#87835,#18171);
#12138=LINE('',#87840,#18172);
#12139=LINE('',#87842,#18173);
#12140=LINE('',#87844,#18174);
#12141=LINE('',#87845,#18175);
#12142=LINE('',#87848,#18176);
#12143=LINE('',#87850,#18177);
#12144=LINE('',#87851,#18178);
#12145=LINE('',#87854,#18179);
#12146=LINE('',#87856,#18180);
#12147=LINE('',#87857,#18181);
#12148=LINE('',#87859,#18182);
#12149=LINE('',#87860,#18183);
#12150=LINE('',#87865,#18184);
#12151=LINE('',#87867,#18185);
#12152=LINE('',#87869,#18186);
#12153=LINE('',#87870,#18187);
#12154=LINE('',#87873,#18188);
#12155=LINE('',#87875,#18189);
#12156=LINE('',#87876,#18190);
#12157=LINE('',#87879,#18191);
#12158=LINE('',#87881,#18192);
#12159=LINE('',#87882,#18193);
#12160=LINE('',#87884,#18194);
#12161=LINE('',#87885,#18195);
#12162=LINE('',#87890,#18196);
#12163=LINE('',#87892,#18197);
#12164=LINE('',#87894,#18198);
#12165=LINE('',#87895,#18199);
#12166=LINE('',#87898,#18200);
#12167=LINE('',#87900,#18201);
#12168=LINE('',#87901,#18202);
#12169=LINE('',#87904,#18203);
#12170=LINE('',#87906,#18204);
#12171=LINE('',#87907,#18205);
#12172=LINE('',#87909,#18206);
#12173=LINE('',#87910,#18207);
#12174=LINE('',#87915,#18208);
#12175=LINE('',#87917,#18209);
#12176=LINE('',#87919,#18210);
#12177=LINE('',#87920,#18211);
#12178=LINE('',#87923,#18212);
#12179=LINE('',#87925,#18213);
#12180=LINE('',#87926,#18214);
#12181=LINE('',#87929,#18215);
#12182=LINE('',#87931,#18216);
#12183=LINE('',#87932,#18217);
#12184=LINE('',#87934,#18218);
#12185=LINE('',#87935,#18219);
#12186=LINE('',#87940,#18220);
#12187=LINE('',#87942,#18221);
#12188=LINE('',#87944,#18222);
#12189=LINE('',#87945,#18223);
#12190=LINE('',#87948,#18224);
#12191=LINE('',#87950,#18225);
#12192=LINE('',#87951,#18226);
#12193=LINE('',#87954,#18227);
#12194=LINE('',#87956,#18228);
#12195=LINE('',#87957,#18229);
#12196=LINE('',#87959,#18230);
#12197=LINE('',#87960,#18231);
#12198=LINE('',#87965,#18232);
#12199=LINE('',#87967,#18233);
#12200=LINE('',#87969,#18234);
#12201=LINE('',#87970,#18235);
#12202=LINE('',#87973,#18236);
#12203=LINE('',#87975,#18237);
#12204=LINE('',#87976,#18238);
#12205=LINE('',#87979,#18239);
#12206=LINE('',#87981,#18240);
#12207=LINE('',#87982,#18241);
#12208=LINE('',#87984,#18242);
#12209=LINE('',#87985,#18243);
#12210=LINE('',#87990,#18244);
#12211=LINE('',#87992,#18245);
#12212=LINE('',#87994,#18246);
#12213=LINE('',#87995,#18247);
#12214=LINE('',#87998,#18248);
#12215=LINE('',#88000,#18249);
#12216=LINE('',#88001,#18250);
#12217=LINE('',#88004,#18251);
#12218=LINE('',#88006,#18252);
#12219=LINE('',#88007,#18253);
#12220=LINE('',#88009,#18254);
#12221=LINE('',#88010,#18255);
#12222=LINE('',#88015,#18256);
#12223=LINE('',#88017,#18257);
#12224=LINE('',#88019,#18258);
#12225=LINE('',#88020,#18259);
#12226=LINE('',#88023,#18260);
#12227=LINE('',#88025,#18261);
#12228=LINE('',#88026,#18262);
#12229=LINE('',#88029,#18263);
#12230=LINE('',#88031,#18264);
#12231=LINE('',#88032,#18265);
#12232=LINE('',#88034,#18266);
#12233=LINE('',#88035,#18267);
#12234=LINE('',#88040,#18268);
#12235=LINE('',#88042,#18269);
#12236=LINE('',#88044,#18270);
#12237=LINE('',#88045,#18271);
#12238=LINE('',#88048,#18272);
#12239=LINE('',#88050,#18273);
#12240=LINE('',#88051,#18274);
#12241=LINE('',#88054,#18275);
#12242=LINE('',#88056,#18276);
#12243=LINE('',#88057,#18277);
#12244=LINE('',#88059,#18278);
#12245=LINE('',#88060,#18279);
#12246=LINE('',#88065,#18280);
#12247=LINE('',#88067,#18281);
#12248=LINE('',#88069,#18282);
#12249=LINE('',#88070,#18283);
#12250=LINE('',#88073,#18284);
#12251=LINE('',#88075,#18285);
#12252=LINE('',#88076,#18286);
#12253=LINE('',#88079,#18287);
#12254=LINE('',#88081,#18288);
#12255=LINE('',#88082,#18289);
#12256=LINE('',#88084,#18290);
#12257=LINE('',#88085,#18291);
#12258=LINE('',#88090,#18292);
#12259=LINE('',#88092,#18293);
#12260=LINE('',#88094,#18294);
#12261=LINE('',#88095,#18295);
#12262=LINE('',#88098,#18296);
#12263=LINE('',#88100,#18297);
#12264=LINE('',#88101,#18298);
#12265=LINE('',#88104,#18299);
#12266=LINE('',#88106,#18300);
#12267=LINE('',#88107,#18301);
#12268=LINE('',#88109,#18302);
#12269=LINE('',#88110,#18303);
#12270=LINE('',#88115,#18304);
#12271=LINE('',#88117,#18305);
#12272=LINE('',#88119,#18306);
#12273=LINE('',#88120,#18307);
#12274=LINE('',#88123,#18308);
#12275=LINE('',#88125,#18309);
#12276=LINE('',#88126,#18310);
#12277=LINE('',#88129,#18311);
#12278=LINE('',#88131,#18312);
#12279=LINE('',#88132,#18313);
#12280=LINE('',#88134,#18314);
#12281=LINE('',#88135,#18315);
#12282=LINE('',#88140,#18316);
#12283=LINE('',#88142,#18317);
#12284=LINE('',#88144,#18318);
#12285=LINE('',#88145,#18319);
#12286=LINE('',#88148,#18320);
#12287=LINE('',#88150,#18321);
#12288=LINE('',#88151,#18322);
#12289=LINE('',#88154,#18323);
#12290=LINE('',#88156,#18324);
#12291=LINE('',#88157,#18325);
#12292=LINE('',#88159,#18326);
#12293=LINE('',#88160,#18327);
#12294=LINE('',#88165,#18328);
#12295=LINE('',#88167,#18329);
#12296=LINE('',#88169,#18330);
#12297=LINE('',#88170,#18331);
#12298=LINE('',#88173,#18332);
#12299=LINE('',#88175,#18333);
#12300=LINE('',#88176,#18334);
#12301=LINE('',#88179,#18335);
#12302=LINE('',#88181,#18336);
#12303=LINE('',#88182,#18337);
#12304=LINE('',#88184,#18338);
#12305=LINE('',#88185,#18339);
#12306=LINE('',#88190,#18340);
#12307=LINE('',#88192,#18341);
#12308=LINE('',#88194,#18342);
#12309=LINE('',#88195,#18343);
#12310=LINE('',#88198,#18344);
#12311=LINE('',#88200,#18345);
#12312=LINE('',#88201,#18346);
#12313=LINE('',#88204,#18347);
#12314=LINE('',#88206,#18348);
#12315=LINE('',#88207,#18349);
#12316=LINE('',#88209,#18350);
#12317=LINE('',#88210,#18351);
#12318=LINE('',#88215,#18352);
#12319=LINE('',#88217,#18353);
#12320=LINE('',#88219,#18354);
#12321=LINE('',#88220,#18355);
#12322=LINE('',#88223,#18356);
#12323=LINE('',#88225,#18357);
#12324=LINE('',#88226,#18358);
#12325=LINE('',#88229,#18359);
#12326=LINE('',#88231,#18360);
#12327=LINE('',#88232,#18361);
#12328=LINE('',#88234,#18362);
#12329=LINE('',#88235,#18363);
#12330=LINE('',#88240,#18364);
#12331=LINE('',#88242,#18365);
#12332=LINE('',#88244,#18366);
#12333=LINE('',#88245,#18367);
#12334=LINE('',#88248,#18368);
#12335=LINE('',#88250,#18369);
#12336=LINE('',#88251,#18370);
#12337=LINE('',#88254,#18371);
#12338=LINE('',#88256,#18372);
#12339=LINE('',#88257,#18373);
#12340=LINE('',#88259,#18374);
#12341=LINE('',#88260,#18375);
#12342=LINE('',#88265,#18376);
#12343=LINE('',#88267,#18377);
#12344=LINE('',#88269,#18378);
#12345=LINE('',#88270,#18379);
#12346=LINE('',#88273,#18380);
#12347=LINE('',#88275,#18381);
#12348=LINE('',#88276,#18382);
#12349=LINE('',#88279,#18383);
#12350=LINE('',#88281,#18384);
#12351=LINE('',#88282,#18385);
#12352=LINE('',#88284,#18386);
#12353=LINE('',#88285,#18387);
#12354=LINE('',#88290,#18388);
#12355=LINE('',#88292,#18389);
#12356=LINE('',#88294,#18390);
#12357=LINE('',#88295,#18391);
#12358=LINE('',#88298,#18392);
#12359=LINE('',#88300,#18393);
#12360=LINE('',#88301,#18394);
#12361=LINE('',#88304,#18395);
#12362=LINE('',#88306,#18396);
#12363=LINE('',#88307,#18397);
#12364=LINE('',#88309,#18398);
#12365=LINE('',#88310,#18399);
#12366=LINE('',#88315,#18400);
#12367=LINE('',#88317,#18401);
#12368=LINE('',#88319,#18402);
#12369=LINE('',#88320,#18403);
#12370=LINE('',#88323,#18404);
#12371=LINE('',#88325,#18405);
#12372=LINE('',#88326,#18406);
#12373=LINE('',#88329,#18407);
#12374=LINE('',#88331,#18408);
#12375=LINE('',#88332,#18409);
#12376=LINE('',#88334,#18410);
#12377=LINE('',#88335,#18411);
#12378=LINE('',#88340,#18412);
#12379=LINE('',#88342,#18413);
#12380=LINE('',#88344,#18414);
#12381=LINE('',#88345,#18415);
#12382=LINE('',#88348,#18416);
#12383=LINE('',#88350,#18417);
#12384=LINE('',#88351,#18418);
#12385=LINE('',#88354,#18419);
#12386=LINE('',#88356,#18420);
#12387=LINE('',#88357,#18421);
#12388=LINE('',#88359,#18422);
#12389=LINE('',#88360,#18423);
#12390=LINE('',#88365,#18424);
#12391=LINE('',#88367,#18425);
#12392=LINE('',#88369,#18426);
#12393=LINE('',#88370,#18427);
#12394=LINE('',#88373,#18428);
#12395=LINE('',#88375,#18429);
#12396=LINE('',#88376,#18430);
#12397=LINE('',#88379,#18431);
#12398=LINE('',#88381,#18432);
#12399=LINE('',#88382,#18433);
#12400=LINE('',#88384,#18434);
#12401=LINE('',#88385,#18435);
#12402=LINE('',#88390,#18436);
#12403=LINE('',#88392,#18437);
#12404=LINE('',#88394,#18438);
#12405=LINE('',#88395,#18439);
#12406=LINE('',#88398,#18440);
#12407=LINE('',#88400,#18441);
#12408=LINE('',#88401,#18442);
#12409=LINE('',#88404,#18443);
#12410=LINE('',#88406,#18444);
#12411=LINE('',#88407,#18445);
#12412=LINE('',#88409,#18446);
#12413=LINE('',#88410,#18447);
#12414=LINE('',#88415,#18448);
#12415=LINE('',#88417,#18449);
#12416=LINE('',#88419,#18450);
#12417=LINE('',#88420,#18451);
#12418=LINE('',#88423,#18452);
#12419=LINE('',#88425,#18453);
#12420=LINE('',#88426,#18454);
#12421=LINE('',#88429,#18455);
#12422=LINE('',#88431,#18456);
#12423=LINE('',#88432,#18457);
#12424=LINE('',#88434,#18458);
#12425=LINE('',#88435,#18459);
#12426=LINE('',#88440,#18460);
#12427=LINE('',#88442,#18461);
#12428=LINE('',#88444,#18462);
#12429=LINE('',#88445,#18463);
#12430=LINE('',#88448,#18464);
#12431=LINE('',#88450,#18465);
#12432=LINE('',#88451,#18466);
#12433=LINE('',#88454,#18467);
#12434=LINE('',#88456,#18468);
#12435=LINE('',#88457,#18469);
#12436=LINE('',#88459,#18470);
#12437=LINE('',#88460,#18471);
#12438=LINE('',#88465,#18472);
#12439=LINE('',#88467,#18473);
#12440=LINE('',#88469,#18474);
#12441=LINE('',#88470,#18475);
#12442=LINE('',#88473,#18476);
#12443=LINE('',#88475,#18477);
#12444=LINE('',#88476,#18478);
#12445=LINE('',#88479,#18479);
#12446=LINE('',#88481,#18480);
#12447=LINE('',#88482,#18481);
#12448=LINE('',#88484,#18482);
#12449=LINE('',#88485,#18483);
#12450=LINE('',#88490,#18484);
#12451=LINE('',#88492,#18485);
#12452=LINE('',#88494,#18486);
#12453=LINE('',#88495,#18487);
#12454=LINE('',#88498,#18488);
#12455=LINE('',#88500,#18489);
#12456=LINE('',#88501,#18490);
#12457=LINE('',#88504,#18491);
#12458=LINE('',#88506,#18492);
#12459=LINE('',#88507,#18493);
#12460=LINE('',#88509,#18494);
#12461=LINE('',#88510,#18495);
#12462=LINE('',#88515,#18496);
#12463=LINE('',#88517,#18497);
#12464=LINE('',#88519,#18498);
#12465=LINE('',#88520,#18499);
#12466=LINE('',#88523,#18500);
#12467=LINE('',#88525,#18501);
#12468=LINE('',#88526,#18502);
#12469=LINE('',#88529,#18503);
#12470=LINE('',#88531,#18504);
#12471=LINE('',#88532,#18505);
#12472=LINE('',#88534,#18506);
#12473=LINE('',#88535,#18507);
#12474=LINE('',#88540,#18508);
#12475=LINE('',#88542,#18509);
#12476=LINE('',#88544,#18510);
#12477=LINE('',#88545,#18511);
#12478=LINE('',#88548,#18512);
#12479=LINE('',#88550,#18513);
#12480=LINE('',#88551,#18514);
#12481=LINE('',#88554,#18515);
#12482=LINE('',#88556,#18516);
#12483=LINE('',#88557,#18517);
#12484=LINE('',#88559,#18518);
#12485=LINE('',#88560,#18519);
#12486=LINE('',#88565,#18520);
#12487=LINE('',#88567,#18521);
#12488=LINE('',#88569,#18522);
#12489=LINE('',#88570,#18523);
#12490=LINE('',#88573,#18524);
#12491=LINE('',#88575,#18525);
#12492=LINE('',#88576,#18526);
#12493=LINE('',#88579,#18527);
#12494=LINE('',#88581,#18528);
#12495=LINE('',#88582,#18529);
#12496=LINE('',#88584,#18530);
#12497=LINE('',#88585,#18531);
#12498=LINE('',#88590,#18532);
#12499=LINE('',#88592,#18533);
#12500=LINE('',#88594,#18534);
#12501=LINE('',#88595,#18535);
#12502=LINE('',#88598,#18536);
#12503=LINE('',#88600,#18537);
#12504=LINE('',#88601,#18538);
#12505=LINE('',#88604,#18539);
#12506=LINE('',#88606,#18540);
#12507=LINE('',#88607,#18541);
#12508=LINE('',#88609,#18542);
#12509=LINE('',#88610,#18543);
#12510=LINE('',#88615,#18544);
#12511=LINE('',#88617,#18545);
#12512=LINE('',#88619,#18546);
#12513=LINE('',#88620,#18547);
#12514=LINE('',#88623,#18548);
#12515=LINE('',#88625,#18549);
#12516=LINE('',#88626,#18550);
#12517=LINE('',#88629,#18551);
#12518=LINE('',#88631,#18552);
#12519=LINE('',#88632,#18553);
#12520=LINE('',#88634,#18554);
#12521=LINE('',#88635,#18555);
#12522=LINE('',#88640,#18556);
#12523=LINE('',#88642,#18557);
#12524=LINE('',#88644,#18558);
#12525=LINE('',#88645,#18559);
#12526=LINE('',#88648,#18560);
#12527=LINE('',#88650,#18561);
#12528=LINE('',#88651,#18562);
#12529=LINE('',#88654,#18563);
#12530=LINE('',#88656,#18564);
#12531=LINE('',#88657,#18565);
#12532=LINE('',#88659,#18566);
#12533=LINE('',#88660,#18567);
#12534=LINE('',#88665,#18568);
#12535=LINE('',#88667,#18569);
#12536=LINE('',#88669,#18570);
#12537=LINE('',#88670,#18571);
#12538=LINE('',#88673,#18572);
#12539=LINE('',#88675,#18573);
#12540=LINE('',#88676,#18574);
#12541=LINE('',#88679,#18575);
#12542=LINE('',#88681,#18576);
#12543=LINE('',#88682,#18577);
#12544=LINE('',#88684,#18578);
#12545=LINE('',#88685,#18579);
#12546=LINE('',#88690,#18580);
#12547=LINE('',#88692,#18581);
#12548=LINE('',#88694,#18582);
#12549=LINE('',#88695,#18583);
#12550=LINE('',#88698,#18584);
#12551=LINE('',#88700,#18585);
#12552=LINE('',#88701,#18586);
#12553=LINE('',#88704,#18587);
#12554=LINE('',#88706,#18588);
#12555=LINE('',#88707,#18589);
#12556=LINE('',#88709,#18590);
#12557=LINE('',#88710,#18591);
#12558=LINE('',#88715,#18592);
#12559=LINE('',#88717,#18593);
#12560=LINE('',#88719,#18594);
#12561=LINE('',#88720,#18595);
#12562=LINE('',#88723,#18596);
#12563=LINE('',#88725,#18597);
#12564=LINE('',#88726,#18598);
#12565=LINE('',#88729,#18599);
#12566=LINE('',#88731,#18600);
#12567=LINE('',#88732,#18601);
#12568=LINE('',#88734,#18602);
#12569=LINE('',#88735,#18603);
#12570=LINE('',#88740,#18604);
#12571=LINE('',#88742,#18605);
#12572=LINE('',#88744,#18606);
#12573=LINE('',#88745,#18607);
#12574=LINE('',#88748,#18608);
#12575=LINE('',#88750,#18609);
#12576=LINE('',#88751,#18610);
#12577=LINE('',#88754,#18611);
#12578=LINE('',#88756,#18612);
#12579=LINE('',#88757,#18613);
#12580=LINE('',#88759,#18614);
#12581=LINE('',#88760,#18615);
#12582=LINE('',#88765,#18616);
#12583=LINE('',#88767,#18617);
#12584=LINE('',#88769,#18618);
#12585=LINE('',#88770,#18619);
#12586=LINE('',#88773,#18620);
#12587=LINE('',#88775,#18621);
#12588=LINE('',#88776,#18622);
#12589=LINE('',#88779,#18623);
#12590=LINE('',#88781,#18624);
#12591=LINE('',#88782,#18625);
#12592=LINE('',#88784,#18626);
#12593=LINE('',#88785,#18627);
#12594=LINE('',#88790,#18628);
#12595=LINE('',#88792,#18629);
#12596=LINE('',#88794,#18630);
#12597=LINE('',#88795,#18631);
#12598=LINE('',#88798,#18632);
#12599=LINE('',#88800,#18633);
#12600=LINE('',#88801,#18634);
#12601=LINE('',#88804,#18635);
#12602=LINE('',#88806,#18636);
#12603=LINE('',#88807,#18637);
#12604=LINE('',#88809,#18638);
#12605=LINE('',#88810,#18639);
#12606=LINE('',#88815,#18640);
#12607=LINE('',#88817,#18641);
#12608=LINE('',#88819,#18642);
#12609=LINE('',#88820,#18643);
#12610=LINE('',#88823,#18644);
#12611=LINE('',#88825,#18645);
#12612=LINE('',#88826,#18646);
#12613=LINE('',#88829,#18647);
#12614=LINE('',#88831,#18648);
#12615=LINE('',#88832,#18649);
#12616=LINE('',#88834,#18650);
#12617=LINE('',#88835,#18651);
#12618=LINE('',#88840,#18652);
#12619=LINE('',#88842,#18653);
#12620=LINE('',#88844,#18654);
#12621=LINE('',#88845,#18655);
#12622=LINE('',#88848,#18656);
#12623=LINE('',#88850,#18657);
#12624=LINE('',#88851,#18658);
#12625=LINE('',#88854,#18659);
#12626=LINE('',#88856,#18660);
#12627=LINE('',#88857,#18661);
#12628=LINE('',#88859,#18662);
#12629=LINE('',#88860,#18663);
#12630=LINE('',#88865,#18664);
#12631=LINE('',#88867,#18665);
#12632=LINE('',#88869,#18666);
#12633=LINE('',#88870,#18667);
#12634=LINE('',#88873,#18668);
#12635=LINE('',#88875,#18669);
#12636=LINE('',#88876,#18670);
#12637=LINE('',#88879,#18671);
#12638=LINE('',#88881,#18672);
#12639=LINE('',#88882,#18673);
#12640=LINE('',#88884,#18674);
#12641=LINE('',#88885,#18675);
#12642=LINE('',#88890,#18676);
#12643=LINE('',#88892,#18677);
#12644=LINE('',#88894,#18678);
#12645=LINE('',#88895,#18679);
#12646=LINE('',#88898,#18680);
#12647=LINE('',#88900,#18681);
#12648=LINE('',#88901,#18682);
#12649=LINE('',#88904,#18683);
#12650=LINE('',#88906,#18684);
#12651=LINE('',#88907,#18685);
#12652=LINE('',#88909,#18686);
#12653=LINE('',#88910,#18687);
#12654=LINE('',#88915,#18688);
#12655=LINE('',#88917,#18689);
#12656=LINE('',#88919,#18690);
#12657=LINE('',#88920,#18691);
#12658=LINE('',#88923,#18692);
#12659=LINE('',#88925,#18693);
#12660=LINE('',#88926,#18694);
#12661=LINE('',#88929,#18695);
#12662=LINE('',#88931,#18696);
#12663=LINE('',#88932,#18697);
#12664=LINE('',#88934,#18698);
#12665=LINE('',#88935,#18699);
#12666=LINE('',#88940,#18700);
#12667=LINE('',#88942,#18701);
#12668=LINE('',#88944,#18702);
#12669=LINE('',#88945,#18703);
#12670=LINE('',#88948,#18704);
#12671=LINE('',#88950,#18705);
#12672=LINE('',#88951,#18706);
#12673=LINE('',#88954,#18707);
#12674=LINE('',#88956,#18708);
#12675=LINE('',#88957,#18709);
#12676=LINE('',#88959,#18710);
#12677=LINE('',#88960,#18711);
#12678=LINE('',#88965,#18712);
#12679=LINE('',#88967,#18713);
#12680=LINE('',#88969,#18714);
#12681=LINE('',#88970,#18715);
#12682=LINE('',#88973,#18716);
#12683=LINE('',#88975,#18717);
#12684=LINE('',#88976,#18718);
#12685=LINE('',#88979,#18719);
#12686=LINE('',#88981,#18720);
#12687=LINE('',#88982,#18721);
#12688=LINE('',#88984,#18722);
#12689=LINE('',#88985,#18723);
#12690=LINE('',#88990,#18724);
#12691=LINE('',#88992,#18725);
#12692=LINE('',#88994,#18726);
#12693=LINE('',#88995,#18727);
#12694=LINE('',#88998,#18728);
#12695=LINE('',#89000,#18729);
#12696=LINE('',#89001,#18730);
#12697=LINE('',#89004,#18731);
#12698=LINE('',#89006,#18732);
#12699=LINE('',#89007,#18733);
#12700=LINE('',#89009,#18734);
#12701=LINE('',#89010,#18735);
#12702=LINE('',#89015,#18736);
#12703=LINE('',#89017,#18737);
#12704=LINE('',#89019,#18738);
#12705=LINE('',#89020,#18739);
#12706=LINE('',#89023,#18740);
#12707=LINE('',#89025,#18741);
#12708=LINE('',#89026,#18742);
#12709=LINE('',#89029,#18743);
#12710=LINE('',#89031,#18744);
#12711=LINE('',#89032,#18745);
#12712=LINE('',#89034,#18746);
#12713=LINE('',#89035,#18747);
#12714=LINE('',#89040,#18748);
#12715=LINE('',#89042,#18749);
#12716=LINE('',#89044,#18750);
#12717=LINE('',#89045,#18751);
#12718=LINE('',#89048,#18752);
#12719=LINE('',#89050,#18753);
#12720=LINE('',#89051,#18754);
#12721=LINE('',#89054,#18755);
#12722=LINE('',#89056,#18756);
#12723=LINE('',#89057,#18757);
#12724=LINE('',#89059,#18758);
#12725=LINE('',#89060,#18759);
#12726=LINE('',#89065,#18760);
#12727=LINE('',#89067,#18761);
#12728=LINE('',#89069,#18762);
#12729=LINE('',#89070,#18763);
#12730=LINE('',#89073,#18764);
#12731=LINE('',#89075,#18765);
#12732=LINE('',#89076,#18766);
#12733=LINE('',#89079,#18767);
#12734=LINE('',#89081,#18768);
#12735=LINE('',#89082,#18769);
#12736=LINE('',#89084,#18770);
#12737=LINE('',#89085,#18771);
#12738=LINE('',#89090,#18772);
#12739=LINE('',#89092,#18773);
#12740=LINE('',#89094,#18774);
#12741=LINE('',#89095,#18775);
#12742=LINE('',#89098,#18776);
#12743=LINE('',#89100,#18777);
#12744=LINE('',#89101,#18778);
#12745=LINE('',#89104,#18779);
#12746=LINE('',#89106,#18780);
#12747=LINE('',#89107,#18781);
#12748=LINE('',#89109,#18782);
#12749=LINE('',#89110,#18783);
#12750=LINE('',#89115,#18784);
#12751=LINE('',#89117,#18785);
#12752=LINE('',#89119,#18786);
#12753=LINE('',#89120,#18787);
#12754=LINE('',#89123,#18788);
#12755=LINE('',#89125,#18789);
#12756=LINE('',#89126,#18790);
#12757=LINE('',#89129,#18791);
#12758=LINE('',#89131,#18792);
#12759=LINE('',#89132,#18793);
#12760=LINE('',#89134,#18794);
#12761=LINE('',#89135,#18795);
#12762=LINE('',#89140,#18796);
#12763=LINE('',#89142,#18797);
#12764=LINE('',#89144,#18798);
#12765=LINE('',#89145,#18799);
#12766=LINE('',#89148,#18800);
#12767=LINE('',#89150,#18801);
#12768=LINE('',#89151,#18802);
#12769=LINE('',#89154,#18803);
#12770=LINE('',#89156,#18804);
#12771=LINE('',#89157,#18805);
#12772=LINE('',#89159,#18806);
#12773=LINE('',#89160,#18807);
#12774=LINE('',#89165,#18808);
#12775=LINE('',#89167,#18809);
#12776=LINE('',#89169,#18810);
#12777=LINE('',#89170,#18811);
#12778=LINE('',#89173,#18812);
#12779=LINE('',#89175,#18813);
#12780=LINE('',#89176,#18814);
#12781=LINE('',#89179,#18815);
#12782=LINE('',#89181,#18816);
#12783=LINE('',#89182,#18817);
#12784=LINE('',#89184,#18818);
#12785=LINE('',#89185,#18819);
#12786=LINE('',#89190,#18820);
#12787=LINE('',#89192,#18821);
#12788=LINE('',#89194,#18822);
#12789=LINE('',#89195,#18823);
#12790=LINE('',#89198,#18824);
#12791=LINE('',#89200,#18825);
#12792=LINE('',#89201,#18826);
#12793=LINE('',#89204,#18827);
#12794=LINE('',#89206,#18828);
#12795=LINE('',#89207,#18829);
#12796=LINE('',#89209,#18830);
#12797=LINE('',#89210,#18831);
#12798=LINE('',#89215,#18832);
#12799=LINE('',#89217,#18833);
#12800=LINE('',#89219,#18834);
#12801=LINE('',#89220,#18835);
#12802=LINE('',#89223,#18836);
#12803=LINE('',#89225,#18837);
#12804=LINE('',#89226,#18838);
#12805=LINE('',#89229,#18839);
#12806=LINE('',#89231,#18840);
#12807=LINE('',#89232,#18841);
#12808=LINE('',#89234,#18842);
#12809=LINE('',#89235,#18843);
#12810=LINE('',#89240,#18844);
#12811=LINE('',#89242,#18845);
#12812=LINE('',#89244,#18846);
#12813=LINE('',#89245,#18847);
#12814=LINE('',#89248,#18848);
#12815=LINE('',#89250,#18849);
#12816=LINE('',#89251,#18850);
#12817=LINE('',#89254,#18851);
#12818=LINE('',#89256,#18852);
#12819=LINE('',#89257,#18853);
#12820=LINE('',#89259,#18854);
#12821=LINE('',#89260,#18855);
#12822=LINE('',#89265,#18856);
#12823=LINE('',#89267,#18857);
#12824=LINE('',#89269,#18858);
#12825=LINE('',#89270,#18859);
#12826=LINE('',#89273,#18860);
#12827=LINE('',#89275,#18861);
#12828=LINE('',#89276,#18862);
#12829=LINE('',#89279,#18863);
#12830=LINE('',#89281,#18864);
#12831=LINE('',#89282,#18865);
#12832=LINE('',#89284,#18866);
#12833=LINE('',#89285,#18867);
#12834=LINE('',#89290,#18868);
#12835=LINE('',#89292,#18869);
#12836=LINE('',#89294,#18870);
#12837=LINE('',#89295,#18871);
#12838=LINE('',#89298,#18872);
#12839=LINE('',#89300,#18873);
#12840=LINE('',#89301,#18874);
#12841=LINE('',#89304,#18875);
#12842=LINE('',#89306,#18876);
#12843=LINE('',#89307,#18877);
#12844=LINE('',#89309,#18878);
#12845=LINE('',#89310,#18879);
#12846=LINE('',#89315,#18880);
#12847=LINE('',#89317,#18881);
#12848=LINE('',#89319,#18882);
#12849=LINE('',#89320,#18883);
#12850=LINE('',#89323,#18884);
#12851=LINE('',#89325,#18885);
#12852=LINE('',#89326,#18886);
#12853=LINE('',#89329,#18887);
#12854=LINE('',#89331,#18888);
#12855=LINE('',#89332,#18889);
#12856=LINE('',#89334,#18890);
#12857=LINE('',#89335,#18891);
#12858=LINE('',#89340,#18892);
#12859=LINE('',#89342,#18893);
#12860=LINE('',#89344,#18894);
#12861=LINE('',#89345,#18895);
#12862=LINE('',#89348,#18896);
#12863=LINE('',#89350,#18897);
#12864=LINE('',#89351,#18898);
#12865=LINE('',#89354,#18899);
#12866=LINE('',#89356,#18900);
#12867=LINE('',#89357,#18901);
#12868=LINE('',#89359,#18902);
#12869=LINE('',#89360,#18903);
#12870=LINE('',#89365,#18904);
#12871=LINE('',#89367,#18905);
#12872=LINE('',#89369,#18906);
#12873=LINE('',#89370,#18907);
#12874=LINE('',#89373,#18908);
#12875=LINE('',#89375,#18909);
#12876=LINE('',#89376,#18910);
#12877=LINE('',#89379,#18911);
#12878=LINE('',#89381,#18912);
#12879=LINE('',#89382,#18913);
#12880=LINE('',#89384,#18914);
#12881=LINE('',#89385,#18915);
#12882=LINE('',#89390,#18916);
#12883=LINE('',#89392,#18917);
#12884=LINE('',#89394,#18918);
#12885=LINE('',#89395,#18919);
#12886=LINE('',#89398,#18920);
#12887=LINE('',#89400,#18921);
#12888=LINE('',#89401,#18922);
#12889=LINE('',#89404,#18923);
#12890=LINE('',#89406,#18924);
#12891=LINE('',#89407,#18925);
#12892=LINE('',#89409,#18926);
#12893=LINE('',#89410,#18927);
#12894=LINE('',#89415,#18928);
#12895=LINE('',#89417,#18929);
#12896=LINE('',#89419,#18930);
#12897=LINE('',#89420,#18931);
#12898=LINE('',#89423,#18932);
#12899=LINE('',#89425,#18933);
#12900=LINE('',#89426,#18934);
#12901=LINE('',#89429,#18935);
#12902=LINE('',#89431,#18936);
#12903=LINE('',#89432,#18937);
#12904=LINE('',#89434,#18938);
#12905=LINE('',#89435,#18939);
#12906=LINE('',#89440,#18940);
#12907=LINE('',#89442,#18941);
#12908=LINE('',#89444,#18942);
#12909=LINE('',#89445,#18943);
#12910=LINE('',#89448,#18944);
#12911=LINE('',#89450,#18945);
#12912=LINE('',#89451,#18946);
#12913=LINE('',#89454,#18947);
#12914=LINE('',#89456,#18948);
#12915=LINE('',#89457,#18949);
#12916=LINE('',#89459,#18950);
#12917=LINE('',#89460,#18951);
#12918=LINE('',#89465,#18952);
#12919=LINE('',#89467,#18953);
#12920=LINE('',#89469,#18954);
#12921=LINE('',#89470,#18955);
#12922=LINE('',#89473,#18956);
#12923=LINE('',#89475,#18957);
#12924=LINE('',#89476,#18958);
#12925=LINE('',#89479,#18959);
#12926=LINE('',#89481,#18960);
#12927=LINE('',#89482,#18961);
#12928=LINE('',#89484,#18962);
#12929=LINE('',#89485,#18963);
#12930=LINE('',#89490,#18964);
#12931=LINE('',#89492,#18965);
#12932=LINE('',#89494,#18966);
#12933=LINE('',#89495,#18967);
#12934=LINE('',#89498,#18968);
#12935=LINE('',#89500,#18969);
#12936=LINE('',#89501,#18970);
#12937=LINE('',#89504,#18971);
#12938=LINE('',#89506,#18972);
#12939=LINE('',#89507,#18973);
#12940=LINE('',#89509,#18974);
#12941=LINE('',#89510,#18975);
#12942=LINE('',#89515,#18976);
#12943=LINE('',#89517,#18977);
#12944=LINE('',#89519,#18978);
#12945=LINE('',#89520,#18979);
#12946=LINE('',#89523,#18980);
#12947=LINE('',#89525,#18981);
#12948=LINE('',#89526,#18982);
#12949=LINE('',#89529,#18983);
#12950=LINE('',#89531,#18984);
#12951=LINE('',#89532,#18985);
#12952=LINE('',#89534,#18986);
#12953=LINE('',#89535,#18987);
#12954=LINE('',#89540,#18988);
#12955=LINE('',#89542,#18989);
#12956=LINE('',#89544,#18990);
#12957=LINE('',#89545,#18991);
#12958=LINE('',#89548,#18992);
#12959=LINE('',#89550,#18993);
#12960=LINE('',#89551,#18994);
#12961=LINE('',#89554,#18995);
#12962=LINE('',#89556,#18996);
#12963=LINE('',#89557,#18997);
#12964=LINE('',#89559,#18998);
#12965=LINE('',#89560,#18999);
#12966=LINE('',#89565,#19000);
#12967=LINE('',#89567,#19001);
#12968=LINE('',#89569,#19002);
#12969=LINE('',#89570,#19003);
#12970=LINE('',#89573,#19004);
#12971=LINE('',#89575,#19005);
#12972=LINE('',#89576,#19006);
#12973=LINE('',#89579,#19007);
#12974=LINE('',#89581,#19008);
#12975=LINE('',#89582,#19009);
#12976=LINE('',#89584,#19010);
#12977=LINE('',#89585,#19011);
#12978=LINE('',#89590,#19012);
#12979=LINE('',#89592,#19013);
#12980=LINE('',#89594,#19014);
#12981=LINE('',#89595,#19015);
#12982=LINE('',#89598,#19016);
#12983=LINE('',#89600,#19017);
#12984=LINE('',#89601,#19018);
#12985=LINE('',#89604,#19019);
#12986=LINE('',#89606,#19020);
#12987=LINE('',#89607,#19021);
#12988=LINE('',#89609,#19022);
#12989=LINE('',#89610,#19023);
#12990=LINE('',#89615,#19024);
#12991=LINE('',#89617,#19025);
#12992=LINE('',#89619,#19026);
#12993=LINE('',#89620,#19027);
#12994=LINE('',#89623,#19028);
#12995=LINE('',#89625,#19029);
#12996=LINE('',#89626,#19030);
#12997=LINE('',#89629,#19031);
#12998=LINE('',#89631,#19032);
#12999=LINE('',#89632,#19033);
#13000=LINE('',#89634,#19034);
#13001=LINE('',#89635,#19035);
#13002=LINE('',#89640,#19036);
#13003=LINE('',#89642,#19037);
#13004=LINE('',#89644,#19038);
#13005=LINE('',#89645,#19039);
#13006=LINE('',#89648,#19040);
#13007=LINE('',#89650,#19041);
#13008=LINE('',#89651,#19042);
#13009=LINE('',#89654,#19043);
#13010=LINE('',#89656,#19044);
#13011=LINE('',#89657,#19045);
#13012=LINE('',#89659,#19046);
#13013=LINE('',#89660,#19047);
#13014=LINE('',#89665,#19048);
#13015=LINE('',#89667,#19049);
#13016=LINE('',#89669,#19050);
#13017=LINE('',#89670,#19051);
#13018=LINE('',#89673,#19052);
#13019=LINE('',#89675,#19053);
#13020=LINE('',#89676,#19054);
#13021=LINE('',#89679,#19055);
#13022=LINE('',#89681,#19056);
#13023=LINE('',#89682,#19057);
#13024=LINE('',#89684,#19058);
#13025=LINE('',#89685,#19059);
#13026=LINE('',#89690,#19060);
#13027=LINE('',#89692,#19061);
#13028=LINE('',#89694,#19062);
#13029=LINE('',#89695,#19063);
#13030=LINE('',#89698,#19064);
#13031=LINE('',#89700,#19065);
#13032=LINE('',#89701,#19066);
#13033=LINE('',#89704,#19067);
#13034=LINE('',#89706,#19068);
#13035=LINE('',#89707,#19069);
#13036=LINE('',#89709,#19070);
#13037=LINE('',#89710,#19071);
#13038=LINE('',#89715,#19072);
#13039=LINE('',#89717,#19073);
#13040=LINE('',#89719,#19074);
#13041=LINE('',#89720,#19075);
#13042=LINE('',#89723,#19076);
#13043=LINE('',#89725,#19077);
#13044=LINE('',#89726,#19078);
#13045=LINE('',#89729,#19079);
#13046=LINE('',#89731,#19080);
#13047=LINE('',#89732,#19081);
#13048=LINE('',#89734,#19082);
#13049=LINE('',#89735,#19083);
#13050=LINE('',#89740,#19084);
#13051=LINE('',#89742,#19085);
#13052=LINE('',#89744,#19086);
#13053=LINE('',#89745,#19087);
#13054=LINE('',#89748,#19088);
#13055=LINE('',#89750,#19089);
#13056=LINE('',#89751,#19090);
#13057=LINE('',#89754,#19091);
#13058=LINE('',#89756,#19092);
#13059=LINE('',#89757,#19093);
#13060=LINE('',#89759,#19094);
#13061=LINE('',#89760,#19095);
#13062=LINE('',#89765,#19096);
#13063=LINE('',#89767,#19097);
#13064=LINE('',#89769,#19098);
#13065=LINE('',#89770,#19099);
#13066=LINE('',#89773,#19100);
#13067=LINE('',#89775,#19101);
#13068=LINE('',#89776,#19102);
#13069=LINE('',#89779,#19103);
#13070=LINE('',#89781,#19104);
#13071=LINE('',#89782,#19105);
#13072=LINE('',#89784,#19106);
#13073=LINE('',#89785,#19107);
#13074=LINE('',#89790,#19108);
#13075=LINE('',#89792,#19109);
#13076=LINE('',#89794,#19110);
#13077=LINE('',#89795,#19111);
#13078=LINE('',#89798,#19112);
#13079=LINE('',#89800,#19113);
#13080=LINE('',#89801,#19114);
#13081=LINE('',#89804,#19115);
#13082=LINE('',#89806,#19116);
#13083=LINE('',#89807,#19117);
#13084=LINE('',#89809,#19118);
#13085=LINE('',#89810,#19119);
#13086=LINE('',#89815,#19120);
#13087=LINE('',#89817,#19121);
#13088=LINE('',#89819,#19122);
#13089=LINE('',#89820,#19123);
#13090=LINE('',#89823,#19124);
#13091=LINE('',#89825,#19125);
#13092=LINE('',#89826,#19126);
#13093=LINE('',#89829,#19127);
#13094=LINE('',#89831,#19128);
#13095=LINE('',#89832,#19129);
#13096=LINE('',#89834,#19130);
#13097=LINE('',#89835,#19131);
#13098=LINE('',#89840,#19132);
#13099=LINE('',#89842,#19133);
#13100=LINE('',#89844,#19134);
#13101=LINE('',#89845,#19135);
#13102=LINE('',#89848,#19136);
#13103=LINE('',#89850,#19137);
#13104=LINE('',#89851,#19138);
#13105=LINE('',#89854,#19139);
#13106=LINE('',#89856,#19140);
#13107=LINE('',#89857,#19141);
#13108=LINE('',#89859,#19142);
#13109=LINE('',#89860,#19143);
#13110=LINE('',#89865,#19144);
#13111=LINE('',#89867,#19145);
#13112=LINE('',#89869,#19146);
#13113=LINE('',#89870,#19147);
#13114=LINE('',#89873,#19148);
#13115=LINE('',#89875,#19149);
#13116=LINE('',#89876,#19150);
#13117=LINE('',#89879,#19151);
#13118=LINE('',#89881,#19152);
#13119=LINE('',#89882,#19153);
#13120=LINE('',#89884,#19154);
#13121=LINE('',#89885,#19155);
#13122=LINE('',#89890,#19156);
#13123=LINE('',#89892,#19157);
#13124=LINE('',#89894,#19158);
#13125=LINE('',#89895,#19159);
#13126=LINE('',#89898,#19160);
#13127=LINE('',#89900,#19161);
#13128=LINE('',#89901,#19162);
#13129=LINE('',#89904,#19163);
#13130=LINE('',#89906,#19164);
#13131=LINE('',#89907,#19165);
#13132=LINE('',#89909,#19166);
#13133=LINE('',#89910,#19167);
#13134=LINE('',#89915,#19168);
#13135=LINE('',#89917,#19169);
#13136=LINE('',#89919,#19170);
#13137=LINE('',#89920,#19171);
#13138=LINE('',#89923,#19172);
#13139=LINE('',#89925,#19173);
#13140=LINE('',#89926,#19174);
#13141=LINE('',#89929,#19175);
#13142=LINE('',#89931,#19176);
#13143=LINE('',#89932,#19177);
#13144=LINE('',#89934,#19178);
#13145=LINE('',#89935,#19179);
#13146=LINE('',#89940,#19180);
#13147=LINE('',#89942,#19181);
#13148=LINE('',#89944,#19182);
#13149=LINE('',#89945,#19183);
#13150=LINE('',#89948,#19184);
#13151=LINE('',#89950,#19185);
#13152=LINE('',#89951,#19186);
#13153=LINE('',#89954,#19187);
#13154=LINE('',#89956,#19188);
#13155=LINE('',#89957,#19189);
#13156=LINE('',#89959,#19190);
#13157=LINE('',#89960,#19191);
#13158=LINE('',#89965,#19192);
#13159=LINE('',#89967,#19193);
#13160=LINE('',#89969,#19194);
#13161=LINE('',#89970,#19195);
#13162=LINE('',#89973,#19196);
#13163=LINE('',#89975,#19197);
#13164=LINE('',#89976,#19198);
#13165=LINE('',#89979,#19199);
#13166=LINE('',#89981,#19200);
#13167=LINE('',#89982,#19201);
#13168=LINE('',#89984,#19202);
#13169=LINE('',#89985,#19203);
#13170=LINE('',#89990,#19204);
#13171=LINE('',#89992,#19205);
#13172=LINE('',#89994,#19206);
#13173=LINE('',#89995,#19207);
#13174=LINE('',#89998,#19208);
#13175=LINE('',#90000,#19209);
#13176=LINE('',#90001,#19210);
#13177=LINE('',#90004,#19211);
#13178=LINE('',#90006,#19212);
#13179=LINE('',#90007,#19213);
#13180=LINE('',#90009,#19214);
#13181=LINE('',#90010,#19215);
#13182=LINE('',#90015,#19216);
#13183=LINE('',#90017,#19217);
#13184=LINE('',#90019,#19218);
#13185=LINE('',#90020,#19219);
#13186=LINE('',#90023,#19220);
#13187=LINE('',#90025,#19221);
#13188=LINE('',#90026,#19222);
#13189=LINE('',#90029,#19223);
#13190=LINE('',#90031,#19224);
#13191=LINE('',#90032,#19225);
#13192=LINE('',#90034,#19226);
#13193=LINE('',#90035,#19227);
#13194=LINE('',#90040,#19228);
#13195=LINE('',#90042,#19229);
#13196=LINE('',#90044,#19230);
#13197=LINE('',#90045,#19231);
#13198=LINE('',#90048,#19232);
#13199=LINE('',#90050,#19233);
#13200=LINE('',#90051,#19234);
#13201=LINE('',#90054,#19235);
#13202=LINE('',#90056,#19236);
#13203=LINE('',#90057,#19237);
#13204=LINE('',#90059,#19238);
#13205=LINE('',#90060,#19239);
#13206=LINE('',#90065,#19240);
#13207=LINE('',#90067,#19241);
#13208=LINE('',#90069,#19242);
#13209=LINE('',#90070,#19243);
#13210=LINE('',#90073,#19244);
#13211=LINE('',#90075,#19245);
#13212=LINE('',#90076,#19246);
#13213=LINE('',#90079,#19247);
#13214=LINE('',#90081,#19248);
#13215=LINE('',#90082,#19249);
#13216=LINE('',#90084,#19250);
#13217=LINE('',#90085,#19251);
#13218=LINE('',#90090,#19252);
#13219=LINE('',#90092,#19253);
#13220=LINE('',#90094,#19254);
#13221=LINE('',#90095,#19255);
#13222=LINE('',#90098,#19256);
#13223=LINE('',#90100,#19257);
#13224=LINE('',#90101,#19258);
#13225=LINE('',#90104,#19259);
#13226=LINE('',#90106,#19260);
#13227=LINE('',#90107,#19261);
#13228=LINE('',#90109,#19262);
#13229=LINE('',#90110,#19263);
#13230=LINE('',#90115,#19264);
#13231=LINE('',#90117,#19265);
#13232=LINE('',#90119,#19266);
#13233=LINE('',#90120,#19267);
#13234=LINE('',#90123,#19268);
#13235=LINE('',#90125,#19269);
#13236=LINE('',#90126,#19270);
#13237=LINE('',#90129,#19271);
#13238=LINE('',#90131,#19272);
#13239=LINE('',#90132,#19273);
#13240=LINE('',#90134,#19274);
#13241=LINE('',#90135,#19275);
#13242=LINE('',#90140,#19276);
#13243=LINE('',#90142,#19277);
#13244=LINE('',#90144,#19278);
#13245=LINE('',#90145,#19279);
#13246=LINE('',#90148,#19280);
#13247=LINE('',#90150,#19281);
#13248=LINE('',#90151,#19282);
#13249=LINE('',#90154,#19283);
#13250=LINE('',#90156,#19284);
#13251=LINE('',#90157,#19285);
#13252=LINE('',#90159,#19286);
#13253=LINE('',#90160,#19287);
#13254=LINE('',#90165,#19288);
#13255=LINE('',#90167,#19289);
#13256=LINE('',#90169,#19290);
#13257=LINE('',#90170,#19291);
#13258=LINE('',#90173,#19292);
#13259=LINE('',#90175,#19293);
#13260=LINE('',#90176,#19294);
#13261=LINE('',#90179,#19295);
#13262=LINE('',#90181,#19296);
#13263=LINE('',#90182,#19297);
#13264=LINE('',#90184,#19298);
#13265=LINE('',#90185,#19299);
#13266=LINE('',#90190,#19300);
#13267=LINE('',#90192,#19301);
#13268=LINE('',#90194,#19302);
#13269=LINE('',#90195,#19303);
#13270=LINE('',#90198,#19304);
#13271=LINE('',#90200,#19305);
#13272=LINE('',#90201,#19306);
#13273=LINE('',#90204,#19307);
#13274=LINE('',#90206,#19308);
#13275=LINE('',#90207,#19309);
#13276=LINE('',#90209,#19310);
#13277=LINE('',#90210,#19311);
#13278=LINE('',#90215,#19312);
#13279=LINE('',#90217,#19313);
#13280=LINE('',#90219,#19314);
#13281=LINE('',#90220,#19315);
#13282=LINE('',#90223,#19316);
#13283=LINE('',#90225,#19317);
#13284=LINE('',#90226,#19318);
#13285=LINE('',#90229,#19319);
#13286=LINE('',#90231,#19320);
#13287=LINE('',#90232,#19321);
#13288=LINE('',#90234,#19322);
#13289=LINE('',#90235,#19323);
#13290=LINE('',#90240,#19324);
#13291=LINE('',#90242,#19325);
#13292=LINE('',#90244,#19326);
#13293=LINE('',#90245,#19327);
#13294=LINE('',#90248,#19328);
#13295=LINE('',#90250,#19329);
#13296=LINE('',#90251,#19330);
#13297=LINE('',#90254,#19331);
#13298=LINE('',#90256,#19332);
#13299=LINE('',#90257,#19333);
#13300=LINE('',#90259,#19334);
#13301=LINE('',#90260,#19335);
#13302=LINE('',#90265,#19336);
#13303=LINE('',#90267,#19337);
#13304=LINE('',#90269,#19338);
#13305=LINE('',#90270,#19339);
#13306=LINE('',#90273,#19340);
#13307=LINE('',#90275,#19341);
#13308=LINE('',#90276,#19342);
#13309=LINE('',#90279,#19343);
#13310=LINE('',#90281,#19344);
#13311=LINE('',#90282,#19345);
#13312=LINE('',#90284,#19346);
#13313=LINE('',#90285,#19347);
#13314=LINE('',#90290,#19348);
#13315=LINE('',#90292,#19349);
#13316=LINE('',#90294,#19350);
#13317=LINE('',#90295,#19351);
#13318=LINE('',#90298,#19352);
#13319=LINE('',#90300,#19353);
#13320=LINE('',#90301,#19354);
#13321=LINE('',#90304,#19355);
#13322=LINE('',#90306,#19356);
#13323=LINE('',#90307,#19357);
#13324=LINE('',#90309,#19358);
#13325=LINE('',#90310,#19359);
#13326=LINE('',#90315,#19360);
#13327=LINE('',#90317,#19361);
#13328=LINE('',#90319,#19362);
#13329=LINE('',#90320,#19363);
#13330=LINE('',#90323,#19364);
#13331=LINE('',#90325,#19365);
#13332=LINE('',#90326,#19366);
#13333=LINE('',#90329,#19367);
#13334=LINE('',#90331,#19368);
#13335=LINE('',#90332,#19369);
#13336=LINE('',#90334,#19370);
#13337=LINE('',#90335,#19371);
#13338=LINE('',#90340,#19372);
#13339=LINE('',#90342,#19373);
#13340=LINE('',#90344,#19374);
#13341=LINE('',#90345,#19375);
#13342=LINE('',#90348,#19376);
#13343=LINE('',#90350,#19377);
#13344=LINE('',#90351,#19378);
#13345=LINE('',#90354,#19379);
#13346=LINE('',#90356,#19380);
#13347=LINE('',#90357,#19381);
#13348=LINE('',#90359,#19382);
#13349=LINE('',#90360,#19383);
#13350=LINE('',#90365,#19384);
#13351=LINE('',#90367,#19385);
#13352=LINE('',#90369,#19386);
#13353=LINE('',#90370,#19387);
#13354=LINE('',#90373,#19388);
#13355=LINE('',#90375,#19389);
#13356=LINE('',#90376,#19390);
#13357=LINE('',#90379,#19391);
#13358=LINE('',#90381,#19392);
#13359=LINE('',#90382,#19393);
#13360=LINE('',#90384,#19394);
#13361=LINE('',#90385,#19395);
#13362=LINE('',#90390,#19396);
#13363=LINE('',#90392,#19397);
#13364=LINE('',#90394,#19398);
#13365=LINE('',#90395,#19399);
#13366=LINE('',#90398,#19400);
#13367=LINE('',#90400,#19401);
#13368=LINE('',#90401,#19402);
#13369=LINE('',#90404,#19403);
#13370=LINE('',#90406,#19404);
#13371=LINE('',#90407,#19405);
#13372=LINE('',#90409,#19406);
#13373=LINE('',#90410,#19407);
#13374=LINE('',#90415,#19408);
#13375=LINE('',#90417,#19409);
#13376=LINE('',#90419,#19410);
#13377=LINE('',#90420,#19411);
#13378=LINE('',#90423,#19412);
#13379=LINE('',#90425,#19413);
#13380=LINE('',#90426,#19414);
#13381=LINE('',#90429,#19415);
#13382=LINE('',#90431,#19416);
#13383=LINE('',#90432,#19417);
#13384=LINE('',#90434,#19418);
#13385=LINE('',#90435,#19419);
#13386=LINE('',#90440,#19420);
#13387=LINE('',#90442,#19421);
#13388=LINE('',#90444,#19422);
#13389=LINE('',#90445,#19423);
#13390=LINE('',#90448,#19424);
#13391=LINE('',#90450,#19425);
#13392=LINE('',#90451,#19426);
#13393=LINE('',#90454,#19427);
#13394=LINE('',#90456,#19428);
#13395=LINE('',#90457,#19429);
#13396=LINE('',#90459,#19430);
#13397=LINE('',#90460,#19431);
#13398=LINE('',#90465,#19432);
#13399=LINE('',#90467,#19433);
#13400=LINE('',#90469,#19434);
#13401=LINE('',#90470,#19435);
#13402=LINE('',#90473,#19436);
#13403=LINE('',#90475,#19437);
#13404=LINE('',#90476,#19438);
#13405=LINE('',#90479,#19439);
#13406=LINE('',#90481,#19440);
#13407=LINE('',#90482,#19441);
#13408=LINE('',#90484,#19442);
#13409=LINE('',#90485,#19443);
#13410=LINE('',#90490,#19444);
#13411=LINE('',#90492,#19445);
#13412=LINE('',#90494,#19446);
#13413=LINE('',#90495,#19447);
#13414=LINE('',#90498,#19448);
#13415=LINE('',#90500,#19449);
#13416=LINE('',#90501,#19450);
#13417=LINE('',#90504,#19451);
#13418=LINE('',#90506,#19452);
#13419=LINE('',#90507,#19453);
#13420=LINE('',#90509,#19454);
#13421=LINE('',#90510,#19455);
#13422=LINE('',#90515,#19456);
#13423=LINE('',#90517,#19457);
#13424=LINE('',#90519,#19458);
#13425=LINE('',#90520,#19459);
#13426=LINE('',#90523,#19460);
#13427=LINE('',#90525,#19461);
#13428=LINE('',#90526,#19462);
#13429=LINE('',#90529,#19463);
#13430=LINE('',#90531,#19464);
#13431=LINE('',#90532,#19465);
#13432=LINE('',#90534,#19466);
#13433=LINE('',#90535,#19467);
#13434=LINE('',#90540,#19468);
#13435=LINE('',#90542,#19469);
#13436=LINE('',#90544,#19470);
#13437=LINE('',#90545,#19471);
#13438=LINE('',#90548,#19472);
#13439=LINE('',#90550,#19473);
#13440=LINE('',#90551,#19474);
#13441=LINE('',#90554,#19475);
#13442=LINE('',#90556,#19476);
#13443=LINE('',#90557,#19477);
#13444=LINE('',#90559,#19478);
#13445=LINE('',#90560,#19479);
#13446=LINE('',#90565,#19480);
#13447=LINE('',#90567,#19481);
#13448=LINE('',#90569,#19482);
#13449=LINE('',#90570,#19483);
#13450=LINE('',#90573,#19484);
#13451=LINE('',#90575,#19485);
#13452=LINE('',#90576,#19486);
#13453=LINE('',#90579,#19487);
#13454=LINE('',#90581,#19488);
#13455=LINE('',#90582,#19489);
#13456=LINE('',#90584,#19490);
#13457=LINE('',#90585,#19491);
#13458=LINE('',#90590,#19492);
#13459=LINE('',#90592,#19493);
#13460=LINE('',#90594,#19494);
#13461=LINE('',#90595,#19495);
#13462=LINE('',#90598,#19496);
#13463=LINE('',#90600,#19497);
#13464=LINE('',#90601,#19498);
#13465=LINE('',#90604,#19499);
#13466=LINE('',#90606,#19500);
#13467=LINE('',#90607,#19501);
#13468=LINE('',#90609,#19502);
#13469=LINE('',#90610,#19503);
#13470=LINE('',#90615,#19504);
#13471=LINE('',#90617,#19505);
#13472=LINE('',#90619,#19506);
#13473=LINE('',#90620,#19507);
#13474=LINE('',#90623,#19508);
#13475=LINE('',#90625,#19509);
#13476=LINE('',#90626,#19510);
#13477=LINE('',#90629,#19511);
#13478=LINE('',#90631,#19512);
#13479=LINE('',#90632,#19513);
#13480=LINE('',#90634,#19514);
#13481=LINE('',#90635,#19515);
#13482=LINE('',#90640,#19516);
#13483=LINE('',#90642,#19517);
#13484=LINE('',#90644,#19518);
#13485=LINE('',#90645,#19519);
#13486=LINE('',#90648,#19520);
#13487=LINE('',#90650,#19521);
#13488=LINE('',#90651,#19522);
#13489=LINE('',#90654,#19523);
#13490=LINE('',#90656,#19524);
#13491=LINE('',#90657,#19525);
#13492=LINE('',#90659,#19526);
#13493=LINE('',#90660,#19527);
#13494=LINE('',#90665,#19528);
#13495=LINE('',#90667,#19529);
#13496=LINE('',#90669,#19530);
#13497=LINE('',#90670,#19531);
#13498=LINE('',#90673,#19532);
#13499=LINE('',#90675,#19533);
#13500=LINE('',#90676,#19534);
#13501=LINE('',#90679,#19535);
#13502=LINE('',#90681,#19536);
#13503=LINE('',#90682,#19537);
#13504=LINE('',#90684,#19538);
#13505=LINE('',#90685,#19539);
#13506=LINE('',#90690,#19540);
#13507=LINE('',#90692,#19541);
#13508=LINE('',#90694,#19542);
#13509=LINE('',#90695,#19543);
#13510=LINE('',#90698,#19544);
#13511=LINE('',#90700,#19545);
#13512=LINE('',#90701,#19546);
#13513=LINE('',#90704,#19547);
#13514=LINE('',#90706,#19548);
#13515=LINE('',#90707,#19549);
#13516=LINE('',#90709,#19550);
#13517=LINE('',#90710,#19551);
#13518=LINE('',#90715,#19552);
#13519=LINE('',#90717,#19553);
#13520=LINE('',#90719,#19554);
#13521=LINE('',#90720,#19555);
#13522=LINE('',#90723,#19556);
#13523=LINE('',#90725,#19557);
#13524=LINE('',#90726,#19558);
#13525=LINE('',#90729,#19559);
#13526=LINE('',#90731,#19560);
#13527=LINE('',#90732,#19561);
#13528=LINE('',#90734,#19562);
#13529=LINE('',#90735,#19563);
#13530=LINE('',#90740,#19564);
#13531=LINE('',#90742,#19565);
#13532=LINE('',#90744,#19566);
#13533=LINE('',#90745,#19567);
#13534=LINE('',#90748,#19568);
#13535=LINE('',#90750,#19569);
#13536=LINE('',#90751,#19570);
#13537=LINE('',#90754,#19571);
#13538=LINE('',#90756,#19572);
#13539=LINE('',#90757,#19573);
#13540=LINE('',#90759,#19574);
#13541=LINE('',#90760,#19575);
#13542=LINE('',#90765,#19576);
#13543=LINE('',#90767,#19577);
#13544=LINE('',#90769,#19578);
#13545=LINE('',#90770,#19579);
#13546=LINE('',#90773,#19580);
#13547=LINE('',#90775,#19581);
#13548=LINE('',#90776,#19582);
#13549=LINE('',#90779,#19583);
#13550=LINE('',#90781,#19584);
#13551=LINE('',#90782,#19585);
#13552=LINE('',#90784,#19586);
#13553=LINE('',#90785,#19587);
#13554=LINE('',#90790,#19588);
#13555=LINE('',#90792,#19589);
#13556=LINE('',#90794,#19590);
#13557=LINE('',#90795,#19591);
#13558=LINE('',#90798,#19592);
#13559=LINE('',#90800,#19593);
#13560=LINE('',#90801,#19594);
#13561=LINE('',#90804,#19595);
#13562=LINE('',#90806,#19596);
#13563=LINE('',#90807,#19597);
#13564=LINE('',#90809,#19598);
#13565=LINE('',#90810,#19599);
#13566=LINE('',#90815,#19600);
#13567=LINE('',#90817,#19601);
#13568=LINE('',#90819,#19602);
#13569=LINE('',#90820,#19603);
#13570=LINE('',#90823,#19604);
#13571=LINE('',#90825,#19605);
#13572=LINE('',#90826,#19606);
#13573=LINE('',#90829,#19607);
#13574=LINE('',#90831,#19608);
#13575=LINE('',#90832,#19609);
#13576=LINE('',#90834,#19610);
#13577=LINE('',#90835,#19611);
#13578=LINE('',#90840,#19612);
#13579=LINE('',#90842,#19613);
#13580=LINE('',#90844,#19614);
#13581=LINE('',#90845,#19615);
#13582=LINE('',#90848,#19616);
#13583=LINE('',#90850,#19617);
#13584=LINE('',#90851,#19618);
#13585=LINE('',#90854,#19619);
#13586=LINE('',#90856,#19620);
#13587=LINE('',#90857,#19621);
#13588=LINE('',#90859,#19622);
#13589=LINE('',#90860,#19623);
#13590=LINE('',#90865,#19624);
#13591=LINE('',#90867,#19625);
#13592=LINE('',#90869,#19626);
#13593=LINE('',#90870,#19627);
#13594=LINE('',#90873,#19628);
#13595=LINE('',#90875,#19629);
#13596=LINE('',#90876,#19630);
#13597=LINE('',#90879,#19631);
#13598=LINE('',#90881,#19632);
#13599=LINE('',#90882,#19633);
#13600=LINE('',#90884,#19634);
#13601=LINE('',#90885,#19635);
#13602=LINE('',#90890,#19636);
#13603=LINE('',#90892,#19637);
#13604=LINE('',#90894,#19638);
#13605=LINE('',#90895,#19639);
#13606=LINE('',#90898,#19640);
#13607=LINE('',#90900,#19641);
#13608=LINE('',#90901,#19642);
#13609=LINE('',#90904,#19643);
#13610=LINE('',#90906,#19644);
#13611=LINE('',#90907,#19645);
#13612=LINE('',#90909,#19646);
#13613=LINE('',#90910,#19647);
#13614=LINE('',#90915,#19648);
#13615=LINE('',#90917,#19649);
#13616=LINE('',#90919,#19650);
#13617=LINE('',#90920,#19651);
#13618=LINE('',#90923,#19652);
#13619=LINE('',#90925,#19653);
#13620=LINE('',#90926,#19654);
#13621=LINE('',#90929,#19655);
#13622=LINE('',#90931,#19656);
#13623=LINE('',#90932,#19657);
#13624=LINE('',#90934,#19658);
#13625=LINE('',#90935,#19659);
#13626=LINE('',#90940,#19660);
#13627=LINE('',#90942,#19661);
#13628=LINE('',#90944,#19662);
#13629=LINE('',#90945,#19663);
#13630=LINE('',#90948,#19664);
#13631=LINE('',#90950,#19665);
#13632=LINE('',#90951,#19666);
#13633=LINE('',#90954,#19667);
#13634=LINE('',#90956,#19668);
#13635=LINE('',#90957,#19669);
#13636=LINE('',#90959,#19670);
#13637=LINE('',#90960,#19671);
#13638=LINE('',#90965,#19672);
#13639=LINE('',#90967,#19673);
#13640=LINE('',#90969,#19674);
#13641=LINE('',#90970,#19675);
#13642=LINE('',#90973,#19676);
#13643=LINE('',#90975,#19677);
#13644=LINE('',#90976,#19678);
#13645=LINE('',#90979,#19679);
#13646=LINE('',#90981,#19680);
#13647=LINE('',#90982,#19681);
#13648=LINE('',#90984,#19682);
#13649=LINE('',#90985,#19683);
#13650=LINE('',#90990,#19684);
#13651=LINE('',#90992,#19685);
#13652=LINE('',#90994,#19686);
#13653=LINE('',#90995,#19687);
#13654=LINE('',#90998,#19688);
#13655=LINE('',#91000,#19689);
#13656=LINE('',#91001,#19690);
#13657=LINE('',#91004,#19691);
#13658=LINE('',#91006,#19692);
#13659=LINE('',#91007,#19693);
#13660=LINE('',#91009,#19694);
#13661=LINE('',#91010,#19695);
#13662=LINE('',#91015,#19696);
#13663=LINE('',#91017,#19697);
#13664=LINE('',#91019,#19698);
#13665=LINE('',#91020,#19699);
#13666=LINE('',#91023,#19700);
#13667=LINE('',#91025,#19701);
#13668=LINE('',#91026,#19702);
#13669=LINE('',#91029,#19703);
#13670=LINE('',#91031,#19704);
#13671=LINE('',#91032,#19705);
#13672=LINE('',#91034,#19706);
#13673=LINE('',#91035,#19707);
#13674=LINE('',#91040,#19708);
#13675=LINE('',#91042,#19709);
#13676=LINE('',#91044,#19710);
#13677=LINE('',#91045,#19711);
#13678=LINE('',#91048,#19712);
#13679=LINE('',#91050,#19713);
#13680=LINE('',#91051,#19714);
#13681=LINE('',#91054,#19715);
#13682=LINE('',#91056,#19716);
#13683=LINE('',#91057,#19717);
#13684=LINE('',#91059,#19718);
#13685=LINE('',#91060,#19719);
#13686=LINE('',#91065,#19720);
#13687=LINE('',#91067,#19721);
#13688=LINE('',#91069,#19722);
#13689=LINE('',#91070,#19723);
#13690=LINE('',#91073,#19724);
#13691=LINE('',#91075,#19725);
#13692=LINE('',#91076,#19726);
#13693=LINE('',#91079,#19727);
#13694=LINE('',#91081,#19728);
#13695=LINE('',#91082,#19729);
#13696=LINE('',#91084,#19730);
#13697=LINE('',#91085,#19731);
#13698=LINE('',#91090,#19732);
#13699=LINE('',#91092,#19733);
#13700=LINE('',#91094,#19734);
#13701=LINE('',#91095,#19735);
#13702=LINE('',#91098,#19736);
#13703=LINE('',#91100,#19737);
#13704=LINE('',#91101,#19738);
#13705=LINE('',#91104,#19739);
#13706=LINE('',#91106,#19740);
#13707=LINE('',#91107,#19741);
#13708=LINE('',#91109,#19742);
#13709=LINE('',#91110,#19743);
#13710=LINE('',#91115,#19744);
#13711=LINE('',#91117,#19745);
#13712=LINE('',#91119,#19746);
#13713=LINE('',#91120,#19747);
#13714=LINE('',#91123,#19748);
#13715=LINE('',#91125,#19749);
#13716=LINE('',#91126,#19750);
#13717=LINE('',#91129,#19751);
#13718=LINE('',#91131,#19752);
#13719=LINE('',#91132,#19753);
#13720=LINE('',#91134,#19754);
#13721=LINE('',#91135,#19755);
#13722=LINE('',#91140,#19756);
#13723=LINE('',#91142,#19757);
#13724=LINE('',#91144,#19758);
#13725=LINE('',#91145,#19759);
#13726=LINE('',#91148,#19760);
#13727=LINE('',#91150,#19761);
#13728=LINE('',#91151,#19762);
#13729=LINE('',#91154,#19763);
#13730=LINE('',#91156,#19764);
#13731=LINE('',#91157,#19765);
#13732=LINE('',#91159,#19766);
#13733=LINE('',#91160,#19767);
#13734=LINE('',#91165,#19768);
#13735=LINE('',#91167,#19769);
#13736=LINE('',#91169,#19770);
#13737=LINE('',#91170,#19771);
#13738=LINE('',#91173,#19772);
#13739=LINE('',#91175,#19773);
#13740=LINE('',#91176,#19774);
#13741=LINE('',#91179,#19775);
#13742=LINE('',#91181,#19776);
#13743=LINE('',#91182,#19777);
#13744=LINE('',#91184,#19778);
#13745=LINE('',#91185,#19779);
#13746=LINE('',#91190,#19780);
#13747=LINE('',#91192,#19781);
#13748=LINE('',#91194,#19782);
#13749=LINE('',#91195,#19783);
#13750=LINE('',#91198,#19784);
#13751=LINE('',#91200,#19785);
#13752=LINE('',#91201,#19786);
#13753=LINE('',#91204,#19787);
#13754=LINE('',#91206,#19788);
#13755=LINE('',#91207,#19789);
#13756=LINE('',#91209,#19790);
#13757=LINE('',#91210,#19791);
#13758=LINE('',#91215,#19792);
#13759=LINE('',#91217,#19793);
#13760=LINE('',#91219,#19794);
#13761=LINE('',#91220,#19795);
#13762=LINE('',#91223,#19796);
#13763=LINE('',#91225,#19797);
#13764=LINE('',#91226,#19798);
#13765=LINE('',#91229,#19799);
#13766=LINE('',#91231,#19800);
#13767=LINE('',#91232,#19801);
#13768=LINE('',#91234,#19802);
#13769=LINE('',#91235,#19803);
#13770=LINE('',#91240,#19804);
#13771=LINE('',#91242,#19805);
#13772=LINE('',#91244,#19806);
#13773=LINE('',#91245,#19807);
#13774=LINE('',#91248,#19808);
#13775=LINE('',#91250,#19809);
#13776=LINE('',#91251,#19810);
#13777=LINE('',#91254,#19811);
#13778=LINE('',#91256,#19812);
#13779=LINE('',#91257,#19813);
#13780=LINE('',#91259,#19814);
#13781=LINE('',#91260,#19815);
#13782=LINE('',#91265,#19816);
#13783=LINE('',#91267,#19817);
#13784=LINE('',#91269,#19818);
#13785=LINE('',#91270,#19819);
#13786=LINE('',#91273,#19820);
#13787=LINE('',#91275,#19821);
#13788=LINE('',#91276,#19822);
#13789=LINE('',#91279,#19823);
#13790=LINE('',#91281,#19824);
#13791=LINE('',#91282,#19825);
#13792=LINE('',#91284,#19826);
#13793=LINE('',#91285,#19827);
#13794=LINE('',#91290,#19828);
#13795=LINE('',#91292,#19829);
#13796=LINE('',#91294,#19830);
#13797=LINE('',#91295,#19831);
#13798=LINE('',#91298,#19832);
#13799=LINE('',#91300,#19833);
#13800=LINE('',#91301,#19834);
#13801=LINE('',#91304,#19835);
#13802=LINE('',#91306,#19836);
#13803=LINE('',#91307,#19837);
#13804=LINE('',#91309,#19838);
#13805=LINE('',#91310,#19839);
#13806=LINE('',#91315,#19840);
#13807=LINE('',#91317,#19841);
#13808=LINE('',#91319,#19842);
#13809=LINE('',#91320,#19843);
#13810=LINE('',#91323,#19844);
#13811=LINE('',#91325,#19845);
#13812=LINE('',#91326,#19846);
#13813=LINE('',#91329,#19847);
#13814=LINE('',#91331,#19848);
#13815=LINE('',#91332,#19849);
#13816=LINE('',#91334,#19850);
#13817=LINE('',#91335,#19851);
#13818=LINE('',#91340,#19852);
#13819=LINE('',#91342,#19853);
#13820=LINE('',#91344,#19854);
#13821=LINE('',#91345,#19855);
#13822=LINE('',#91348,#19856);
#13823=LINE('',#91350,#19857);
#13824=LINE('',#91351,#19858);
#13825=LINE('',#91354,#19859);
#13826=LINE('',#91356,#19860);
#13827=LINE('',#91357,#19861);
#13828=LINE('',#91359,#19862);
#13829=LINE('',#91360,#19863);
#13830=LINE('',#91365,#19864);
#13831=LINE('',#91367,#19865);
#13832=LINE('',#91369,#19866);
#13833=LINE('',#91370,#19867);
#13834=LINE('',#91373,#19868);
#13835=LINE('',#91375,#19869);
#13836=LINE('',#91376,#19870);
#13837=LINE('',#91379,#19871);
#13838=LINE('',#91381,#19872);
#13839=LINE('',#91382,#19873);
#13840=LINE('',#91384,#19874);
#13841=LINE('',#91385,#19875);
#13842=LINE('',#91390,#19876);
#13843=LINE('',#91392,#19877);
#13844=LINE('',#91394,#19878);
#13845=LINE('',#91395,#19879);
#13846=LINE('',#91398,#19880);
#13847=LINE('',#91400,#19881);
#13848=LINE('',#91401,#19882);
#13849=LINE('',#91404,#19883);
#13850=LINE('',#91406,#19884);
#13851=LINE('',#91407,#19885);
#13852=LINE('',#91409,#19886);
#13853=LINE('',#91410,#19887);
#13854=LINE('',#91415,#19888);
#13855=LINE('',#91417,#19889);
#13856=LINE('',#91419,#19890);
#13857=LINE('',#91420,#19891);
#13858=LINE('',#91423,#19892);
#13859=LINE('',#91425,#19893);
#13860=LINE('',#91426,#19894);
#13861=LINE('',#91429,#19895);
#13862=LINE('',#91431,#19896);
#13863=LINE('',#91432,#19897);
#13864=LINE('',#91434,#19898);
#13865=LINE('',#91435,#19899);
#13866=LINE('',#91440,#19900);
#13867=LINE('',#91442,#19901);
#13868=LINE('',#91444,#19902);
#13869=LINE('',#91445,#19903);
#13870=LINE('',#91448,#19904);
#13871=LINE('',#91450,#19905);
#13872=LINE('',#91451,#19906);
#13873=LINE('',#91454,#19907);
#13874=LINE('',#91456,#19908);
#13875=LINE('',#91457,#19909);
#13876=LINE('',#91459,#19910);
#13877=LINE('',#91460,#19911);
#13878=LINE('',#91465,#19912);
#13879=LINE('',#91467,#19913);
#13880=LINE('',#91469,#19914);
#13881=LINE('',#91470,#19915);
#13882=LINE('',#91473,#19916);
#13883=LINE('',#91475,#19917);
#13884=LINE('',#91476,#19918);
#13885=LINE('',#91479,#19919);
#13886=LINE('',#91481,#19920);
#13887=LINE('',#91482,#19921);
#13888=LINE('',#91484,#19922);
#13889=LINE('',#91485,#19923);
#13890=LINE('',#91490,#19924);
#13891=LINE('',#91492,#19925);
#13892=LINE('',#91494,#19926);
#13893=LINE('',#91495,#19927);
#13894=LINE('',#91498,#19928);
#13895=LINE('',#91500,#19929);
#13896=LINE('',#91501,#19930);
#13897=LINE('',#91504,#19931);
#13898=LINE('',#91506,#19932);
#13899=LINE('',#91507,#19933);
#13900=LINE('',#91509,#19934);
#13901=LINE('',#91510,#19935);
#13902=LINE('',#91515,#19936);
#13903=LINE('',#91517,#19937);
#13904=LINE('',#91519,#19938);
#13905=LINE('',#91520,#19939);
#13906=LINE('',#91523,#19940);
#13907=LINE('',#91525,#19941);
#13908=LINE('',#91526,#19942);
#13909=LINE('',#91529,#19943);
#13910=LINE('',#91531,#19944);
#13911=LINE('',#91532,#19945);
#13912=LINE('',#91534,#19946);
#13913=LINE('',#91535,#19947);
#13914=LINE('',#91540,#19948);
#13915=LINE('',#91542,#19949);
#13916=LINE('',#91544,#19950);
#13917=LINE('',#91545,#19951);
#13918=LINE('',#91548,#19952);
#13919=LINE('',#91550,#19953);
#13920=LINE('',#91551,#19954);
#13921=LINE('',#91554,#19955);
#13922=LINE('',#91556,#19956);
#13923=LINE('',#91557,#19957);
#13924=LINE('',#91559,#19958);
#13925=LINE('',#91560,#19959);
#13926=LINE('',#91565,#19960);
#13927=LINE('',#91567,#19961);
#13928=LINE('',#91569,#19962);
#13929=LINE('',#91570,#19963);
#13930=LINE('',#91573,#19964);
#13931=LINE('',#91575,#19965);
#13932=LINE('',#91576,#19966);
#13933=LINE('',#91579,#19967);
#13934=LINE('',#91581,#19968);
#13935=LINE('',#91582,#19969);
#13936=LINE('',#91584,#19970);
#13937=LINE('',#91585,#19971);
#13938=LINE('',#91590,#19972);
#13939=LINE('',#91592,#19973);
#13940=LINE('',#91594,#19974);
#13941=LINE('',#91595,#19975);
#13942=LINE('',#91598,#19976);
#13943=LINE('',#91600,#19977);
#13944=LINE('',#91601,#19978);
#13945=LINE('',#91604,#19979);
#13946=LINE('',#91606,#19980);
#13947=LINE('',#91607,#19981);
#13948=LINE('',#91609,#19982);
#13949=LINE('',#91610,#19983);
#13950=LINE('',#91615,#19984);
#13951=LINE('',#91617,#19985);
#13952=LINE('',#91619,#19986);
#13953=LINE('',#91620,#19987);
#13954=LINE('',#91623,#19988);
#13955=LINE('',#91625,#19989);
#13956=LINE('',#91626,#19990);
#13957=LINE('',#91629,#19991);
#13958=LINE('',#91631,#19992);
#13959=LINE('',#91632,#19993);
#13960=LINE('',#91634,#19994);
#13961=LINE('',#91635,#19995);
#13962=LINE('',#91640,#19996);
#13963=LINE('',#91642,#19997);
#13964=LINE('',#91644,#19998);
#13965=LINE('',#91645,#19999);
#13966=LINE('',#91648,#20000);
#13967=LINE('',#91650,#20001);
#13968=LINE('',#91651,#20002);
#13969=LINE('',#91654,#20003);
#13970=LINE('',#91656,#20004);
#13971=LINE('',#91657,#20005);
#13972=LINE('',#91659,#20006);
#13973=LINE('',#91660,#20007);
#13974=LINE('',#91665,#20008);
#13975=LINE('',#91667,#20009);
#13976=LINE('',#91669,#20010);
#13977=LINE('',#91670,#20011);
#13978=LINE('',#91673,#20012);
#13979=LINE('',#91675,#20013);
#13980=LINE('',#91676,#20014);
#13981=LINE('',#91679,#20015);
#13982=LINE('',#91681,#20016);
#13983=LINE('',#91682,#20017);
#13984=LINE('',#91684,#20018);
#13985=LINE('',#91685,#20019);
#13986=LINE('',#91690,#20020);
#13987=LINE('',#91692,#20021);
#13988=LINE('',#91694,#20022);
#13989=LINE('',#91696,#20023);
#13990=LINE('',#91698,#20024);
#13991=LINE('',#91699,#20025);
#13992=LINE('',#91703,#20026);
#13993=LINE('',#91705,#20027);
#13994=LINE('',#91707,#20028);
#13995=LINE('',#91709,#20029);
#13996=LINE('',#91711,#20030);
#13997=LINE('',#91712,#20031);
#13998=LINE('',#91714,#20032);
#13999=LINE('',#91715,#20033);
#14000=LINE('',#91718,#20034);
#14001=LINE('',#91720,#20035);
#14002=LINE('',#91722,#20036);
#14003=LINE('',#91724,#20037);
#14004=LINE('',#91726,#20038);
#14005=LINE('',#91730,#20039);
#14006=LINE('',#91732,#20040);
#14007=LINE('',#91734,#20041);
#14008=LINE('',#91736,#20042);
#14009=LINE('',#91738,#20043);
#14010=LINE('',#91740,#20044);
#14011=LINE('',#91742,#20045);
#14012=LINE('',#91744,#20046);
#14013=LINE('',#91746,#20047);
#14014=LINE('',#91750,#20048);
#14015=LINE('',#91752,#20049);
#14016=LINE('',#91754,#20050);
#14017=LINE('',#91756,#20051);
#14018=LINE('',#91757,#20052);
#14019=LINE('',#91760,#20053);
#14020=LINE('',#91762,#20054);
#14021=LINE('',#91763,#20055);
#14022=LINE('',#91766,#20056);
#14023=LINE('',#91768,#20057);
#14024=LINE('',#91769,#20058);
#14025=LINE('',#91772,#20059);
#14026=LINE('',#91773,#20060);
#14027=LINE('',#91775,#20061);
#14028=LINE('',#91786,#20062);
#14029=LINE('',#91791,#20063);
#14030=LINE('',#91795,#20064);
#14031=LINE('',#91799,#20065);
#14032=LINE('',#91804,#20066);
#14033=LINE('',#91808,#20067);
#14034=LINE('',#91813,#20068);
#14035=LINE('',#91815,#20069);
#14036=LINE('',#91817,#20070);
#14037=LINE('',#91818,#20071);
#14038=LINE('',#91823,#20072);
#14039=LINE('',#91826,#20073);
#14040=LINE('',#91830,#20074);
#14041=LINE('',#91834,#20075);
#14042=LINE('',#91839,#20076);
#14043=LINE('',#91848,#20077);
#14044=LINE('',#91857,#20078);
#14045=LINE('',#91866,#20079);
#14046=LINE('',#91875,#20080);
#14047=LINE('',#91884,#20081);
#14048=LINE('',#91891,#20082);
#14049=LINE('',#91895,#20083);
#14050=LINE('',#91896,#20084);
#14051=LINE('',#91904,#20085);
#14052=LINE('',#91907,#20086);
#14053=LINE('',#91910,#20087);
#14054=LINE('',#91913,#20088);
#14055=LINE('',#91916,#20089);
#14056=LINE('',#91919,#20090);
#14057=LINE('',#91922,#20091);
#14058=LINE('',#91925,#20092);
#14059=LINE('',#91928,#20093);
#14060=LINE('',#91931,#20094);
#14061=LINE('',#91934,#20095);
#14062=LINE('',#91938,#20096);
#14063=LINE('',#91942,#20097);
#14064=LINE('',#91943,#20098);
#14065=LINE('',#91946,#20099);
#14066=LINE('',#91948,#20100);
#14067=LINE('',#91949,#20101);
#14068=LINE('',#91952,#20102);
#14069=LINE('',#91954,#20103);
#14070=LINE('',#91955,#20104);
#14071=LINE('',#91959,#20105);
#14072=LINE('',#91961,#20106);
#14073=LINE('',#91962,#20107);
#14074=LINE('',#91963,#20108);
#14075=LINE('',#91966,#20109);
#14076=LINE('',#91968,#20110);
#14077=LINE('',#91969,#20111);
#14078=LINE('',#91972,#20112);
#14079=LINE('',#91974,#20113);
#14080=LINE('',#91975,#20114);
#14081=LINE('',#91978,#20115);
#14082=LINE('',#91981,#20116);
#14083=LINE('',#91984,#20117);
#14084=LINE('',#91985,#20118);
#14085=LINE('',#91987,#20119);
#14086=LINE('',#91988,#20120);
#14087=LINE('',#91991,#20121);
#14088=LINE('',#91996,#20122);
#14089=LINE('',#92002,#20123);
#14090=LINE('',#92003,#20124);
#14091=LINE('',#92006,#20125);
#14092=LINE('',#92007,#20126);
#14093=LINE('',#92010,#20127);
#14094=LINE('',#92011,#20128);
#14095=LINE('',#92013,#20129);
#14096=LINE('',#92016,#20130);
#14097=LINE('',#92017,#20131);
#14098=LINE('',#92021,#20132);
#14099=LINE('',#92025,#20133);
#14100=LINE('',#92026,#20134);
#14101=LINE('',#92029,#20135);
#14102=LINE('',#92031,#20136);
#14103=LINE('',#92032,#20137);
#14104=LINE('',#92035,#20138);
#14105=LINE('',#92037,#20139);
#14106=LINE('',#92038,#20140);
#14107=LINE('',#92040,#20141);
#14108=LINE('',#92041,#20142);
#14109=LINE('',#92044,#20143);
#14110=LINE('',#92046,#20144);
#14111=LINE('',#92047,#20145);
#14112=LINE('',#92050,#20146);
#14113=LINE('',#92052,#20147);
#14114=LINE('',#92053,#20148);
#14115=LINE('',#92056,#20149);
#14116=LINE('',#92058,#20150);
#14117=LINE('',#92059,#20151);
#14118=LINE('',#92061,#20152);
#14119=LINE('',#92062,#20153);
#14120=LINE('',#92065,#20154);
#14121=LINE('',#92067,#20155);
#14122=LINE('',#92068,#20156);
#14123=LINE('',#92071,#20157);
#14124=LINE('',#92072,#20158);
#14125=LINE('',#92075,#20159);
#14126=LINE('',#92076,#20160);
#14127=LINE('',#92078,#20161);
#14128=LINE('',#92081,#20162);
#14129=LINE('',#92082,#20163);
#14130=LINE('',#92085,#20164);
#14131=LINE('',#92086,#20165);
#14132=LINE('',#92089,#20166);
#14133=LINE('',#92090,#20167);
#14134=LINE('',#92092,#20168);
#14135=LINE('',#92096,#20169);
#14136=LINE('',#92098,#20170);
#14137=LINE('',#92101,#20171);
#14138=LINE('',#92102,#20172);
#14139=LINE('',#92104,#20173);
#14140=LINE('',#92105,#20174);
#14141=LINE('',#92107,#20175);
#14142=LINE('',#92109,#20176);
#14143=LINE('',#92111,#20177);
#14144=LINE('',#92113,#20178);
#14145=LINE('',#92115,#20179);
#14146=LINE('',#92118,#20180);
#14147=LINE('',#92120,#20181);
#14148=LINE('',#92122,#20182);
#14149=LINE('',#92125,#20183);
#14150=LINE('',#92127,#20184);
#14151=LINE('',#92129,#20185);
#14152=LINE('',#92131,#20186);
#14153=LINE('',#92137,#20187);
#14154=LINE('',#92139,#20188);
#14155=LINE('',#92141,#20189);
#16910=VECTOR('',#63780,10.);
#16911=VECTOR('',#63781,10.);
#16912=VECTOR('',#63782,10.);
#16913=VECTOR('',#63783,10.);
#16914=VECTOR('',#63784,10.);
#16915=VECTOR('',#63785,10.);
#16916=VECTOR('',#63786,10.);
#16917=VECTOR('',#63787,10.);
#16918=VECTOR('',#63788,10.);
#16919=VECTOR('',#63789,10.);
#16920=VECTOR('',#63790,10.);
#16921=VECTOR('',#63791,10.);
#16922=VECTOR('',#63792,10.);
#16923=VECTOR('',#63793,10.);
#16924=VECTOR('',#63794,10.);
#16925=VECTOR('',#63795,10.);
#16926=VECTOR('',#63796,10.);
#16927=VECTOR('',#63797,10.);
#16928=VECTOR('',#63798,10.);
#16929=VECTOR('',#63799,10.);
#16930=VECTOR('',#63802,10.);
#16931=VECTOR('',#63803,10.);
#16932=VECTOR('',#63804,10.);
#16933=VECTOR('',#63805,10.);
#16934=VECTOR('',#63806,10.);
#16935=VECTOR('',#63807,10.);
#16936=VECTOR('',#63808,10.);
#16937=VECTOR('',#63809,10.);
#16938=VECTOR('',#63810,10.);
#16939=VECTOR('',#63811,10.);
#16940=VECTOR('',#63812,10.);
#16941=VECTOR('',#63813,10.);
#16942=VECTOR('',#63814,10.);
#16943=VECTOR('',#63815,10.);
#16944=VECTOR('',#63816,10.);
#16945=VECTOR('',#63817,10.);
#16946=VECTOR('',#63818,10.);
#16947=VECTOR('',#63819,10.);
#16948=VECTOR('',#63820,10.);
#16949=VECTOR('',#63821,10.);
#16950=VECTOR('',#63822,10.);
#16951=VECTOR('',#63823,10.);
#16952=VECTOR('',#63824,10.);
#16953=VECTOR('',#63825,10.);
#16954=VECTOR('',#63826,10.);
#16955=VECTOR('',#63827,10.);
#16956=VECTOR('',#63828,10.);
#16957=VECTOR('',#63829,10.);
#16958=VECTOR('',#63830,10.);
#16959=VECTOR('',#63833,10.);
#16960=VECTOR('',#63834,10.);
#16961=VECTOR('',#63835,10.);
#16962=VECTOR('',#63842,10.);
#16963=VECTOR('',#63843,10.);
#16964=VECTOR('',#63844,10.);
#16965=VECTOR('',#63845,10.);
#16966=VECTOR('',#63846,10.);
#16967=VECTOR('',#63847,10.);
#16968=VECTOR('',#63848,10.);
#16969=VECTOR('',#63849,10.);
#16970=VECTOR('',#63850,10.);
#16971=VECTOR('',#63851,10.);
#16972=VECTOR('',#63852,10.);
#16973=VECTOR('',#63853,10.);
#16974=VECTOR('',#63854,10.);
#16975=VECTOR('',#63855,10.);
#16976=VECTOR('',#63856,10.);
#16977=VECTOR('',#63857,10.);
#16978=VECTOR('',#63858,10.);
#16979=VECTOR('',#63859,10.);
#16980=VECTOR('',#63860,10.);
#16981=VECTOR('',#63861,10.);
#16982=VECTOR('',#63864,10.);
#16983=VECTOR('',#63865,10.);
#16984=VECTOR('',#63866,10.);
#16985=VECTOR('',#63867,10.);
#16986=VECTOR('',#63868,10.);
#16987=VECTOR('',#63869,10.);
#16988=VECTOR('',#63870,10.);
#16989=VECTOR('',#63871,10.);
#16990=VECTOR('',#63872,10.);
#16991=VECTOR('',#63873,10.);
#16992=VECTOR('',#63874,10.);
#16993=VECTOR('',#63875,10.);
#16994=VECTOR('',#63876,10.);
#16995=VECTOR('',#63877,10.);
#16996=VECTOR('',#63878,10.);
#16997=VECTOR('',#63879,10.);
#16998=VECTOR('',#63880,10.);
#16999=VECTOR('',#63881,10.);
#17000=VECTOR('',#63882,10.);
#17001=VECTOR('',#63883,10.);
#17002=VECTOR('',#63884,10.);
#17003=VECTOR('',#63885,10.);
#17004=VECTOR('',#63886,10.);
#17005=VECTOR('',#63887,10.);
#17006=VECTOR('',#63888,10.);
#17007=VECTOR('',#63889,10.);
#17008=VECTOR('',#63890,10.);
#17009=VECTOR('',#63891,10.);
#17010=VECTOR('',#63892,10.);
#17011=VECTOR('',#63893,10.);
#17012=VECTOR('',#63894,10.);
#17013=VECTOR('',#63895,10.);
#17014=VECTOR('',#63896,10.);
#17015=VECTOR('',#63905,10.);
#17016=VECTOR('',#63906,10.);
#17017=VECTOR('',#63907,10.);
#17018=VECTOR('',#63908,10.);
#17019=VECTOR('',#63909,10.);
#17020=VECTOR('',#63910,10.);
#17021=VECTOR('',#63911,10.);
#17022=VECTOR('',#63912,10.);
#17023=VECTOR('',#63913,10.);
#17024=VECTOR('',#63914,10.);
#17025=VECTOR('',#63915,10.);
#17026=VECTOR('',#63916,10.);
#17027=VECTOR('',#63917,10.);
#17028=VECTOR('',#63918,10.);
#17029=VECTOR('',#63919,10.);
#17030=VECTOR('',#63920,10.);
#17031=VECTOR('',#63921,10.);
#17032=VECTOR('',#63922,10.);
#17033=VECTOR('',#63923,10.);
#17034=VECTOR('',#63924,10.);
#17035=VECTOR('',#63927,10.);
#17036=VECTOR('',#63928,10.);
#17037=VECTOR('',#63929,10.);
#17038=VECTOR('',#63930,10.);
#17039=VECTOR('',#63933,10.);
#17040=VECTOR('',#63934,10.);
#17041=VECTOR('',#63935,10.);
#17042=VECTOR('',#63936,10.);
#17043=VECTOR('',#63937,10.);
#17044=VECTOR('',#63938,10.);
#17045=VECTOR('',#63941,10.);
#17046=VECTOR('',#63942,10.);
#17047=VECTOR('',#63943,10.);
#17048=VECTOR('',#63946,10.);
#17049=VECTOR('',#63947,10.);
#17050=VECTOR('',#63948,10.);
#17051=VECTOR('',#63951,10.);
#17052=VECTOR('',#63952,10.);
#17053=VECTOR('',#63953,10.);
#17054=VECTOR('',#63956,10.);
#17055=VECTOR('',#63957,10.);
#17056=VECTOR('',#63962,10.);
#17057=VECTOR('',#63963,10.);
#17058=VECTOR('',#63964,10.);
#17059=VECTOR('',#63965,10.);
#17060=VECTOR('',#63966,10.);
#17061=VECTOR('',#63967,10.);
#17062=VECTOR('',#63968,10.);
#17063=VECTOR('',#63969,10.);
#17064=VECTOR('',#63970,10.);
#17065=VECTOR('',#63971,10.);
#17066=VECTOR('',#63972,10.);
#17067=VECTOR('',#63973,10.);
#17068=VECTOR('',#63974,10.);
#17069=VECTOR('',#63975,10.);
#17070=VECTOR('',#63976,10.);
#17071=VECTOR('',#63977,10.);
#17072=VECTOR('',#63978,10.);
#17073=VECTOR('',#63979,10.);
#17074=VECTOR('',#63980,10.);
#17075=VECTOR('',#63981,10.);
#17076=VECTOR('',#63984,10.);
#17077=VECTOR('',#63985,10.);
#17078=VECTOR('',#63986,10.);
#17079=VECTOR('',#63987,10.);
#17080=VECTOR('',#63988,10.);
#17081=VECTOR('',#63989,10.);
#17082=VECTOR('',#63990,10.);
#17083=VECTOR('',#63991,10.);
#17084=VECTOR('',#63992,10.);
#17085=VECTOR('',#63993,10.);
#17086=VECTOR('',#63994,10.);
#17087=VECTOR('',#63995,10.);
#17088=VECTOR('',#63996,10.);
#17089=VECTOR('',#63997,10.);
#17090=VECTOR('',#63998,10.);
#17091=VECTOR('',#63999,10.);
#17092=VECTOR('',#64000,10.);
#17093=VECTOR('',#64001,10.);
#17094=VECTOR('',#64002,10.);
#17095=VECTOR('',#64003,10.);
#17096=VECTOR('',#64004,10.);
#17097=VECTOR('',#64005,10.);
#17098=VECTOR('',#64006,10.);
#17099=VECTOR('',#64007,10.);
#17100=VECTOR('',#64008,10.);
#17101=VECTOR('',#64009,10.);
#17102=VECTOR('',#64010,10.);
#17103=VECTOR('',#64013,10.);
#17104=VECTOR('',#64014,10.);
#17105=VECTOR('',#64015,10.);
#17106=VECTOR('',#64022,10.);
#17107=VECTOR('',#64023,10.);
#17108=VECTOR('',#64024,10.);
#17109=VECTOR('',#64025,10.);
#17110=VECTOR('',#64026,10.);
#17111=VECTOR('',#64027,10.);
#17112=VECTOR('',#64028,10.);
#17113=VECTOR('',#64029,10.);
#17114=VECTOR('',#64030,10.);
#17115=VECTOR('',#64031,10.);
#17116=VECTOR('',#64032,10.);
#17117=VECTOR('',#64033,10.);
#17118=VECTOR('',#64034,10.);
#17119=VECTOR('',#64035,10.);
#17120=VECTOR('',#64036,10.);
#17121=VECTOR('',#64037,10.);
#17122=VECTOR('',#64038,10.);
#17123=VECTOR('',#64039,10.);
#17124=VECTOR('',#64040,10.);
#17125=VECTOR('',#64041,10.);
#17126=VECTOR('',#64044,10.);
#17127=VECTOR('',#64045,10.);
#17128=VECTOR('',#64046,10.);
#17129=VECTOR('',#64047,10.);
#17130=VECTOR('',#64048,10.);
#17131=VECTOR('',#64049,10.);
#17132=VECTOR('',#64050,10.);
#17133=VECTOR('',#64053,10.);
#17134=VECTOR('',#64054,10.);
#17135=VECTOR('',#64055,10.);
#17136=VECTOR('',#64058,10.);
#17137=VECTOR('',#64059,10.);
#17138=VECTOR('',#64060,10.);
#17139=VECTOR('',#64063,10.);
#17140=VECTOR('',#64064,10.);
#17141=VECTOR('',#64065,10.);
#17142=VECTOR('',#64068,10.);
#17143=VECTOR('',#64069,10.);
#17144=VECTOR('',#64070,10.);
#17145=VECTOR('',#64073,10.);
#17146=VECTOR('',#64074,10.);
#17147=VECTOR('',#64075,10.);
#17148=VECTOR('',#64078,10.);
#17149=VECTOR('',#64079,10.);
#17150=VECTOR('',#64080,10.);
#17151=VECTOR('',#64081,10.);
#17152=VECTOR('',#64082,10.);
#17153=VECTOR('',#64083,10.);
#17154=VECTOR('',#64084,10.);
#17155=VECTOR('',#64085,10.);
#17156=VECTOR('',#64086,10.);
#17157=VECTOR('',#64087,10.);
#17158=VECTOR('',#64088,10.);
#17159=VECTOR('',#64091,10.);
#17160=VECTOR('',#64092,10.);
#17161=VECTOR('',#64093,10.);
#17162=VECTOR('',#64098,10.);
#17163=VECTOR('',#64099,10.);
#17164=VECTOR('',#64100,10.);
#17165=VECTOR('',#64101,10.);
#17166=VECTOR('',#64102,10.);
#17167=VECTOR('',#64103,10.);
#17168=VECTOR('',#64104,10.);
#17169=VECTOR('',#64105,10.);
#17170=VECTOR('',#64106,10.);
#17171=VECTOR('',#64107,10.);
#17172=VECTOR('',#64108,10.);
#17173=VECTOR('',#64109,10.);
#17174=VECTOR('',#64110,10.);
#17175=VECTOR('',#64111,10.);
#17176=VECTOR('',#64112,10.);
#17177=VECTOR('',#64113,10.);
#17178=VECTOR('',#64114,10.);
#17179=VECTOR('',#64115,10.);
#17180=VECTOR('',#64116,10.);
#17181=VECTOR('',#64117,10.);
#17182=VECTOR('',#64122,10.);
#17183=VECTOR('',#64123,10.);
#17184=VECTOR('',#64124,10.);
#17185=VECTOR('',#64125,10.);
#17186=VECTOR('',#64128,10.);
#17187=VECTOR('',#64129,10.);
#17188=VECTOR('',#64130,10.);
#17189=VECTOR('',#64133,10.);
#17190=VECTOR('',#64134,10.);
#17191=VECTOR('',#64137,10.);
#17192=VECTOR('',#64138,10.);
#17193=VECTOR('',#64139,10.);
#17194=VECTOR('',#64140,10.);
#17195=VECTOR('',#64143,10.);
#17196=VECTOR('',#64144,10.);
#17197=VECTOR('',#64145,10.);
#17198=VECTOR('',#64148,10.);
#17199=VECTOR('',#64149,10.);
#17200=VECTOR('',#64150,10.);
#17201=VECTOR('',#64153,10.);
#17202=VECTOR('',#64154,10.);
#17203=VECTOR('',#64155,10.);
#17204=VECTOR('',#64158,10.);
#17205=VECTOR('',#64159,10.);
#17206=VECTOR('',#64160,10.);
#17207=VECTOR('',#64163,10.);
#17208=VECTOR('',#64164,10.);
#17209=VECTOR('',#64165,10.);
#17210=VECTOR('',#64168,10.);
#17211=VECTOR('',#64169,10.);
#17212=VECTOR('',#64170,10.);
#17213=VECTOR('',#64173,10.);
#17214=VECTOR('',#64174,10.);
#17215=VECTOR('',#64175,10.);
#17216=VECTOR('',#64178,10.);
#17217=VECTOR('',#64179,10.);
#17218=VECTOR('',#64180,10.);
#17219=VECTOR('',#64183,10.);
#17220=VECTOR('',#64184,10.);
#17221=VECTOR('',#64185,10.);
#17222=VECTOR('',#64188,10.);
#17223=VECTOR('',#64189,10.);
#17224=VECTOR('',#64196,10.);
#17225=VECTOR('',#64197,10.);
#17226=VECTOR('',#64198,10.);
#17227=VECTOR('',#64199,10.);
#17228=VECTOR('',#64200,10.);
#17229=VECTOR('',#64201,10.);
#17230=VECTOR('',#64202,10.);
#17231=VECTOR('',#64203,10.);
#17232=VECTOR('',#64204,10.);
#17233=VECTOR('',#64205,10.);
#17234=VECTOR('',#64206,10.);
#17235=VECTOR('',#64207,10.);
#17236=VECTOR('',#64208,10.);
#17237=VECTOR('',#64209,10.);
#17238=VECTOR('',#64210,10.);
#17239=VECTOR('',#64211,10.);
#17240=VECTOR('',#64212,10.);
#17241=VECTOR('',#64213,10.);
#17242=VECTOR('',#64214,10.);
#17243=VECTOR('',#64215,10.);
#17244=VECTOR('',#64218,10.);
#17245=VECTOR('',#64219,10.);
#17246=VECTOR('',#64220,10.);
#17247=VECTOR('',#64221,10.);
#17248=VECTOR('',#64222,10.);
#17249=VECTOR('',#64223,10.);
#17250=VECTOR('',#64224,10.);
#17251=VECTOR('',#64225,10.);
#17252=VECTOR('',#64226,10.);
#17253=VECTOR('',#64227,10.);
#17254=VECTOR('',#64228,10.);
#17255=VECTOR('',#64229,10.);
#17256=VECTOR('',#64230,10.);
#17257=VECTOR('',#64233,10.);
#17258=VECTOR('',#64234,10.);
#17259=VECTOR('',#64235,10.);
#17260=VECTOR('',#64236,10.);
#17261=VECTOR('',#64237,10.);
#17262=VECTOR('',#64238,10.);
#17263=VECTOR('',#64239,10.);
#17264=VECTOR('',#64240,10.);
#17265=VECTOR('',#64241,10.);
#17266=VECTOR('',#64242,10.);
#17267=VECTOR('',#64245,10.);
#17268=VECTOR('',#64246,10.);
#17269=VECTOR('',#64247,10.);
#17270=VECTOR('',#64248,10.);
#17271=VECTOR('',#64249,10.);
#17272=VECTOR('',#64250,10.);
#17273=VECTOR('',#64251,10.);
#17274=VECTOR('',#64252,10.);
#17275=VECTOR('',#64253,10.);
#17276=VECTOR('',#64254,10.);
#17277=VECTOR('',#64257,10.);
#17278=VECTOR('',#64258,10.);
#17279=VECTOR('',#64259,10.);
#17280=VECTOR('',#64264,10.);
#17281=VECTOR('',#64265,10.);
#17282=VECTOR('',#64266,10.);
#17283=VECTOR('',#64267,10.);
#17284=VECTOR('',#64268,10.);
#17285=VECTOR('',#64269,10.);
#17286=VECTOR('',#64270,10.);
#17287=VECTOR('',#64271,10.);
#17288=VECTOR('',#64272,10.);
#17289=VECTOR('',#64273,10.);
#17290=VECTOR('',#64274,10.);
#17291=VECTOR('',#64275,10.);
#17292=VECTOR('',#64276,10.);
#17293=VECTOR('',#64277,10.);
#17294=VECTOR('',#64278,10.);
#17295=VECTOR('',#64279,10.);
#17296=VECTOR('',#64280,10.);
#17297=VECTOR('',#64281,10.);
#17298=VECTOR('',#64282,10.);
#17299=VECTOR('',#64283,10.);
#17300=VECTOR('',#64286,10.);
#17301=VECTOR('',#64287,10.);
#17302=VECTOR('',#64288,10.);
#17303=VECTOR('',#64289,10.);
#17304=VECTOR('',#64290,10.);
#17305=VECTOR('',#64291,10.);
#17306=VECTOR('',#64292,10.);
#17307=VECTOR('',#64293,10.);
#17308=VECTOR('',#64294,10.);
#17309=VECTOR('',#64295,10.);
#17310=VECTOR('',#64298,10.);
#17311=VECTOR('',#64299,10.);
#17312=VECTOR('',#64300,10.);
#17313=VECTOR('',#64301,10.);
#17314=VECTOR('',#64302,10.);
#17315=VECTOR('',#64303,10.);
#17316=VECTOR('',#64304,10.);
#17317=VECTOR('',#64305,10.);
#17318=VECTOR('',#64306,10.);
#17319=VECTOR('',#64307,10.);
#17320=VECTOR('',#64308,10.);
#17321=VECTOR('',#64309,10.);
#17322=VECTOR('',#64312,10.);
#17323=VECTOR('',#64313,10.);
#17324=VECTOR('',#64314,10.);
#17325=VECTOR('',#64317,10.);
#17326=VECTOR('',#64318,10.);
#17327=VECTOR('',#64319,10.);
#17328=VECTOR('',#64322,10.);
#17329=VECTOR('',#64323,10.);
#17330=VECTOR('',#64328,10.);
#17331=VECTOR('',#64329,10.);
#17332=VECTOR('',#64330,10.);
#17333=VECTOR('',#64331,10.);
#17334=VECTOR('',#64332,10.);
#17335=VECTOR('',#64333,10.);
#17336=VECTOR('',#64334,10.);
#17337=VECTOR('',#64335,10.);
#17338=VECTOR('',#64336,10.);
#17339=VECTOR('',#64337,10.);
#17340=VECTOR('',#64338,10.);
#17341=VECTOR('',#64339,10.);
#17342=VECTOR('',#64340,10.);
#17343=VECTOR('',#64341,10.);
#17344=VECTOR('',#64342,10.);
#17345=VECTOR('',#64343,10.);
#17346=VECTOR('',#64344,10.);
#17347=VECTOR('',#64345,10.);
#17348=VECTOR('',#64346,10.);
#17349=VECTOR('',#64347,10.);
#17350=VECTOR('',#64352,10.);
#17351=VECTOR('',#64353,10.);
#17352=VECTOR('',#64354,10.);
#17353=VECTOR('',#64355,10.);
#17354=VECTOR('',#64356,10.);
#17355=VECTOR('',#64357,10.);
#17356=VECTOR('',#64360,10.);
#17357=VECTOR('',#64361,10.);
#17358=VECTOR('',#64362,10.);
#17359=VECTOR('',#64363,10.);
#17360=VECTOR('',#64364,10.);
#17361=VECTOR('',#64367,10.);
#17362=VECTOR('',#64368,10.);
#17363=VECTOR('',#64369,10.);
#17364=VECTOR('',#64372,10.);
#17365=VECTOR('',#64373,10.);
#17366=VECTOR('',#64374,10.);
#17367=VECTOR('',#64377,10.);
#17368=VECTOR('',#64378,10.);
#17369=VECTOR('',#64383,10.);
#17370=VECTOR('',#64384,10.);
#17371=VECTOR('',#64385,10.);
#17372=VECTOR('',#64386,10.);
#17373=VECTOR('',#64387,10.);
#17374=VECTOR('',#64388,10.);
#17375=VECTOR('',#64389,10.);
#17376=VECTOR('',#64390,10.);
#17377=VECTOR('',#64391,10.);
#17378=VECTOR('',#64392,10.);
#17379=VECTOR('',#64393,10.);
#17380=VECTOR('',#64394,10.);
#17381=VECTOR('',#64395,10.);
#17382=VECTOR('',#64396,10.);
#17383=VECTOR('',#64397,10.);
#17384=VECTOR('',#64398,10.);
#17385=VECTOR('',#64399,10.);
#17386=VECTOR('',#64400,10.);
#17387=VECTOR('',#64401,10.);
#17388=VECTOR('',#64402,10.);
#17389=VECTOR('',#64407,10.);
#17390=VECTOR('',#64408,10.);
#17391=VECTOR('',#64409,10.);
#17392=VECTOR('',#64410,10.);
#17393=VECTOR('',#64411,10.);
#17394=VECTOR('',#64412,10.);
#17395=VECTOR('',#64413,10.);
#17396=VECTOR('',#64414,10.);
#17397=VECTOR('',#64415,10.);
#17398=VECTOR('',#64416,10.);
#17399=VECTOR('',#64417,10.);
#17400=VECTOR('',#64418,10.);
#17401=VECTOR('',#64419,10.);
#17402=VECTOR('',#64420,10.);
#17403=VECTOR('',#64421,10.);
#17404=VECTOR('',#64422,10.);
#17405=VECTOR('',#64423,10.);
#17406=VECTOR('',#64424,10.);
#17407=VECTOR('',#64425,10.);
#17408=VECTOR('',#64426,10.);
#17409=VECTOR('',#64431,10.);
#17410=VECTOR('',#64432,10.);
#17411=VECTOR('',#64433,10.);
#17412=VECTOR('',#64434,10.);
#17413=VECTOR('',#64435,10.);
#17414=VECTOR('',#64436,10.);
#17415=VECTOR('',#64439,10.);
#17416=VECTOR('',#64440,10.);
#17417=VECTOR('',#64441,10.);
#17418=VECTOR('',#64442,10.);
#17419=VECTOR('',#64443,10.);
#17420=VECTOR('',#64446,10.);
#17421=VECTOR('',#64447,10.);
#17422=VECTOR('',#64448,10.);
#17423=VECTOR('',#64451,10.);
#17424=VECTOR('',#64452,10.);
#17425=VECTOR('',#64453,10.);
#17426=VECTOR('',#64456,10.);
#17427=VECTOR('',#64457,10.);
#17428=VECTOR('',#64462,10.);
#17429=VECTOR('',#64463,10.);
#17430=VECTOR('',#64464,10.);
#17431=VECTOR('',#64465,10.);
#17432=VECTOR('',#64466,10.);
#17433=VECTOR('',#64467,10.);
#17434=VECTOR('',#64468,10.);
#17435=VECTOR('',#64469,10.);
#17436=VECTOR('',#64470,10.);
#17437=VECTOR('',#64471,10.);
#17438=VECTOR('',#64472,10.);
#17439=VECTOR('',#64473,10.);
#17440=VECTOR('',#64474,10.);
#17441=VECTOR('',#64475,10.);
#17442=VECTOR('',#64476,10.);
#17443=VECTOR('',#64477,10.);
#17444=VECTOR('',#64478,10.);
#17445=VECTOR('',#64479,10.);
#17446=VECTOR('',#64480,10.);
#17447=VECTOR('',#64481,10.);
#17448=VECTOR('',#64484,10.);
#17449=VECTOR('',#64485,10.);
#17450=VECTOR('',#64486,10.);
#17451=VECTOR('',#64487,10.);
#17452=VECTOR('',#64488,10.);
#17453=VECTOR('',#64489,10.);
#17454=VECTOR('',#64490,10.);
#17455=VECTOR('',#64491,10.);
#17456=VECTOR('',#64492,10.);
#17457=VECTOR('',#64493,10.);
#17458=VECTOR('',#64496,10.);
#17459=VECTOR('',#64497,10.);
#17460=VECTOR('',#64498,10.);
#17461=VECTOR('',#64499,10.);
#17462=VECTOR('',#64500,10.);
#17463=VECTOR('',#64501,10.);
#17464=VECTOR('',#64502,10.);
#17465=VECTOR('',#64503,10.);
#17466=VECTOR('',#64504,10.);
#17467=VECTOR('',#64505,10.);
#17468=VECTOR('',#64506,10.);
#17469=VECTOR('',#64507,10.);
#17470=VECTOR('',#64510,10.);
#17471=VECTOR('',#64511,10.);
#17472=VECTOR('',#64512,10.);
#17473=VECTOR('',#64515,10.);
#17474=VECTOR('',#64516,10.);
#17475=VECTOR('',#64517,10.);
#17476=VECTOR('',#64520,10.);
#17477=VECTOR('',#64521,10.);
#17478=VECTOR('',#64526,10.);
#17479=VECTOR('',#64527,10.);
#17480=VECTOR('',#64528,10.);
#17481=VECTOR('',#64529,10.);
#17482=VECTOR('',#64530,10.);
#17483=VECTOR('',#64531,10.);
#17484=VECTOR('',#64532,10.);
#17485=VECTOR('',#64533,10.);
#17486=VECTOR('',#64534,10.);
#17487=VECTOR('',#64535,10.);
#17488=VECTOR('',#64536,10.);
#17489=VECTOR('',#64537,10.);
#17490=VECTOR('',#64538,10.);
#17491=VECTOR('',#64539,10.);
#17492=VECTOR('',#64540,10.);
#17493=VECTOR('',#64541,10.);
#17494=VECTOR('',#64542,10.);
#17495=VECTOR('',#64543,10.);
#17496=VECTOR('',#64544,10.);
#17497=VECTOR('',#64545,10.);
#17498=VECTOR('',#64548,10.);
#17499=VECTOR('',#64549,10.);
#17500=VECTOR('',#64550,10.);
#17501=VECTOR('',#64551,10.);
#17502=VECTOR('',#64552,10.);
#17503=VECTOR('',#64553,10.);
#17504=VECTOR('',#64554,10.);
#17505=VECTOR('',#64555,10.);
#17506=VECTOR('',#64556,10.);
#17507=VECTOR('',#64557,10.);
#17508=VECTOR('',#64558,10.);
#17509=VECTOR('',#64559,10.);
#17510=VECTOR('',#64560,10.);
#17511=VECTOR('',#64563,10.);
#17512=VECTOR('',#64564,10.);
#17513=VECTOR('',#64565,10.);
#17514=VECTOR('',#64566,10.);
#17515=VECTOR('',#64567,10.);
#17516=VECTOR('',#64568,10.);
#17517=VECTOR('',#64569,10.);
#17518=VECTOR('',#64570,10.);
#17519=VECTOR('',#64571,10.);
#17520=VECTOR('',#64572,10.);
#17521=VECTOR('',#64575,10.);
#17522=VECTOR('',#64576,10.);
#17523=VECTOR('',#64577,10.);
#17524=VECTOR('',#64578,10.);
#17525=VECTOR('',#64579,10.);
#17526=VECTOR('',#64580,10.);
#17527=VECTOR('',#64581,10.);
#17528=VECTOR('',#64582,10.);
#17529=VECTOR('',#64583,10.);
#17530=VECTOR('',#64584,10.);
#17531=VECTOR('',#64587,10.);
#17532=VECTOR('',#64588,10.);
#17533=VECTOR('',#64589,10.);
#17534=VECTOR('',#64594,10.);
#17535=VECTOR('',#64595,10.);
#17536=VECTOR('',#64596,10.);
#17537=VECTOR('',#64597,10.);
#17538=VECTOR('',#64598,10.);
#17539=VECTOR('',#64599,10.);
#17540=VECTOR('',#64600,10.);
#17541=VECTOR('',#64601,10.);
#17542=VECTOR('',#64602,10.);
#17543=VECTOR('',#64603,10.);
#17544=VECTOR('',#64604,10.);
#17545=VECTOR('',#64605,10.);
#17546=VECTOR('',#64606,10.);
#17547=VECTOR('',#64607,10.);
#17548=VECTOR('',#64608,10.);
#17549=VECTOR('',#64609,10.);
#17550=VECTOR('',#64610,10.);
#17551=VECTOR('',#64611,10.);
#17552=VECTOR('',#64612,10.);
#17553=VECTOR('',#64613,10.);
#17554=VECTOR('',#64618,10.);
#17555=VECTOR('',#64619,10.);
#17556=VECTOR('',#64620,10.);
#17557=VECTOR('',#64621,10.);
#17558=VECTOR('',#64624,10.);
#17559=VECTOR('',#64625,10.);
#17560=VECTOR('',#64626,10.);
#17561=VECTOR('',#64629,10.);
#17562=VECTOR('',#64630,10.);
#17563=VECTOR('',#64633,10.);
#17564=VECTOR('',#64634,10.);
#17565=VECTOR('',#64635,10.);
#17566=VECTOR('',#64636,10.);
#17567=VECTOR('',#64639,10.);
#17568=VECTOR('',#64640,10.);
#17569=VECTOR('',#64641,10.);
#17570=VECTOR('',#64644,10.);
#17571=VECTOR('',#64645,10.);
#17572=VECTOR('',#64646,10.);
#17573=VECTOR('',#64649,10.);
#17574=VECTOR('',#64650,10.);
#17575=VECTOR('',#64651,10.);
#17576=VECTOR('',#64654,10.);
#17577=VECTOR('',#64655,10.);
#17578=VECTOR('',#64656,10.);
#17579=VECTOR('',#64659,10.);
#17580=VECTOR('',#64660,10.);
#17581=VECTOR('',#64661,10.);
#17582=VECTOR('',#64664,10.);
#17583=VECTOR('',#64665,10.);
#17584=VECTOR('',#64666,10.);
#17585=VECTOR('',#64669,10.);
#17586=VECTOR('',#64670,10.);
#17587=VECTOR('',#64671,10.);
#17588=VECTOR('',#64674,10.);
#17589=VECTOR('',#64675,10.);
#17590=VECTOR('',#64676,10.);
#17591=VECTOR('',#64679,10.);
#17592=VECTOR('',#64680,10.);
#17593=VECTOR('',#64681,10.);
#17594=VECTOR('',#64684,10.);
#17595=VECTOR('',#64685,10.);
#17596=VECTOR('',#64692,10.);
#17597=VECTOR('',#64693,10.);
#17598=VECTOR('',#64694,10.);
#17599=VECTOR('',#64695,10.);
#17600=VECTOR('',#64696,10.);
#17601=VECTOR('',#64697,10.);
#17602=VECTOR('',#64698,10.);
#17603=VECTOR('',#64699,10.);
#17604=VECTOR('',#64700,10.);
#17605=VECTOR('',#64701,10.);
#17606=VECTOR('',#64702,10.);
#17607=VECTOR('',#64703,10.);
#17608=VECTOR('',#64704,10.);
#17609=VECTOR('',#64705,10.);
#17610=VECTOR('',#64706,10.);
#17611=VECTOR('',#64707,10.);
#17612=VECTOR('',#64708,10.);
#17613=VECTOR('',#64709,10.);
#17614=VECTOR('',#64710,10.);
#17615=VECTOR('',#64711,10.);
#17616=VECTOR('',#64714,10.);
#17617=VECTOR('',#64715,10.);
#17618=VECTOR('',#64716,10.);
#17619=VECTOR('',#64717,10.);
#17620=VECTOR('',#64718,10.);
#17621=VECTOR('',#64719,10.);
#17622=VECTOR('',#64720,10.);
#17623=VECTOR('',#64723,10.);
#17624=VECTOR('',#64724,10.);
#17625=VECTOR('',#64725,10.);
#17626=VECTOR('',#64728,10.);
#17627=VECTOR('',#64729,10.);
#17628=VECTOR('',#64730,10.);
#17629=VECTOR('',#64733,10.);
#17630=VECTOR('',#64734,10.);
#17631=VECTOR('',#64735,10.);
#17632=VECTOR('',#64738,10.);
#17633=VECTOR('',#64739,10.);
#17634=VECTOR('',#64740,10.);
#17635=VECTOR('',#64743,10.);
#17636=VECTOR('',#64744,10.);
#17637=VECTOR('',#64745,10.);
#17638=VECTOR('',#64748,10.);
#17639=VECTOR('',#64749,10.);
#17640=VECTOR('',#64750,10.);
#17641=VECTOR('',#64751,10.);
#17642=VECTOR('',#64752,10.);
#17643=VECTOR('',#64753,10.);
#17644=VECTOR('',#64754,10.);
#17645=VECTOR('',#64755,10.);
#17646=VECTOR('',#64756,10.);
#17647=VECTOR('',#64757,10.);
#17648=VECTOR('',#64758,10.);
#17649=VECTOR('',#64761,10.);
#17650=VECTOR('',#64762,10.);
#17651=VECTOR('',#64763,10.);
#17652=VECTOR('',#64768,10.);
#17653=VECTOR('',#64769,10.);
#17654=VECTOR('',#64770,10.);
#17655=VECTOR('',#64771,10.);
#17656=VECTOR('',#64772,10.);
#17657=VECTOR('',#64773,10.);
#17658=VECTOR('',#64774,10.);
#17659=VECTOR('',#64775,10.);
#17660=VECTOR('',#64776,10.);
#17661=VECTOR('',#64777,10.);
#17662=VECTOR('',#64778,10.);
#17663=VECTOR('',#64779,10.);
#17664=VECTOR('',#64780,10.);
#17665=VECTOR('',#64781,10.);
#17666=VECTOR('',#64782,10.);
#17667=VECTOR('',#64783,10.);
#17668=VECTOR('',#64784,10.);
#17669=VECTOR('',#64785,10.);
#17670=VECTOR('',#64786,10.);
#17671=VECTOR('',#64787,10.);
#17672=VECTOR('',#64790,10.);
#17673=VECTOR('',#64791,10.);
#17674=VECTOR('',#64792,10.);
#17675=VECTOR('',#64793,10.);
#17676=VECTOR('',#64794,10.);
#17677=VECTOR('',#64795,10.);
#17678=VECTOR('',#64796,10.);
#17679=VECTOR('',#64797,10.);
#17680=VECTOR('',#64798,10.);
#17681=VECTOR('',#64799,10.);
#17682=VECTOR('',#64800,10.);
#17683=VECTOR('',#64801,10.);
#17684=VECTOR('',#64802,10.);
#17685=VECTOR('',#64803,10.);
#17686=VECTOR('',#64804,10.);
#17687=VECTOR('',#64805,10.);
#17688=VECTOR('',#64806,10.);
#17689=VECTOR('',#64807,10.);
#17690=VECTOR('',#64808,10.);
#17691=VECTOR('',#64809,10.);
#17692=VECTOR('',#64810,10.);
#17693=VECTOR('',#64811,10.);
#17694=VECTOR('',#64812,10.);
#17695=VECTOR('',#64813,10.);
#17696=VECTOR('',#64814,10.);
#17697=VECTOR('',#64815,10.);
#17698=VECTOR('',#64816,10.);
#17699=VECTOR('',#64819,10.);
#17700=VECTOR('',#64820,10.);
#17701=VECTOR('',#64821,10.);
#17702=VECTOR('',#64828,10.);
#17703=VECTOR('',#64829,10.);
#17704=VECTOR('',#64830,10.);
#17705=VECTOR('',#64831,10.);
#17706=VECTOR('',#64832,10.);
#17707=VECTOR('',#64833,10.);
#17708=VECTOR('',#64834,10.);
#17709=VECTOR('',#64835,10.);
#17710=VECTOR('',#64836,10.);
#17711=VECTOR('',#64837,10.);
#17712=VECTOR('',#64838,10.);
#17713=VECTOR('',#64839,10.);
#17714=VECTOR('',#64840,10.);
#17715=VECTOR('',#64841,10.);
#17716=VECTOR('',#64842,10.);
#17717=VECTOR('',#64843,10.);
#17718=VECTOR('',#64844,10.);
#17719=VECTOR('',#64845,10.);
#17720=VECTOR('',#64846,10.);
#17721=VECTOR('',#64847,10.);
#17722=VECTOR('',#64850,10.);
#17723=VECTOR('',#64851,10.);
#17724=VECTOR('',#64852,10.);
#17725=VECTOR('',#64853,10.);
#17726=VECTOR('',#64856,10.);
#17727=VECTOR('',#64857,10.);
#17728=VECTOR('',#64858,10.);
#17729=VECTOR('',#64859,10.);
#17730=VECTOR('',#64860,10.);
#17731=VECTOR('',#64861,10.);
#17732=VECTOR('',#64864,10.);
#17733=VECTOR('',#64865,10.);
#17734=VECTOR('',#64866,10.);
#17735=VECTOR('',#64869,10.);
#17736=VECTOR('',#64870,10.);
#17737=VECTOR('',#64871,10.);
#17738=VECTOR('',#64874,10.);
#17739=VECTOR('',#64875,10.);
#17740=VECTOR('',#64876,10.);
#17741=VECTOR('',#64879,10.);
#17742=VECTOR('',#64880,10.);
#17743=VECTOR('',#64885,10.);
#17744=VECTOR('',#64886,10.);
#17745=VECTOR('',#64887,10.);
#17746=VECTOR('',#64888,10.);
#17747=VECTOR('',#64889,10.);
#17748=VECTOR('',#64890,10.);
#17749=VECTOR('',#64891,10.);
#17750=VECTOR('',#64892,10.);
#17751=VECTOR('',#64893,10.);
#17752=VECTOR('',#64894,10.);
#17753=VECTOR('',#64895,10.);
#17754=VECTOR('',#64896,10.);
#17755=VECTOR('',#64897,10.);
#17756=VECTOR('',#64898,10.);
#17757=VECTOR('',#64899,10.);
#17758=VECTOR('',#64900,10.);
#17759=VECTOR('',#64901,10.);
#17760=VECTOR('',#64902,10.);
#17761=VECTOR('',#64903,10.);
#17762=VECTOR('',#64904,10.);
#17763=VECTOR('',#64907,10.);
#17764=VECTOR('',#64908,10.);
#17765=VECTOR('',#64909,10.);
#17766=VECTOR('',#64910,10.);
#17767=VECTOR('',#64911,10.);
#17768=VECTOR('',#64912,10.);
#17769=VECTOR('',#64913,10.);
#17770=VECTOR('',#64914,10.);
#17771=VECTOR('',#64915,10.);
#17772=VECTOR('',#64916,10.);
#17773=VECTOR('',#64917,10.);
#17774=VECTOR('',#64918,10.);
#17775=VECTOR('',#64919,10.);
#17776=VECTOR('',#64920,10.);
#17777=VECTOR('',#64921,10.);
#17778=VECTOR('',#64922,10.);
#17779=VECTOR('',#64923,10.);
#17780=VECTOR('',#64924,10.);
#17781=VECTOR('',#64925,10.);
#17782=VECTOR('',#64926,10.);
#17783=VECTOR('',#64927,10.);
#17784=VECTOR('',#64928,10.);
#17785=VECTOR('',#64929,10.);
#17786=VECTOR('',#64930,10.);
#17787=VECTOR('',#64931,10.);
#17788=VECTOR('',#64932,10.);
#17789=VECTOR('',#64933,10.);
#17790=VECTOR('',#64934,10.);
#17791=VECTOR('',#64935,10.);
#17792=VECTOR('',#64936,10.);
#17793=VECTOR('',#64937,10.);
#17794=VECTOR('',#64938,10.);
#17795=VECTOR('',#64939,10.);
#17796=VECTOR('',#64948,10.);
#17797=VECTOR('',#64949,10.);
#17798=VECTOR('',#64950,10.);
#17799=VECTOR('',#64951,10.);
#17800=VECTOR('',#64952,10.);
#17801=VECTOR('',#64953,10.);
#17802=VECTOR('',#64954,10.);
#17803=VECTOR('',#64955,10.);
#17804=VECTOR('',#64956,10.);
#17805=VECTOR('',#64957,10.);
#17806=VECTOR('',#64958,10.);
#17807=VECTOR('',#64959,10.);
#17808=VECTOR('',#64960,10.);
#17809=VECTOR('',#64961,10.);
#17810=VECTOR('',#64962,10.);
#17811=VECTOR('',#64963,10.);
#17812=VECTOR('',#64964,10.);
#17813=VECTOR('',#64965,10.);
#17814=VECTOR('',#64966,10.);
#17815=VECTOR('',#64967,10.);
#17816=VECTOR('',#64970,10.);
#17817=VECTOR('',#64971,10.);
#17818=VECTOR('',#64972,10.);
#17819=VECTOR('',#64973,10.);
#17820=VECTOR('',#64974,10.);
#17821=VECTOR('',#64975,10.);
#17822=VECTOR('',#64976,10.);
#17823=VECTOR('',#64977,10.);
#17824=VECTOR('',#64978,10.);
#17825=VECTOR('',#64979,10.);
#17826=VECTOR('',#64980,10.);
#17827=VECTOR('',#64981,10.);
#17828=VECTOR('',#64982,10.);
#17829=VECTOR('',#64983,10.);
#17830=VECTOR('',#64984,10.);
#17831=VECTOR('',#64985,10.);
#17832=VECTOR('',#64986,10.);
#17833=VECTOR('',#64987,10.);
#17834=VECTOR('',#64988,10.);
#17835=VECTOR('',#64989,10.);
#17836=VECTOR('',#64990,10.);
#17837=VECTOR('',#64991,10.);
#17838=VECTOR('',#64992,10.);
#17839=VECTOR('',#64993,10.);
#17840=VECTOR('',#64994,10.);
#17841=VECTOR('',#64995,10.);
#17842=VECTOR('',#64996,10.);
#17843=VECTOR('',#64997,10.);
#17844=VECTOR('',#64998,10.);
#17845=VECTOR('',#65001,10.);
#17846=VECTOR('',#65002,10.);
#17847=VECTOR('',#65003,10.);
#17848=VECTOR('',#65012,10.);
#17849=VECTOR('',#65013,10.);
#17850=VECTOR('',#65014,10.);
#17851=VECTOR('',#65015,10.);
#17852=VECTOR('',#65018,10.);
#17853=VECTOR('',#65019,10.);
#17854=VECTOR('',#65020,10.);
#17855=VECTOR('',#65023,10.);
#17856=VECTOR('',#65024,10.);
#17857=VECTOR('',#65025,10.);
#17858=VECTOR('',#65028,10.);
#17859=VECTOR('',#65029,10.);
#17860=VECTOR('',#65034,10.);
#17861=VECTOR('',#65035,10.);
#17862=VECTOR('',#65036,10.);
#17863=VECTOR('',#65037,10.);
#17864=VECTOR('',#65040,10.);
#17865=VECTOR('',#65041,10.);
#17866=VECTOR('',#65042,10.);
#17867=VECTOR('',#65045,10.);
#17868=VECTOR('',#65046,10.);
#17869=VECTOR('',#65047,10.);
#17870=VECTOR('',#65050,10.);
#17871=VECTOR('',#65051,10.);
#17872=VECTOR('',#65056,10.);
#17873=VECTOR('',#65057,10.);
#17874=VECTOR('',#65058,10.);
#17875=VECTOR('',#65059,10.);
#17876=VECTOR('',#65062,10.);
#17877=VECTOR('',#65063,10.);
#17878=VECTOR('',#65064,10.);
#17879=VECTOR('',#65067,10.);
#17880=VECTOR('',#65068,10.);
#17881=VECTOR('',#65069,10.);
#17882=VECTOR('',#65072,10.);
#17883=VECTOR('',#65073,10.);
#17884=VECTOR('',#65078,10.);
#17885=VECTOR('',#65079,10.);
#17886=VECTOR('',#65080,10.);
#17887=VECTOR('',#65081,10.);
#17888=VECTOR('',#65084,10.);
#17889=VECTOR('',#65085,10.);
#17890=VECTOR('',#65086,10.);
#17891=VECTOR('',#65089,10.);
#17892=VECTOR('',#65090,10.);
#17893=VECTOR('',#65091,10.);
#17894=VECTOR('',#65094,10.);
#17895=VECTOR('',#65095,10.);
#17896=VECTOR('',#65100,10.);
#17897=VECTOR('',#65101,10.);
#17898=VECTOR('',#65102,10.);
#17899=VECTOR('',#65103,10.);
#17900=VECTOR('',#65106,10.);
#17901=VECTOR('',#65107,10.);
#17902=VECTOR('',#65108,10.);
#17903=VECTOR('',#65111,10.);
#17904=VECTOR('',#65112,10.);
#17905=VECTOR('',#65113,10.);
#17906=VECTOR('',#65116,10.);
#17907=VECTOR('',#65117,10.);
#17908=VECTOR('',#65122,10.);
#17909=VECTOR('',#65123,10.);
#17910=VECTOR('',#65124,10.);
#17911=VECTOR('',#65125,10.);
#17912=VECTOR('',#65128,10.);
#17913=VECTOR('',#65129,10.);
#17914=VECTOR('',#65130,10.);
#17915=VECTOR('',#65133,10.);
#17916=VECTOR('',#65134,10.);
#17917=VECTOR('',#65135,10.);
#17918=VECTOR('',#65138,10.);
#17919=VECTOR('',#65139,10.);
#17920=VECTOR('',#65144,10.);
#17921=VECTOR('',#65145,10.);
#17922=VECTOR('',#65146,10.);
#17923=VECTOR('',#65147,10.);
#17924=VECTOR('',#65150,10.);
#17925=VECTOR('',#65151,10.);
#17926=VECTOR('',#65152,10.);
#17927=VECTOR('',#65155,10.);
#17928=VECTOR('',#65156,10.);
#17929=VECTOR('',#65157,10.);
#17930=VECTOR('',#65160,10.);
#17931=VECTOR('',#65161,10.);
#17932=VECTOR('',#65166,10.);
#17933=VECTOR('',#65167,10.);
#17934=VECTOR('',#65168,10.);
#17935=VECTOR('',#65169,10.);
#17936=VECTOR('',#65172,10.);
#17937=VECTOR('',#65173,10.);
#17938=VECTOR('',#65174,10.);
#17939=VECTOR('',#65177,10.);
#17940=VECTOR('',#65178,10.);
#17941=VECTOR('',#65179,10.);
#17942=VECTOR('',#65182,10.);
#17943=VECTOR('',#65183,10.);
#17944=VECTOR('',#65188,10.);
#17945=VECTOR('',#65189,10.);
#17946=VECTOR('',#65190,10.);
#17947=VECTOR('',#65191,10.);
#17948=VECTOR('',#65194,10.);
#17949=VECTOR('',#65195,10.);
#17950=VECTOR('',#65196,10.);
#17951=VECTOR('',#65199,10.);
#17952=VECTOR('',#65200,10.);
#17953=VECTOR('',#65201,10.);
#17954=VECTOR('',#65204,10.);
#17955=VECTOR('',#65205,10.);
#17956=VECTOR('',#65210,10.);
#17957=VECTOR('',#65211,10.);
#17958=VECTOR('',#65212,10.);
#17959=VECTOR('',#65213,10.);
#17960=VECTOR('',#65216,10.);
#17961=VECTOR('',#65217,10.);
#17962=VECTOR('',#65218,10.);
#17963=VECTOR('',#65221,10.);
#17964=VECTOR('',#65222,10.);
#17965=VECTOR('',#65223,10.);
#17966=VECTOR('',#65226,10.);
#17967=VECTOR('',#65227,10.);
#17968=VECTOR('',#65232,10.);
#17969=VECTOR('',#65233,10.);
#17970=VECTOR('',#65234,10.);
#17971=VECTOR('',#65235,10.);
#17972=VECTOR('',#65238,10.);
#17973=VECTOR('',#65239,10.);
#17974=VECTOR('',#65240,10.);
#17975=VECTOR('',#65243,10.);
#17976=VECTOR('',#65244,10.);
#17977=VECTOR('',#65245,10.);
#17978=VECTOR('',#65248,10.);
#17979=VECTOR('',#65249,10.);
#17980=VECTOR('',#65254,10.);
#17981=VECTOR('',#65255,10.);
#17982=VECTOR('',#65256,10.);
#17983=VECTOR('',#65257,10.);
#17984=VECTOR('',#65260,10.);
#17985=VECTOR('',#65261,10.);
#17986=VECTOR('',#65262,10.);
#17987=VECTOR('',#65265,10.);
#17988=VECTOR('',#65266,10.);
#17989=VECTOR('',#65267,10.);
#17990=VECTOR('',#65270,10.);
#17991=VECTOR('',#65271,10.);
#17992=VECTOR('',#65276,10.);
#17993=VECTOR('',#65277,10.);
#17994=VECTOR('',#65278,10.);
#17995=VECTOR('',#65279,10.);
#17996=VECTOR('',#65282,10.);
#17997=VECTOR('',#65283,10.);
#17998=VECTOR('',#65284,10.);
#17999=VECTOR('',#65287,10.);
#18000=VECTOR('',#65288,10.);
#18001=VECTOR('',#65289,10.);
#18002=VECTOR('',#65292,10.);
#18003=VECTOR('',#65293,10.);
#18004=VECTOR('',#65298,10.);
#18005=VECTOR('',#65299,10.);
#18006=VECTOR('',#65300,10.);
#18007=VECTOR('',#65301,10.);
#18008=VECTOR('',#65304,10.);
#18009=VECTOR('',#65305,10.);
#18010=VECTOR('',#65306,10.);
#18011=VECTOR('',#65309,10.);
#18012=VECTOR('',#65310,10.);
#18013=VECTOR('',#65311,10.);
#18014=VECTOR('',#65314,10.);
#18015=VECTOR('',#65315,10.);
#18016=VECTOR('',#65320,10.);
#18017=VECTOR('',#65321,10.);
#18018=VECTOR('',#65322,10.);
#18019=VECTOR('',#65323,10.);
#18020=VECTOR('',#65326,10.);
#18021=VECTOR('',#65327,10.);
#18022=VECTOR('',#65328,10.);
#18023=VECTOR('',#65331,10.);
#18024=VECTOR('',#65332,10.);
#18025=VECTOR('',#65333,10.);
#18026=VECTOR('',#65336,10.);
#18027=VECTOR('',#65337,10.);
#18028=VECTOR('',#65342,10.);
#18029=VECTOR('',#65343,10.);
#18030=VECTOR('',#65344,10.);
#18031=VECTOR('',#65345,10.);
#18032=VECTOR('',#65348,10.);
#18033=VECTOR('',#65349,10.);
#18034=VECTOR('',#65350,10.);
#18035=VECTOR('',#65353,10.);
#18036=VECTOR('',#65354,10.);
#18037=VECTOR('',#65355,10.);
#18038=VECTOR('',#65358,10.);
#18039=VECTOR('',#65359,10.);
#18040=VECTOR('',#65364,10.);
#18041=VECTOR('',#65365,10.);
#18042=VECTOR('',#65366,10.);
#18043=VECTOR('',#65367,10.);
#18044=VECTOR('',#65370,10.);
#18045=VECTOR('',#65371,10.);
#18046=VECTOR('',#65372,10.);
#18047=VECTOR('',#65375,10.);
#18048=VECTOR('',#65376,10.);
#18049=VECTOR('',#65377,10.);
#18050=VECTOR('',#65380,10.);
#18051=VECTOR('',#65381,10.);
#18052=VECTOR('',#65386,10.);
#18053=VECTOR('',#65387,10.);
#18054=VECTOR('',#65388,10.);
#18055=VECTOR('',#65389,10.);
#18056=VECTOR('',#65392,10.);
#18057=VECTOR('',#65393,10.);
#18058=VECTOR('',#65394,10.);
#18059=VECTOR('',#65397,10.);
#18060=VECTOR('',#65398,10.);
#18061=VECTOR('',#65399,10.);
#18062=VECTOR('',#65402,10.);
#18063=VECTOR('',#65403,10.);
#18064=VECTOR('',#65408,10.);
#18065=VECTOR('',#65409,10.);
#18066=VECTOR('',#65410,10.);
#18067=VECTOR('',#65411,10.);
#18068=VECTOR('',#65414,10.);
#18069=VECTOR('',#65415,10.);
#18070=VECTOR('',#65416,10.);
#18071=VECTOR('',#65419,10.);
#18072=VECTOR('',#65420,10.);
#18073=VECTOR('',#65421,10.);
#18074=VECTOR('',#65424,10.);
#18075=VECTOR('',#65425,10.);
#18076=VECTOR('',#65430,10.);
#18077=VECTOR('',#65431,10.);
#18078=VECTOR('',#65432,10.);
#18079=VECTOR('',#65433,10.);
#18080=VECTOR('',#65436,10.);
#18081=VECTOR('',#65437,10.);
#18082=VECTOR('',#65438,10.);
#18083=VECTOR('',#65441,10.);
#18084=VECTOR('',#65442,10.);
#18085=VECTOR('',#65443,10.);
#18086=VECTOR('',#65446,10.);
#18087=VECTOR('',#65447,10.);
#18088=VECTOR('',#65452,10.);
#18089=VECTOR('',#65453,10.);
#18090=VECTOR('',#65454,10.);
#18091=VECTOR('',#65455,10.);
#18092=VECTOR('',#65458,10.);
#18093=VECTOR('',#65459,10.);
#18094=VECTOR('',#65460,10.);
#18095=VECTOR('',#65463,10.);
#18096=VECTOR('',#65464,10.);
#18097=VECTOR('',#65465,10.);
#18098=VECTOR('',#65468,10.);
#18099=VECTOR('',#65469,10.);
#18100=VECTOR('',#65474,10.);
#18101=VECTOR('',#65475,10.);
#18102=VECTOR('',#65476,10.);
#18103=VECTOR('',#65477,10.);
#18104=VECTOR('',#65480,10.);
#18105=VECTOR('',#65481,10.);
#18106=VECTOR('',#65482,10.);
#18107=VECTOR('',#65485,10.);
#18108=VECTOR('',#65486,10.);
#18109=VECTOR('',#65487,10.);
#18110=VECTOR('',#65490,10.);
#18111=VECTOR('',#65491,10.);
#18112=VECTOR('',#65496,10.);
#18113=VECTOR('',#65497,10.);
#18114=VECTOR('',#65498,10.);
#18115=VECTOR('',#65499,10.);
#18116=VECTOR('',#65502,10.);
#18117=VECTOR('',#65503,10.);
#18118=VECTOR('',#65504,10.);
#18119=VECTOR('',#65507,10.);
#18120=VECTOR('',#65508,10.);
#18121=VECTOR('',#65509,10.);
#18122=VECTOR('',#65512,10.);
#18123=VECTOR('',#65513,10.);
#18124=VECTOR('',#65518,10.);
#18125=VECTOR('',#65519,10.);
#18126=VECTOR('',#65520,10.);
#18127=VECTOR('',#65521,10.);
#18128=VECTOR('',#65524,10.);
#18129=VECTOR('',#65525,10.);
#18130=VECTOR('',#65526,10.);
#18131=VECTOR('',#65529,10.);
#18132=VECTOR('',#65530,10.);
#18133=VECTOR('',#65531,10.);
#18134=VECTOR('',#65534,10.);
#18135=VECTOR('',#65535,10.);
#18136=VECTOR('',#65540,10.);
#18137=VECTOR('',#65541,10.);
#18138=VECTOR('',#65542,10.);
#18139=VECTOR('',#65543,10.);
#18140=VECTOR('',#65546,10.);
#18141=VECTOR('',#65547,10.);
#18142=VECTOR('',#65548,10.);
#18143=VECTOR('',#65551,10.);
#18144=VECTOR('',#65552,10.);
#18145=VECTOR('',#65553,10.);
#18146=VECTOR('',#65556,10.);
#18147=VECTOR('',#65557,10.);
#18148=VECTOR('',#65562,10.);
#18149=VECTOR('',#65563,10.);
#18150=VECTOR('',#65564,10.);
#18151=VECTOR('',#65565,10.);
#18152=VECTOR('',#65568,10.);
#18153=VECTOR('',#65569,10.);
#18154=VECTOR('',#65570,10.);
#18155=VECTOR('',#65573,10.);
#18156=VECTOR('',#65574,10.);
#18157=VECTOR('',#65575,10.);
#18158=VECTOR('',#65578,10.);
#18159=VECTOR('',#65579,10.);
#18160=VECTOR('',#65584,10.);
#18161=VECTOR('',#65585,10.);
#18162=VECTOR('',#65586,10.);
#18163=VECTOR('',#65587,10.);
#18164=VECTOR('',#65590,10.);
#18165=VECTOR('',#65591,10.);
#18166=VECTOR('',#65592,10.);
#18167=VECTOR('',#65595,10.);
#18168=VECTOR('',#65596,10.);
#18169=VECTOR('',#65597,10.);
#18170=VECTOR('',#65600,10.);
#18171=VECTOR('',#65601,10.);
#18172=VECTOR('',#65606,10.);
#18173=VECTOR('',#65607,10.);
#18174=VECTOR('',#65608,10.);
#18175=VECTOR('',#65609,10.);
#18176=VECTOR('',#65612,10.);
#18177=VECTOR('',#65613,10.);
#18178=VECTOR('',#65614,10.);
#18179=VECTOR('',#65617,10.);
#18180=VECTOR('',#65618,10.);
#18181=VECTOR('',#65619,10.);
#18182=VECTOR('',#65622,10.);
#18183=VECTOR('',#65623,10.);
#18184=VECTOR('',#65628,10.);
#18185=VECTOR('',#65629,10.);
#18186=VECTOR('',#65630,10.);
#18187=VECTOR('',#65631,10.);
#18188=VECTOR('',#65634,10.);
#18189=VECTOR('',#65635,10.);
#18190=VECTOR('',#65636,10.);
#18191=VECTOR('',#65639,10.);
#18192=VECTOR('',#65640,10.);
#18193=VECTOR('',#65641,10.);
#18194=VECTOR('',#65644,10.);
#18195=VECTOR('',#65645,10.);
#18196=VECTOR('',#65650,10.);
#18197=VECTOR('',#65651,10.);
#18198=VECTOR('',#65652,10.);
#18199=VECTOR('',#65653,10.);
#18200=VECTOR('',#65656,10.);
#18201=VECTOR('',#65657,10.);
#18202=VECTOR('',#65658,10.);
#18203=VECTOR('',#65661,10.);
#18204=VECTOR('',#65662,10.);
#18205=VECTOR('',#65663,10.);
#18206=VECTOR('',#65666,10.);
#18207=VECTOR('',#65667,10.);
#18208=VECTOR('',#65672,10.);
#18209=VECTOR('',#65673,10.);
#18210=VECTOR('',#65674,10.);
#18211=VECTOR('',#65675,10.);
#18212=VECTOR('',#65678,10.);
#18213=VECTOR('',#65679,10.);
#18214=VECTOR('',#65680,10.);
#18215=VECTOR('',#65683,10.);
#18216=VECTOR('',#65684,10.);
#18217=VECTOR('',#65685,10.);
#18218=VECTOR('',#65688,10.);
#18219=VECTOR('',#65689,10.);
#18220=VECTOR('',#65694,10.);
#18221=VECTOR('',#65695,10.);
#18222=VECTOR('',#65696,10.);
#18223=VECTOR('',#65697,10.);
#18224=VECTOR('',#65700,10.);
#18225=VECTOR('',#65701,10.);
#18226=VECTOR('',#65702,10.);
#18227=VECTOR('',#65705,10.);
#18228=VECTOR('',#65706,10.);
#18229=VECTOR('',#65707,10.);
#18230=VECTOR('',#65710,10.);
#18231=VECTOR('',#65711,10.);
#18232=VECTOR('',#65716,10.);
#18233=VECTOR('',#65717,10.);
#18234=VECTOR('',#65718,10.);
#18235=VECTOR('',#65719,10.);
#18236=VECTOR('',#65722,10.);
#18237=VECTOR('',#65723,10.);
#18238=VECTOR('',#65724,10.);
#18239=VECTOR('',#65727,10.);
#18240=VECTOR('',#65728,10.);
#18241=VECTOR('',#65729,10.);
#18242=VECTOR('',#65732,10.);
#18243=VECTOR('',#65733,10.);
#18244=VECTOR('',#65738,10.);
#18245=VECTOR('',#65739,10.);
#18246=VECTOR('',#65740,10.);
#18247=VECTOR('',#65741,10.);
#18248=VECTOR('',#65744,10.);
#18249=VECTOR('',#65745,10.);
#18250=VECTOR('',#65746,10.);
#18251=VECTOR('',#65749,10.);
#18252=VECTOR('',#65750,10.);
#18253=VECTOR('',#65751,10.);
#18254=VECTOR('',#65754,10.);
#18255=VECTOR('',#65755,10.);
#18256=VECTOR('',#65760,10.);
#18257=VECTOR('',#65761,10.);
#18258=VECTOR('',#65762,10.);
#18259=VECTOR('',#65763,10.);
#18260=VECTOR('',#65766,10.);
#18261=VECTOR('',#65767,10.);
#18262=VECTOR('',#65768,10.);
#18263=VECTOR('',#65771,10.);
#18264=VECTOR('',#65772,10.);
#18265=VECTOR('',#65773,10.);
#18266=VECTOR('',#65776,10.);
#18267=VECTOR('',#65777,10.);
#18268=VECTOR('',#65782,10.);
#18269=VECTOR('',#65783,10.);
#18270=VECTOR('',#65784,10.);
#18271=VECTOR('',#65785,10.);
#18272=VECTOR('',#65788,10.);
#18273=VECTOR('',#65789,10.);
#18274=VECTOR('',#65790,10.);
#18275=VECTOR('',#65793,10.);
#18276=VECTOR('',#65794,10.);
#18277=VECTOR('',#65795,10.);
#18278=VECTOR('',#65798,10.);
#18279=VECTOR('',#65799,10.);
#18280=VECTOR('',#65804,10.);
#18281=VECTOR('',#65805,10.);
#18282=VECTOR('',#65806,10.);
#18283=VECTOR('',#65807,10.);
#18284=VECTOR('',#65810,10.);
#18285=VECTOR('',#65811,10.);
#18286=VECTOR('',#65812,10.);
#18287=VECTOR('',#65815,10.);
#18288=VECTOR('',#65816,10.);
#18289=VECTOR('',#65817,10.);
#18290=VECTOR('',#65820,10.);
#18291=VECTOR('',#65821,10.);
#18292=VECTOR('',#65826,10.);
#18293=VECTOR('',#65827,10.);
#18294=VECTOR('',#65828,10.);
#18295=VECTOR('',#65829,10.);
#18296=VECTOR('',#65832,10.);
#18297=VECTOR('',#65833,10.);
#18298=VECTOR('',#65834,10.);
#18299=VECTOR('',#65837,10.);
#18300=VECTOR('',#65838,10.);
#18301=VECTOR('',#65839,10.);
#18302=VECTOR('',#65842,10.);
#18303=VECTOR('',#65843,10.);
#18304=VECTOR('',#65848,10.);
#18305=VECTOR('',#65849,10.);
#18306=VECTOR('',#65850,10.);
#18307=VECTOR('',#65851,10.);
#18308=VECTOR('',#65854,10.);
#18309=VECTOR('',#65855,10.);
#18310=VECTOR('',#65856,10.);
#18311=VECTOR('',#65859,10.);
#18312=VECTOR('',#65860,10.);
#18313=VECTOR('',#65861,10.);
#18314=VECTOR('',#65864,10.);
#18315=VECTOR('',#65865,10.);
#18316=VECTOR('',#65870,10.);
#18317=VECTOR('',#65871,10.);
#18318=VECTOR('',#65872,10.);
#18319=VECTOR('',#65873,10.);
#18320=VECTOR('',#65876,10.);
#18321=VECTOR('',#65877,10.);
#18322=VECTOR('',#65878,10.);
#18323=VECTOR('',#65881,10.);
#18324=VECTOR('',#65882,10.);
#18325=VECTOR('',#65883,10.);
#18326=VECTOR('',#65886,10.);
#18327=VECTOR('',#65887,10.);
#18328=VECTOR('',#65892,10.);
#18329=VECTOR('',#65893,10.);
#18330=VECTOR('',#65894,10.);
#18331=VECTOR('',#65895,10.);
#18332=VECTOR('',#65898,10.);
#18333=VECTOR('',#65899,10.);
#18334=VECTOR('',#65900,10.);
#18335=VECTOR('',#65903,10.);
#18336=VECTOR('',#65904,10.);
#18337=VECTOR('',#65905,10.);
#18338=VECTOR('',#65908,10.);
#18339=VECTOR('',#65909,10.);
#18340=VECTOR('',#65914,10.);
#18341=VECTOR('',#65915,10.);
#18342=VECTOR('',#65916,10.);
#18343=VECTOR('',#65917,10.);
#18344=VECTOR('',#65920,10.);
#18345=VECTOR('',#65921,10.);
#18346=VECTOR('',#65922,10.);
#18347=VECTOR('',#65925,10.);
#18348=VECTOR('',#65926,10.);
#18349=VECTOR('',#65927,10.);
#18350=VECTOR('',#65930,10.);
#18351=VECTOR('',#65931,10.);
#18352=VECTOR('',#65936,10.);
#18353=VECTOR('',#65937,10.);
#18354=VECTOR('',#65938,10.);
#18355=VECTOR('',#65939,10.);
#18356=VECTOR('',#65942,10.);
#18357=VECTOR('',#65943,10.);
#18358=VECTOR('',#65944,10.);
#18359=VECTOR('',#65947,10.);
#18360=VECTOR('',#65948,10.);
#18361=VECTOR('',#65949,10.);
#18362=VECTOR('',#65952,10.);
#18363=VECTOR('',#65953,10.);
#18364=VECTOR('',#65958,10.);
#18365=VECTOR('',#65959,10.);
#18366=VECTOR('',#65960,10.);
#18367=VECTOR('',#65961,10.);
#18368=VECTOR('',#65964,10.);
#18369=VECTOR('',#65965,10.);
#18370=VECTOR('',#65966,10.);
#18371=VECTOR('',#65969,10.);
#18372=VECTOR('',#65970,10.);
#18373=VECTOR('',#65971,10.);
#18374=VECTOR('',#65974,10.);
#18375=VECTOR('',#65975,10.);
#18376=VECTOR('',#65980,10.);
#18377=VECTOR('',#65981,10.);
#18378=VECTOR('',#65982,10.);
#18379=VECTOR('',#65983,10.);
#18380=VECTOR('',#65986,10.);
#18381=VECTOR('',#65987,10.);
#18382=VECTOR('',#65988,10.);
#18383=VECTOR('',#65991,10.);
#18384=VECTOR('',#65992,10.);
#18385=VECTOR('',#65993,10.);
#18386=VECTOR('',#65996,10.);
#18387=VECTOR('',#65997,10.);
#18388=VECTOR('',#66002,10.);
#18389=VECTOR('',#66003,10.);
#18390=VECTOR('',#66004,10.);
#18391=VECTOR('',#66005,10.);
#18392=VECTOR('',#66008,10.);
#18393=VECTOR('',#66009,10.);
#18394=VECTOR('',#66010,10.);
#18395=VECTOR('',#66013,10.);
#18396=VECTOR('',#66014,10.);
#18397=VECTOR('',#66015,10.);
#18398=VECTOR('',#66018,10.);
#18399=VECTOR('',#66019,10.);
#18400=VECTOR('',#66024,10.);
#18401=VECTOR('',#66025,10.);
#18402=VECTOR('',#66026,10.);
#18403=VECTOR('',#66027,10.);
#18404=VECTOR('',#66030,10.);
#18405=VECTOR('',#66031,10.);
#18406=VECTOR('',#66032,10.);
#18407=VECTOR('',#66035,10.);
#18408=VECTOR('',#66036,10.);
#18409=VECTOR('',#66037,10.);
#18410=VECTOR('',#66040,10.);
#18411=VECTOR('',#66041,10.);
#18412=VECTOR('',#66046,10.);
#18413=VECTOR('',#66047,10.);
#18414=VECTOR('',#66048,10.);
#18415=VECTOR('',#66049,10.);
#18416=VECTOR('',#66052,10.);
#18417=VECTOR('',#66053,10.);
#18418=VECTOR('',#66054,10.);
#18419=VECTOR('',#66057,10.);
#18420=VECTOR('',#66058,10.);
#18421=VECTOR('',#66059,10.);
#18422=VECTOR('',#66062,10.);
#18423=VECTOR('',#66063,10.);
#18424=VECTOR('',#66068,10.);
#18425=VECTOR('',#66069,10.);
#18426=VECTOR('',#66070,10.);
#18427=VECTOR('',#66071,10.);
#18428=VECTOR('',#66074,10.);
#18429=VECTOR('',#66075,10.);
#18430=VECTOR('',#66076,10.);
#18431=VECTOR('',#66079,10.);
#18432=VECTOR('',#66080,10.);
#18433=VECTOR('',#66081,10.);
#18434=VECTOR('',#66084,10.);
#18435=VECTOR('',#66085,10.);
#18436=VECTOR('',#66090,10.);
#18437=VECTOR('',#66091,10.);
#18438=VECTOR('',#66092,10.);
#18439=VECTOR('',#66093,10.);
#18440=VECTOR('',#66096,10.);
#18441=VECTOR('',#66097,10.);
#18442=VECTOR('',#66098,10.);
#18443=VECTOR('',#66101,10.);
#18444=VECTOR('',#66102,10.);
#18445=VECTOR('',#66103,10.);
#18446=VECTOR('',#66106,10.);
#18447=VECTOR('',#66107,10.);
#18448=VECTOR('',#66112,10.);
#18449=VECTOR('',#66113,10.);
#18450=VECTOR('',#66114,10.);
#18451=VECTOR('',#66115,10.);
#18452=VECTOR('',#66118,10.);
#18453=VECTOR('',#66119,10.);
#18454=VECTOR('',#66120,10.);
#18455=VECTOR('',#66123,10.);
#18456=VECTOR('',#66124,10.);
#18457=VECTOR('',#66125,10.);
#18458=VECTOR('',#66128,10.);
#18459=VECTOR('',#66129,10.);
#18460=VECTOR('',#66134,10.);
#18461=VECTOR('',#66135,10.);
#18462=VECTOR('',#66136,10.);
#18463=VECTOR('',#66137,10.);
#18464=VECTOR('',#66140,10.);
#18465=VECTOR('',#66141,10.);
#18466=VECTOR('',#66142,10.);
#18467=VECTOR('',#66145,10.);
#18468=VECTOR('',#66146,10.);
#18469=VECTOR('',#66147,10.);
#18470=VECTOR('',#66150,10.);
#18471=VECTOR('',#66151,10.);
#18472=VECTOR('',#66156,10.);
#18473=VECTOR('',#66157,10.);
#18474=VECTOR('',#66158,10.);
#18475=VECTOR('',#66159,10.);
#18476=VECTOR('',#66162,10.);
#18477=VECTOR('',#66163,10.);
#18478=VECTOR('',#66164,10.);
#18479=VECTOR('',#66167,10.);
#18480=VECTOR('',#66168,10.);
#18481=VECTOR('',#66169,10.);
#18482=VECTOR('',#66172,10.);
#18483=VECTOR('',#66173,10.);
#18484=VECTOR('',#66178,10.);
#18485=VECTOR('',#66179,10.);
#18486=VECTOR('',#66180,10.);
#18487=VECTOR('',#66181,10.);
#18488=VECTOR('',#66184,10.);
#18489=VECTOR('',#66185,10.);
#18490=VECTOR('',#66186,10.);
#18491=VECTOR('',#66189,10.);
#18492=VECTOR('',#66190,10.);
#18493=VECTOR('',#66191,10.);
#18494=VECTOR('',#66194,10.);
#18495=VECTOR('',#66195,10.);
#18496=VECTOR('',#66200,10.);
#18497=VECTOR('',#66201,10.);
#18498=VECTOR('',#66202,10.);
#18499=VECTOR('',#66203,10.);
#18500=VECTOR('',#66206,10.);
#18501=VECTOR('',#66207,10.);
#18502=VECTOR('',#66208,10.);
#18503=VECTOR('',#66211,10.);
#18504=VECTOR('',#66212,10.);
#18505=VECTOR('',#66213,10.);
#18506=VECTOR('',#66216,10.);
#18507=VECTOR('',#66217,10.);
#18508=VECTOR('',#66222,10.);
#18509=VECTOR('',#66223,10.);
#18510=VECTOR('',#66224,10.);
#18511=VECTOR('',#66225,10.);
#18512=VECTOR('',#66228,10.);
#18513=VECTOR('',#66229,10.);
#18514=VECTOR('',#66230,10.);
#18515=VECTOR('',#66233,10.);
#18516=VECTOR('',#66234,10.);
#18517=VECTOR('',#66235,10.);
#18518=VECTOR('',#66238,10.);
#18519=VECTOR('',#66239,10.);
#18520=VECTOR('',#66244,10.);
#18521=VECTOR('',#66245,10.);
#18522=VECTOR('',#66246,10.);
#18523=VECTOR('',#66247,10.);
#18524=VECTOR('',#66250,10.);
#18525=VECTOR('',#66251,10.);
#18526=VECTOR('',#66252,10.);
#18527=VECTOR('',#66255,10.);
#18528=VECTOR('',#66256,10.);
#18529=VECTOR('',#66257,10.);
#18530=VECTOR('',#66260,10.);
#18531=VECTOR('',#66261,10.);
#18532=VECTOR('',#66266,10.);
#18533=VECTOR('',#66267,10.);
#18534=VECTOR('',#66268,10.);
#18535=VECTOR('',#66269,10.);
#18536=VECTOR('',#66272,10.);
#18537=VECTOR('',#66273,10.);
#18538=VECTOR('',#66274,10.);
#18539=VECTOR('',#66277,10.);
#18540=VECTOR('',#66278,10.);
#18541=VECTOR('',#66279,10.);
#18542=VECTOR('',#66282,10.);
#18543=VECTOR('',#66283,10.);
#18544=VECTOR('',#66288,10.);
#18545=VECTOR('',#66289,10.);
#18546=VECTOR('',#66290,10.);
#18547=VECTOR('',#66291,10.);
#18548=VECTOR('',#66294,10.);
#18549=VECTOR('',#66295,10.);
#18550=VECTOR('',#66296,10.);
#18551=VECTOR('',#66299,10.);
#18552=VECTOR('',#66300,10.);
#18553=VECTOR('',#66301,10.);
#18554=VECTOR('',#66304,10.);
#18555=VECTOR('',#66305,10.);
#18556=VECTOR('',#66310,10.);
#18557=VECTOR('',#66311,10.);
#18558=VECTOR('',#66312,10.);
#18559=VECTOR('',#66313,10.);
#18560=VECTOR('',#66316,10.);
#18561=VECTOR('',#66317,10.);
#18562=VECTOR('',#66318,10.);
#18563=VECTOR('',#66321,10.);
#18564=VECTOR('',#66322,10.);
#18565=VECTOR('',#66323,10.);
#18566=VECTOR('',#66326,10.);
#18567=VECTOR('',#66327,10.);
#18568=VECTOR('',#66332,10.);
#18569=VECTOR('',#66333,10.);
#18570=VECTOR('',#66334,10.);
#18571=VECTOR('',#66335,10.);
#18572=VECTOR('',#66338,10.);
#18573=VECTOR('',#66339,10.);
#18574=VECTOR('',#66340,10.);
#18575=VECTOR('',#66343,10.);
#18576=VECTOR('',#66344,10.);
#18577=VECTOR('',#66345,10.);
#18578=VECTOR('',#66348,10.);
#18579=VECTOR('',#66349,10.);
#18580=VECTOR('',#66354,10.);
#18581=VECTOR('',#66355,10.);
#18582=VECTOR('',#66356,10.);
#18583=VECTOR('',#66357,10.);
#18584=VECTOR('',#66360,10.);
#18585=VECTOR('',#66361,10.);
#18586=VECTOR('',#66362,10.);
#18587=VECTOR('',#66365,10.);
#18588=VECTOR('',#66366,10.);
#18589=VECTOR('',#66367,10.);
#18590=VECTOR('',#66370,10.);
#18591=VECTOR('',#66371,10.);
#18592=VECTOR('',#66376,10.);
#18593=VECTOR('',#66377,10.);
#18594=VECTOR('',#66378,10.);
#18595=VECTOR('',#66379,10.);
#18596=VECTOR('',#66382,10.);
#18597=VECTOR('',#66383,10.);
#18598=VECTOR('',#66384,10.);
#18599=VECTOR('',#66387,10.);
#18600=VECTOR('',#66388,10.);
#18601=VECTOR('',#66389,10.);
#18602=VECTOR('',#66392,10.);
#18603=VECTOR('',#66393,10.);
#18604=VECTOR('',#66398,10.);
#18605=VECTOR('',#66399,10.);
#18606=VECTOR('',#66400,10.);
#18607=VECTOR('',#66401,10.);
#18608=VECTOR('',#66404,10.);
#18609=VECTOR('',#66405,10.);
#18610=VECTOR('',#66406,10.);
#18611=VECTOR('',#66409,10.);
#18612=VECTOR('',#66410,10.);
#18613=VECTOR('',#66411,10.);
#18614=VECTOR('',#66414,10.);
#18615=VECTOR('',#66415,10.);
#18616=VECTOR('',#66420,10.);
#18617=VECTOR('',#66421,10.);
#18618=VECTOR('',#66422,10.);
#18619=VECTOR('',#66423,10.);
#18620=VECTOR('',#66426,10.);
#18621=VECTOR('',#66427,10.);
#18622=VECTOR('',#66428,10.);
#18623=VECTOR('',#66431,10.);
#18624=VECTOR('',#66432,10.);
#18625=VECTOR('',#66433,10.);
#18626=VECTOR('',#66436,10.);
#18627=VECTOR('',#66437,10.);
#18628=VECTOR('',#66442,10.);
#18629=VECTOR('',#66443,10.);
#18630=VECTOR('',#66444,10.);
#18631=VECTOR('',#66445,10.);
#18632=VECTOR('',#66448,10.);
#18633=VECTOR('',#66449,10.);
#18634=VECTOR('',#66450,10.);
#18635=VECTOR('',#66453,10.);
#18636=VECTOR('',#66454,10.);
#18637=VECTOR('',#66455,10.);
#18638=VECTOR('',#66458,10.);
#18639=VECTOR('',#66459,10.);
#18640=VECTOR('',#66464,10.);
#18641=VECTOR('',#66465,10.);
#18642=VECTOR('',#66466,10.);
#18643=VECTOR('',#66467,10.);
#18644=VECTOR('',#66470,10.);
#18645=VECTOR('',#66471,10.);
#18646=VECTOR('',#66472,10.);
#18647=VECTOR('',#66475,10.);
#18648=VECTOR('',#66476,10.);
#18649=VECTOR('',#66477,10.);
#18650=VECTOR('',#66480,10.);
#18651=VECTOR('',#66481,10.);
#18652=VECTOR('',#66486,10.);
#18653=VECTOR('',#66487,10.);
#18654=VECTOR('',#66488,10.);
#18655=VECTOR('',#66489,10.);
#18656=VECTOR('',#66492,10.);
#18657=VECTOR('',#66493,10.);
#18658=VECTOR('',#66494,10.);
#18659=VECTOR('',#66497,10.);
#18660=VECTOR('',#66498,10.);
#18661=VECTOR('',#66499,10.);
#18662=VECTOR('',#66502,10.);
#18663=VECTOR('',#66503,10.);
#18664=VECTOR('',#66508,10.);
#18665=VECTOR('',#66509,10.);
#18666=VECTOR('',#66510,10.);
#18667=VECTOR('',#66511,10.);
#18668=VECTOR('',#66514,10.);
#18669=VECTOR('',#66515,10.);
#18670=VECTOR('',#66516,10.);
#18671=VECTOR('',#66519,10.);
#18672=VECTOR('',#66520,10.);
#18673=VECTOR('',#66521,10.);
#18674=VECTOR('',#66524,10.);
#18675=VECTOR('',#66525,10.);
#18676=VECTOR('',#66530,10.);
#18677=VECTOR('',#66531,10.);
#18678=VECTOR('',#66532,10.);
#18679=VECTOR('',#66533,10.);
#18680=VECTOR('',#66536,10.);
#18681=VECTOR('',#66537,10.);
#18682=VECTOR('',#66538,10.);
#18683=VECTOR('',#66541,10.);
#18684=VECTOR('',#66542,10.);
#18685=VECTOR('',#66543,10.);
#18686=VECTOR('',#66546,10.);
#18687=VECTOR('',#66547,10.);
#18688=VECTOR('',#66552,10.);
#18689=VECTOR('',#66553,10.);
#18690=VECTOR('',#66554,10.);
#18691=VECTOR('',#66555,10.);
#18692=VECTOR('',#66558,10.);
#18693=VECTOR('',#66559,10.);
#18694=VECTOR('',#66560,10.);
#18695=VECTOR('',#66563,10.);
#18696=VECTOR('',#66564,10.);
#18697=VECTOR('',#66565,10.);
#18698=VECTOR('',#66568,10.);
#18699=VECTOR('',#66569,10.);
#18700=VECTOR('',#66574,10.);
#18701=VECTOR('',#66575,10.);
#18702=VECTOR('',#66576,10.);
#18703=VECTOR('',#66577,10.);
#18704=VECTOR('',#66580,10.);
#18705=VECTOR('',#66581,10.);
#18706=VECTOR('',#66582,10.);
#18707=VECTOR('',#66585,10.);
#18708=VECTOR('',#66586,10.);
#18709=VECTOR('',#66587,10.);
#18710=VECTOR('',#66590,10.);
#18711=VECTOR('',#66591,10.);
#18712=VECTOR('',#66596,10.);
#18713=VECTOR('',#66597,10.);
#18714=VECTOR('',#66598,10.);
#18715=VECTOR('',#66599,10.);
#18716=VECTOR('',#66602,10.);
#18717=VECTOR('',#66603,10.);
#18718=VECTOR('',#66604,10.);
#18719=VECTOR('',#66607,10.);
#18720=VECTOR('',#66608,10.);
#18721=VECTOR('',#66609,10.);
#18722=VECTOR('',#66612,10.);
#18723=VECTOR('',#66613,10.);
#18724=VECTOR('',#66618,10.);
#18725=VECTOR('',#66619,10.);
#18726=VECTOR('',#66620,10.);
#18727=VECTOR('',#66621,10.);
#18728=VECTOR('',#66624,10.);
#18729=VECTOR('',#66625,10.);
#18730=VECTOR('',#66626,10.);
#18731=VECTOR('',#66629,10.);
#18732=VECTOR('',#66630,10.);
#18733=VECTOR('',#66631,10.);
#18734=VECTOR('',#66634,10.);
#18735=VECTOR('',#66635,10.);
#18736=VECTOR('',#66640,10.);
#18737=VECTOR('',#66641,10.);
#18738=VECTOR('',#66642,10.);
#18739=VECTOR('',#66643,10.);
#18740=VECTOR('',#66646,10.);
#18741=VECTOR('',#66647,10.);
#18742=VECTOR('',#66648,10.);
#18743=VECTOR('',#66651,10.);
#18744=VECTOR('',#66652,10.);
#18745=VECTOR('',#66653,10.);
#18746=VECTOR('',#66656,10.);
#18747=VECTOR('',#66657,10.);
#18748=VECTOR('',#66662,10.);
#18749=VECTOR('',#66663,10.);
#18750=VECTOR('',#66664,10.);
#18751=VECTOR('',#66665,10.);
#18752=VECTOR('',#66668,10.);
#18753=VECTOR('',#66669,10.);
#18754=VECTOR('',#66670,10.);
#18755=VECTOR('',#66673,10.);
#18756=VECTOR('',#66674,10.);
#18757=VECTOR('',#66675,10.);
#18758=VECTOR('',#66678,10.);
#18759=VECTOR('',#66679,10.);
#18760=VECTOR('',#66684,10.);
#18761=VECTOR('',#66685,10.);
#18762=VECTOR('',#66686,10.);
#18763=VECTOR('',#66687,10.);
#18764=VECTOR('',#66690,10.);
#18765=VECTOR('',#66691,10.);
#18766=VECTOR('',#66692,10.);
#18767=VECTOR('',#66695,10.);
#18768=VECTOR('',#66696,10.);
#18769=VECTOR('',#66697,10.);
#18770=VECTOR('',#66700,10.);
#18771=VECTOR('',#66701,10.);
#18772=VECTOR('',#66706,10.);
#18773=VECTOR('',#66707,10.);
#18774=VECTOR('',#66708,10.);
#18775=VECTOR('',#66709,10.);
#18776=VECTOR('',#66712,10.);
#18777=VECTOR('',#66713,10.);
#18778=VECTOR('',#66714,10.);
#18779=VECTOR('',#66717,10.);
#18780=VECTOR('',#66718,10.);
#18781=VECTOR('',#66719,10.);
#18782=VECTOR('',#66722,10.);
#18783=VECTOR('',#66723,10.);
#18784=VECTOR('',#66728,10.);
#18785=VECTOR('',#66729,10.);
#18786=VECTOR('',#66730,10.);
#18787=VECTOR('',#66731,10.);
#18788=VECTOR('',#66734,10.);
#18789=VECTOR('',#66735,10.);
#18790=VECTOR('',#66736,10.);
#18791=VECTOR('',#66739,10.);
#18792=VECTOR('',#66740,10.);
#18793=VECTOR('',#66741,10.);
#18794=VECTOR('',#66744,10.);
#18795=VECTOR('',#66745,10.);
#18796=VECTOR('',#66750,10.);
#18797=VECTOR('',#66751,10.);
#18798=VECTOR('',#66752,10.);
#18799=VECTOR('',#66753,10.);
#18800=VECTOR('',#66756,10.);
#18801=VECTOR('',#66757,10.);
#18802=VECTOR('',#66758,10.);
#18803=VECTOR('',#66761,10.);
#18804=VECTOR('',#66762,10.);
#18805=VECTOR('',#66763,10.);
#18806=VECTOR('',#66766,10.);
#18807=VECTOR('',#66767,10.);
#18808=VECTOR('',#66772,10.);
#18809=VECTOR('',#66773,10.);
#18810=VECTOR('',#66774,10.);
#18811=VECTOR('',#66775,10.);
#18812=VECTOR('',#66778,10.);
#18813=VECTOR('',#66779,10.);
#18814=VECTOR('',#66780,10.);
#18815=VECTOR('',#66783,10.);
#18816=VECTOR('',#66784,10.);
#18817=VECTOR('',#66785,10.);
#18818=VECTOR('',#66788,10.);
#18819=VECTOR('',#66789,10.);
#18820=VECTOR('',#66794,10.);
#18821=VECTOR('',#66795,10.);
#18822=VECTOR('',#66796,10.);
#18823=VECTOR('',#66797,10.);
#18824=VECTOR('',#66800,10.);
#18825=VECTOR('',#66801,10.);
#18826=VECTOR('',#66802,10.);
#18827=VECTOR('',#66805,10.);
#18828=VECTOR('',#66806,10.);
#18829=VECTOR('',#66807,10.);
#18830=VECTOR('',#66810,10.);
#18831=VECTOR('',#66811,10.);
#18832=VECTOR('',#66816,10.);
#18833=VECTOR('',#66817,10.);
#18834=VECTOR('',#66818,10.);
#18835=VECTOR('',#66819,10.);
#18836=VECTOR('',#66822,10.);
#18837=VECTOR('',#66823,10.);
#18838=VECTOR('',#66824,10.);
#18839=VECTOR('',#66827,10.);
#18840=VECTOR('',#66828,10.);
#18841=VECTOR('',#66829,10.);
#18842=VECTOR('',#66832,10.);
#18843=VECTOR('',#66833,10.);
#18844=VECTOR('',#66838,10.);
#18845=VECTOR('',#66839,10.);
#18846=VECTOR('',#66840,10.);
#18847=VECTOR('',#66841,10.);
#18848=VECTOR('',#66844,10.);
#18849=VECTOR('',#66845,10.);
#18850=VECTOR('',#66846,10.);
#18851=VECTOR('',#66849,10.);
#18852=VECTOR('',#66850,10.);
#18853=VECTOR('',#66851,10.);
#18854=VECTOR('',#66854,10.);
#18855=VECTOR('',#66855,10.);
#18856=VECTOR('',#66860,10.);
#18857=VECTOR('',#66861,10.);
#18858=VECTOR('',#66862,10.);
#18859=VECTOR('',#66863,10.);
#18860=VECTOR('',#66866,10.);
#18861=VECTOR('',#66867,10.);
#18862=VECTOR('',#66868,10.);
#18863=VECTOR('',#66871,10.);
#18864=VECTOR('',#66872,10.);
#18865=VECTOR('',#66873,10.);
#18866=VECTOR('',#66876,10.);
#18867=VECTOR('',#66877,10.);
#18868=VECTOR('',#66882,10.);
#18869=VECTOR('',#66883,10.);
#18870=VECTOR('',#66884,10.);
#18871=VECTOR('',#66885,10.);
#18872=VECTOR('',#66888,10.);
#18873=VECTOR('',#66889,10.);
#18874=VECTOR('',#66890,10.);
#18875=VECTOR('',#66893,10.);
#18876=VECTOR('',#66894,10.);
#18877=VECTOR('',#66895,10.);
#18878=VECTOR('',#66898,10.);
#18879=VECTOR('',#66899,10.);
#18880=VECTOR('',#66904,10.);
#18881=VECTOR('',#66905,10.);
#18882=VECTOR('',#66906,10.);
#18883=VECTOR('',#66907,10.);
#18884=VECTOR('',#66910,10.);
#18885=VECTOR('',#66911,10.);
#18886=VECTOR('',#66912,10.);
#18887=VECTOR('',#66915,10.);
#18888=VECTOR('',#66916,10.);
#18889=VECTOR('',#66917,10.);
#18890=VECTOR('',#66920,10.);
#18891=VECTOR('',#66921,10.);
#18892=VECTOR('',#66926,10.);
#18893=VECTOR('',#66927,10.);
#18894=VECTOR('',#66928,10.);
#18895=VECTOR('',#66929,10.);
#18896=VECTOR('',#66932,10.);
#18897=VECTOR('',#66933,10.);
#18898=VECTOR('',#66934,10.);
#18899=VECTOR('',#66937,10.);
#18900=VECTOR('',#66938,10.);
#18901=VECTOR('',#66939,10.);
#18902=VECTOR('',#66942,10.);
#18903=VECTOR('',#66943,10.);
#18904=VECTOR('',#66948,10.);
#18905=VECTOR('',#66949,10.);
#18906=VECTOR('',#66950,10.);
#18907=VECTOR('',#66951,10.);
#18908=VECTOR('',#66954,10.);
#18909=VECTOR('',#66955,10.);
#18910=VECTOR('',#66956,10.);
#18911=VECTOR('',#66959,10.);
#18912=VECTOR('',#66960,10.);
#18913=VECTOR('',#66961,10.);
#18914=VECTOR('',#66964,10.);
#18915=VECTOR('',#66965,10.);
#18916=VECTOR('',#66970,10.);
#18917=VECTOR('',#66971,10.);
#18918=VECTOR('',#66972,10.);
#18919=VECTOR('',#66973,10.);
#18920=VECTOR('',#66976,10.);
#18921=VECTOR('',#66977,10.);
#18922=VECTOR('',#66978,10.);
#18923=VECTOR('',#66981,10.);
#18924=VECTOR('',#66982,10.);
#18925=VECTOR('',#66983,10.);
#18926=VECTOR('',#66986,10.);
#18927=VECTOR('',#66987,10.);
#18928=VECTOR('',#66992,10.);
#18929=VECTOR('',#66993,10.);
#18930=VECTOR('',#66994,10.);
#18931=VECTOR('',#66995,10.);
#18932=VECTOR('',#66998,10.);
#18933=VECTOR('',#66999,10.);
#18934=VECTOR('',#67000,10.);
#18935=VECTOR('',#67003,10.);
#18936=VECTOR('',#67004,10.);
#18937=VECTOR('',#67005,10.);
#18938=VECTOR('',#67008,10.);
#18939=VECTOR('',#67009,10.);
#18940=VECTOR('',#67014,10.);
#18941=VECTOR('',#67015,10.);
#18942=VECTOR('',#67016,10.);
#18943=VECTOR('',#67017,10.);
#18944=VECTOR('',#67020,10.);
#18945=VECTOR('',#67021,10.);
#18946=VECTOR('',#67022,10.);
#18947=VECTOR('',#67025,10.);
#18948=VECTOR('',#67026,10.);
#18949=VECTOR('',#67027,10.);
#18950=VECTOR('',#67030,10.);
#18951=VECTOR('',#67031,10.);
#18952=VECTOR('',#67036,10.);
#18953=VECTOR('',#67037,10.);
#18954=VECTOR('',#67038,10.);
#18955=VECTOR('',#67039,10.);
#18956=VECTOR('',#67042,10.);
#18957=VECTOR('',#67043,10.);
#18958=VECTOR('',#67044,10.);
#18959=VECTOR('',#67047,10.);
#18960=VECTOR('',#67048,10.);
#18961=VECTOR('',#67049,10.);
#18962=VECTOR('',#67052,10.);
#18963=VECTOR('',#67053,10.);
#18964=VECTOR('',#67058,10.);
#18965=VECTOR('',#67059,10.);
#18966=VECTOR('',#67060,10.);
#18967=VECTOR('',#67061,10.);
#18968=VECTOR('',#67064,10.);
#18969=VECTOR('',#67065,10.);
#18970=VECTOR('',#67066,10.);
#18971=VECTOR('',#67069,10.);
#18972=VECTOR('',#67070,10.);
#18973=VECTOR('',#67071,10.);
#18974=VECTOR('',#67074,10.);
#18975=VECTOR('',#67075,10.);
#18976=VECTOR('',#67080,10.);
#18977=VECTOR('',#67081,10.);
#18978=VECTOR('',#67082,10.);
#18979=VECTOR('',#67083,10.);
#18980=VECTOR('',#67086,10.);
#18981=VECTOR('',#67087,10.);
#18982=VECTOR('',#67088,10.);
#18983=VECTOR('',#67091,10.);
#18984=VECTOR('',#67092,10.);
#18985=VECTOR('',#67093,10.);
#18986=VECTOR('',#67096,10.);
#18987=VECTOR('',#67097,10.);
#18988=VECTOR('',#67102,10.);
#18989=VECTOR('',#67103,10.);
#18990=VECTOR('',#67104,10.);
#18991=VECTOR('',#67105,10.);
#18992=VECTOR('',#67108,10.);
#18993=VECTOR('',#67109,10.);
#18994=VECTOR('',#67110,10.);
#18995=VECTOR('',#67113,10.);
#18996=VECTOR('',#67114,10.);
#18997=VECTOR('',#67115,10.);
#18998=VECTOR('',#67118,10.);
#18999=VECTOR('',#67119,10.);
#19000=VECTOR('',#67124,10.);
#19001=VECTOR('',#67125,10.);
#19002=VECTOR('',#67126,10.);
#19003=VECTOR('',#67127,10.);
#19004=VECTOR('',#67130,10.);
#19005=VECTOR('',#67131,10.);
#19006=VECTOR('',#67132,10.);
#19007=VECTOR('',#67135,10.);
#19008=VECTOR('',#67136,10.);
#19009=VECTOR('',#67137,10.);
#19010=VECTOR('',#67140,10.);
#19011=VECTOR('',#67141,10.);
#19012=VECTOR('',#67146,10.);
#19013=VECTOR('',#67147,10.);
#19014=VECTOR('',#67148,10.);
#19015=VECTOR('',#67149,10.);
#19016=VECTOR('',#67152,10.);
#19017=VECTOR('',#67153,10.);
#19018=VECTOR('',#67154,10.);
#19019=VECTOR('',#67157,10.);
#19020=VECTOR('',#67158,10.);
#19021=VECTOR('',#67159,10.);
#19022=VECTOR('',#67162,10.);
#19023=VECTOR('',#67163,10.);
#19024=VECTOR('',#67168,10.);
#19025=VECTOR('',#67169,10.);
#19026=VECTOR('',#67170,10.);
#19027=VECTOR('',#67171,10.);
#19028=VECTOR('',#67174,10.);
#19029=VECTOR('',#67175,10.);
#19030=VECTOR('',#67176,10.);
#19031=VECTOR('',#67179,10.);
#19032=VECTOR('',#67180,10.);
#19033=VECTOR('',#67181,10.);
#19034=VECTOR('',#67184,10.);
#19035=VECTOR('',#67185,10.);
#19036=VECTOR('',#67190,10.);
#19037=VECTOR('',#67191,10.);
#19038=VECTOR('',#67192,10.);
#19039=VECTOR('',#67193,10.);
#19040=VECTOR('',#67196,10.);
#19041=VECTOR('',#67197,10.);
#19042=VECTOR('',#67198,10.);
#19043=VECTOR('',#67201,10.);
#19044=VECTOR('',#67202,10.);
#19045=VECTOR('',#67203,10.);
#19046=VECTOR('',#67206,10.);
#19047=VECTOR('',#67207,10.);
#19048=VECTOR('',#67212,10.);
#19049=VECTOR('',#67213,10.);
#19050=VECTOR('',#67214,10.);
#19051=VECTOR('',#67215,10.);
#19052=VECTOR('',#67218,10.);
#19053=VECTOR('',#67219,10.);
#19054=VECTOR('',#67220,10.);
#19055=VECTOR('',#67223,10.);
#19056=VECTOR('',#67224,10.);
#19057=VECTOR('',#67225,10.);
#19058=VECTOR('',#67228,10.);
#19059=VECTOR('',#67229,10.);
#19060=VECTOR('',#67234,10.);
#19061=VECTOR('',#67235,10.);
#19062=VECTOR('',#67236,10.);
#19063=VECTOR('',#67237,10.);
#19064=VECTOR('',#67240,10.);
#19065=VECTOR('',#67241,10.);
#19066=VECTOR('',#67242,10.);
#19067=VECTOR('',#67245,10.);
#19068=VECTOR('',#67246,10.);
#19069=VECTOR('',#67247,10.);
#19070=VECTOR('',#67250,10.);
#19071=VECTOR('',#67251,10.);
#19072=VECTOR('',#67256,10.);
#19073=VECTOR('',#67257,10.);
#19074=VECTOR('',#67258,10.);
#19075=VECTOR('',#67259,10.);
#19076=VECTOR('',#67262,10.);
#19077=VECTOR('',#67263,10.);
#19078=VECTOR('',#67264,10.);
#19079=VECTOR('',#67267,10.);
#19080=VECTOR('',#67268,10.);
#19081=VECTOR('',#67269,10.);
#19082=VECTOR('',#67272,10.);
#19083=VECTOR('',#67273,10.);
#19084=VECTOR('',#67278,10.);
#19085=VECTOR('',#67279,10.);
#19086=VECTOR('',#67280,10.);
#19087=VECTOR('',#67281,10.);
#19088=VECTOR('',#67284,10.);
#19089=VECTOR('',#67285,10.);
#19090=VECTOR('',#67286,10.);
#19091=VECTOR('',#67289,10.);
#19092=VECTOR('',#67290,10.);
#19093=VECTOR('',#67291,10.);
#19094=VECTOR('',#67294,10.);
#19095=VECTOR('',#67295,10.);
#19096=VECTOR('',#67300,10.);
#19097=VECTOR('',#67301,10.);
#19098=VECTOR('',#67302,10.);
#19099=VECTOR('',#67303,10.);
#19100=VECTOR('',#67306,10.);
#19101=VECTOR('',#67307,10.);
#19102=VECTOR('',#67308,10.);
#19103=VECTOR('',#67311,10.);
#19104=VECTOR('',#67312,10.);
#19105=VECTOR('',#67313,10.);
#19106=VECTOR('',#67316,10.);
#19107=VECTOR('',#67317,10.);
#19108=VECTOR('',#67322,10.);
#19109=VECTOR('',#67323,10.);
#19110=VECTOR('',#67324,10.);
#19111=VECTOR('',#67325,10.);
#19112=VECTOR('',#67328,10.);
#19113=VECTOR('',#67329,10.);
#19114=VECTOR('',#67330,10.);
#19115=VECTOR('',#67333,10.);
#19116=VECTOR('',#67334,10.);
#19117=VECTOR('',#67335,10.);
#19118=VECTOR('',#67338,10.);
#19119=VECTOR('',#67339,10.);
#19120=VECTOR('',#67344,10.);
#19121=VECTOR('',#67345,10.);
#19122=VECTOR('',#67346,10.);
#19123=VECTOR('',#67347,10.);
#19124=VECTOR('',#67350,10.);
#19125=VECTOR('',#67351,10.);
#19126=VECTOR('',#67352,10.);
#19127=VECTOR('',#67355,10.);
#19128=VECTOR('',#67356,10.);
#19129=VECTOR('',#67357,10.);
#19130=VECTOR('',#67360,10.);
#19131=VECTOR('',#67361,10.);
#19132=VECTOR('',#67366,10.);
#19133=VECTOR('',#67367,10.);
#19134=VECTOR('',#67368,10.);
#19135=VECTOR('',#67369,10.);
#19136=VECTOR('',#67372,10.);
#19137=VECTOR('',#67373,10.);
#19138=VECTOR('',#67374,10.);
#19139=VECTOR('',#67377,10.);
#19140=VECTOR('',#67378,10.);
#19141=VECTOR('',#67379,10.);
#19142=VECTOR('',#67382,10.);
#19143=VECTOR('',#67383,10.);
#19144=VECTOR('',#67388,10.);
#19145=VECTOR('',#67389,10.);
#19146=VECTOR('',#67390,10.);
#19147=VECTOR('',#67391,10.);
#19148=VECTOR('',#67394,10.);
#19149=VECTOR('',#67395,10.);
#19150=VECTOR('',#67396,10.);
#19151=VECTOR('',#67399,10.);
#19152=VECTOR('',#67400,10.);
#19153=VECTOR('',#67401,10.);
#19154=VECTOR('',#67404,10.);
#19155=VECTOR('',#67405,10.);
#19156=VECTOR('',#67410,10.);
#19157=VECTOR('',#67411,10.);
#19158=VECTOR('',#67412,10.);
#19159=VECTOR('',#67413,10.);
#19160=VECTOR('',#67416,10.);
#19161=VECTOR('',#67417,10.);
#19162=VECTOR('',#67418,10.);
#19163=VECTOR('',#67421,10.);
#19164=VECTOR('',#67422,10.);
#19165=VECTOR('',#67423,10.);
#19166=VECTOR('',#67426,10.);
#19167=VECTOR('',#67427,10.);
#19168=VECTOR('',#67432,10.);
#19169=VECTOR('',#67433,10.);
#19170=VECTOR('',#67434,10.);
#19171=VECTOR('',#67435,10.);
#19172=VECTOR('',#67438,10.);
#19173=VECTOR('',#67439,10.);
#19174=VECTOR('',#67440,10.);
#19175=VECTOR('',#67443,10.);
#19176=VECTOR('',#67444,10.);
#19177=VECTOR('',#67445,10.);
#19178=VECTOR('',#67448,10.);
#19179=VECTOR('',#67449,10.);
#19180=VECTOR('',#67454,10.);
#19181=VECTOR('',#67455,10.);
#19182=VECTOR('',#67456,10.);
#19183=VECTOR('',#67457,10.);
#19184=VECTOR('',#67460,10.);
#19185=VECTOR('',#67461,10.);
#19186=VECTOR('',#67462,10.);
#19187=VECTOR('',#67465,10.);
#19188=VECTOR('',#67466,10.);
#19189=VECTOR('',#67467,10.);
#19190=VECTOR('',#67470,10.);
#19191=VECTOR('',#67471,10.);
#19192=VECTOR('',#67476,10.);
#19193=VECTOR('',#67477,10.);
#19194=VECTOR('',#67478,10.);
#19195=VECTOR('',#67479,10.);
#19196=VECTOR('',#67482,10.);
#19197=VECTOR('',#67483,10.);
#19198=VECTOR('',#67484,10.);
#19199=VECTOR('',#67487,10.);
#19200=VECTOR('',#67488,10.);
#19201=VECTOR('',#67489,10.);
#19202=VECTOR('',#67492,10.);
#19203=VECTOR('',#67493,10.);
#19204=VECTOR('',#67498,10.);
#19205=VECTOR('',#67499,10.);
#19206=VECTOR('',#67500,10.);
#19207=VECTOR('',#67501,10.);
#19208=VECTOR('',#67504,10.);
#19209=VECTOR('',#67505,10.);
#19210=VECTOR('',#67506,10.);
#19211=VECTOR('',#67509,10.);
#19212=VECTOR('',#67510,10.);
#19213=VECTOR('',#67511,10.);
#19214=VECTOR('',#67514,10.);
#19215=VECTOR('',#67515,10.);
#19216=VECTOR('',#67520,10.);
#19217=VECTOR('',#67521,10.);
#19218=VECTOR('',#67522,10.);
#19219=VECTOR('',#67523,10.);
#19220=VECTOR('',#67526,10.);
#19221=VECTOR('',#67527,10.);
#19222=VECTOR('',#67528,10.);
#19223=VECTOR('',#67531,10.);
#19224=VECTOR('',#67532,10.);
#19225=VECTOR('',#67533,10.);
#19226=VECTOR('',#67536,10.);
#19227=VECTOR('',#67537,10.);
#19228=VECTOR('',#67542,10.);
#19229=VECTOR('',#67543,10.);
#19230=VECTOR('',#67544,10.);
#19231=VECTOR('',#67545,10.);
#19232=VECTOR('',#67548,10.);
#19233=VECTOR('',#67549,10.);
#19234=VECTOR('',#67550,10.);
#19235=VECTOR('',#67553,10.);
#19236=VECTOR('',#67554,10.);
#19237=VECTOR('',#67555,10.);
#19238=VECTOR('',#67558,10.);
#19239=VECTOR('',#67559,10.);
#19240=VECTOR('',#67564,10.);
#19241=VECTOR('',#67565,10.);
#19242=VECTOR('',#67566,10.);
#19243=VECTOR('',#67567,10.);
#19244=VECTOR('',#67570,10.);
#19245=VECTOR('',#67571,10.);
#19246=VECTOR('',#67572,10.);
#19247=VECTOR('',#67575,10.);
#19248=VECTOR('',#67576,10.);
#19249=VECTOR('',#67577,10.);
#19250=VECTOR('',#67580,10.);
#19251=VECTOR('',#67581,10.);
#19252=VECTOR('',#67586,10.);
#19253=VECTOR('',#67587,10.);
#19254=VECTOR('',#67588,10.);
#19255=VECTOR('',#67589,10.);
#19256=VECTOR('',#67592,10.);
#19257=VECTOR('',#67593,10.);
#19258=VECTOR('',#67594,10.);
#19259=VECTOR('',#67597,10.);
#19260=VECTOR('',#67598,10.);
#19261=VECTOR('',#67599,10.);
#19262=VECTOR('',#67602,10.);
#19263=VECTOR('',#67603,10.);
#19264=VECTOR('',#67608,10.);
#19265=VECTOR('',#67609,10.);
#19266=VECTOR('',#67610,10.);
#19267=VECTOR('',#67611,10.);
#19268=VECTOR('',#67614,10.);
#19269=VECTOR('',#67615,10.);
#19270=VECTOR('',#67616,10.);
#19271=VECTOR('',#67619,10.);
#19272=VECTOR('',#67620,10.);
#19273=VECTOR('',#67621,10.);
#19274=VECTOR('',#67624,10.);
#19275=VECTOR('',#67625,10.);
#19276=VECTOR('',#67630,10.);
#19277=VECTOR('',#67631,10.);
#19278=VECTOR('',#67632,10.);
#19279=VECTOR('',#67633,10.);
#19280=VECTOR('',#67636,10.);
#19281=VECTOR('',#67637,10.);
#19282=VECTOR('',#67638,10.);
#19283=VECTOR('',#67641,10.);
#19284=VECTOR('',#67642,10.);
#19285=VECTOR('',#67643,10.);
#19286=VECTOR('',#67646,10.);
#19287=VECTOR('',#67647,10.);
#19288=VECTOR('',#67652,10.);
#19289=VECTOR('',#67653,10.);
#19290=VECTOR('',#67654,10.);
#19291=VECTOR('',#67655,10.);
#19292=VECTOR('',#67658,10.);
#19293=VECTOR('',#67659,10.);
#19294=VECTOR('',#67660,10.);
#19295=VECTOR('',#67663,10.);
#19296=VECTOR('',#67664,10.);
#19297=VECTOR('',#67665,10.);
#19298=VECTOR('',#67668,10.);
#19299=VECTOR('',#67669,10.);
#19300=VECTOR('',#67674,10.);
#19301=VECTOR('',#67675,10.);
#19302=VECTOR('',#67676,10.);
#19303=VECTOR('',#67677,10.);
#19304=VECTOR('',#67680,10.);
#19305=VECTOR('',#67681,10.);
#19306=VECTOR('',#67682,10.);
#19307=VECTOR('',#67685,10.);
#19308=VECTOR('',#67686,10.);
#19309=VECTOR('',#67687,10.);
#19310=VECTOR('',#67690,10.);
#19311=VECTOR('',#67691,10.);
#19312=VECTOR('',#67696,10.);
#19313=VECTOR('',#67697,10.);
#19314=VECTOR('',#67698,10.);
#19315=VECTOR('',#67699,10.);
#19316=VECTOR('',#67702,10.);
#19317=VECTOR('',#67703,10.);
#19318=VECTOR('',#67704,10.);
#19319=VECTOR('',#67707,10.);
#19320=VECTOR('',#67708,10.);
#19321=VECTOR('',#67709,10.);
#19322=VECTOR('',#67712,10.);
#19323=VECTOR('',#67713,10.);
#19324=VECTOR('',#67718,10.);
#19325=VECTOR('',#67719,10.);
#19326=VECTOR('',#67720,10.);
#19327=VECTOR('',#67721,10.);
#19328=VECTOR('',#67724,10.);
#19329=VECTOR('',#67725,10.);
#19330=VECTOR('',#67726,10.);
#19331=VECTOR('',#67729,10.);
#19332=VECTOR('',#67730,10.);
#19333=VECTOR('',#67731,10.);
#19334=VECTOR('',#67734,10.);
#19335=VECTOR('',#67735,10.);
#19336=VECTOR('',#67740,10.);
#19337=VECTOR('',#67741,10.);
#19338=VECTOR('',#67742,10.);
#19339=VECTOR('',#67743,10.);
#19340=VECTOR('',#67746,10.);
#19341=VECTOR('',#67747,10.);
#19342=VECTOR('',#67748,10.);
#19343=VECTOR('',#67751,10.);
#19344=VECTOR('',#67752,10.);
#19345=VECTOR('',#67753,10.);
#19346=VECTOR('',#67756,10.);
#19347=VECTOR('',#67757,10.);
#19348=VECTOR('',#67762,10.);
#19349=VECTOR('',#67763,10.);
#19350=VECTOR('',#67764,10.);
#19351=VECTOR('',#67765,10.);
#19352=VECTOR('',#67768,10.);
#19353=VECTOR('',#67769,10.);
#19354=VECTOR('',#67770,10.);
#19355=VECTOR('',#67773,10.);
#19356=VECTOR('',#67774,10.);
#19357=VECTOR('',#67775,10.);
#19358=VECTOR('',#67778,10.);
#19359=VECTOR('',#67779,10.);
#19360=VECTOR('',#67784,10.);
#19361=VECTOR('',#67785,10.);
#19362=VECTOR('',#67786,10.);
#19363=VECTOR('',#67787,10.);
#19364=VECTOR('',#67790,10.);
#19365=VECTOR('',#67791,10.);
#19366=VECTOR('',#67792,10.);
#19367=VECTOR('',#67795,10.);
#19368=VECTOR('',#67796,10.);
#19369=VECTOR('',#67797,10.);
#19370=VECTOR('',#67800,10.);
#19371=VECTOR('',#67801,10.);
#19372=VECTOR('',#67806,10.);
#19373=VECTOR('',#67807,10.);
#19374=VECTOR('',#67808,10.);
#19375=VECTOR('',#67809,10.);
#19376=VECTOR('',#67812,10.);
#19377=VECTOR('',#67813,10.);
#19378=VECTOR('',#67814,10.);
#19379=VECTOR('',#67817,10.);
#19380=VECTOR('',#67818,10.);
#19381=VECTOR('',#67819,10.);
#19382=VECTOR('',#67822,10.);
#19383=VECTOR('',#67823,10.);
#19384=VECTOR('',#67828,10.);
#19385=VECTOR('',#67829,10.);
#19386=VECTOR('',#67830,10.);
#19387=VECTOR('',#67831,10.);
#19388=VECTOR('',#67834,10.);
#19389=VECTOR('',#67835,10.);
#19390=VECTOR('',#67836,10.);
#19391=VECTOR('',#67839,10.);
#19392=VECTOR('',#67840,10.);
#19393=VECTOR('',#67841,10.);
#19394=VECTOR('',#67844,10.);
#19395=VECTOR('',#67845,10.);
#19396=VECTOR('',#67850,10.);
#19397=VECTOR('',#67851,10.);
#19398=VECTOR('',#67852,10.);
#19399=VECTOR('',#67853,10.);
#19400=VECTOR('',#67856,10.);
#19401=VECTOR('',#67857,10.);
#19402=VECTOR('',#67858,10.);
#19403=VECTOR('',#67861,10.);
#19404=VECTOR('',#67862,10.);
#19405=VECTOR('',#67863,10.);
#19406=VECTOR('',#67866,10.);
#19407=VECTOR('',#67867,10.);
#19408=VECTOR('',#67872,10.);
#19409=VECTOR('',#67873,10.);
#19410=VECTOR('',#67874,10.);
#19411=VECTOR('',#67875,10.);
#19412=VECTOR('',#67878,10.);
#19413=VECTOR('',#67879,10.);
#19414=VECTOR('',#67880,10.);
#19415=VECTOR('',#67883,10.);
#19416=VECTOR('',#67884,10.);
#19417=VECTOR('',#67885,10.);
#19418=VECTOR('',#67888,10.);
#19419=VECTOR('',#67889,10.);
#19420=VECTOR('',#67894,10.);
#19421=VECTOR('',#67895,10.);
#19422=VECTOR('',#67896,10.);
#19423=VECTOR('',#67897,10.);
#19424=VECTOR('',#67900,10.);
#19425=VECTOR('',#67901,10.);
#19426=VECTOR('',#67902,10.);
#19427=VECTOR('',#67905,10.);
#19428=VECTOR('',#67906,10.);
#19429=VECTOR('',#67907,10.);
#19430=VECTOR('',#67910,10.);
#19431=VECTOR('',#67911,10.);
#19432=VECTOR('',#67916,10.);
#19433=VECTOR('',#67917,10.);
#19434=VECTOR('',#67918,10.);
#19435=VECTOR('',#67919,10.);
#19436=VECTOR('',#67922,10.);
#19437=VECTOR('',#67923,10.);
#19438=VECTOR('',#67924,10.);
#19439=VECTOR('',#67927,10.);
#19440=VECTOR('',#67928,10.);
#19441=VECTOR('',#67929,10.);
#19442=VECTOR('',#67932,10.);
#19443=VECTOR('',#67933,10.);
#19444=VECTOR('',#67938,10.);
#19445=VECTOR('',#67939,10.);
#19446=VECTOR('',#67940,10.);
#19447=VECTOR('',#67941,10.);
#19448=VECTOR('',#67944,10.);
#19449=VECTOR('',#67945,10.);
#19450=VECTOR('',#67946,10.);
#19451=VECTOR('',#67949,10.);
#19452=VECTOR('',#67950,10.);
#19453=VECTOR('',#67951,10.);
#19454=VECTOR('',#67954,10.);
#19455=VECTOR('',#67955,10.);
#19456=VECTOR('',#67960,10.);
#19457=VECTOR('',#67961,10.);
#19458=VECTOR('',#67962,10.);
#19459=VECTOR('',#67963,10.);
#19460=VECTOR('',#67966,10.);
#19461=VECTOR('',#67967,10.);
#19462=VECTOR('',#67968,10.);
#19463=VECTOR('',#67971,10.);
#19464=VECTOR('',#67972,10.);
#19465=VECTOR('',#67973,10.);
#19466=VECTOR('',#67976,10.);
#19467=VECTOR('',#67977,10.);
#19468=VECTOR('',#67982,10.);
#19469=VECTOR('',#67983,10.);
#19470=VECTOR('',#67984,10.);
#19471=VECTOR('',#67985,10.);
#19472=VECTOR('',#67988,10.);
#19473=VECTOR('',#67989,10.);
#19474=VECTOR('',#67990,10.);
#19475=VECTOR('',#67993,10.);
#19476=VECTOR('',#67994,10.);
#19477=VECTOR('',#67995,10.);
#19478=VECTOR('',#67998,10.);
#19479=VECTOR('',#67999,10.);
#19480=VECTOR('',#68004,10.);
#19481=VECTOR('',#68005,10.);
#19482=VECTOR('',#68006,10.);
#19483=VECTOR('',#68007,10.);
#19484=VECTOR('',#68010,10.);
#19485=VECTOR('',#68011,10.);
#19486=VECTOR('',#68012,10.);
#19487=VECTOR('',#68015,10.);
#19488=VECTOR('',#68016,10.);
#19489=VECTOR('',#68017,10.);
#19490=VECTOR('',#68020,10.);
#19491=VECTOR('',#68021,10.);
#19492=VECTOR('',#68026,10.);
#19493=VECTOR('',#68027,10.);
#19494=VECTOR('',#68028,10.);
#19495=VECTOR('',#68029,10.);
#19496=VECTOR('',#68032,10.);
#19497=VECTOR('',#68033,10.);
#19498=VECTOR('',#68034,10.);
#19499=VECTOR('',#68037,10.);
#19500=VECTOR('',#68038,10.);
#19501=VECTOR('',#68039,10.);
#19502=VECTOR('',#68042,10.);
#19503=VECTOR('',#68043,10.);
#19504=VECTOR('',#68048,10.);
#19505=VECTOR('',#68049,10.);
#19506=VECTOR('',#68050,10.);
#19507=VECTOR('',#68051,10.);
#19508=VECTOR('',#68054,10.);
#19509=VECTOR('',#68055,10.);
#19510=VECTOR('',#68056,10.);
#19511=VECTOR('',#68059,10.);
#19512=VECTOR('',#68060,10.);
#19513=VECTOR('',#68061,10.);
#19514=VECTOR('',#68064,10.);
#19515=VECTOR('',#68065,10.);
#19516=VECTOR('',#68070,10.);
#19517=VECTOR('',#68071,10.);
#19518=VECTOR('',#68072,10.);
#19519=VECTOR('',#68073,10.);
#19520=VECTOR('',#68076,10.);
#19521=VECTOR('',#68077,10.);
#19522=VECTOR('',#68078,10.);
#19523=VECTOR('',#68081,10.);
#19524=VECTOR('',#68082,10.);
#19525=VECTOR('',#68083,10.);
#19526=VECTOR('',#68086,10.);
#19527=VECTOR('',#68087,10.);
#19528=VECTOR('',#68092,10.);
#19529=VECTOR('',#68093,10.);
#19530=VECTOR('',#68094,10.);
#19531=VECTOR('',#68095,10.);
#19532=VECTOR('',#68098,10.);
#19533=VECTOR('',#68099,10.);
#19534=VECTOR('',#68100,10.);
#19535=VECTOR('',#68103,10.);
#19536=VECTOR('',#68104,10.);
#19537=VECTOR('',#68105,10.);
#19538=VECTOR('',#68108,10.);
#19539=VECTOR('',#68109,10.);
#19540=VECTOR('',#68114,10.);
#19541=VECTOR('',#68115,10.);
#19542=VECTOR('',#68116,10.);
#19543=VECTOR('',#68117,10.);
#19544=VECTOR('',#68120,10.);
#19545=VECTOR('',#68121,10.);
#19546=VECTOR('',#68122,10.);
#19547=VECTOR('',#68125,10.);
#19548=VECTOR('',#68126,10.);
#19549=VECTOR('',#68127,10.);
#19550=VECTOR('',#68130,10.);
#19551=VECTOR('',#68131,10.);
#19552=VECTOR('',#68136,10.);
#19553=VECTOR('',#68137,10.);
#19554=VECTOR('',#68138,10.);
#19555=VECTOR('',#68139,10.);
#19556=VECTOR('',#68142,10.);
#19557=VECTOR('',#68143,10.);
#19558=VECTOR('',#68144,10.);
#19559=VECTOR('',#68147,10.);
#19560=VECTOR('',#68148,10.);
#19561=VECTOR('',#68149,10.);
#19562=VECTOR('',#68152,10.);
#19563=VECTOR('',#68153,10.);
#19564=VECTOR('',#68158,10.);
#19565=VECTOR('',#68159,10.);
#19566=VECTOR('',#68160,10.);
#19567=VECTOR('',#68161,10.);
#19568=VECTOR('',#68164,10.);
#19569=VECTOR('',#68165,10.);
#19570=VECTOR('',#68166,10.);
#19571=VECTOR('',#68169,10.);
#19572=VECTOR('',#68170,10.);
#19573=VECTOR('',#68171,10.);
#19574=VECTOR('',#68174,10.);
#19575=VECTOR('',#68175,10.);
#19576=VECTOR('',#68180,10.);
#19577=VECTOR('',#68181,10.);
#19578=VECTOR('',#68182,10.);
#19579=VECTOR('',#68183,10.);
#19580=VECTOR('',#68186,10.);
#19581=VECTOR('',#68187,10.);
#19582=VECTOR('',#68188,10.);
#19583=VECTOR('',#68191,10.);
#19584=VECTOR('',#68192,10.);
#19585=VECTOR('',#68193,10.);
#19586=VECTOR('',#68196,10.);
#19587=VECTOR('',#68197,10.);
#19588=VECTOR('',#68202,10.);
#19589=VECTOR('',#68203,10.);
#19590=VECTOR('',#68204,10.);
#19591=VECTOR('',#68205,10.);
#19592=VECTOR('',#68208,10.);
#19593=VECTOR('',#68209,10.);
#19594=VECTOR('',#68210,10.);
#19595=VECTOR('',#68213,10.);
#19596=VECTOR('',#68214,10.);
#19597=VECTOR('',#68215,10.);
#19598=VECTOR('',#68218,10.);
#19599=VECTOR('',#68219,10.);
#19600=VECTOR('',#68224,10.);
#19601=VECTOR('',#68225,10.);
#19602=VECTOR('',#68226,10.);
#19603=VECTOR('',#68227,10.);
#19604=VECTOR('',#68230,10.);
#19605=VECTOR('',#68231,10.);
#19606=VECTOR('',#68232,10.);
#19607=VECTOR('',#68235,10.);
#19608=VECTOR('',#68236,10.);
#19609=VECTOR('',#68237,10.);
#19610=VECTOR('',#68240,10.);
#19611=VECTOR('',#68241,10.);
#19612=VECTOR('',#68246,10.);
#19613=VECTOR('',#68247,10.);
#19614=VECTOR('',#68248,10.);
#19615=VECTOR('',#68249,10.);
#19616=VECTOR('',#68252,10.);
#19617=VECTOR('',#68253,10.);
#19618=VECTOR('',#68254,10.);
#19619=VECTOR('',#68257,10.);
#19620=VECTOR('',#68258,10.);
#19621=VECTOR('',#68259,10.);
#19622=VECTOR('',#68262,10.);
#19623=VECTOR('',#68263,10.);
#19624=VECTOR('',#68268,10.);
#19625=VECTOR('',#68269,10.);
#19626=VECTOR('',#68270,10.);
#19627=VECTOR('',#68271,10.);
#19628=VECTOR('',#68274,10.);
#19629=VECTOR('',#68275,10.);
#19630=VECTOR('',#68276,10.);
#19631=VECTOR('',#68279,10.);
#19632=VECTOR('',#68280,10.);
#19633=VECTOR('',#68281,10.);
#19634=VECTOR('',#68284,10.);
#19635=VECTOR('',#68285,10.);
#19636=VECTOR('',#68290,10.);
#19637=VECTOR('',#68291,10.);
#19638=VECTOR('',#68292,10.);
#19639=VECTOR('',#68293,10.);
#19640=VECTOR('',#68296,10.);
#19641=VECTOR('',#68297,10.);
#19642=VECTOR('',#68298,10.);
#19643=VECTOR('',#68301,10.);
#19644=VECTOR('',#68302,10.);
#19645=VECTOR('',#68303,10.);
#19646=VECTOR('',#68306,10.);
#19647=VECTOR('',#68307,10.);
#19648=VECTOR('',#68312,10.);
#19649=VECTOR('',#68313,10.);
#19650=VECTOR('',#68314,10.);
#19651=VECTOR('',#68315,10.);
#19652=VECTOR('',#68318,10.);
#19653=VECTOR('',#68319,10.);
#19654=VECTOR('',#68320,10.);
#19655=VECTOR('',#68323,10.);
#19656=VECTOR('',#68324,10.);
#19657=VECTOR('',#68325,10.);
#19658=VECTOR('',#68328,10.);
#19659=VECTOR('',#68329,10.);
#19660=VECTOR('',#68334,10.);
#19661=VECTOR('',#68335,10.);
#19662=VECTOR('',#68336,10.);
#19663=VECTOR('',#68337,10.);
#19664=VECTOR('',#68340,10.);
#19665=VECTOR('',#68341,10.);
#19666=VECTOR('',#68342,10.);
#19667=VECTOR('',#68345,10.);
#19668=VECTOR('',#68346,10.);
#19669=VECTOR('',#68347,10.);
#19670=VECTOR('',#68350,10.);
#19671=VECTOR('',#68351,10.);
#19672=VECTOR('',#68356,10.);
#19673=VECTOR('',#68357,10.);
#19674=VECTOR('',#68358,10.);
#19675=VECTOR('',#68359,10.);
#19676=VECTOR('',#68362,10.);
#19677=VECTOR('',#68363,10.);
#19678=VECTOR('',#68364,10.);
#19679=VECTOR('',#68367,10.);
#19680=VECTOR('',#68368,10.);
#19681=VECTOR('',#68369,10.);
#19682=VECTOR('',#68372,10.);
#19683=VECTOR('',#68373,10.);
#19684=VECTOR('',#68378,10.);
#19685=VECTOR('',#68379,10.);
#19686=VECTOR('',#68380,10.);
#19687=VECTOR('',#68381,10.);
#19688=VECTOR('',#68384,10.);
#19689=VECTOR('',#68385,10.);
#19690=VECTOR('',#68386,10.);
#19691=VECTOR('',#68389,10.);
#19692=VECTOR('',#68390,10.);
#19693=VECTOR('',#68391,10.);
#19694=VECTOR('',#68394,10.);
#19695=VECTOR('',#68395,10.);
#19696=VECTOR('',#68400,10.);
#19697=VECTOR('',#68401,10.);
#19698=VECTOR('',#68402,10.);
#19699=VECTOR('',#68403,10.);
#19700=VECTOR('',#68406,10.);
#19701=VECTOR('',#68407,10.);
#19702=VECTOR('',#68408,10.);
#19703=VECTOR('',#68411,10.);
#19704=VECTOR('',#68412,10.);
#19705=VECTOR('',#68413,10.);
#19706=VECTOR('',#68416,10.);
#19707=VECTOR('',#68417,10.);
#19708=VECTOR('',#68422,10.);
#19709=VECTOR('',#68423,10.);
#19710=VECTOR('',#68424,10.);
#19711=VECTOR('',#68425,10.);
#19712=VECTOR('',#68428,10.);
#19713=VECTOR('',#68429,10.);
#19714=VECTOR('',#68430,10.);
#19715=VECTOR('',#68433,10.);
#19716=VECTOR('',#68434,10.);
#19717=VECTOR('',#68435,10.);
#19718=VECTOR('',#68438,10.);
#19719=VECTOR('',#68439,10.);
#19720=VECTOR('',#68444,10.);
#19721=VECTOR('',#68445,10.);
#19722=VECTOR('',#68446,10.);
#19723=VECTOR('',#68447,10.);
#19724=VECTOR('',#68450,10.);
#19725=VECTOR('',#68451,10.);
#19726=VECTOR('',#68452,10.);
#19727=VECTOR('',#68455,10.);
#19728=VECTOR('',#68456,10.);
#19729=VECTOR('',#68457,10.);
#19730=VECTOR('',#68460,10.);
#19731=VECTOR('',#68461,10.);
#19732=VECTOR('',#68466,10.);
#19733=VECTOR('',#68467,10.);
#19734=VECTOR('',#68468,10.);
#19735=VECTOR('',#68469,10.);
#19736=VECTOR('',#68472,10.);
#19737=VECTOR('',#68473,10.);
#19738=VECTOR('',#68474,10.);
#19739=VECTOR('',#68477,10.);
#19740=VECTOR('',#68478,10.);
#19741=VECTOR('',#68479,10.);
#19742=VECTOR('',#68482,10.);
#19743=VECTOR('',#68483,10.);
#19744=VECTOR('',#68488,10.);
#19745=VECTOR('',#68489,10.);
#19746=VECTOR('',#68490,10.);
#19747=VECTOR('',#68491,10.);
#19748=VECTOR('',#68494,10.);
#19749=VECTOR('',#68495,10.);
#19750=VECTOR('',#68496,10.);
#19751=VECTOR('',#68499,10.);
#19752=VECTOR('',#68500,10.);
#19753=VECTOR('',#68501,10.);
#19754=VECTOR('',#68504,10.);
#19755=VECTOR('',#68505,10.);
#19756=VECTOR('',#68510,10.);
#19757=VECTOR('',#68511,10.);
#19758=VECTOR('',#68512,10.);
#19759=VECTOR('',#68513,10.);
#19760=VECTOR('',#68516,10.);
#19761=VECTOR('',#68517,10.);
#19762=VECTOR('',#68518,10.);
#19763=VECTOR('',#68521,10.);
#19764=VECTOR('',#68522,10.);
#19765=VECTOR('',#68523,10.);
#19766=VECTOR('',#68526,10.);
#19767=VECTOR('',#68527,10.);
#19768=VECTOR('',#68532,10.);
#19769=VECTOR('',#68533,10.);
#19770=VECTOR('',#68534,10.);
#19771=VECTOR('',#68535,10.);
#19772=VECTOR('',#68538,10.);
#19773=VECTOR('',#68539,10.);
#19774=VECTOR('',#68540,10.);
#19775=VECTOR('',#68543,10.);
#19776=VECTOR('',#68544,10.);
#19777=VECTOR('',#68545,10.);
#19778=VECTOR('',#68548,10.);
#19779=VECTOR('',#68549,10.);
#19780=VECTOR('',#68554,10.);
#19781=VECTOR('',#68555,10.);
#19782=VECTOR('',#68556,10.);
#19783=VECTOR('',#68557,10.);
#19784=VECTOR('',#68560,10.);
#19785=VECTOR('',#68561,10.);
#19786=VECTOR('',#68562,10.);
#19787=VECTOR('',#68565,10.);
#19788=VECTOR('',#68566,10.);
#19789=VECTOR('',#68567,10.);
#19790=VECTOR('',#68570,10.);
#19791=VECTOR('',#68571,10.);
#19792=VECTOR('',#68576,10.);
#19793=VECTOR('',#68577,10.);
#19794=VECTOR('',#68578,10.);
#19795=VECTOR('',#68579,10.);
#19796=VECTOR('',#68582,10.);
#19797=VECTOR('',#68583,10.);
#19798=VECTOR('',#68584,10.);
#19799=VECTOR('',#68587,10.);
#19800=VECTOR('',#68588,10.);
#19801=VECTOR('',#68589,10.);
#19802=VECTOR('',#68592,10.);
#19803=VECTOR('',#68593,10.);
#19804=VECTOR('',#68598,10.);
#19805=VECTOR('',#68599,10.);
#19806=VECTOR('',#68600,10.);
#19807=VECTOR('',#68601,10.);
#19808=VECTOR('',#68604,10.);
#19809=VECTOR('',#68605,10.);
#19810=VECTOR('',#68606,10.);
#19811=VECTOR('',#68609,10.);
#19812=VECTOR('',#68610,10.);
#19813=VECTOR('',#68611,10.);
#19814=VECTOR('',#68614,10.);
#19815=VECTOR('',#68615,10.);
#19816=VECTOR('',#68620,10.);
#19817=VECTOR('',#68621,10.);
#19818=VECTOR('',#68622,10.);
#19819=VECTOR('',#68623,10.);
#19820=VECTOR('',#68626,10.);
#19821=VECTOR('',#68627,10.);
#19822=VECTOR('',#68628,10.);
#19823=VECTOR('',#68631,10.);
#19824=VECTOR('',#68632,10.);
#19825=VECTOR('',#68633,10.);
#19826=VECTOR('',#68636,10.);
#19827=VECTOR('',#68637,10.);
#19828=VECTOR('',#68642,10.);
#19829=VECTOR('',#68643,10.);
#19830=VECTOR('',#68644,10.);
#19831=VECTOR('',#68645,10.);
#19832=VECTOR('',#68648,10.);
#19833=VECTOR('',#68649,10.);
#19834=VECTOR('',#68650,10.);
#19835=VECTOR('',#68653,10.);
#19836=VECTOR('',#68654,10.);
#19837=VECTOR('',#68655,10.);
#19838=VECTOR('',#68658,10.);
#19839=VECTOR('',#68659,10.);
#19840=VECTOR('',#68664,10.);
#19841=VECTOR('',#68665,10.);
#19842=VECTOR('',#68666,10.);
#19843=VECTOR('',#68667,10.);
#19844=VECTOR('',#68670,10.);
#19845=VECTOR('',#68671,10.);
#19846=VECTOR('',#68672,10.);
#19847=VECTOR('',#68675,10.);
#19848=VECTOR('',#68676,10.);
#19849=VECTOR('',#68677,10.);
#19850=VECTOR('',#68680,10.);
#19851=VECTOR('',#68681,10.);
#19852=VECTOR('',#68686,10.);
#19853=VECTOR('',#68687,10.);
#19854=VECTOR('',#68688,10.);
#19855=VECTOR('',#68689,10.);
#19856=VECTOR('',#68692,10.);
#19857=VECTOR('',#68693,10.);
#19858=VECTOR('',#68694,10.);
#19859=VECTOR('',#68697,10.);
#19860=VECTOR('',#68698,10.);
#19861=VECTOR('',#68699,10.);
#19862=VECTOR('',#68702,10.);
#19863=VECTOR('',#68703,10.);
#19864=VECTOR('',#68708,10.);
#19865=VECTOR('',#68709,10.);
#19866=VECTOR('',#68710,10.);
#19867=VECTOR('',#68711,10.);
#19868=VECTOR('',#68714,10.);
#19869=VECTOR('',#68715,10.);
#19870=VECTOR('',#68716,10.);
#19871=VECTOR('',#68719,10.);
#19872=VECTOR('',#68720,10.);
#19873=VECTOR('',#68721,10.);
#19874=VECTOR('',#68724,10.);
#19875=VECTOR('',#68725,10.);
#19876=VECTOR('',#68730,10.);
#19877=VECTOR('',#68731,10.);
#19878=VECTOR('',#68732,10.);
#19879=VECTOR('',#68733,10.);
#19880=VECTOR('',#68736,10.);
#19881=VECTOR('',#68737,10.);
#19882=VECTOR('',#68738,10.);
#19883=VECTOR('',#68741,10.);
#19884=VECTOR('',#68742,10.);
#19885=VECTOR('',#68743,10.);
#19886=VECTOR('',#68746,10.);
#19887=VECTOR('',#68747,10.);
#19888=VECTOR('',#68752,10.);
#19889=VECTOR('',#68753,10.);
#19890=VECTOR('',#68754,10.);
#19891=VECTOR('',#68755,10.);
#19892=VECTOR('',#68758,10.);
#19893=VECTOR('',#68759,10.);
#19894=VECTOR('',#68760,10.);
#19895=VECTOR('',#68763,10.);
#19896=VECTOR('',#68764,10.);
#19897=VECTOR('',#68765,10.);
#19898=VECTOR('',#68768,10.);
#19899=VECTOR('',#68769,10.);
#19900=VECTOR('',#68774,10.);
#19901=VECTOR('',#68775,10.);
#19902=VECTOR('',#68776,10.);
#19903=VECTOR('',#68777,10.);
#19904=VECTOR('',#68780,10.);
#19905=VECTOR('',#68781,10.);
#19906=VECTOR('',#68782,10.);
#19907=VECTOR('',#68785,10.);
#19908=VECTOR('',#68786,10.);
#19909=VECTOR('',#68787,10.);
#19910=VECTOR('',#68790,10.);
#19911=VECTOR('',#68791,10.);
#19912=VECTOR('',#68796,10.);
#19913=VECTOR('',#68797,10.);
#19914=VECTOR('',#68798,10.);
#19915=VECTOR('',#68799,10.);
#19916=VECTOR('',#68802,10.);
#19917=VECTOR('',#68803,10.);
#19918=VECTOR('',#68804,10.);
#19919=VECTOR('',#68807,10.);
#19920=VECTOR('',#68808,10.);
#19921=VECTOR('',#68809,10.);
#19922=VECTOR('',#68812,10.);
#19923=VECTOR('',#68813,10.);
#19924=VECTOR('',#68818,10.);
#19925=VECTOR('',#68819,10.);
#19926=VECTOR('',#68820,10.);
#19927=VECTOR('',#68821,10.);
#19928=VECTOR('',#68824,10.);
#19929=VECTOR('',#68825,10.);
#19930=VECTOR('',#68826,10.);
#19931=VECTOR('',#68829,10.);
#19932=VECTOR('',#68830,10.);
#19933=VECTOR('',#68831,10.);
#19934=VECTOR('',#68834,10.);
#19935=VECTOR('',#68835,10.);
#19936=VECTOR('',#68840,10.);
#19937=VECTOR('',#68841,10.);
#19938=VECTOR('',#68842,10.);
#19939=VECTOR('',#68843,10.);
#19940=VECTOR('',#68846,10.);
#19941=VECTOR('',#68847,10.);
#19942=VECTOR('',#68848,10.);
#19943=VECTOR('',#68851,10.);
#19944=VECTOR('',#68852,10.);
#19945=VECTOR('',#68853,10.);
#19946=VECTOR('',#68856,10.);
#19947=VECTOR('',#68857,10.);
#19948=VECTOR('',#68862,10.);
#19949=VECTOR('',#68863,10.);
#19950=VECTOR('',#68864,10.);
#19951=VECTOR('',#68865,10.);
#19952=VECTOR('',#68868,10.);
#19953=VECTOR('',#68869,10.);
#19954=VECTOR('',#68870,10.);
#19955=VECTOR('',#68873,10.);
#19956=VECTOR('',#68874,10.);
#19957=VECTOR('',#68875,10.);
#19958=VECTOR('',#68878,10.);
#19959=VECTOR('',#68879,10.);
#19960=VECTOR('',#68884,10.);
#19961=VECTOR('',#68885,10.);
#19962=VECTOR('',#68886,10.);
#19963=VECTOR('',#68887,10.);
#19964=VECTOR('',#68890,10.);
#19965=VECTOR('',#68891,10.);
#19966=VECTOR('',#68892,10.);
#19967=VECTOR('',#68895,10.);
#19968=VECTOR('',#68896,10.);
#19969=VECTOR('',#68897,10.);
#19970=VECTOR('',#68900,10.);
#19971=VECTOR('',#68901,10.);
#19972=VECTOR('',#68906,10.);
#19973=VECTOR('',#68907,10.);
#19974=VECTOR('',#68908,10.);
#19975=VECTOR('',#68909,10.);
#19976=VECTOR('',#68912,10.);
#19977=VECTOR('',#68913,10.);
#19978=VECTOR('',#68914,10.);
#19979=VECTOR('',#68917,10.);
#19980=VECTOR('',#68918,10.);
#19981=VECTOR('',#68919,10.);
#19982=VECTOR('',#68922,10.);
#19983=VECTOR('',#68923,10.);
#19984=VECTOR('',#68928,10.);
#19985=VECTOR('',#68929,10.);
#19986=VECTOR('',#68930,10.);
#19987=VECTOR('',#68931,10.);
#19988=VECTOR('',#68934,10.);
#19989=VECTOR('',#68935,10.);
#19990=VECTOR('',#68936,10.);
#19991=VECTOR('',#68939,10.);
#19992=VECTOR('',#68940,10.);
#19993=VECTOR('',#68941,10.);
#19994=VECTOR('',#68944,10.);
#19995=VECTOR('',#68945,10.);
#19996=VECTOR('',#68950,10.);
#19997=VECTOR('',#68951,10.);
#19998=VECTOR('',#68952,10.);
#19999=VECTOR('',#68953,10.);
#20000=VECTOR('',#68956,10.);
#20001=VECTOR('',#68957,10.);
#20002=VECTOR('',#68958,10.);
#20003=VECTOR('',#68961,10.);
#20004=VECTOR('',#68962,10.);
#20005=VECTOR('',#68963,10.);
#20006=VECTOR('',#68966,10.);
#20007=VECTOR('',#68967,10.);
#20008=VECTOR('',#68972,10.);
#20009=VECTOR('',#68973,10.);
#20010=VECTOR('',#68974,10.);
#20011=VECTOR('',#68975,10.);
#20012=VECTOR('',#68978,10.);
#20013=VECTOR('',#68979,10.);
#20014=VECTOR('',#68980,10.);
#20015=VECTOR('',#68983,10.);
#20016=VECTOR('',#68984,10.);
#20017=VECTOR('',#68985,10.);
#20018=VECTOR('',#68988,10.);
#20019=VECTOR('',#68989,10.);
#20020=VECTOR('',#68994,10.);
#20021=VECTOR('',#68995,10.);
#20022=VECTOR('',#68996,10.);
#20023=VECTOR('',#68997,10.);
#20024=VECTOR('',#68998,10.);
#20025=VECTOR('',#68999,10.);
#20026=VECTOR('',#69002,10.);
#20027=VECTOR('',#69003,10.);
#20028=VECTOR('',#69004,10.);
#20029=VECTOR('',#69005,10.);
#20030=VECTOR('',#69006,10.);
#20031=VECTOR('',#69007,10.);
#20032=VECTOR('',#69010,10.);
#20033=VECTOR('',#69011,10.);
#20034=VECTOR('',#69014,10.);
#20035=VECTOR('',#69015,10.);
#20036=VECTOR('',#69016,10.);
#20037=VECTOR('',#69017,10.);
#20038=VECTOR('',#69018,10.);
#20039=VECTOR('',#69021,10.);
#20040=VECTOR('',#69022,10.);
#20041=VECTOR('',#69023,10.);
#20042=VECTOR('',#69024,10.);
#20043=VECTOR('',#69025,10.);
#20044=VECTOR('',#69026,10.);
#20045=VECTOR('',#69027,10.);
#20046=VECTOR('',#69028,10.);
#20047=VECTOR('',#69029,10.);
#20048=VECTOR('',#69032,10.);
#20049=VECTOR('',#69033,10.);
#20050=VECTOR('',#69034,10.);
#20051=VECTOR('',#69035,10.);
#20052=VECTOR('',#69036,10.);
#20053=VECTOR('',#69039,10.);
#20054=VECTOR('',#69040,10.);
#20055=VECTOR('',#69041,10.);
#20056=VECTOR('',#69044,10.);
#20057=VECTOR('',#69045,10.);
#20058=VECTOR('',#69046,10.);
#20059=VECTOR('',#69049,10.);
#20060=VECTOR('',#69050,10.);
#20061=VECTOR('',#69053,10.);
#20062=VECTOR('',#69064,0.999999999999979);
#20063=VECTOR('',#69069,1.);
#20064=VECTOR('',#69074,1.);
#20065=VECTOR('',#69079,1.00000000000001);
#20066=VECTOR('',#69084,1.39999999999999);
#20067=VECTOR('',#69089,1.29999999999999);
#20068=VECTOR('',#69094,10.);
#20069=VECTOR('',#69095,10.);
#20070=VECTOR('',#69096,10.);
#20071=VECTOR('',#69097,10.);
#20072=VECTOR('',#69102,1.30000000000003);
#20073=VECTOR('',#69105,1.4);
#20074=VECTOR('',#69110,1.3);
#20075=VECTOR('',#69115,1.3);
#20076=VECTOR('',#69120,3.00000000000001);
#20077=VECTOR('',#69131,3.);
#20078=VECTOR('',#69142,3.);
#20079=VECTOR('',#69153,3.00000000000001);
#20080=VECTOR('',#69164,3.00000000000001);
#20081=VECTOR('',#69175,3.00000000000001);
#20082=VECTOR('',#69184,2.19999999999999);
#20083=VECTOR('',#69189,10.);
#20084=VECTOR('',#69190,10.);
#20085=VECTOR('',#69199,2.04999999999998);
#20086=VECTOR('',#69202,2.2);
#20087=VECTOR('',#69207,2.05);
#20088=VECTOR('',#69210,2.2);
#20089=VECTOR('',#69215,2.05);
#20090=VECTOR('',#69218,2.2);
#20091=VECTOR('',#69223,2.05);
#20092=VECTOR('',#69226,2.2);
#20093=VECTOR('',#69231,2.05);
#20094=VECTOR('',#69234,2.19999999999999);
#20095=VECTOR('',#69239,2.04999999999998);
#20096=VECTOR('',#69242,10.);
#20097=VECTOR('',#69245,10.);
#20098=VECTOR('',#69246,10.);
#20099=VECTOR('',#69249,10.);
#20100=VECTOR('',#69250,10.);
#20101=VECTOR('',#69251,10.);
#20102=VECTOR('',#69254,10.);
#20103=VECTOR('',#69255,10.);
#20104=VECTOR('',#69256,10.);
#20105=VECTOR('',#69259,10.);
#20106=VECTOR('',#69260,10.);
#20107=VECTOR('',#69261,10.);
#20108=VECTOR('',#69262,10.);
#20109=VECTOR('',#69265,10.);
#20110=VECTOR('',#69266,10.);
#20111=VECTOR('',#69267,10.);
#20112=VECTOR('',#69270,10.);
#20113=VECTOR('',#69271,10.);
#20114=VECTOR('',#69272,10.);
#20115=VECTOR('',#69275,10.);
#20116=VECTOR('',#69278,10.);
#20117=VECTOR('',#69281,10.);
#20118=VECTOR('',#69282,10.);
#20119=VECTOR('',#69285,10.);
#20120=VECTOR('',#69286,10.);
#20121=VECTOR('',#69289,10.);
#20122=VECTOR('',#69294,10.);
#20123=VECTOR('',#69301,10.);
#20124=VECTOR('',#69302,10.);
#20125=VECTOR('',#69305,10.);
#20126=VECTOR('',#69306,10.);
#20127=VECTOR('',#69309,10.);
#20128=VECTOR('',#69310,10.);
#20129=VECTOR('',#69313,10.);
#20130=VECTOR('',#69316,10.);
#20131=VECTOR('',#69317,10.);
#20132=VECTOR('',#69320,10.);
#20133=VECTOR('',#69323,10.);
#20134=VECTOR('',#69324,10.);
#20135=VECTOR('',#69327,10.);
#20136=VECTOR('',#69328,10.);
#20137=VECTOR('',#69329,10.);
#20138=VECTOR('',#69332,10.);
#20139=VECTOR('',#69333,10.);
#20140=VECTOR('',#69334,10.);
#20141=VECTOR('',#69337,10.);
#20142=VECTOR('',#69338,10.);
#20143=VECTOR('',#69341,10.);
#20144=VECTOR('',#69342,10.);
#20145=VECTOR('',#69343,10.);
#20146=VECTOR('',#69346,10.);
#20147=VECTOR('',#69347,10.);
#20148=VECTOR('',#69348,10.);
#20149=VECTOR('',#69351,10.);
#20150=VECTOR('',#69352,10.);
#20151=VECTOR('',#69353,10.);
#20152=VECTOR('',#69356,10.);
#20153=VECTOR('',#69357,10.);
#20154=VECTOR('',#69360,10.);
#20155=VECTOR('',#69361,10.);
#20156=VECTOR('',#69362,10.);
#20157=VECTOR('',#69365,10.);
#20158=VECTOR('',#69366,10.);
#20159=VECTOR('',#69369,10.);
#20160=VECTOR('',#69370,10.);
#20161=VECTOR('',#69373,10.);
#20162=VECTOR('',#69376,10.);
#20163=VECTOR('',#69377,10.);
#20164=VECTOR('',#69380,10.);
#20165=VECTOR('',#69381,10.);
#20166=VECTOR('',#69384,10.);
#20167=VECTOR('',#69385,10.);
#20168=VECTOR('',#69388,10.);
#20169=VECTOR('',#69391,10.);
#20170=VECTOR('',#69394,10.);
#20171=VECTOR('',#69397,10.);
#20172=VECTOR('',#69398,10.);
#20173=VECTOR('',#69401,10.);
#20174=VECTOR('',#69402,10.);
#20175=VECTOR('',#69405,10.);
#20176=VECTOR('',#69408,10.);
#20177=VECTOR('',#69411,10.);
#20178=VECTOR('',#69414,10.);
#20179=VECTOR('',#69417,10.);
#20180=VECTOR('',#69422,10.);
#20181=VECTOR('',#69425,10.);
#20182=VECTOR('',#69428,10.);
#20183=VECTOR('',#69433,10.);
#20184=VECTOR('',#69436,10.);
#20185=VECTOR('',#69439,10.);
#20186=VECTOR('',#69442,10.);
#20187=VECTOR('',#69453,10.);
#20188=VECTOR('',#69456,10.);
#20189=VECTOR('',#69459,10.);
#22944=B_SPLINE_CURVE_WITH_KNOTS('',2,(#76154,#76155,#76156),
 .UNSPECIFIED.,.F.,.F.,(3,3),(0.,1.),.UNSPECIFIED.);
#22945=B_SPLINE_CURVE_WITH_KNOTS('',2,(#76160,#76161,#76162),
 .UNSPECIFIED.,.F.,.F.,(3,3),(0.,1.),.UNSPECIFIED.);
#22946=B_SPLINE_CURVE_WITH_KNOTS('',2,(#76171,#76172,#76173),
 .UNSPECIFIED.,.F.,.F.,(3,3),(0.,1.),.UNSPECIFIED.);
#22947=B_SPLINE_CURVE_WITH_KNOTS('',2,(#76176,#76177,#76178),
 .UNSPECIFIED.,.F.,.F.,(3,3),(0.,1.),.UNSPECIFIED.);
#22948=B_SPLINE_CURVE_WITH_KNOTS('',2,(#76186,#76187,#76188),
 .UNSPECIFIED.,.F.,.F.,(3,3),(0.,1.),.UNSPECIFIED.);
#22949=B_SPLINE_CURVE_WITH_KNOTS('',2,(#76191,#76192,#76193),
 .UNSPECIFIED.,.F.,.F.,(3,3),(0.,1.),.UNSPECIFIED.);
#22950=B_SPLINE_CURVE_WITH_KNOTS('',2,(#76201,#76202,#76203),
 .UNSPECIFIED.,.F.,.F.,(3,3),(0.,1.),.UNSPECIFIED.);
#22951=B_SPLINE_CURVE_WITH_KNOTS('',2,(#76206,#76207,#76208),
 .UNSPECIFIED.,.F.,.F.,(3,3),(0.,1.),.UNSPECIFIED.);
#22952=B_SPLINE_CURVE_WITH_KNOTS('',2,(#76216,#76217,#76218),
 .UNSPECIFIED.,.F.,.F.,(3,3),(0.,1.),.UNSPECIFIED.);
#22953=B_SPLINE_CURVE_WITH_KNOTS('',2,(#76221,#76222,#76223),
 .UNSPECIFIED.,.F.,.F.,(3,3),(0.,1.),.UNSPECIFIED.);
#22954=B_SPLINE_CURVE_WITH_KNOTS('',2,(#76231,#76232,#76233),
 .UNSPECIFIED.,.F.,.F.,(3,3),(0.,1.),.UNSPECIFIED.);
#22955=B_SPLINE_CURVE_WITH_KNOTS('',2,(#76236,#76237,#76238),
 .UNSPECIFIED.,.F.,.F.,(3,3),(0.,1.),.UNSPECIFIED.);
#22956=B_SPLINE_CURVE_WITH_KNOTS('',2,(#76246,#76247,#76248),
 .UNSPECIFIED.,.F.,.F.,(3,3),(0.,1.),.UNSPECIFIED.);
#22957=B_SPLINE_CURVE_WITH_KNOTS('',2,(#76251,#76252,#76253),
 .UNSPECIFIED.,.F.,.F.,(3,3),(0.,1.),.UNSPECIFIED.);
#22958=B_SPLINE_CURVE_WITH_KNOTS('',2,(#76260,#76261,#76262),
 .UNSPECIFIED.,.F.,.F.,(3,3),(0.,1.),.UNSPECIFIED.);
#22959=B_SPLINE_CURVE_WITH_KNOTS('',2,(#76263,#76264,#76265),
 .UNSPECIFIED.,.F.,.F.,(3,3),(0.,1.),.UNSPECIFIED.);
#22960=B_SPLINE_CURVE_WITH_KNOTS('',2,(#76274,#76275,#76276),
 .UNSPECIFIED.,.F.,.F.,(3,3),(0.,1.),.UNSPECIFIED.);
#22961=B_SPLINE_CURVE_WITH_KNOTS('',2,(#76280,#76281,#76282),
 .UNSPECIFIED.,.F.,.F.,(3,3),(0.,1.),.UNSPECIFIED.);
#22962=B_SPLINE_CURVE_WITH_KNOTS('',2,(#76291,#76292,#76293),
 .UNSPECIFIED.,.F.,.F.,(3,3),(0.,1.),.UNSPECIFIED.);
#22963=B_SPLINE_CURVE_WITH_KNOTS('',2,(#76296,#76297,#76298),
 .UNSPECIFIED.,.F.,.F.,(3,3),(0.,1.),.UNSPECIFIED.);
#22964=B_SPLINE_CURVE_WITH_KNOTS('',2,(#76306,#76307,#76308),
 .UNSPECIFIED.,.F.,.F.,(3,3),(0.,1.),.UNSPECIFIED.);
#22965=B_SPLINE_CURVE_WITH_KNOTS('',2,(#76311,#76312,#76313),
 .UNSPECIFIED.,.F.,.F.,(3,3),(0.,1.),.UNSPECIFIED.);
#22966=B_SPLINE_CURVE_WITH_KNOTS('',2,(#76321,#76322,#76323),
 .UNSPECIFIED.,.F.,.F.,(3,3),(0.,1.),.UNSPECIFIED.);
#22967=B_SPLINE_CURVE_WITH_KNOTS('',2,(#76326,#76327,#76328),
 .UNSPECIFIED.,.F.,.F.,(3,3),(0.,1.),.UNSPECIFIED.);
#22968=B_SPLINE_CURVE_WITH_KNOTS('',2,(#76336,#76337,#76338),
 .UNSPECIFIED.,.F.,.F.,(3,3),(0.,1.),.UNSPECIFIED.);
#22969=B_SPLINE_CURVE_WITH_KNOTS('',2,(#76341,#76342,#76343),
 .UNSPECIFIED.,.F.,.F.,(3,3),(0.,1.),.UNSPECIFIED.);
#22970=B_SPLINE_CURVE_WITH_KNOTS('',2,(#76351,#76352,#76353),
 .UNSPECIFIED.,.F.,.F.,(3,3),(0.,1.),.UNSPECIFIED.);
#22971=B_SPLINE_CURVE_WITH_KNOTS('',2,(#76356,#76357,#76358),
 .UNSPECIFIED.,.F.,.F.,(3,3),(0.,1.),.UNSPECIFIED.);
#22972=B_SPLINE_CURVE_WITH_KNOTS('',2,(#76366,#76367,#76368),
 .UNSPECIFIED.,.F.,.F.,(3,3),(0.,1.),.UNSPECIFIED.);
#22973=B_SPLINE_CURVE_WITH_KNOTS('',2,(#76371,#76372,#76373),
 .UNSPECIFIED.,.F.,.F.,(3,3),(0.,1.),.UNSPECIFIED.);
#22974=B_SPLINE_CURVE_WITH_KNOTS('',2,(#76381,#76382,#76383),
 .UNSPECIFIED.,.F.,.F.,(3,3),(0.,1.),.UNSPECIFIED.);
#22975=B_SPLINE_CURVE_WITH_KNOTS('',2,(#76386,#76387,#76388),
 .UNSPECIFIED.,.F.,.F.,(3,3),(0.,1.),.UNSPECIFIED.);
#22976=B_SPLINE_CURVE_WITH_KNOTS('',2,(#76396,#76397,#76398),
 .UNSPECIFIED.,.F.,.F.,(3,3),(0.,1.),.UNSPECIFIED.);
#22977=B_SPLINE_CURVE_WITH_KNOTS('',2,(#76401,#76402,#76403),
 .UNSPECIFIED.,.F.,.F.,(3,3),(0.,1.),.UNSPECIFIED.);
#22978=B_SPLINE_CURVE_WITH_KNOTS('',2,(#76411,#76412,#76413),
 .UNSPECIFIED.,.F.,.F.,(3,3),(0.,1.),.UNSPECIFIED.);
#22979=B_SPLINE_CURVE_WITH_KNOTS('',2,(#76416,#76417,#76418),
 .UNSPECIFIED.,.F.,.F.,(3,3),(0.,1.),.UNSPECIFIED.);
#22980=B_SPLINE_CURVE_WITH_KNOTS('',2,(#76426,#76427,#76428),
 .UNSPECIFIED.,.F.,.F.,(3,3),(0.,1.),.UNSPECIFIED.);
#22981=B_SPLINE_CURVE_WITH_KNOTS('',2,(#76431,#76432,#76433),
 .UNSPECIFIED.,.F.,.F.,(3,3),(0.,1.),.UNSPECIFIED.);
#22982=B_SPLINE_CURVE_WITH_KNOTS('',2,(#76440,#76441,#76442),
 .UNSPECIFIED.,.F.,.F.,(3,3),(0.,1.),.UNSPECIFIED.);
#22983=B_SPLINE_CURVE_WITH_KNOTS('',2,(#76443,#76444,#76445),
 .UNSPECIFIED.,.F.,.F.,(3,3),(0.,1.),.UNSPECIFIED.);
#22984=B_SPLINE_CURVE_WITH_KNOTS('',2,(#76455,#76456,#76457),
 .UNSPECIFIED.,.F.,.F.,(3,3),(0.,1.),.UNSPECIFIED.);
#22985=B_SPLINE_CURVE_WITH_KNOTS('',2,(#76461,#76462,#76463),
 .UNSPECIFIED.,.F.,.F.,(3,3),(0.,1.),.UNSPECIFIED.);
#22986=B_SPLINE_CURVE_WITH_KNOTS('',2,(#76472,#76473,#76474),
 .UNSPECIFIED.,.F.,.F.,(3,3),(0.,1.),.UNSPECIFIED.);
#22987=B_SPLINE_CURVE_WITH_KNOTS('',2,(#76477,#76478,#76479),
 .UNSPECIFIED.,.F.,.F.,(3,3),(0.,1.),.UNSPECIFIED.);
#22988=B_SPLINE_CURVE_WITH_KNOTS('',2,(#76487,#76488,#76489),
 .UNSPECIFIED.,.F.,.F.,(3,3),(0.,1.),.UNSPECIFIED.);
#22989=B_SPLINE_CURVE_WITH_KNOTS('',2,(#76492,#76493,#76494),
 .UNSPECIFIED.,.F.,.F.,(3,3),(0.,1.),.UNSPECIFIED.);
#22990=B_SPLINE_CURVE_WITH_KNOTS('',2,(#76502,#76503,#76504),
 .UNSPECIFIED.,.F.,.F.,(3,3),(0.,1.),.UNSPECIFIED.);
#22991=B_SPLINE_CURVE_WITH_KNOTS('',2,(#76507,#76508,#76509),
 .UNSPECIFIED.,.F.,.F.,(3,3),(0.,1.),.UNSPECIFIED.);
#22992=B_SPLINE_CURVE_WITH_KNOTS('',2,(#76517,#76518,#76519),
 .UNSPECIFIED.,.F.,.F.,(3,3),(0.,1.),.UNSPECIFIED.);
#22993=B_SPLINE_CURVE_WITH_KNOTS('',2,(#76522,#76523,#76524),
 .UNSPECIFIED.,.F.,.F.,(3,3),(0.,1.),.UNSPECIFIED.);
#22994=B_SPLINE_CURVE_WITH_KNOTS('',2,(#76532,#76533,#76534),
 .UNSPECIFIED.,.F.,.F.,(3,3),(0.,1.),.UNSPECIFIED.);
#22995=B_SPLINE_CURVE_WITH_KNOTS('',2,(#76537,#76538,#76539),
 .UNSPECIFIED.,.F.,.F.,(3,3),(0.,1.),.UNSPECIFIED.);
#22996=B_SPLINE_CURVE_WITH_KNOTS('',2,(#76547,#76548,#76549),
 .UNSPECIFIED.,.F.,.F.,(3,3),(0.,1.),.UNSPECIFIED.);
#22997=B_SPLINE_CURVE_WITH_KNOTS('',2,(#76552,#76553,#76554),
 .UNSPECIFIED.,.F.,.F.,(3,3),(0.,1.),.UNSPECIFIED.);
#22998=B_SPLINE_CURVE_WITH_KNOTS('',2,(#76561,#76562,#76563),
 .UNSPECIFIED.,.F.,.F.,(3,3),(0.,1.),.UNSPECIFIED.);
#22999=B_SPLINE_CURVE_WITH_KNOTS('',2,(#76564,#76565,#76566),
 .UNSPECIFIED.,.F.,.F.,(3,3),(0.,1.),.UNSPECIFIED.);
#23000=B_SPLINE_CURVE_WITH_KNOTS('',2,(#76575,#76576,#76577),
 .UNSPECIFIED.,.F.,.F.,(3,3),(0.,1.),.UNSPECIFIED.);
#23001=B_SPLINE_CURVE_WITH_KNOTS('',2,(#76581,#76582,#76583),
 .UNSPECIFIED.,.F.,.F.,(3,3),(0.,1.),.UNSPECIFIED.);
#23002=B_SPLINE_CURVE_WITH_KNOTS('',2,(#76592,#76593,#76594),
 .UNSPECIFIED.,.F.,.F.,(3,3),(0.,1.),.UNSPECIFIED.);
#23003=B_SPLINE_CURVE_WITH_KNOTS('',2,(#76597,#76598,#76599),
 .UNSPECIFIED.,.F.,.F.,(3,3),(0.,1.),.UNSPECIFIED.);
#23004=B_SPLINE_CURVE_WITH_KNOTS('',2,(#76607,#76608,#76609),
 .UNSPECIFIED.,.F.,.F.,(3,3),(0.,1.),.UNSPECIFIED.);
#23005=B_SPLINE_CURVE_WITH_KNOTS('',2,(#76612,#76613,#76614),
 .UNSPECIFIED.,.F.,.F.,(3,3),(0.,1.),.UNSPECIFIED.);
#23006=B_SPLINE_CURVE_WITH_KNOTS('',2,(#76622,#76623,#76624),
 .UNSPECIFIED.,.F.,.F.,(3,3),(0.,1.),.UNSPECIFIED.);
#23007=B_SPLINE_CURVE_WITH_KNOTS('',2,(#76627,#76628,#76629),
 .UNSPECIFIED.,.F.,.F.,(3,3),(0.,1.),.UNSPECIFIED.);
#23008=B_SPLINE_CURVE_WITH_KNOTS('',2,(#76637,#76638,#76639),
 .UNSPECIFIED.,.F.,.F.,(3,3),(0.,1.),.UNSPECIFIED.);
#23009=B_SPLINE_CURVE_WITH_KNOTS('',2,(#76642,#76643,#76644),
 .UNSPECIFIED.,.F.,.F.,(3,3),(0.,1.),.UNSPECIFIED.);
#23010=B_SPLINE_CURVE_WITH_KNOTS('',2,(#76652,#76653,#76654),
 .UNSPECIFIED.,.F.,.F.,(3,3),(0.,1.),.UNSPECIFIED.);
#23011=B_SPLINE_CURVE_WITH_KNOTS('',2,(#76657,#76658,#76659),
 .UNSPECIFIED.,.F.,.F.,(3,3),(0.,1.),.UNSPECIFIED.);
#23012=B_SPLINE_CURVE_WITH_KNOTS('',2,(#76667,#76668,#76669),
 .UNSPECIFIED.,.F.,.F.,(3,3),(0.,1.),.UNSPECIFIED.);
#23013=B_SPLINE_CURVE_WITH_KNOTS('',2,(#76672,#76673,#76674),
 .UNSPECIFIED.,.F.,.F.,(3,3),(0.,1.),.UNSPECIFIED.);
#23014=B_SPLINE_CURVE_WITH_KNOTS('',2,(#76682,#76683,#76684),
 .UNSPECIFIED.,.F.,.F.,(3,3),(0.,1.),.UNSPECIFIED.);
#23015=B_SPLINE_CURVE_WITH_KNOTS('',2,(#76687,#76688,#76689),
 .UNSPECIFIED.,.F.,.F.,(3,3),(0.,1.),.UNSPECIFIED.);
#23016=B_SPLINE_CURVE_WITH_KNOTS('',2,(#76697,#76698,#76699),
 .UNSPECIFIED.,.F.,.F.,(3,3),(0.,1.),.UNSPECIFIED.);
#23017=B_SPLINE_CURVE_WITH_KNOTS('',2,(#76702,#76703,#76704),
 .UNSPECIFIED.,.F.,.F.,(3,3),(0.,1.),.UNSPECIFIED.);
#23018=B_SPLINE_CURVE_WITH_KNOTS('',2,(#76712,#76713,#76714),
 .UNSPECIFIED.,.F.,.F.,(3,3),(0.,1.),.UNSPECIFIED.);
#23019=B_SPLINE_CURVE_WITH_KNOTS('',2,(#76717,#76718,#76719),
 .UNSPECIFIED.,.F.,.F.,(3,3),(0.,1.),.UNSPECIFIED.);
#23020=B_SPLINE_CURVE_WITH_KNOTS('',2,(#76727,#76728,#76729),
 .UNSPECIFIED.,.F.,.F.,(3,3),(0.,1.),.UNSPECIFIED.);
#23021=B_SPLINE_CURVE_WITH_KNOTS('',2,(#76732,#76733,#76734),
 .UNSPECIFIED.,.F.,.F.,(3,3),(0.,1.),.UNSPECIFIED.);
#23022=B_SPLINE_CURVE_WITH_KNOTS('',2,(#76742,#76743,#76744),
 .UNSPECIFIED.,.F.,.F.,(3,3),(0.,1.),.UNSPECIFIED.);
#23023=B_SPLINE_CURVE_WITH_KNOTS('',2,(#76747,#76748,#76749),
 .UNSPECIFIED.,.F.,.F.,(3,3),(0.,1.),.UNSPECIFIED.);
#23024=B_SPLINE_CURVE_WITH_KNOTS('',2,(#76757,#76758,#76759),
 .UNSPECIFIED.,.F.,.F.,(3,3),(0.,1.),.UNSPECIFIED.);
#23025=B_SPLINE_CURVE_WITH_KNOTS('',2,(#76762,#76763,#76764),
 .UNSPECIFIED.,.F.,.F.,(3,3),(0.,1.),.UNSPECIFIED.);
#23026=B_SPLINE_CURVE_WITH_KNOTS('',2,(#76772,#76773,#76774),
 .UNSPECIFIED.,.F.,.F.,(3,3),(0.,1.),.UNSPECIFIED.);
#23027=B_SPLINE_CURVE_WITH_KNOTS('',2,(#76777,#76778,#76779),
 .UNSPECIFIED.,.F.,.F.,(3,3),(0.,1.),.UNSPECIFIED.);
#23028=B_SPLINE_CURVE_WITH_KNOTS('',2,(#76787,#76788,#76789),
 .UNSPECIFIED.,.F.,.F.,(3,3),(0.,1.),.UNSPECIFIED.);
#23029=B_SPLINE_CURVE_WITH_KNOTS('',2,(#76792,#76793,#76794),
 .UNSPECIFIED.,.F.,.F.,(3,3),(0.,1.),.UNSPECIFIED.);
#23030=B_SPLINE_CURVE_WITH_KNOTS('',2,(#76802,#76803,#76804),
 .UNSPECIFIED.,.F.,.F.,(3,3),(0.,1.),.UNSPECIFIED.);
#23031=B_SPLINE_CURVE_WITH_KNOTS('',2,(#76807,#76808,#76809),
 .UNSPECIFIED.,.F.,.F.,(3,3),(0.,1.),.UNSPECIFIED.);
#23032=B_SPLINE_CURVE_WITH_KNOTS('',2,(#76817,#76818,#76819),
 .UNSPECIFIED.,.F.,.F.,(3,3),(0.,1.),.UNSPECIFIED.);
#23033=B_SPLINE_CURVE_WITH_KNOTS('',2,(#76822,#76823,#76824),
 .UNSPECIFIED.,.F.,.F.,(3,3),(0.,1.),.UNSPECIFIED.);
#23034=B_SPLINE_CURVE_WITH_KNOTS('',2,(#76832,#76833,#76834),
 .UNSPECIFIED.,.F.,.F.,(3,3),(0.,1.),.UNSPECIFIED.);
#23035=B_SPLINE_CURVE_WITH_KNOTS('',2,(#76837,#76838,#76839),
 .UNSPECIFIED.,.F.,.F.,(3,3),(0.,1.),.UNSPECIFIED.);
#23036=B_SPLINE_CURVE_WITH_KNOTS('',2,(#76847,#76848,#76849),
 .UNSPECIFIED.,.F.,.F.,(3,3),(0.,1.),.UNSPECIFIED.);
#23037=B_SPLINE_CURVE_WITH_KNOTS('',2,(#76852,#76853,#76854),
 .UNSPECIFIED.,.F.,.F.,(3,3),(0.,1.),.UNSPECIFIED.);
#23038=B_SPLINE_CURVE_WITH_KNOTS('',2,(#76862,#76863,#76864),
 .UNSPECIFIED.,.F.,.F.,(3,3),(0.,1.),.UNSPECIFIED.);
#23039=B_SPLINE_CURVE_WITH_KNOTS('',2,(#76867,#76868,#76869),
 .UNSPECIFIED.,.F.,.F.,(3,3),(0.,1.),.UNSPECIFIED.);
#23040=B_SPLINE_CURVE_WITH_KNOTS('',2,(#76882,#76883,#76884),
 .UNSPECIFIED.,.F.,.F.,(3,3),(0.,1.),.UNSPECIFIED.);
#23041=B_SPLINE_CURVE_WITH_KNOTS('',2,(#76885,#76886,#76887),
 .UNSPECIFIED.,.F.,.F.,(3,3),(0.,1.),.UNSPECIFIED.);
#23042=B_SPLINE_CURVE_WITH_KNOTS('',2,(#76899,#76900,#76901),
 .UNSPECIFIED.,.F.,.F.,(3,3),(0.,1.),.UNSPECIFIED.);
#23043=B_SPLINE_CURVE_WITH_KNOTS('',2,(#76905,#76906,#76907),
 .UNSPECIFIED.,.F.,.F.,(3,3),(0.,1.),.UNSPECIFIED.);
#23044=B_SPLINE_CURVE_WITH_KNOTS('',2,(#76916,#76917,#76918),
 .UNSPECIFIED.,.F.,.F.,(3,3),(0.,1.),.UNSPECIFIED.);
#23045=B_SPLINE_CURVE_WITH_KNOTS('',2,(#76921,#76922,#76923),
 .UNSPECIFIED.,.F.,.F.,(3,3),(0.,1.),.UNSPECIFIED.);
#23046=B_SPLINE_CURVE_WITH_KNOTS('',2,(#76931,#76932,#76933),
 .UNSPECIFIED.,.F.,.F.,(3,3),(0.,1.),.UNSPECIFIED.);
#23047=B_SPLINE_CURVE_WITH_KNOTS('',2,(#76936,#76937,#76938),
 .UNSPECIFIED.,.F.,.F.,(3,3),(0.,1.),.UNSPECIFIED.);
#23048=B_SPLINE_CURVE_WITH_KNOTS('',2,(#76946,#76947,#76948),
 .UNSPECIFIED.,.F.,.F.,(3,3),(0.,1.),.UNSPECIFIED.);
#23049=B_SPLINE_CURVE_WITH_KNOTS('',2,(#76951,#76952,#76953),
 .UNSPECIFIED.,.F.,.F.,(3,3),(0.,1.),.UNSPECIFIED.);
#23050=B_SPLINE_CURVE_WITH_KNOTS('',2,(#76961,#76962,#76963),
 .UNSPECIFIED.,.F.,.F.,(3,3),(0.,1.),.UNSPECIFIED.);
#23051=B_SPLINE_CURVE_WITH_KNOTS('',2,(#76966,#76967,#76968),
 .UNSPECIFIED.,.F.,.F.,(3,3),(0.,1.),.UNSPECIFIED.);
#23052=B_SPLINE_CURVE_WITH_KNOTS('',2,(#76976,#76977,#76978),
 .UNSPECIFIED.,.F.,.F.,(3,3),(0.,1.),.UNSPECIFIED.);
#23053=B_SPLINE_CURVE_WITH_KNOTS('',2,(#76981,#76982,#76983),
 .UNSPECIFIED.,.F.,.F.,(3,3),(0.,1.),.UNSPECIFIED.);
#23054=B_SPLINE_CURVE_WITH_KNOTS('',2,(#76991,#76992,#76993),
 .UNSPECIFIED.,.F.,.F.,(3,3),(0.,1.),.UNSPECIFIED.);
#23055=B_SPLINE_CURVE_WITH_KNOTS('',2,(#76996,#76997,#76998),
 .UNSPECIFIED.,.F.,.F.,(3,3),(0.,1.),.UNSPECIFIED.);
#23056=B_SPLINE_CURVE_WITH_KNOTS('',2,(#77005,#77006,#77007),
 .UNSPECIFIED.,.F.,.F.,(3,3),(0.,1.),.UNSPECIFIED.);
#23057=B_SPLINE_CURVE_WITH_KNOTS('',2,(#77008,#77009,#77010),
 .UNSPECIFIED.,.F.,.F.,(3,3),(0.,1.),.UNSPECIFIED.);
#23058=B_SPLINE_CURVE_WITH_KNOTS('',2,(#77019,#77020,#77021),
 .UNSPECIFIED.,.F.,.F.,(3,3),(0.,1.),.UNSPECIFIED.);
#23059=B_SPLINE_CURVE_WITH_KNOTS('',2,(#77025,#77026,#77027),
 .UNSPECIFIED.,.F.,.F.,(3,3),(0.,1.),.UNSPECIFIED.);
#23060=B_SPLINE_CURVE_WITH_KNOTS('',2,(#77036,#77037,#77038),
 .UNSPECIFIED.,.F.,.F.,(3,3),(0.,1.),.UNSPECIFIED.);
#23061=B_SPLINE_CURVE_WITH_KNOTS('',2,(#77041,#77042,#77043),
 .UNSPECIFIED.,.F.,.F.,(3,3),(0.,1.),.UNSPECIFIED.);
#23062=B_SPLINE_CURVE_WITH_KNOTS('',2,(#77051,#77052,#77053),
 .UNSPECIFIED.,.F.,.F.,(3,3),(0.,1.),.UNSPECIFIED.);
#23063=B_SPLINE_CURVE_WITH_KNOTS('',2,(#77056,#77057,#77058),
 .UNSPECIFIED.,.F.,.F.,(3,3),(0.,1.),.UNSPECIFIED.);
#23064=B_SPLINE_CURVE_WITH_KNOTS('',2,(#77066,#77067,#77068),
 .UNSPECIFIED.,.F.,.F.,(3,3),(0.,1.),.UNSPECIFIED.);
#23065=B_SPLINE_CURVE_WITH_KNOTS('',2,(#77071,#77072,#77073),
 .UNSPECIFIED.,.F.,.F.,(3,3),(0.,1.),.UNSPECIFIED.);
#23066=B_SPLINE_CURVE_WITH_KNOTS('',2,(#77081,#77082,#77083),
 .UNSPECIFIED.,.F.,.F.,(3,3),(0.,1.),.UNSPECIFIED.);
#23067=B_SPLINE_CURVE_WITH_KNOTS('',2,(#77086,#77087,#77088),
 .UNSPECIFIED.,.F.,.F.,(3,3),(0.,1.),.UNSPECIFIED.);
#23068=B_SPLINE_CURVE_WITH_KNOTS('',2,(#77096,#77097,#77098),
 .UNSPECIFIED.,.F.,.F.,(3,3),(0.,1.),.UNSPECIFIED.);
#23069=B_SPLINE_CURVE_WITH_KNOTS('',2,(#77101,#77102,#77103),
 .UNSPECIFIED.,.F.,.F.,(3,3),(0.,1.),.UNSPECIFIED.);
#23070=B_SPLINE_CURVE_WITH_KNOTS('',2,(#77111,#77112,#77113),
 .UNSPECIFIED.,.F.,.F.,(3,3),(0.,1.),.UNSPECIFIED.);
#23071=B_SPLINE_CURVE_WITH_KNOTS('',2,(#77116,#77117,#77118),
 .UNSPECIFIED.,.F.,.F.,(3,3),(0.,1.),.UNSPECIFIED.);
#23072=B_SPLINE_CURVE_WITH_KNOTS('',2,(#77126,#77127,#77128),
 .UNSPECIFIED.,.F.,.F.,(3,3),(0.,1.),.UNSPECIFIED.);
#23073=B_SPLINE_CURVE_WITH_KNOTS('',2,(#77131,#77132,#77133),
 .UNSPECIFIED.,.F.,.F.,(3,3),(0.,1.),.UNSPECIFIED.);
#23074=B_SPLINE_CURVE_WITH_KNOTS('',2,(#77141,#77142,#77143),
 .UNSPECIFIED.,.F.,.F.,(3,3),(0.,1.),.UNSPECIFIED.);
#23075=B_SPLINE_CURVE_WITH_KNOTS('',2,(#77146,#77147,#77148),
 .UNSPECIFIED.,.F.,.F.,(3,3),(0.,1.),.UNSPECIFIED.);
#23076=B_SPLINE_CURVE_WITH_KNOTS('',2,(#77156,#77157,#77158),
 .UNSPECIFIED.,.F.,.F.,(3,3),(0.,1.),.UNSPECIFIED.);
#23077=B_SPLINE_CURVE_WITH_KNOTS('',2,(#77161,#77162,#77163),
 .UNSPECIFIED.,.F.,.F.,(3,3),(0.,1.),.UNSPECIFIED.);
#23078=B_SPLINE_CURVE_WITH_KNOTS('',2,(#77171,#77172,#77173),
 .UNSPECIFIED.,.F.,.F.,(3,3),(0.,1.),.UNSPECIFIED.);
#23079=B_SPLINE_CURVE_WITH_KNOTS('',2,(#77176,#77177,#77178),
 .UNSPECIFIED.,.F.,.F.,(3,3),(0.,1.),.UNSPECIFIED.);
#23080=B_SPLINE_CURVE_WITH_KNOTS('',2,(#77185,#77186,#77187),
 .UNSPECIFIED.,.F.,.F.,(3,3),(0.,1.),.UNSPECIFIED.);
#23081=B_SPLINE_CURVE_WITH_KNOTS('',2,(#77188,#77189,#77190),
 .UNSPECIFIED.,.F.,.F.,(3,3),(0.,1.),.UNSPECIFIED.);
#23082=B_SPLINE_CURVE_WITH_KNOTS('',2,(#77200,#77201,#77202),
 .UNSPECIFIED.,.F.,.F.,(3,3),(0.,1.),.UNSPECIFIED.);
#23083=B_SPLINE_CURVE_WITH_KNOTS('',2,(#77206,#77207,#77208),
 .UNSPECIFIED.,.F.,.F.,(3,3),(0.,1.),.UNSPECIFIED.);
#23084=B_SPLINE_CURVE_WITH_KNOTS('',2,(#77217,#77218,#77219),
 .UNSPECIFIED.,.F.,.F.,(3,3),(0.,1.),.UNSPECIFIED.);
#23085=B_SPLINE_CURVE_WITH_KNOTS('',2,(#77222,#77223,#77224),
 .UNSPECIFIED.,.F.,.F.,(3,3),(0.,1.),.UNSPECIFIED.);
#23086=B_SPLINE_CURVE_WITH_KNOTS('',2,(#77232,#77233,#77234),
 .UNSPECIFIED.,.F.,.F.,(3,3),(0.,1.),.UNSPECIFIED.);
#23087=B_SPLINE_CURVE_WITH_KNOTS('',2,(#77237,#77238,#77239),
 .UNSPECIFIED.,.F.,.F.,(3,3),(0.,1.),.UNSPECIFIED.);
#23088=B_SPLINE_CURVE_WITH_KNOTS('',2,(#77247,#77248,#77249),
 .UNSPECIFIED.,.F.,.F.,(3,3),(0.,1.),.UNSPECIFIED.);
#23089=B_SPLINE_CURVE_WITH_KNOTS('',2,(#77252,#77253,#77254),
 .UNSPECIFIED.,.F.,.F.,(3,3),(0.,1.),.UNSPECIFIED.);
#23090=B_SPLINE_CURVE_WITH_KNOTS('',2,(#77262,#77263,#77264),
 .UNSPECIFIED.,.F.,.F.,(3,3),(0.,1.),.UNSPECIFIED.);
#23091=B_SPLINE_CURVE_WITH_KNOTS('',2,(#77267,#77268,#77269),
 .UNSPECIFIED.,.F.,.F.,(3,3),(0.,1.),.UNSPECIFIED.);
#23092=B_SPLINE_CURVE_WITH_KNOTS('',2,(#77277,#77278,#77279),
 .UNSPECIFIED.,.F.,.F.,(3,3),(0.,1.),.UNSPECIFIED.);
#23093=B_SPLINE_CURVE_WITH_KNOTS('',2,(#77282,#77283,#77284),
 .UNSPECIFIED.,.F.,.F.,(3,3),(0.,1.),.UNSPECIFIED.);
#23094=B_SPLINE_CURVE_WITH_KNOTS('',2,(#77292,#77293,#77294),
 .UNSPECIFIED.,.F.,.F.,(3,3),(0.,1.),.UNSPECIFIED.);
#23095=B_SPLINE_CURVE_WITH_KNOTS('',2,(#77297,#77298,#77299),
 .UNSPECIFIED.,.F.,.F.,(3,3),(0.,1.),.UNSPECIFIED.);
#23096=B_SPLINE_CURVE_WITH_KNOTS('',2,(#77306,#77307,#77308),
 .UNSPECIFIED.,.F.,.F.,(3,3),(0.,1.),.UNSPECIFIED.);
#23097=B_SPLINE_CURVE_WITH_KNOTS('',2,(#77309,#77310,#77311),
 .UNSPECIFIED.,.F.,.F.,(3,3),(0.,1.),.UNSPECIFIED.);
#23098=B_SPLINE_CURVE_WITH_KNOTS('',2,(#77320,#77321,#77322),
 .UNSPECIFIED.,.F.,.F.,(3,3),(0.,1.),.UNSPECIFIED.);
#23099=B_SPLINE_CURVE_WITH_KNOTS('',2,(#77326,#77327,#77328),
 .UNSPECIFIED.,.F.,.F.,(3,3),(0.,1.),.UNSPECIFIED.);
#23100=B_SPLINE_CURVE_WITH_KNOTS('',2,(#77337,#77338,#77339),
 .UNSPECIFIED.,.F.,.F.,(3,3),(0.,1.),.UNSPECIFIED.);
#23101=B_SPLINE_CURVE_WITH_KNOTS('',2,(#77342,#77343,#77344),
 .UNSPECIFIED.,.F.,.F.,(3,3),(0.,1.),.UNSPECIFIED.);
#23102=B_SPLINE_CURVE_WITH_KNOTS('',2,(#77352,#77353,#77354),
 .UNSPECIFIED.,.F.,.F.,(3,3),(0.,1.),.UNSPECIFIED.);
#23103=B_SPLINE_CURVE_WITH_KNOTS('',2,(#77357,#77358,#77359),
 .UNSPECIFIED.,.F.,.F.,(3,3),(0.,1.),.UNSPECIFIED.);
#23104=B_SPLINE_CURVE_WITH_KNOTS('',2,(#77367,#77368,#77369),
 .UNSPECIFIED.,.F.,.F.,(3,3),(0.,1.),.UNSPECIFIED.);
#23105=B_SPLINE_CURVE_WITH_KNOTS('',2,(#77372,#77373,#77374),
 .UNSPECIFIED.,.F.,.F.,(3,3),(0.,1.),.UNSPECIFIED.);
#23106=B_SPLINE_CURVE_WITH_KNOTS('',2,(#77382,#77383,#77384),
 .UNSPECIFIED.,.F.,.F.,(3,3),(0.,1.),.UNSPECIFIED.);
#23107=B_SPLINE_CURVE_WITH_KNOTS('',2,(#77387,#77388,#77389),
 .UNSPECIFIED.,.F.,.F.,(3,3),(0.,1.),.UNSPECIFIED.);
#23108=B_SPLINE_CURVE_WITH_KNOTS('',2,(#77397,#77398,#77399),
 .UNSPECIFIED.,.F.,.F.,(3,3),(0.,1.),.UNSPECIFIED.);
#23109=B_SPLINE_CURVE_WITH_KNOTS('',2,(#77402,#77403,#77404),
 .UNSPECIFIED.,.F.,.F.,(3,3),(0.,1.),.UNSPECIFIED.);
#23110=B_SPLINE_CURVE_WITH_KNOTS('',2,(#77412,#77413,#77414),
 .UNSPECIFIED.,.F.,.F.,(3,3),(0.,1.),.UNSPECIFIED.);
#23111=B_SPLINE_CURVE_WITH_KNOTS('',2,(#77417,#77418,#77419),
 .UNSPECIFIED.,.F.,.F.,(3,3),(0.,1.),.UNSPECIFIED.);
#23112=B_SPLINE_CURVE_WITH_KNOTS('',2,(#77427,#77428,#77429),
 .UNSPECIFIED.,.F.,.F.,(3,3),(0.,1.),.UNSPECIFIED.);
#23113=B_SPLINE_CURVE_WITH_KNOTS('',2,(#77432,#77433,#77434),
 .UNSPECIFIED.,.F.,.F.,(3,3),(0.,1.),.UNSPECIFIED.);
#23114=B_SPLINE_CURVE_WITH_KNOTS('',2,(#77441,#77442,#77443),
 .UNSPECIFIED.,.F.,.F.,(3,3),(0.,1.),.UNSPECIFIED.);
#23115=B_SPLINE_CURVE_WITH_KNOTS('',2,(#77444,#77445,#77446),
 .UNSPECIFIED.,.F.,.F.,(3,3),(0.,1.),.UNSPECIFIED.);
#23116=B_SPLINE_CURVE_WITH_KNOTS('',2,(#77455,#77456,#77457),
 .UNSPECIFIED.,.F.,.F.,(3,3),(0.,1.),.UNSPECIFIED.);
#23117=B_SPLINE_CURVE_WITH_KNOTS('',2,(#77461,#77462,#77463),
 .UNSPECIFIED.,.F.,.F.,(3,3),(0.,1.),.UNSPECIFIED.);
#23118=B_SPLINE_CURVE_WITH_KNOTS('',2,(#77472,#77473,#77474),
 .UNSPECIFIED.,.F.,.F.,(3,3),(0.,1.),.UNSPECIFIED.);
#23119=B_SPLINE_CURVE_WITH_KNOTS('',2,(#77477,#77478,#77479),
 .UNSPECIFIED.,.F.,.F.,(3,3),(0.,1.),.UNSPECIFIED.);
#23120=B_SPLINE_CURVE_WITH_KNOTS('',2,(#77487,#77488,#77489),
 .UNSPECIFIED.,.F.,.F.,(3,3),(0.,1.),.UNSPECIFIED.);
#23121=B_SPLINE_CURVE_WITH_KNOTS('',2,(#77492,#77493,#77494),
 .UNSPECIFIED.,.F.,.F.,(3,3),(0.,1.),.UNSPECIFIED.);
#23122=B_SPLINE_CURVE_WITH_KNOTS('',2,(#77502,#77503,#77504),
 .UNSPECIFIED.,.F.,.F.,(3,3),(0.,1.),.UNSPECIFIED.);
#23123=B_SPLINE_CURVE_WITH_KNOTS('',2,(#77507,#77508,#77509),
 .UNSPECIFIED.,.F.,.F.,(3,3),(0.,1.),.UNSPECIFIED.);
#23124=B_SPLINE_CURVE_WITH_KNOTS('',2,(#77517,#77518,#77519),
 .UNSPECIFIED.,.F.,.F.,(3,3),(0.,1.),.UNSPECIFIED.);
#23125=B_SPLINE_CURVE_WITH_KNOTS('',2,(#77522,#77523,#77524),
 .UNSPECIFIED.,.F.,.F.,(3,3),(0.,1.),.UNSPECIFIED.);
#23126=B_SPLINE_CURVE_WITH_KNOTS('',2,(#77532,#77533,#77534),
 .UNSPECIFIED.,.F.,.F.,(3,3),(0.,1.),.UNSPECIFIED.);
#23127=B_SPLINE_CURVE_WITH_KNOTS('',2,(#77537,#77538,#77539),
 .UNSPECIFIED.,.F.,.F.,(3,3),(0.,1.),.UNSPECIFIED.);
#23128=B_SPLINE_CURVE_WITH_KNOTS('',2,(#77547,#77548,#77549),
 .UNSPECIFIED.,.F.,.F.,(3,3),(0.,1.),.UNSPECIFIED.);
#23129=B_SPLINE_CURVE_WITH_KNOTS('',2,(#77552,#77553,#77554),
 .UNSPECIFIED.,.F.,.F.,(3,3),(0.,1.),.UNSPECIFIED.);
#23130=B_SPLINE_CURVE_WITH_KNOTS('',2,(#77562,#77563,#77564),
 .UNSPECIFIED.,.F.,.F.,(3,3),(0.,1.),.UNSPECIFIED.);
#23131=B_SPLINE_CURVE_WITH_KNOTS('',2,(#77567,#77568,#77569),
 .UNSPECIFIED.,.F.,.F.,(3,3),(0.,1.),.UNSPECIFIED.);
#23132=B_SPLINE_CURVE_WITH_KNOTS('',2,(#77577,#77578,#77579),
 .UNSPECIFIED.,.F.,.F.,(3,3),(0.,1.),.UNSPECIFIED.);
#23133=B_SPLINE_CURVE_WITH_KNOTS('',2,(#77582,#77583,#77584),
 .UNSPECIFIED.,.F.,.F.,(3,3),(0.,1.),.UNSPECIFIED.);
#23134=B_SPLINE_CURVE_WITH_KNOTS('',2,(#77592,#77593,#77594),
 .UNSPECIFIED.,.F.,.F.,(3,3),(0.,1.),.UNSPECIFIED.);
#23135=B_SPLINE_CURVE_WITH_KNOTS('',2,(#77597,#77598,#77599),
 .UNSPECIFIED.,.F.,.F.,(3,3),(0.,1.),.UNSPECIFIED.);
#23136=B_SPLINE_CURVE_WITH_KNOTS('',2,(#77607,#77608,#77609),
 .UNSPECIFIED.,.F.,.F.,(3,3),(0.,1.),.UNSPECIFIED.);
#23137=B_SPLINE_CURVE_WITH_KNOTS('',2,(#77612,#77613,#77614),
 .UNSPECIFIED.,.F.,.F.,(3,3),(0.,1.),.UNSPECIFIED.);
#23138=B_SPLINE_CURVE_WITH_KNOTS('',2,(#77622,#77623,#77624),
 .UNSPECIFIED.,.F.,.F.,(3,3),(0.,1.),.UNSPECIFIED.);
#23139=B_SPLINE_CURVE_WITH_KNOTS('',2,(#77627,#77628,#77629),
 .UNSPECIFIED.,.F.,.F.,(3,3),(0.,1.),.UNSPECIFIED.);
#23140=B_SPLINE_CURVE_WITH_KNOTS('',2,(#77637,#77638,#77639),
 .UNSPECIFIED.,.F.,.F.,(3,3),(0.,1.),.UNSPECIFIED.);
#23141=B_SPLINE_CURVE_WITH_KNOTS('',2,(#77642,#77643,#77644),
 .UNSPECIFIED.,.F.,.F.,(3,3),(0.,1.),.UNSPECIFIED.);
#23142=B_SPLINE_CURVE_WITH_KNOTS('',2,(#77652,#77653,#77654),
 .UNSPECIFIED.,.F.,.F.,(3,3),(0.,1.),.UNSPECIFIED.);
#23143=B_SPLINE_CURVE_WITH_KNOTS('',2,(#77657,#77658,#77659),
 .UNSPECIFIED.,.F.,.F.,(3,3),(0.,1.),.UNSPECIFIED.);
#23144=B_SPLINE_CURVE_WITH_KNOTS('',2,(#77667,#77668,#77669),
 .UNSPECIFIED.,.F.,.F.,(3,3),(0.,1.),.UNSPECIFIED.);
#23145=B_SPLINE_CURVE_WITH_KNOTS('',2,(#77672,#77673,#77674),
 .UNSPECIFIED.,.F.,.F.,(3,3),(0.,1.),.UNSPECIFIED.);
#23146=B_SPLINE_CURVE_WITH_KNOTS('',2,(#77681,#77682,#77683),
 .UNSPECIFIED.,.F.,.F.,(3,3),(0.,1.),.UNSPECIFIED.);
#23147=B_SPLINE_CURVE_WITH_KNOTS('',2,(#77684,#77685,#77686),
 .UNSPECIFIED.,.F.,.F.,(3,3),(0.,1.),.UNSPECIFIED.);
#23148=B_SPLINE_CURVE_WITH_KNOTS('',2,(#77699,#77700,#77701),
 .UNSPECIFIED.,.F.,.F.,(3,3),(0.,1.),.UNSPECIFIED.);
#23149=B_SPLINE_CURVE_WITH_KNOTS('',2,(#77705,#77706,#77707),
 .UNSPECIFIED.,.F.,.F.,(3,3),(0.,1.),.UNSPECIFIED.);
#23150=B_SPLINE_CURVE_WITH_KNOTS('',2,(#77716,#77717,#77718),
 .UNSPECIFIED.,.F.,.F.,(3,3),(0.,1.),.UNSPECIFIED.);
#23151=B_SPLINE_CURVE_WITH_KNOTS('',2,(#77721,#77722,#77723),
 .UNSPECIFIED.,.F.,.F.,(3,3),(0.,1.),.UNSPECIFIED.);
#23152=B_SPLINE_CURVE_WITH_KNOTS('',2,(#77731,#77732,#77733),
 .UNSPECIFIED.,.F.,.F.,(3,3),(0.,1.),.UNSPECIFIED.);
#23153=B_SPLINE_CURVE_WITH_KNOTS('',2,(#77736,#77737,#77738),
 .UNSPECIFIED.,.F.,.F.,(3,3),(0.,1.),.UNSPECIFIED.);
#23154=B_SPLINE_CURVE_WITH_KNOTS('',2,(#77746,#77747,#77748),
 .UNSPECIFIED.,.F.,.F.,(3,3),(0.,1.),.UNSPECIFIED.);
#23155=B_SPLINE_CURVE_WITH_KNOTS('',2,(#77751,#77752,#77753),
 .UNSPECIFIED.,.F.,.F.,(3,3),(0.,1.),.UNSPECIFIED.);
#23156=B_SPLINE_CURVE_WITH_KNOTS('',2,(#77761,#77762,#77763),
 .UNSPECIFIED.,.F.,.F.,(3,3),(0.,1.),.UNSPECIFIED.);
#23157=B_SPLINE_CURVE_WITH_KNOTS('',2,(#77766,#77767,#77768),
 .UNSPECIFIED.,.F.,.F.,(3,3),(0.,1.),.UNSPECIFIED.);
#23158=B_SPLINE_CURVE_WITH_KNOTS('',2,(#77776,#77777,#77778),
 .UNSPECIFIED.,.F.,.F.,(3,3),(0.,1.),.UNSPECIFIED.);
#23159=B_SPLINE_CURVE_WITH_KNOTS('',2,(#77781,#77782,#77783),
 .UNSPECIFIED.,.F.,.F.,(3,3),(0.,1.),.UNSPECIFIED.);
#23160=B_SPLINE_CURVE_WITH_KNOTS('',2,(#77791,#77792,#77793),
 .UNSPECIFIED.,.F.,.F.,(3,3),(0.,1.),.UNSPECIFIED.);
#23161=B_SPLINE_CURVE_WITH_KNOTS('',2,(#77796,#77797,#77798),
 .UNSPECIFIED.,.F.,.F.,(3,3),(0.,1.),.UNSPECIFIED.);
#23162=B_SPLINE_CURVE_WITH_KNOTS('',2,(#77805,#77806,#77807),
 .UNSPECIFIED.,.F.,.F.,(3,3),(0.,1.),.UNSPECIFIED.);
#23163=B_SPLINE_CURVE_WITH_KNOTS('',2,(#77808,#77809,#77810),
 .UNSPECIFIED.,.F.,.F.,(3,3),(0.,1.),.UNSPECIFIED.);
#23164=B_SPLINE_CURVE_WITH_KNOTS('',2,(#77819,#77820,#77821),
 .UNSPECIFIED.,.F.,.F.,(3,3),(0.,1.),.UNSPECIFIED.);
#23165=B_SPLINE_CURVE_WITH_KNOTS('',2,(#77825,#77826,#77827),
 .UNSPECIFIED.,.F.,.F.,(3,3),(0.,1.),.UNSPECIFIED.);
#23166=B_SPLINE_CURVE_WITH_KNOTS('',2,(#77836,#77837,#77838),
 .UNSPECIFIED.,.F.,.F.,(3,3),(0.,1.),.UNSPECIFIED.);
#23167=B_SPLINE_CURVE_WITH_KNOTS('',2,(#77841,#77842,#77843),
 .UNSPECIFIED.,.F.,.F.,(3,3),(0.,1.),.UNSPECIFIED.);
#23168=B_SPLINE_CURVE_WITH_KNOTS('',2,(#77851,#77852,#77853),
 .UNSPECIFIED.,.F.,.F.,(3,3),(0.,1.),.UNSPECIFIED.);
#23169=B_SPLINE_CURVE_WITH_KNOTS('',2,(#77856,#77857,#77858),
 .UNSPECIFIED.,.F.,.F.,(3,3),(0.,1.),.UNSPECIFIED.);
#23170=B_SPLINE_CURVE_WITH_KNOTS('',2,(#77866,#77867,#77868),
 .UNSPECIFIED.,.F.,.F.,(3,3),(0.,1.),.UNSPECIFIED.);
#23171=B_SPLINE_CURVE_WITH_KNOTS('',2,(#77871,#77872,#77873),
 .UNSPECIFIED.,.F.,.F.,(3,3),(0.,1.),.UNSPECIFIED.);
#23172=B_SPLINE_CURVE_WITH_KNOTS('',2,(#77881,#77882,#77883),
 .UNSPECIFIED.,.F.,.F.,(3,3),(0.,1.),.UNSPECIFIED.);
#23173=B_SPLINE_CURVE_WITH_KNOTS('',2,(#77886,#77887,#77888),
 .UNSPECIFIED.,.F.,.F.,(3,3),(0.,1.),.UNSPECIFIED.);
#23174=B_SPLINE_CURVE_WITH_KNOTS('',2,(#77896,#77897,#77898),
 .UNSPECIFIED.,.F.,.F.,(3,3),(0.,1.),.UNSPECIFIED.);
#23175=B_SPLINE_CURVE_WITH_KNOTS('',2,(#77901,#77902,#77903),
 .UNSPECIFIED.,.F.,.F.,(3,3),(0.,1.),.UNSPECIFIED.);
#23176=B_SPLINE_CURVE_WITH_KNOTS('',2,(#77911,#77912,#77913),
 .UNSPECIFIED.,.F.,.F.,(3,3),(0.,1.),.UNSPECIFIED.);
#23177=B_SPLINE_CURVE_WITH_KNOTS('',2,(#77916,#77917,#77918),
 .UNSPECIFIED.,.F.,.F.,(3,3),(0.,1.),.UNSPECIFIED.);
#23178=B_SPLINE_CURVE_WITH_KNOTS('',2,(#77926,#77927,#77928),
 .UNSPECIFIED.,.F.,.F.,(3,3),(0.,1.),.UNSPECIFIED.);
#23179=B_SPLINE_CURVE_WITH_KNOTS('',2,(#77931,#77932,#77933),
 .UNSPECIFIED.,.F.,.F.,(3,3),(0.,1.),.UNSPECIFIED.);
#23180=B_SPLINE_CURVE_WITH_KNOTS('',2,(#77941,#77942,#77943),
 .UNSPECIFIED.,.F.,.F.,(3,3),(0.,1.),.UNSPECIFIED.);
#23181=B_SPLINE_CURVE_WITH_KNOTS('',2,(#77946,#77947,#77948),
 .UNSPECIFIED.,.F.,.F.,(3,3),(0.,1.),.UNSPECIFIED.);
#23182=B_SPLINE_CURVE_WITH_KNOTS('',2,(#77956,#77957,#77958),
 .UNSPECIFIED.,.F.,.F.,(3,3),(0.,1.),.UNSPECIFIED.);
#23183=B_SPLINE_CURVE_WITH_KNOTS('',2,(#77961,#77962,#77963),
 .UNSPECIFIED.,.F.,.F.,(3,3),(0.,1.),.UNSPECIFIED.);
#23184=B_SPLINE_CURVE_WITH_KNOTS('',2,(#77971,#77972,#77973),
 .UNSPECIFIED.,.F.,.F.,(3,3),(0.,1.),.UNSPECIFIED.);
#23185=B_SPLINE_CURVE_WITH_KNOTS('',2,(#77976,#77977,#77978),
 .UNSPECIFIED.,.F.,.F.,(3,3),(0.,1.),.UNSPECIFIED.);
#23186=B_SPLINE_CURVE_WITH_KNOTS('',2,(#77985,#77986,#77987),
 .UNSPECIFIED.,.F.,.F.,(3,3),(0.,1.),.UNSPECIFIED.);
#23187=B_SPLINE_CURVE_WITH_KNOTS('',2,(#77988,#77989,#77990),
 .UNSPECIFIED.,.F.,.F.,(3,3),(0.,1.),.UNSPECIFIED.);
#23188=B_SPLINE_CURVE_WITH_KNOTS('',2,(#78000,#78001,#78002),
 .UNSPECIFIED.,.F.,.F.,(3,3),(0.,1.),.UNSPECIFIED.);
#23189=B_SPLINE_CURVE_WITH_KNOTS('',2,(#78006,#78007,#78008),
 .UNSPECIFIED.,.F.,.F.,(3,3),(0.,1.),.UNSPECIFIED.);
#23190=B_SPLINE_CURVE_WITH_KNOTS('',2,(#78017,#78018,#78019),
 .UNSPECIFIED.,.F.,.F.,(3,3),(0.,1.),.UNSPECIFIED.);
#23191=B_SPLINE_CURVE_WITH_KNOTS('',2,(#78022,#78023,#78024),
 .UNSPECIFIED.,.F.,.F.,(3,3),(0.,1.),.UNSPECIFIED.);
#23192=B_SPLINE_CURVE_WITH_KNOTS('',2,(#78032,#78033,#78034),
 .UNSPECIFIED.,.F.,.F.,(3,3),(0.,1.),.UNSPECIFIED.);
#23193=B_SPLINE_CURVE_WITH_KNOTS('',2,(#78037,#78038,#78039),
 .UNSPECIFIED.,.F.,.F.,(3,3),(0.,1.),.UNSPECIFIED.);
#23194=B_SPLINE_CURVE_WITH_KNOTS('',2,(#78053,#78054,#78055),
 .UNSPECIFIED.,.F.,.F.,(3,3),(0.,1.),.UNSPECIFIED.);
#23195=B_SPLINE_CURVE_WITH_KNOTS('',2,(#78058,#78059,#78060),
 .UNSPECIFIED.,.F.,.F.,(3,3),(0.,1.),.UNSPECIFIED.);
#23196=B_SPLINE_CURVE_WITH_KNOTS('',2,(#78068,#78069,#78070),
 .UNSPECIFIED.,.F.,.F.,(3,3),(0.,1.),.UNSPECIFIED.);
#23197=B_SPLINE_CURVE_WITH_KNOTS('',2,(#78073,#78074,#78075),
 .UNSPECIFIED.,.F.,.F.,(3,3),(0.,1.),.UNSPECIFIED.);
#23198=B_SPLINE_CURVE_WITH_KNOTS('',2,(#78083,#78084,#78085),
 .UNSPECIFIED.,.F.,.F.,(3,3),(0.,1.),.UNSPECIFIED.);
#23199=B_SPLINE_CURVE_WITH_KNOTS('',2,(#78088,#78089,#78090),
 .UNSPECIFIED.,.F.,.F.,(3,3),(0.,1.),.UNSPECIFIED.);
#23200=B_SPLINE_CURVE_WITH_KNOTS('',2,(#78122,#78123,#78124),
 .UNSPECIFIED.,.F.,.F.,(3,3),(0.,1.),.UNSPECIFIED.);
#23201=B_SPLINE_CURVE_WITH_KNOTS('',2,(#78128,#78129,#78130),
 .UNSPECIFIED.,.F.,.F.,(3,3),(0.,1.),.UNSPECIFIED.);
#23202=B_SPLINE_CURVE_WITH_KNOTS('',2,(#78139,#78140,#78141),
 .UNSPECIFIED.,.F.,.F.,(3,3),(0.,1.),.UNSPECIFIED.);
#23203=B_SPLINE_CURVE_WITH_KNOTS('',2,(#78144,#78145,#78146),
 .UNSPECIFIED.,.F.,.F.,(3,3),(0.,1.),.UNSPECIFIED.);
#23204=B_SPLINE_CURVE_WITH_KNOTS('',2,(#78154,#78155,#78156),
 .UNSPECIFIED.,.F.,.F.,(3,3),(0.,1.),.UNSPECIFIED.);
#23205=B_SPLINE_CURVE_WITH_KNOTS('',2,(#78159,#78160,#78161),
 .UNSPECIFIED.,.F.,.F.,(3,3),(0.,1.),.UNSPECIFIED.);
#23206=B_SPLINE_CURVE_WITH_KNOTS('',2,(#78169,#78170,#78171),
 .UNSPECIFIED.,.F.,.F.,(3,3),(0.,1.),.UNSPECIFIED.);
#23207=B_SPLINE_CURVE_WITH_KNOTS('',2,(#78174,#78175,#78176),
 .UNSPECIFIED.,.F.,.F.,(3,3),(0.,1.),.UNSPECIFIED.);
#23208=B_SPLINE_CURVE_WITH_KNOTS('',2,(#78184,#78185,#78186),
 .UNSPECIFIED.,.F.,.F.,(3,3),(0.,1.),.UNSPECIFIED.);
#23209=B_SPLINE_CURVE_WITH_KNOTS('',2,(#78189,#78190,#78191),
 .UNSPECIFIED.,.F.,.F.,(3,3),(0.,1.),.UNSPECIFIED.);
#23210=B_SPLINE_CURVE_WITH_KNOTS('',2,(#78199,#78200,#78201),
 .UNSPECIFIED.,.F.,.F.,(3,3),(0.,1.),.UNSPECIFIED.);
#23211=B_SPLINE_CURVE_WITH_KNOTS('',2,(#78204,#78205,#78206),
 .UNSPECIFIED.,.F.,.F.,(3,3),(0.,1.),.UNSPECIFIED.);
#23212=B_SPLINE_CURVE_WITH_KNOTS('',2,(#78214,#78215,#78216),
 .UNSPECIFIED.,.F.,.F.,(3,3),(0.,1.),.UNSPECIFIED.);
#23213=B_SPLINE_CURVE_WITH_KNOTS('',2,(#78219,#78220,#78221),
 .UNSPECIFIED.,.F.,.F.,(3,3),(0.,1.),.UNSPECIFIED.);
#23214=B_SPLINE_CURVE_WITH_KNOTS('',2,(#78228,#78229,#78230),
 .UNSPECIFIED.,.F.,.F.,(3,3),(0.,1.),.UNSPECIFIED.);
#23215=B_SPLINE_CURVE_WITH_KNOTS('',2,(#78231,#78232,#78233),
 .UNSPECIFIED.,.F.,.F.,(3,3),(0.,1.),.UNSPECIFIED.);
#23216=B_SPLINE_CURVE_WITH_KNOTS('',2,(#78242,#78243,#78244),
 .UNSPECIFIED.,.F.,.F.,(3,3),(0.,1.),.UNSPECIFIED.);
#23217=B_SPLINE_CURVE_WITH_KNOTS('',2,(#78248,#78249,#78250),
 .UNSPECIFIED.,.F.,.F.,(3,3),(0.,1.),.UNSPECIFIED.);
#23218=B_SPLINE_CURVE_WITH_KNOTS('',2,(#78259,#78260,#78261),
 .UNSPECIFIED.,.F.,.F.,(3,3),(0.,1.),.UNSPECIFIED.);
#23219=B_SPLINE_CURVE_WITH_KNOTS('',2,(#78264,#78265,#78266),
 .UNSPECIFIED.,.F.,.F.,(3,3),(0.,1.),.UNSPECIFIED.);
#23220=B_SPLINE_CURVE_WITH_KNOTS('',2,(#78274,#78275,#78276),
 .UNSPECIFIED.,.F.,.F.,(3,3),(0.,1.),.UNSPECIFIED.);
#23221=B_SPLINE_CURVE_WITH_KNOTS('',2,(#78279,#78280,#78281),
 .UNSPECIFIED.,.F.,.F.,(3,3),(0.,1.),.UNSPECIFIED.);
#23222=B_SPLINE_CURVE_WITH_KNOTS('',2,(#78289,#78290,#78291),
 .UNSPECIFIED.,.F.,.F.,(3,3),(0.,1.),.UNSPECIFIED.);
#23223=B_SPLINE_CURVE_WITH_KNOTS('',2,(#78294,#78295,#78296),
 .UNSPECIFIED.,.F.,.F.,(3,3),(0.,1.),.UNSPECIFIED.);
#23224=B_SPLINE_CURVE_WITH_KNOTS('',2,(#78304,#78305,#78306),
 .UNSPECIFIED.,.F.,.F.,(3,3),(0.,1.),.UNSPECIFIED.);
#23225=B_SPLINE_CURVE_WITH_KNOTS('',2,(#78309,#78310,#78311),
 .UNSPECIFIED.,.F.,.F.,(3,3),(0.,1.),.UNSPECIFIED.);
#23226=B_SPLINE_CURVE_WITH_KNOTS('',2,(#78319,#78320,#78321),
 .UNSPECIFIED.,.F.,.F.,(3,3),(0.,1.),.UNSPECIFIED.);
#23227=B_SPLINE_CURVE_WITH_KNOTS('',2,(#78324,#78325,#78326),
 .UNSPECIFIED.,.F.,.F.,(3,3),(0.,1.),.UNSPECIFIED.);
#23228=B_SPLINE_CURVE_WITH_KNOTS('',2,(#78334,#78335,#78336),
 .UNSPECIFIED.,.F.,.F.,(3,3),(0.,1.),.UNSPECIFIED.);
#23229=B_SPLINE_CURVE_WITH_KNOTS('',2,(#78339,#78340,#78341),
 .UNSPECIFIED.,.F.,.F.,(3,3),(0.,1.),.UNSPECIFIED.);
#23230=B_SPLINE_CURVE_WITH_KNOTS('',2,(#78349,#78350,#78351),
 .UNSPECIFIED.,.F.,.F.,(3,3),(0.,1.),.UNSPECIFIED.);
#23231=B_SPLINE_CURVE_WITH_KNOTS('',2,(#78354,#78355,#78356),
 .UNSPECIFIED.,.F.,.F.,(3,3),(0.,1.),.UNSPECIFIED.);
#23232=B_SPLINE_CURVE_WITH_KNOTS('',2,(#78364,#78365,#78366),
 .UNSPECIFIED.,.F.,.F.,(3,3),(0.,1.),.UNSPECIFIED.);
#23233=B_SPLINE_CURVE_WITH_KNOTS('',2,(#78369,#78370,#78371),
 .UNSPECIFIED.,.F.,.F.,(3,3),(0.,1.),.UNSPECIFIED.);
#23234=B_SPLINE_CURVE_WITH_KNOTS('',2,(#78379,#78380,#78381),
 .UNSPECIFIED.,.F.,.F.,(3,3),(0.,1.),.UNSPECIFIED.);
#23235=B_SPLINE_CURVE_WITH_KNOTS('',2,(#78384,#78385,#78386),
 .UNSPECIFIED.,.F.,.F.,(3,3),(0.,1.),.UNSPECIFIED.);
#23236=B_SPLINE_CURVE_WITH_KNOTS('',2,(#78394,#78395,#78396),
 .UNSPECIFIED.,.F.,.F.,(3,3),(0.,1.),.UNSPECIFIED.);
#23237=B_SPLINE_CURVE_WITH_KNOTS('',2,(#78399,#78400,#78401),
 .UNSPECIFIED.,.F.,.F.,(3,3),(0.,1.),.UNSPECIFIED.);
#23238=B_SPLINE_CURVE_WITH_KNOTS('',2,(#78408,#78409,#78410),
 .UNSPECIFIED.,.F.,.F.,(3,3),(0.,1.),.UNSPECIFIED.);
#23239=B_SPLINE_CURVE_WITH_KNOTS('',2,(#78411,#78412,#78413),
 .UNSPECIFIED.,.F.,.F.,(3,3),(0.,1.),.UNSPECIFIED.);
#23240=B_SPLINE_CURVE_WITH_KNOTS('',2,(#78423,#78424,#78425),
 .UNSPECIFIED.,.F.,.F.,(3,3),(0.,1.),.UNSPECIFIED.);
#23241=B_SPLINE_CURVE_WITH_KNOTS('',2,(#78429,#78430,#78431),
 .UNSPECIFIED.,.F.,.F.,(3,3),(0.,1.),.UNSPECIFIED.);
#23242=B_SPLINE_CURVE_WITH_KNOTS('',2,(#78440,#78441,#78442),
 .UNSPECIFIED.,.F.,.F.,(3,3),(0.,1.),.UNSPECIFIED.);
#23243=B_SPLINE_CURVE_WITH_KNOTS('',2,(#78445,#78446,#78447),
 .UNSPECIFIED.,.F.,.F.,(3,3),(0.,1.),.UNSPECIFIED.);
#23244=B_SPLINE_CURVE_WITH_KNOTS('',2,(#78455,#78456,#78457),
 .UNSPECIFIED.,.F.,.F.,(3,3),(0.,1.),.UNSPECIFIED.);
#23245=B_SPLINE_CURVE_WITH_KNOTS('',2,(#78460,#78461,#78462),
 .UNSPECIFIED.,.F.,.F.,(3,3),(0.,1.),.UNSPECIFIED.);
#23246=B_SPLINE_CURVE_WITH_KNOTS('',2,(#78470,#78471,#78472),
 .UNSPECIFIED.,.F.,.F.,(3,3),(0.,1.),.UNSPECIFIED.);
#23247=B_SPLINE_CURVE_WITH_KNOTS('',2,(#78475,#78476,#78477),
 .UNSPECIFIED.,.F.,.F.,(3,3),(0.,1.),.UNSPECIFIED.);
#23248=B_SPLINE_CURVE_WITH_KNOTS('',2,(#78485,#78486,#78487),
 .UNSPECIFIED.,.F.,.F.,(3,3),(0.,1.),.UNSPECIFIED.);
#23249=B_SPLINE_CURVE_WITH_KNOTS('',2,(#78490,#78491,#78492),
 .UNSPECIFIED.,.F.,.F.,(3,3),(0.,1.),.UNSPECIFIED.);
#23250=B_SPLINE_CURVE_WITH_KNOTS('',2,(#78500,#78501,#78502),
 .UNSPECIFIED.,.F.,.F.,(3,3),(0.,1.),.UNSPECIFIED.);
#23251=B_SPLINE_CURVE_WITH_KNOTS('',2,(#78505,#78506,#78507),
 .UNSPECIFIED.,.F.,.F.,(3,3),(0.,1.),.UNSPECIFIED.);
#23252=B_SPLINE_CURVE_WITH_KNOTS('',2,(#78515,#78516,#78517),
 .UNSPECIFIED.,.F.,.F.,(3,3),(0.,1.),.UNSPECIFIED.);
#23253=B_SPLINE_CURVE_WITH_KNOTS('',2,(#78520,#78521,#78522),
 .UNSPECIFIED.,.F.,.F.,(3,3),(0.,1.),.UNSPECIFIED.);
#23254=B_SPLINE_CURVE_WITH_KNOTS('',2,(#78530,#78531,#78532),
 .UNSPECIFIED.,.F.,.F.,(3,3),(0.,1.),.UNSPECIFIED.);
#23255=B_SPLINE_CURVE_WITH_KNOTS('',2,(#78535,#78536,#78537),
 .UNSPECIFIED.,.F.,.F.,(3,3),(0.,1.),.UNSPECIFIED.);
#23256=B_SPLINE_CURVE_WITH_KNOTS('',2,(#78544,#78545,#78546),
 .UNSPECIFIED.,.F.,.F.,(3,3),(0.,1.),.UNSPECIFIED.);
#23257=B_SPLINE_CURVE_WITH_KNOTS('',2,(#78547,#78548,#78549),
 .UNSPECIFIED.,.F.,.F.,(3,3),(0.,1.),.UNSPECIFIED.);
#23258=B_SPLINE_CURVE_WITH_KNOTS('',2,(#78558,#78559,#78560),
 .UNSPECIFIED.,.F.,.F.,(3,3),(0.,1.),.UNSPECIFIED.);
#23259=B_SPLINE_CURVE_WITH_KNOTS('',2,(#78564,#78565,#78566),
 .UNSPECIFIED.,.F.,.F.,(3,3),(0.,1.),.UNSPECIFIED.);
#23260=B_SPLINE_CURVE_WITH_KNOTS('',2,(#78575,#78576,#78577),
 .UNSPECIFIED.,.F.,.F.,(3,3),(0.,1.),.UNSPECIFIED.);
#23261=B_SPLINE_CURVE_WITH_KNOTS('',2,(#78580,#78581,#78582),
 .UNSPECIFIED.,.F.,.F.,(3,3),(0.,1.),.UNSPECIFIED.);
#23262=B_SPLINE_CURVE_WITH_KNOTS('',2,(#78590,#78591,#78592),
 .UNSPECIFIED.,.F.,.F.,(3,3),(0.,1.),.UNSPECIFIED.);
#23263=B_SPLINE_CURVE_WITH_KNOTS('',2,(#78595,#78596,#78597),
 .UNSPECIFIED.,.F.,.F.,(3,3),(0.,1.),.UNSPECIFIED.);
#23264=B_SPLINE_CURVE_WITH_KNOTS('',2,(#78605,#78606,#78607),
 .UNSPECIFIED.,.F.,.F.,(3,3),(0.,1.),.UNSPECIFIED.);
#23265=B_SPLINE_CURVE_WITH_KNOTS('',2,(#78610,#78611,#78612),
 .UNSPECIFIED.,.F.,.F.,(3,3),(0.,1.),.UNSPECIFIED.);
#23266=B_SPLINE_CURVE_WITH_KNOTS('',2,(#78620,#78621,#78622),
 .UNSPECIFIED.,.F.,.F.,(3,3),(0.,1.),.UNSPECIFIED.);
#23267=B_SPLINE_CURVE_WITH_KNOTS('',2,(#78625,#78626,#78627),
 .UNSPECIFIED.,.F.,.F.,(3,3),(0.,1.),.UNSPECIFIED.);
#23268=B_SPLINE_CURVE_WITH_KNOTS('',2,(#78635,#78636,#78637),
 .UNSPECIFIED.,.F.,.F.,(3,3),(0.,1.),.UNSPECIFIED.);
#23269=B_SPLINE_CURVE_WITH_KNOTS('',2,(#78640,#78641,#78642),
 .UNSPECIFIED.,.F.,.F.,(3,3),(0.,1.),.UNSPECIFIED.);
#23270=B_SPLINE_CURVE_WITH_KNOTS('',2,(#78650,#78651,#78652),
 .UNSPECIFIED.,.F.,.F.,(3,3),(0.,1.),.UNSPECIFIED.);
#23271=B_SPLINE_CURVE_WITH_KNOTS('',2,(#78655,#78656,#78657),
 .UNSPECIFIED.,.F.,.F.,(3,3),(0.,1.),.UNSPECIFIED.);
#23272=B_SPLINE_CURVE_WITH_KNOTS('',2,(#78665,#78666,#78667),
 .UNSPECIFIED.,.F.,.F.,(3,3),(0.,1.),.UNSPECIFIED.);
#23273=B_SPLINE_CURVE_WITH_KNOTS('',2,(#78670,#78671,#78672),
 .UNSPECIFIED.,.F.,.F.,(3,3),(0.,1.),.UNSPECIFIED.);
#23274=B_SPLINE_CURVE_WITH_KNOTS('',2,(#78680,#78681,#78682),
 .UNSPECIFIED.,.F.,.F.,(3,3),(0.,1.),.UNSPECIFIED.);
#23275=B_SPLINE_CURVE_WITH_KNOTS('',2,(#78685,#78686,#78687),
 .UNSPECIFIED.,.F.,.F.,(3,3),(0.,1.),.UNSPECIFIED.);
#23276=B_SPLINE_CURVE_WITH_KNOTS('',2,(#78695,#78696,#78697),
 .UNSPECIFIED.,.F.,.F.,(3,3),(0.,1.),.UNSPECIFIED.);
#23277=B_SPLINE_CURVE_WITH_KNOTS('',2,(#78700,#78701,#78702),
 .UNSPECIFIED.,.F.,.F.,(3,3),(0.,1.),.UNSPECIFIED.);
#23278=B_SPLINE_CURVE_WITH_KNOTS('',2,(#78710,#78711,#78712),
 .UNSPECIFIED.,.F.,.F.,(3,3),(0.,1.),.UNSPECIFIED.);
#23279=B_SPLINE_CURVE_WITH_KNOTS('',2,(#78715,#78716,#78717),
 .UNSPECIFIED.,.F.,.F.,(3,3),(0.,1.),.UNSPECIFIED.);
#23280=B_SPLINE_CURVE_WITH_KNOTS('',2,(#78725,#78726,#78727),
 .UNSPECIFIED.,.F.,.F.,(3,3),(0.,1.),.UNSPECIFIED.);
#23281=B_SPLINE_CURVE_WITH_KNOTS('',2,(#78730,#78731,#78732),
 .UNSPECIFIED.,.F.,.F.,(3,3),(0.,1.),.UNSPECIFIED.);
#23282=B_SPLINE_CURVE_WITH_KNOTS('',2,(#78740,#78741,#78742),
 .UNSPECIFIED.,.F.,.F.,(3,3),(0.,1.),.UNSPECIFIED.);
#23283=B_SPLINE_CURVE_WITH_KNOTS('',2,(#78745,#78746,#78747),
 .UNSPECIFIED.,.F.,.F.,(3,3),(0.,1.),.UNSPECIFIED.);
#23284=B_SPLINE_CURVE_WITH_KNOTS('',2,(#78755,#78756,#78757),
 .UNSPECIFIED.,.F.,.F.,(3,3),(0.,1.),.UNSPECIFIED.);
#23285=B_SPLINE_CURVE_WITH_KNOTS('',2,(#78760,#78761,#78762),
 .UNSPECIFIED.,.F.,.F.,(3,3),(0.,1.),.UNSPECIFIED.);
#23286=B_SPLINE_CURVE_WITH_KNOTS('',2,(#78770,#78771,#78772),
 .UNSPECIFIED.,.F.,.F.,(3,3),(0.,1.),.UNSPECIFIED.);
#23287=B_SPLINE_CURVE_WITH_KNOTS('',2,(#78775,#78776,#78777),
 .UNSPECIFIED.,.F.,.F.,(3,3),(0.,1.),.UNSPECIFIED.);
#23288=B_SPLINE_CURVE_WITH_KNOTS('',2,(#78785,#78786,#78787),
 .UNSPECIFIED.,.F.,.F.,(3,3),(0.,1.),.UNSPECIFIED.);
#23289=B_SPLINE_CURVE_WITH_KNOTS('',2,(#78790,#78791,#78792),
 .UNSPECIFIED.,.F.,.F.,(3,3),(0.,1.),.UNSPECIFIED.);
#23290=B_SPLINE_CURVE_WITH_KNOTS('',2,(#78800,#78801,#78802),
 .UNSPECIFIED.,.F.,.F.,(3,3),(0.,1.),.UNSPECIFIED.);
#23291=B_SPLINE_CURVE_WITH_KNOTS('',2,(#78805,#78806,#78807),
 .UNSPECIFIED.,.F.,.F.,(3,3),(0.,1.),.UNSPECIFIED.);
#23292=B_SPLINE_CURVE_WITH_KNOTS('',2,(#78820,#78821,#78822),
 .UNSPECIFIED.,.F.,.F.,(3,3),(0.,1.),.UNSPECIFIED.);
#23293=B_SPLINE_CURVE_WITH_KNOTS('',2,(#78823,#78824,#78825),
 .UNSPECIFIED.,.F.,.F.,(3,3),(0.,1.),.UNSPECIFIED.);
#23294=B_SPLINE_CURVE_WITH_KNOTS('',2,(#78837,#78838,#78839),
 .UNSPECIFIED.,.F.,.F.,(3,3),(0.,1.),.UNSPECIFIED.);
#23295=B_SPLINE_CURVE_WITH_KNOTS('',2,(#78843,#78844,#78845),
 .UNSPECIFIED.,.F.,.F.,(3,3),(0.,1.),.UNSPECIFIED.);
#23296=B_SPLINE_CURVE_WITH_KNOTS('',2,(#78854,#78855,#78856),
 .UNSPECIFIED.,.F.,.F.,(3,3),(0.,1.),.UNSPECIFIED.);
#23297=B_SPLINE_CURVE_WITH_KNOTS('',2,(#78859,#78860,#78861),
 .UNSPECIFIED.,.F.,.F.,(3,3),(0.,1.),.UNSPECIFIED.);
#23298=B_SPLINE_CURVE_WITH_KNOTS('',2,(#78869,#78870,#78871),
 .UNSPECIFIED.,.F.,.F.,(3,3),(0.,1.),.UNSPECIFIED.);
#23299=B_SPLINE_CURVE_WITH_KNOTS('',2,(#78874,#78875,#78876),
 .UNSPECIFIED.,.F.,.F.,(3,3),(0.,1.),.UNSPECIFIED.);
#23300=B_SPLINE_CURVE_WITH_KNOTS('',2,(#78884,#78885,#78886),
 .UNSPECIFIED.,.F.,.F.,(3,3),(0.,1.),.UNSPECIFIED.);
#23301=B_SPLINE_CURVE_WITH_KNOTS('',2,(#78889,#78890,#78891),
 .UNSPECIFIED.,.F.,.F.,(3,3),(0.,1.),.UNSPECIFIED.);
#23302=B_SPLINE_CURVE_WITH_KNOTS('',2,(#78899,#78900,#78901),
 .UNSPECIFIED.,.F.,.F.,(3,3),(0.,1.),.UNSPECIFIED.);
#23303=B_SPLINE_CURVE_WITH_KNOTS('',2,(#78904,#78905,#78906),
 .UNSPECIFIED.,.F.,.F.,(3,3),(0.,1.),.UNSPECIFIED.);
#23304=B_SPLINE_CURVE_WITH_KNOTS('',2,(#78914,#78915,#78916),
 .UNSPECIFIED.,.F.,.F.,(3,3),(0.,1.),.UNSPECIFIED.);
#23305=B_SPLINE_CURVE_WITH_KNOTS('',2,(#78919,#78920,#78921),
 .UNSPECIFIED.,.F.,.F.,(3,3),(0.,1.),.UNSPECIFIED.);
#23306=B_SPLINE_CURVE_WITH_KNOTS('',2,(#78929,#78930,#78931),
 .UNSPECIFIED.,.F.,.F.,(3,3),(0.,1.),.UNSPECIFIED.);
#23307=B_SPLINE_CURVE_WITH_KNOTS('',2,(#78934,#78935,#78936),
 .UNSPECIFIED.,.F.,.F.,(3,3),(0.,1.),.UNSPECIFIED.);
#23308=B_SPLINE_CURVE_WITH_KNOTS('',2,(#78943,#78944,#78945),
 .UNSPECIFIED.,.F.,.F.,(3,3),(0.,1.),.UNSPECIFIED.);
#23309=B_SPLINE_CURVE_WITH_KNOTS('',2,(#78946,#78947,#78948),
 .UNSPECIFIED.,.F.,.F.,(3,3),(0.,1.),.UNSPECIFIED.);
#23310=B_SPLINE_CURVE_WITH_KNOTS('',2,(#78957,#78958,#78959),
 .UNSPECIFIED.,.F.,.F.,(3,3),(0.,1.),.UNSPECIFIED.);
#23311=B_SPLINE_CURVE_WITH_KNOTS('',2,(#78963,#78964,#78965),
 .UNSPECIFIED.,.F.,.F.,(3,3),(0.,1.),.UNSPECIFIED.);
#23312=B_SPLINE_CURVE_WITH_KNOTS('',2,(#78974,#78975,#78976),
 .UNSPECIFIED.,.F.,.F.,(3,3),(0.,1.),.UNSPECIFIED.);
#23313=B_SPLINE_CURVE_WITH_KNOTS('',2,(#78979,#78980,#78981),
 .UNSPECIFIED.,.F.,.F.,(3,3),(0.,1.),.UNSPECIFIED.);
#23314=B_SPLINE_CURVE_WITH_KNOTS('',2,(#78989,#78990,#78991),
 .UNSPECIFIED.,.F.,.F.,(3,3),(0.,1.),.UNSPECIFIED.);
#23315=B_SPLINE_CURVE_WITH_KNOTS('',2,(#78994,#78995,#78996),
 .UNSPECIFIED.,.F.,.F.,(3,3),(0.,1.),.UNSPECIFIED.);
#23316=B_SPLINE_CURVE_WITH_KNOTS('',2,(#79004,#79005,#79006),
 .UNSPECIFIED.,.F.,.F.,(3,3),(0.,1.),.UNSPECIFIED.);
#23317=B_SPLINE_CURVE_WITH_KNOTS('',2,(#79009,#79010,#79011),
 .UNSPECIFIED.,.F.,.F.,(3,3),(0.,1.),.UNSPECIFIED.);
#23318=B_SPLINE_CURVE_WITH_KNOTS('',2,(#79019,#79020,#79021),
 .UNSPECIFIED.,.F.,.F.,(3,3),(0.,1.),.UNSPECIFIED.);
#23319=B_SPLINE_CURVE_WITH_KNOTS('',2,(#79024,#79025,#79026),
 .UNSPECIFIED.,.F.,.F.,(3,3),(0.,1.),.UNSPECIFIED.);
#23320=B_SPLINE_CURVE_WITH_KNOTS('',2,(#79034,#79035,#79036),
 .UNSPECIFIED.,.F.,.F.,(3,3),(0.,1.),.UNSPECIFIED.);
#23321=B_SPLINE_CURVE_WITH_KNOTS('',2,(#79039,#79040,#79041),
 .UNSPECIFIED.,.F.,.F.,(3,3),(0.,1.),.UNSPECIFIED.);
#23322=B_SPLINE_CURVE_WITH_KNOTS('',2,(#79049,#79050,#79051),
 .UNSPECIFIED.,.F.,.F.,(3,3),(0.,1.),.UNSPECIFIED.);
#23323=B_SPLINE_CURVE_WITH_KNOTS('',2,(#79054,#79055,#79056),
 .UNSPECIFIED.,.F.,.F.,(3,3),(0.,1.),.UNSPECIFIED.);
#23324=B_SPLINE_CURVE_WITH_KNOTS('',2,(#79064,#79065,#79066),
 .UNSPECIFIED.,.F.,.F.,(3,3),(0.,1.),.UNSPECIFIED.);
#23325=B_SPLINE_CURVE_WITH_KNOTS('',2,(#79069,#79070,#79071),
 .UNSPECIFIED.,.F.,.F.,(3,3),(0.,1.),.UNSPECIFIED.);
#23326=B_SPLINE_CURVE_WITH_KNOTS('',2,(#79079,#79080,#79081),
 .UNSPECIFIED.,.F.,.F.,(3,3),(0.,1.),.UNSPECIFIED.);
#23327=B_SPLINE_CURVE_WITH_KNOTS('',2,(#79084,#79085,#79086),
 .UNSPECIFIED.,.F.,.F.,(3,3),(0.,1.),.UNSPECIFIED.);
#23328=B_SPLINE_CURVE_WITH_KNOTS('',2,(#79094,#79095,#79096),
 .UNSPECIFIED.,.F.,.F.,(3,3),(0.,1.),.UNSPECIFIED.);
#23329=B_SPLINE_CURVE_WITH_KNOTS('',2,(#79099,#79100,#79101),
 .UNSPECIFIED.,.F.,.F.,(3,3),(0.,1.),.UNSPECIFIED.);
#23330=B_SPLINE_CURVE_WITH_KNOTS('',2,(#79109,#79110,#79111),
 .UNSPECIFIED.,.F.,.F.,(3,3),(0.,1.),.UNSPECIFIED.);
#23331=B_SPLINE_CURVE_WITH_KNOTS('',2,(#79114,#79115,#79116),
 .UNSPECIFIED.,.F.,.F.,(3,3),(0.,1.),.UNSPECIFIED.);
#23332=B_SPLINE_CURVE_WITH_KNOTS('',2,(#79123,#79124,#79125),
 .UNSPECIFIED.,.F.,.F.,(3,3),(0.,1.),.UNSPECIFIED.);
#23333=B_SPLINE_CURVE_WITH_KNOTS('',2,(#79126,#79127,#79128),
 .UNSPECIFIED.,.F.,.F.,(3,3),(0.,1.),.UNSPECIFIED.);
#23334=B_SPLINE_CURVE_WITH_KNOTS('',2,(#79138,#79139,#79140),
 .UNSPECIFIED.,.F.,.F.,(3,3),(0.,1.),.UNSPECIFIED.);
#23335=B_SPLINE_CURVE_WITH_KNOTS('',2,(#79144,#79145,#79146),
 .UNSPECIFIED.,.F.,.F.,(3,3),(0.,1.),.UNSPECIFIED.);
#23336=B_SPLINE_CURVE_WITH_KNOTS('',2,(#79155,#79156,#79157),
 .UNSPECIFIED.,.F.,.F.,(3,3),(0.,1.),.UNSPECIFIED.);
#23337=B_SPLINE_CURVE_WITH_KNOTS('',2,(#79160,#79161,#79162),
 .UNSPECIFIED.,.F.,.F.,(3,3),(0.,1.),.UNSPECIFIED.);
#23338=B_SPLINE_CURVE_WITH_KNOTS('',2,(#79170,#79171,#79172),
 .UNSPECIFIED.,.F.,.F.,(3,3),(0.,1.),.UNSPECIFIED.);
#23339=B_SPLINE_CURVE_WITH_KNOTS('',2,(#79175,#79176,#79177),
 .UNSPECIFIED.,.F.,.F.,(3,3),(0.,1.),.UNSPECIFIED.);
#23340=B_SPLINE_CURVE_WITH_KNOTS('',2,(#79185,#79186,#79187),
 .UNSPECIFIED.,.F.,.F.,(3,3),(0.,1.),.UNSPECIFIED.);
#23341=B_SPLINE_CURVE_WITH_KNOTS('',2,(#79190,#79191,#79192),
 .UNSPECIFIED.,.F.,.F.,(3,3),(0.,1.),.UNSPECIFIED.);
#23342=B_SPLINE_CURVE_WITH_KNOTS('',2,(#79200,#79201,#79202),
 .UNSPECIFIED.,.F.,.F.,(3,3),(0.,1.),.UNSPECIFIED.);
#23343=B_SPLINE_CURVE_WITH_KNOTS('',2,(#79205,#79206,#79207),
 .UNSPECIFIED.,.F.,.F.,(3,3),(0.,1.),.UNSPECIFIED.);
#23344=B_SPLINE_CURVE_WITH_KNOTS('',2,(#79215,#79216,#79217),
 .UNSPECIFIED.,.F.,.F.,(3,3),(0.,1.),.UNSPECIFIED.);
#23345=B_SPLINE_CURVE_WITH_KNOTS('',2,(#79220,#79221,#79222),
 .UNSPECIFIED.,.F.,.F.,(3,3),(0.,1.),.UNSPECIFIED.);
#23346=B_SPLINE_CURVE_WITH_KNOTS('',2,(#79266,#79267,#79268),
 .UNSPECIFIED.,.F.,.F.,(3,3),(0.,1.),.UNSPECIFIED.);
#23347=B_SPLINE_CURVE_WITH_KNOTS('',2,(#79271,#79272,#79273),
 .UNSPECIFIED.,.F.,.F.,(3,3),(0.,1.),.UNSPECIFIED.);
#23348=B_SPLINE_CURVE_WITH_KNOTS('',2,(#79281,#79282,#79283),
 .UNSPECIFIED.,.F.,.F.,(3,3),(0.,1.),.UNSPECIFIED.);
#23349=B_SPLINE_CURVE_WITH_KNOTS('',2,(#79286,#79287,#79288),
 .UNSPECIFIED.,.F.,.F.,(3,3),(0.,1.),.UNSPECIFIED.);
#23350=B_SPLINE_CURVE_WITH_KNOTS('',2,(#79296,#79297,#79298),
 .UNSPECIFIED.,.F.,.F.,(3,3),(0.,1.),.UNSPECIFIED.);
#23351=B_SPLINE_CURVE_WITH_KNOTS('',2,(#79301,#79302,#79303),
 .UNSPECIFIED.,.F.,.F.,(3,3),(0.,1.),.UNSPECIFIED.);
#23352=B_SPLINE_CURVE_WITH_KNOTS('',2,(#79311,#79312,#79313),
 .UNSPECIFIED.,.F.,.F.,(3,3),(0.,1.),.UNSPECIFIED.);
#23353=B_SPLINE_CURVE_WITH_KNOTS('',2,(#79316,#79317,#79318),
 .UNSPECIFIED.,.F.,.F.,(3,3),(0.,1.),.UNSPECIFIED.);
#23354=B_SPLINE_CURVE_WITH_KNOTS('',2,(#79326,#79327,#79328),
 .UNSPECIFIED.,.F.,.F.,(3,3),(0.,1.),.UNSPECIFIED.);
#23355=B_SPLINE_CURVE_WITH_KNOTS('',2,(#79331,#79332,#79333),
 .UNSPECIFIED.,.F.,.F.,(3,3),(0.,1.),.UNSPECIFIED.);
#23356=B_SPLINE_CURVE_WITH_KNOTS('',2,(#79341,#79342,#79343),
 .UNSPECIFIED.,.F.,.F.,(3,3),(0.,1.),.UNSPECIFIED.);
#23357=B_SPLINE_CURVE_WITH_KNOTS('',2,(#79346,#79347,#79348),
 .UNSPECIFIED.,.F.,.F.,(3,3),(0.,1.),.UNSPECIFIED.);
#23358=B_SPLINE_CURVE_WITH_KNOTS('',2,(#79356,#79357,#79358),
 .UNSPECIFIED.,.F.,.F.,(3,3),(0.,1.),.UNSPECIFIED.);
#23359=B_SPLINE_CURVE_WITH_KNOTS('',2,(#79361,#79362,#79363),
 .UNSPECIFIED.,.F.,.F.,(3,3),(0.,1.),.UNSPECIFIED.);
#23360=B_SPLINE_CURVE_WITH_KNOTS('',2,(#79371,#79372,#79373),
 .UNSPECIFIED.,.F.,.F.,(3,3),(0.,1.),.UNSPECIFIED.);
#23361=B_SPLINE_CURVE_WITH_KNOTS('',2,(#79376,#79377,#79378),
 .UNSPECIFIED.,.F.,.F.,(3,3),(0.,1.),.UNSPECIFIED.);
#23362=B_SPLINE_CURVE_WITH_KNOTS('',2,(#79391,#79392,#79393),
 .UNSPECIFIED.,.F.,.F.,(3,3),(0.,1.),.UNSPECIFIED.);
#23363=B_SPLINE_CURVE_WITH_KNOTS('',2,(#79394,#79395,#79396),
 .UNSPECIFIED.,.F.,.F.,(3,3),(0.,1.),.UNSPECIFIED.);
#23364=B_SPLINE_CURVE_WITH_KNOTS('',2,(#79407,#79408,#79409),
 .UNSPECIFIED.,.F.,.F.,(3,3),(0.,1.),.UNSPECIFIED.);
#23365=B_SPLINE_CURVE_WITH_KNOTS('',2,(#79413,#79414,#79415),
 .UNSPECIFIED.,.F.,.F.,(3,3),(0.,1.),.UNSPECIFIED.);
#23366=B_SPLINE_CURVE_WITH_KNOTS('',2,(#79424,#79425,#79426),
 .UNSPECIFIED.,.F.,.F.,(3,3),(0.,1.),.UNSPECIFIED.);
#23367=B_SPLINE_CURVE_WITH_KNOTS('',2,(#79429,#79430,#79431),
 .UNSPECIFIED.,.F.,.F.,(3,3),(0.,1.),.UNSPECIFIED.);
#23368=B_SPLINE_CURVE_WITH_KNOTS('',2,(#79439,#79440,#79441),
 .UNSPECIFIED.,.F.,.F.,(3,3),(0.,1.),.UNSPECIFIED.);
#23369=B_SPLINE_CURVE_WITH_KNOTS('',2,(#79444,#79445,#79446),
 .UNSPECIFIED.,.F.,.F.,(3,3),(0.,1.),.UNSPECIFIED.);
#23370=B_SPLINE_CURVE_WITH_KNOTS('',2,(#79454,#79455,#79456),
 .UNSPECIFIED.,.F.,.F.,(3,3),(0.,1.),.UNSPECIFIED.);
#23371=B_SPLINE_CURVE_WITH_KNOTS('',2,(#79459,#79460,#79461),
 .UNSPECIFIED.,.F.,.F.,(3,3),(0.,1.),.UNSPECIFIED.);
#23372=B_SPLINE_CURVE_WITH_KNOTS('',2,(#79469,#79470,#79471),
 .UNSPECIFIED.,.F.,.F.,(3,3),(0.,1.),.UNSPECIFIED.);
#23373=B_SPLINE_CURVE_WITH_KNOTS('',2,(#79474,#79475,#79476),
 .UNSPECIFIED.,.F.,.F.,(3,3),(0.,1.),.UNSPECIFIED.);
#23374=B_SPLINE_CURVE_WITH_KNOTS('',2,(#79484,#79485,#79486),
 .UNSPECIFIED.,.F.,.F.,(3,3),(0.,1.),.UNSPECIFIED.);
#23375=B_SPLINE_CURVE_WITH_KNOTS('',2,(#79489,#79490,#79491),
 .UNSPECIFIED.,.F.,.F.,(3,3),(0.,1.),.UNSPECIFIED.);
#23376=B_SPLINE_CURVE_WITH_KNOTS('',2,(#79499,#79500,#79501),
 .UNSPECIFIED.,.F.,.F.,(3,3),(0.,1.),.UNSPECIFIED.);
#23377=B_SPLINE_CURVE_WITH_KNOTS('',2,(#79504,#79505,#79506),
 .UNSPECIFIED.,.F.,.F.,(3,3),(0.,1.),.UNSPECIFIED.);
#23378=B_SPLINE_CURVE_WITH_KNOTS('',2,(#79513,#79514,#79515),
 .UNSPECIFIED.,.F.,.F.,(3,3),(0.,1.),.UNSPECIFIED.);
#23379=B_SPLINE_CURVE_WITH_KNOTS('',2,(#79516,#79517,#79518),
 .UNSPECIFIED.,.F.,.F.,(3,3),(0.,1.),.UNSPECIFIED.);
#23380=B_SPLINE_CURVE_WITH_KNOTS('',2,(#79527,#79528,#79529),
 .UNSPECIFIED.,.F.,.F.,(3,3),(0.,1.),.UNSPECIFIED.);
#23381=B_SPLINE_CURVE_WITH_KNOTS('',2,(#79533,#79534,#79535),
 .UNSPECIFIED.,.F.,.F.,(3,3),(0.,1.),.UNSPECIFIED.);
#23382=B_SPLINE_CURVE_WITH_KNOTS('',2,(#79544,#79545,#79546),
 .UNSPECIFIED.,.F.,.F.,(3,3),(0.,1.),.UNSPECIFIED.);
#23383=B_SPLINE_CURVE_WITH_KNOTS('',2,(#79549,#79550,#79551),
 .UNSPECIFIED.,.F.,.F.,(3,3),(0.,1.),.UNSPECIFIED.);
#23384=B_SPLINE_CURVE_WITH_KNOTS('',2,(#79559,#79560,#79561),
 .UNSPECIFIED.,.F.,.F.,(3,3),(0.,1.),.UNSPECIFIED.);
#23385=B_SPLINE_CURVE_WITH_KNOTS('',2,(#79564,#79565,#79566),
 .UNSPECIFIED.,.F.,.F.,(3,3),(0.,1.),.UNSPECIFIED.);
#23386=B_SPLINE_CURVE_WITH_KNOTS('',2,(#79574,#79575,#79576),
 .UNSPECIFIED.,.F.,.F.,(3,3),(0.,1.),.UNSPECIFIED.);
#23387=B_SPLINE_CURVE_WITH_KNOTS('',2,(#79579,#79580,#79581),
 .UNSPECIFIED.,.F.,.F.,(3,3),(0.,1.),.UNSPECIFIED.);
#23388=B_SPLINE_CURVE_WITH_KNOTS('',2,(#79589,#79590,#79591),
 .UNSPECIFIED.,.F.,.F.,(3,3),(0.,1.),.UNSPECIFIED.);
#23389=B_SPLINE_CURVE_WITH_KNOTS('',2,(#79594,#79595,#79596),
 .UNSPECIFIED.,.F.,.F.,(3,3),(0.,1.),.UNSPECIFIED.);
#23390=B_SPLINE_CURVE_WITH_KNOTS('',2,(#79604,#79605,#79606),
 .UNSPECIFIED.,.F.,.F.,(3,3),(0.,1.),.UNSPECIFIED.);
#23391=B_SPLINE_CURVE_WITH_KNOTS('',2,(#79609,#79610,#79611),
 .UNSPECIFIED.,.F.,.F.,(3,3),(0.,1.),.UNSPECIFIED.);
#23392=B_SPLINE_CURVE_WITH_KNOTS('',2,(#79619,#79620,#79621),
 .UNSPECIFIED.,.F.,.F.,(3,3),(0.,1.),.UNSPECIFIED.);
#23393=B_SPLINE_CURVE_WITH_KNOTS('',2,(#79624,#79625,#79626),
 .UNSPECIFIED.,.F.,.F.,(3,3),(0.,1.),.UNSPECIFIED.);
#23394=B_SPLINE_CURVE_WITH_KNOTS('',2,(#79634,#79635,#79636),
 .UNSPECIFIED.,.F.,.F.,(3,3),(0.,1.),.UNSPECIFIED.);
#23395=B_SPLINE_CURVE_WITH_KNOTS('',2,(#79639,#79640,#79641),
 .UNSPECIFIED.,.F.,.F.,(3,3),(0.,1.),.UNSPECIFIED.);
#23396=B_SPLINE_CURVE_WITH_KNOTS('',2,(#79649,#79650,#79651),
 .UNSPECIFIED.,.F.,.F.,(3,3),(0.,1.),.UNSPECIFIED.);
#23397=B_SPLINE_CURVE_WITH_KNOTS('',2,(#79654,#79655,#79656),
 .UNSPECIFIED.,.F.,.F.,(3,3),(0.,1.),.UNSPECIFIED.);
#23398=B_SPLINE_CURVE_WITH_KNOTS('',2,(#79664,#79665,#79666),
 .UNSPECIFIED.,.F.,.F.,(3,3),(0.,1.),.UNSPECIFIED.);
#23399=B_SPLINE_CURVE_WITH_KNOTS('',2,(#79669,#79670,#79671),
 .UNSPECIFIED.,.F.,.F.,(3,3),(0.,1.),.UNSPECIFIED.);
#23400=B_SPLINE_CURVE_WITH_KNOTS('',2,(#79679,#79680,#79681),
 .UNSPECIFIED.,.F.,.F.,(3,3),(0.,1.),.UNSPECIFIED.);
#23401=B_SPLINE_CURVE_WITH_KNOTS('',2,(#79684,#79685,#79686),
 .UNSPECIFIED.,.F.,.F.,(3,3),(0.,1.),.UNSPECIFIED.);
#23402=B_SPLINE_CURVE_WITH_KNOTS('',2,(#79693,#79694,#79695),
 .UNSPECIFIED.,.F.,.F.,(3,3),(0.,1.),.UNSPECIFIED.);
#23403=B_SPLINE_CURVE_WITH_KNOTS('',2,(#79696,#79697,#79698),
 .UNSPECIFIED.,.F.,.F.,(3,3),(0.,1.),.UNSPECIFIED.);
#23404=B_SPLINE_CURVE_WITH_KNOTS('',2,(#79795,#79796,#79797),
 .UNSPECIFIED.,.F.,.F.,(3,3),(0.,1.),.UNSPECIFIED.);
#23405=B_SPLINE_CURVE_WITH_KNOTS('',2,(#79801,#79802,#79803),
 .UNSPECIFIED.,.F.,.F.,(3,3),(0.,1.),.UNSPECIFIED.);
#23406=B_SPLINE_CURVE_WITH_KNOTS('',2,(#79812,#79813,#79814),
 .UNSPECIFIED.,.F.,.F.,(3,3),(0.,1.),.UNSPECIFIED.);
#23407=B_SPLINE_CURVE_WITH_KNOTS('',2,(#79817,#79818,#79819),
 .UNSPECIFIED.,.F.,.F.,(3,3),(0.,1.),.UNSPECIFIED.);
#23408=B_SPLINE_CURVE_WITH_KNOTS('',2,(#79827,#79828,#79829),
 .UNSPECIFIED.,.F.,.F.,(3,3),(0.,1.),.UNSPECIFIED.);
#23409=B_SPLINE_CURVE_WITH_KNOTS('',2,(#79832,#79833,#79834),
 .UNSPECIFIED.,.F.,.F.,(3,3),(0.,1.),.UNSPECIFIED.);
#23410=B_SPLINE_CURVE_WITH_KNOTS('',2,(#79842,#79843,#79844),
 .UNSPECIFIED.,.F.,.F.,(3,3),(0.,1.),.UNSPECIFIED.);
#23411=B_SPLINE_CURVE_WITH_KNOTS('',2,(#79847,#79848,#79849),
 .UNSPECIFIED.,.F.,.F.,(3,3),(0.,1.),.UNSPECIFIED.);
#23412=B_SPLINE_CURVE_WITH_KNOTS('',2,(#79857,#79858,#79859),
 .UNSPECIFIED.,.F.,.F.,(3,3),(0.,1.),.UNSPECIFIED.);
#23413=B_SPLINE_CURVE_WITH_KNOTS('',2,(#79862,#79863,#79864),
 .UNSPECIFIED.,.F.,.F.,(3,3),(0.,1.),.UNSPECIFIED.);
#23414=B_SPLINE_CURVE_WITH_KNOTS('',2,(#79872,#79873,#79874),
 .UNSPECIFIED.,.F.,.F.,(3,3),(0.,1.),.UNSPECIFIED.);
#23415=B_SPLINE_CURVE_WITH_KNOTS('',2,(#79877,#79878,#79879),
 .UNSPECIFIED.,.F.,.F.,(3,3),(0.,1.),.UNSPECIFIED.);
#23416=B_SPLINE_CURVE_WITH_KNOTS('',2,(#79887,#79888,#79889),
 .UNSPECIFIED.,.F.,.F.,(3,3),(0.,1.),.UNSPECIFIED.);
#23417=B_SPLINE_CURVE_WITH_KNOTS('',2,(#79892,#79893,#79894),
 .UNSPECIFIED.,.F.,.F.,(3,3),(0.,1.),.UNSPECIFIED.);
#23418=B_SPLINE_CURVE_WITH_KNOTS('',2,(#79901,#79902,#79903),
 .UNSPECIFIED.,.F.,.F.,(3,3),(0.,1.),.UNSPECIFIED.);
#23419=B_SPLINE_CURVE_WITH_KNOTS('',2,(#79904,#79905,#79906),
 .UNSPECIFIED.,.F.,.F.,(3,3),(0.,1.),.UNSPECIFIED.);
#23420=B_SPLINE_CURVE_WITH_KNOTS('',2,(#79915,#79916,#79917),
 .UNSPECIFIED.,.F.,.F.,(3,3),(0.,1.),.UNSPECIFIED.);
#23421=B_SPLINE_CURVE_WITH_KNOTS('',2,(#79921,#79922,#79923),
 .UNSPECIFIED.,.F.,.F.,(3,3),(0.,1.),.UNSPECIFIED.);
#23422=B_SPLINE_CURVE_WITH_KNOTS('',2,(#79932,#79933,#79934),
 .UNSPECIFIED.,.F.,.F.,(3,3),(0.,1.),.UNSPECIFIED.);
#23423=B_SPLINE_CURVE_WITH_KNOTS('',2,(#79937,#79938,#79939),
 .UNSPECIFIED.,.F.,.F.,(3,3),(0.,1.),.UNSPECIFIED.);
#23424=B_SPLINE_CURVE_WITH_KNOTS('',2,(#79947,#79948,#79949),
 .UNSPECIFIED.,.F.,.F.,(3,3),(0.,1.),.UNSPECIFIED.);
#23425=B_SPLINE_CURVE_WITH_KNOTS('',2,(#79952,#79953,#79954),
 .UNSPECIFIED.,.F.,.F.,(3,3),(0.,1.),.UNSPECIFIED.);
#23426=B_SPLINE_CURVE_WITH_KNOTS('',2,(#79962,#79963,#79964),
 .UNSPECIFIED.,.F.,.F.,(3,3),(0.,1.),.UNSPECIFIED.);
#23427=B_SPLINE_CURVE_WITH_KNOTS('',2,(#79967,#79968,#79969),
 .UNSPECIFIED.,.F.,.F.,(3,3),(0.,1.),.UNSPECIFIED.);
#23428=B_SPLINE_CURVE_WITH_KNOTS('',2,(#79977,#79978,#79979),
 .UNSPECIFIED.,.F.,.F.,(3,3),(0.,1.),.UNSPECIFIED.);
#23429=B_SPLINE_CURVE_WITH_KNOTS('',2,(#79982,#79983,#79984),
 .UNSPECIFIED.,.F.,.F.,(3,3),(0.,1.),.UNSPECIFIED.);
#23430=B_SPLINE_CURVE_WITH_KNOTS('',2,(#79992,#79993,#79994),
 .UNSPECIFIED.,.F.,.F.,(3,3),(0.,1.),.UNSPECIFIED.);
#23431=B_SPLINE_CURVE_WITH_KNOTS('',2,(#79997,#79998,#79999),
 .UNSPECIFIED.,.F.,.F.,(3,3),(0.,1.),.UNSPECIFIED.);
#23432=B_SPLINE_CURVE_WITH_KNOTS('',2,(#80007,#80008,#80009),
 .UNSPECIFIED.,.F.,.F.,(3,3),(0.,1.),.UNSPECIFIED.);
#23433=B_SPLINE_CURVE_WITH_KNOTS('',2,(#80012,#80013,#80014),
 .UNSPECIFIED.,.F.,.F.,(3,3),(0.,1.),.UNSPECIFIED.);
#23434=B_SPLINE_CURVE_WITH_KNOTS('',2,(#80022,#80023,#80024),
 .UNSPECIFIED.,.F.,.F.,(3,3),(0.,1.),.UNSPECIFIED.);
#23435=B_SPLINE_CURVE_WITH_KNOTS('',2,(#80027,#80028,#80029),
 .UNSPECIFIED.,.F.,.F.,(3,3),(0.,1.),.UNSPECIFIED.);
#23436=B_SPLINE_CURVE_WITH_KNOTS('',2,(#80037,#80038,#80039),
 .UNSPECIFIED.,.F.,.F.,(3,3),(0.,1.),.UNSPECIFIED.);
#23437=B_SPLINE_CURVE_WITH_KNOTS('',2,(#80042,#80043,#80044),
 .UNSPECIFIED.,.F.,.F.,(3,3),(0.,1.),.UNSPECIFIED.);
#23438=B_SPLINE_CURVE_WITH_KNOTS('',2,(#80052,#80053,#80054),
 .UNSPECIFIED.,.F.,.F.,(3,3),(0.,1.),.UNSPECIFIED.);
#23439=B_SPLINE_CURVE_WITH_KNOTS('',2,(#80057,#80058,#80059),
 .UNSPECIFIED.,.F.,.F.,(3,3),(0.,1.),.UNSPECIFIED.);
#23440=B_SPLINE_CURVE_WITH_KNOTS('',2,(#80067,#80068,#80069),
 .UNSPECIFIED.,.F.,.F.,(3,3),(0.,1.),.UNSPECIFIED.);
#23441=B_SPLINE_CURVE_WITH_KNOTS('',2,(#80072,#80073,#80074),
 .UNSPECIFIED.,.F.,.F.,(3,3),(0.,1.),.UNSPECIFIED.);
#23442=B_SPLINE_CURVE_WITH_KNOTS('',2,(#80081,#80082,#80083),
 .UNSPECIFIED.,.F.,.F.,(3,3),(0.,1.),.UNSPECIFIED.);
#23443=B_SPLINE_CURVE_WITH_KNOTS('',2,(#80084,#80085,#80086),
 .UNSPECIFIED.,.F.,.F.,(3,3),(0.,1.),.UNSPECIFIED.);
#23444=B_SPLINE_CURVE_WITH_KNOTS('',2,(#80096,#80097,#80098),
 .UNSPECIFIED.,.F.,.F.,(3,3),(0.,1.),.UNSPECIFIED.);
#23445=B_SPLINE_CURVE_WITH_KNOTS('',2,(#80102,#80103,#80104),
 .UNSPECIFIED.,.F.,.F.,(3,3),(0.,1.),.UNSPECIFIED.);
#23446=B_SPLINE_CURVE_WITH_KNOTS('',2,(#80113,#80114,#80115),
 .UNSPECIFIED.,.F.,.F.,(3,3),(0.,1.),.UNSPECIFIED.);
#23447=B_SPLINE_CURVE_WITH_KNOTS('',2,(#80118,#80119,#80120),
 .UNSPECIFIED.,.F.,.F.,(3,3),(0.,1.),.UNSPECIFIED.);
#23448=B_SPLINE_CURVE_WITH_KNOTS('',2,(#80128,#80129,#80130),
 .UNSPECIFIED.,.F.,.F.,(3,3),(0.,1.),.UNSPECIFIED.);
#23449=B_SPLINE_CURVE_WITH_KNOTS('',2,(#80133,#80134,#80135),
 .UNSPECIFIED.,.F.,.F.,(3,3),(0.,1.),.UNSPECIFIED.);
#23450=B_SPLINE_CURVE_WITH_KNOTS('',2,(#80143,#80144,#80145),
 .UNSPECIFIED.,.F.,.F.,(3,3),(0.,1.),.UNSPECIFIED.);
#23451=B_SPLINE_CURVE_WITH_KNOTS('',2,(#80148,#80149,#80150),
 .UNSPECIFIED.,.F.,.F.,(3,3),(0.,1.),.UNSPECIFIED.);
#23452=B_SPLINE_CURVE_WITH_KNOTS('',2,(#80158,#80159,#80160),
 .UNSPECIFIED.,.F.,.F.,(3,3),(0.,1.),.UNSPECIFIED.);
#23453=B_SPLINE_CURVE_WITH_KNOTS('',2,(#80163,#80164,#80165),
 .UNSPECIFIED.,.F.,.F.,(3,3),(0.,1.),.UNSPECIFIED.);
#23454=B_SPLINE_CURVE_WITH_KNOTS('',2,(#80173,#80174,#80175),
 .UNSPECIFIED.,.F.,.F.,(3,3),(0.,1.),.UNSPECIFIED.);
#23455=B_SPLINE_CURVE_WITH_KNOTS('',2,(#80178,#80179,#80180),
 .UNSPECIFIED.,.F.,.F.,(3,3),(0.,1.),.UNSPECIFIED.);
#23456=B_SPLINE_CURVE_WITH_KNOTS('',2,(#80188,#80189,#80190),
 .UNSPECIFIED.,.F.,.F.,(3,3),(0.,1.),.UNSPECIFIED.);
#23457=B_SPLINE_CURVE_WITH_KNOTS('',2,(#80193,#80194,#80195),
 .UNSPECIFIED.,.F.,.F.,(3,3),(0.,1.),.UNSPECIFIED.);
#23458=B_SPLINE_CURVE_WITH_KNOTS('',2,(#80203,#80204,#80205),
 .UNSPECIFIED.,.F.,.F.,(3,3),(0.,1.),.UNSPECIFIED.);
#23459=B_SPLINE_CURVE_WITH_KNOTS('',2,(#80208,#80209,#80210),
 .UNSPECIFIED.,.F.,.F.,(3,3),(0.,1.),.UNSPECIFIED.);
#23460=B_SPLINE_CURVE_WITH_KNOTS('',2,(#80218,#80219,#80220),
 .UNSPECIFIED.,.F.,.F.,(3,3),(0.,1.),.UNSPECIFIED.);
#23461=B_SPLINE_CURVE_WITH_KNOTS('',2,(#80223,#80224,#80225),
 .UNSPECIFIED.,.F.,.F.,(3,3),(0.,1.),.UNSPECIFIED.);
#23462=B_SPLINE_CURVE_WITH_KNOTS('',2,(#80233,#80234,#80235),
 .UNSPECIFIED.,.F.,.F.,(3,3),(0.,1.),.UNSPECIFIED.);
#23463=B_SPLINE_CURVE_WITH_KNOTS('',2,(#80238,#80239,#80240),
 .UNSPECIFIED.,.F.,.F.,(3,3),(0.,1.),.UNSPECIFIED.);
#23464=B_SPLINE_CURVE_WITH_KNOTS('',2,(#80248,#80249,#80250),
 .UNSPECIFIED.,.F.,.F.,(3,3),(0.,1.),.UNSPECIFIED.);
#23465=B_SPLINE_CURVE_WITH_KNOTS('',2,(#80253,#80254,#80255),
 .UNSPECIFIED.,.F.,.F.,(3,3),(0.,1.),.UNSPECIFIED.);
#23466=B_SPLINE_CURVE_WITH_KNOTS('',2,(#80263,#80264,#80265),
 .UNSPECIFIED.,.F.,.F.,(3,3),(0.,1.),.UNSPECIFIED.);
#23467=B_SPLINE_CURVE_WITH_KNOTS('',2,(#80268,#80269,#80270),
 .UNSPECIFIED.,.F.,.F.,(3,3),(0.,1.),.UNSPECIFIED.);
#23468=B_SPLINE_CURVE_WITH_KNOTS('',2,(#80284,#80285,#80286),
 .UNSPECIFIED.,.F.,.F.,(3,3),(0.,1.),.UNSPECIFIED.);
#23469=B_SPLINE_CURVE_WITH_KNOTS('',2,(#80289,#80290,#80291),
 .UNSPECIFIED.,.F.,.F.,(3,3),(0.,1.),.UNSPECIFIED.);
#23470=B_SPLINE_CURVE_WITH_KNOTS('',2,(#80299,#80300,#80301),
 .UNSPECIFIED.,.F.,.F.,(3,3),(0.,1.),.UNSPECIFIED.);
#23471=B_SPLINE_CURVE_WITH_KNOTS('',2,(#80304,#80305,#80306),
 .UNSPECIFIED.,.F.,.F.,(3,3),(0.,1.),.UNSPECIFIED.);
#23472=B_SPLINE_CURVE_WITH_KNOTS('',2,(#80314,#80315,#80316),
 .UNSPECIFIED.,.F.,.F.,(3,3),(0.,1.),.UNSPECIFIED.);
#23473=B_SPLINE_CURVE_WITH_KNOTS('',2,(#80319,#80320,#80321),
 .UNSPECIFIED.,.F.,.F.,(3,3),(0.,1.),.UNSPECIFIED.);
#23474=B_SPLINE_CURVE_WITH_KNOTS('',2,(#80329,#80330,#80331),
 .UNSPECIFIED.,.F.,.F.,(3,3),(0.,1.),.UNSPECIFIED.);
#23475=B_SPLINE_CURVE_WITH_KNOTS('',2,(#80334,#80335,#80336),
 .UNSPECIFIED.,.F.,.F.,(3,3),(0.,1.),.UNSPECIFIED.);
#23476=B_SPLINE_CURVE_WITH_KNOTS('',2,(#80344,#80345,#80346),
 .UNSPECIFIED.,.F.,.F.,(3,3),(0.,1.),.UNSPECIFIED.);
#23477=B_SPLINE_CURVE_WITH_KNOTS('',2,(#80349,#80350,#80351),
 .UNSPECIFIED.,.F.,.F.,(3,3),(0.,1.),.UNSPECIFIED.);
#23478=B_SPLINE_CURVE_WITH_KNOTS('',2,(#80359,#80360,#80361),
 .UNSPECIFIED.,.F.,.F.,(3,3),(0.,1.),.UNSPECIFIED.);
#23479=B_SPLINE_CURVE_WITH_KNOTS('',2,(#80364,#80365,#80366),
 .UNSPECIFIED.,.F.,.F.,(3,3),(0.,1.),.UNSPECIFIED.);
#23480=B_SPLINE_CURVE_WITH_KNOTS('',2,(#80374,#80375,#80376),
 .UNSPECIFIED.,.F.,.F.,(3,3),(0.,1.),.UNSPECIFIED.);
#23481=B_SPLINE_CURVE_WITH_KNOTS('',2,(#80379,#80380,#80381),
 .UNSPECIFIED.,.F.,.F.,(3,3),(0.,1.),.UNSPECIFIED.);
#23482=B_SPLINE_CURVE_WITH_KNOTS('',2,(#80395,#80396,#80397),
 .UNSPECIFIED.,.F.,.F.,(3,3),(0.,1.),.UNSPECIFIED.);
#23483=B_SPLINE_CURVE_WITH_KNOTS('',2,(#80400,#80401,#80402),
 .UNSPECIFIED.,.F.,.F.,(3,3),(0.,1.),.UNSPECIFIED.);
#23484=B_SPLINE_CURVE_WITH_KNOTS('',2,(#80410,#80411,#80412),
 .UNSPECIFIED.,.F.,.F.,(3,3),(0.,1.),.UNSPECIFIED.);
#23485=B_SPLINE_CURVE_WITH_KNOTS('',2,(#80415,#80416,#80417),
 .UNSPECIFIED.,.F.,.F.,(3,3),(0.,1.),.UNSPECIFIED.);
#23486=B_SPLINE_CURVE_WITH_KNOTS('',2,(#80425,#80426,#80427),
 .UNSPECIFIED.,.F.,.F.,(3,3),(0.,1.),.UNSPECIFIED.);
#23487=B_SPLINE_CURVE_WITH_KNOTS('',2,(#80430,#80431,#80432),
 .UNSPECIFIED.,.F.,.F.,(3,3),(0.,1.),.UNSPECIFIED.);
#23488=B_SPLINE_CURVE_WITH_KNOTS('',2,(#80440,#80441,#80442),
 .UNSPECIFIED.,.F.,.F.,(3,3),(0.,1.),.UNSPECIFIED.);
#23489=B_SPLINE_CURVE_WITH_KNOTS('',2,(#80445,#80446,#80447),
 .UNSPECIFIED.,.F.,.F.,(3,3),(0.,1.),.UNSPECIFIED.);
#23490=B_SPLINE_CURVE_WITH_KNOTS('',2,(#80455,#80456,#80457),
 .UNSPECIFIED.,.F.,.F.,(3,3),(0.,1.),.UNSPECIFIED.);
#23491=B_SPLINE_CURVE_WITH_KNOTS('',2,(#80460,#80461,#80462),
 .UNSPECIFIED.,.F.,.F.,(3,3),(0.,1.),.UNSPECIFIED.);
#23492=B_SPLINE_CURVE_WITH_KNOTS('',2,(#80470,#80471,#80472),
 .UNSPECIFIED.,.F.,.F.,(3,3),(0.,1.),.UNSPECIFIED.);
#23493=B_SPLINE_CURVE_WITH_KNOTS('',2,(#80475,#80476,#80477),
 .UNSPECIFIED.,.F.,.F.,(3,3),(0.,1.),.UNSPECIFIED.);
#23494=B_SPLINE_CURVE_WITH_KNOTS('',2,(#80485,#80486,#80487),
 .UNSPECIFIED.,.F.,.F.,(3,3),(0.,1.),.UNSPECIFIED.);
#23495=B_SPLINE_CURVE_WITH_KNOTS('',2,(#80490,#80491,#80492),
 .UNSPECIFIED.,.F.,.F.,(3,3),(0.,1.),.UNSPECIFIED.);
#23496=B_SPLINE_CURVE_WITH_KNOTS('',2,(#80505,#80506,#80507),
 .UNSPECIFIED.,.F.,.F.,(3,3),(0.,1.),.UNSPECIFIED.);
#23497=B_SPLINE_CURVE_WITH_KNOTS('',2,(#80508,#80509,#80510),
 .UNSPECIFIED.,.F.,.F.,(3,3),(0.,1.),.UNSPECIFIED.);
#23498=B_SPLINE_CURVE_WITH_KNOTS('',2,(#80521,#80522,#80523),
 .UNSPECIFIED.,.F.,.F.,(3,3),(0.,1.),.UNSPECIFIED.);
#23499=B_SPLINE_CURVE_WITH_KNOTS('',2,(#80527,#80528,#80529),
 .UNSPECIFIED.,.F.,.F.,(3,3),(0.,1.),.UNSPECIFIED.);
#23500=B_SPLINE_CURVE_WITH_KNOTS('',2,(#80538,#80539,#80540),
 .UNSPECIFIED.,.F.,.F.,(3,3),(0.,1.),.UNSPECIFIED.);
#23501=B_SPLINE_CURVE_WITH_KNOTS('',2,(#80543,#80544,#80545),
 .UNSPECIFIED.,.F.,.F.,(3,3),(0.,1.),.UNSPECIFIED.);
#23502=B_SPLINE_CURVE_WITH_KNOTS('',2,(#80553,#80554,#80555),
 .UNSPECIFIED.,.F.,.F.,(3,3),(0.,1.),.UNSPECIFIED.);
#23503=B_SPLINE_CURVE_WITH_KNOTS('',2,(#80558,#80559,#80560),
 .UNSPECIFIED.,.F.,.F.,(3,3),(0.,1.),.UNSPECIFIED.);
#23504=B_SPLINE_CURVE_WITH_KNOTS('',2,(#80568,#80569,#80570),
 .UNSPECIFIED.,.F.,.F.,(3,3),(0.,1.),.UNSPECIFIED.);
#23505=B_SPLINE_CURVE_WITH_KNOTS('',2,(#80573,#80574,#80575),
 .UNSPECIFIED.,.F.,.F.,(3,3),(0.,1.),.UNSPECIFIED.);
#23506=B_SPLINE_CURVE_WITH_KNOTS('',2,(#80583,#80584,#80585),
 .UNSPECIFIED.,.F.,.F.,(3,3),(0.,1.),.UNSPECIFIED.);
#23507=B_SPLINE_CURVE_WITH_KNOTS('',2,(#80588,#80589,#80590),
 .UNSPECIFIED.,.F.,.F.,(3,3),(0.,1.),.UNSPECIFIED.);
#23508=B_SPLINE_CURVE_WITH_KNOTS('',2,(#80598,#80599,#80600),
 .UNSPECIFIED.,.F.,.F.,(3,3),(0.,1.),.UNSPECIFIED.);
#23509=B_SPLINE_CURVE_WITH_KNOTS('',2,(#80603,#80604,#80605),
 .UNSPECIFIED.,.F.,.F.,(3,3),(0.,1.),.UNSPECIFIED.);
#23510=B_SPLINE_CURVE_WITH_KNOTS('',2,(#80613,#80614,#80615),
 .UNSPECIFIED.,.F.,.F.,(3,3),(0.,1.),.UNSPECIFIED.);
#23511=B_SPLINE_CURVE_WITH_KNOTS('',2,(#80618,#80619,#80620),
 .UNSPECIFIED.,.F.,.F.,(3,3),(0.,1.),.UNSPECIFIED.);
#23512=B_SPLINE_CURVE_WITH_KNOTS('',2,(#80627,#80628,#80629),
 .UNSPECIFIED.,.F.,.F.,(3,3),(0.,1.),.UNSPECIFIED.);
#23513=B_SPLINE_CURVE_WITH_KNOTS('',2,(#80630,#80631,#80632),
 .UNSPECIFIED.,.F.,.F.,(3,3),(0.,1.),.UNSPECIFIED.);
#23514=B_SPLINE_CURVE_WITH_KNOTS('',2,(#80641,#80642,#80643),
 .UNSPECIFIED.,.F.,.F.,(3,3),(0.,1.),.UNSPECIFIED.);
#23515=B_SPLINE_CURVE_WITH_KNOTS('',2,(#80647,#80648,#80649),
 .UNSPECIFIED.,.F.,.F.,(3,3),(0.,1.),.UNSPECIFIED.);
#23516=B_SPLINE_CURVE_WITH_KNOTS('',2,(#80658,#80659,#80660),
 .UNSPECIFIED.,.F.,.F.,(3,3),(0.,1.),.UNSPECIFIED.);
#23517=B_SPLINE_CURVE_WITH_KNOTS('',2,(#80663,#80664,#80665),
 .UNSPECIFIED.,.F.,.F.,(3,3),(0.,1.),.UNSPECIFIED.);
#23518=B_SPLINE_CURVE_WITH_KNOTS('',2,(#80673,#80674,#80675),
 .UNSPECIFIED.,.F.,.F.,(3,3),(0.,1.),.UNSPECIFIED.);
#23519=B_SPLINE_CURVE_WITH_KNOTS('',2,(#80678,#80679,#80680),
 .UNSPECIFIED.,.F.,.F.,(3,3),(0.,1.),.UNSPECIFIED.);
#23520=B_SPLINE_CURVE_WITH_KNOTS('',2,(#80688,#80689,#80690),
 .UNSPECIFIED.,.F.,.F.,(3,3),(0.,1.),.UNSPECIFIED.);
#23521=B_SPLINE_CURVE_WITH_KNOTS('',2,(#80693,#80694,#80695),
 .UNSPECIFIED.,.F.,.F.,(3,3),(0.,1.),.UNSPECIFIED.);
#23522=B_SPLINE_CURVE_WITH_KNOTS('',2,(#80703,#80704,#80705),
 .UNSPECIFIED.,.F.,.F.,(3,3),(0.,1.),.UNSPECIFIED.);
#23523=B_SPLINE_CURVE_WITH_KNOTS('',2,(#80708,#80709,#80710),
 .UNSPECIFIED.,.F.,.F.,(3,3),(0.,1.),.UNSPECIFIED.);
#23524=B_SPLINE_CURVE_WITH_KNOTS('',2,(#80718,#80719,#80720),
 .UNSPECIFIED.,.F.,.F.,(3,3),(0.,1.),.UNSPECIFIED.);
#23525=B_SPLINE_CURVE_WITH_KNOTS('',2,(#80723,#80724,#80725),
 .UNSPECIFIED.,.F.,.F.,(3,3),(0.,1.),.UNSPECIFIED.);
#23526=B_SPLINE_CURVE_WITH_KNOTS('',2,(#80733,#80734,#80735),
 .UNSPECIFIED.,.F.,.F.,(3,3),(0.,1.),.UNSPECIFIED.);
#23527=B_SPLINE_CURVE_WITH_KNOTS('',2,(#80738,#80739,#80740),
 .UNSPECIFIED.,.F.,.F.,(3,3),(0.,1.),.UNSPECIFIED.);
#23528=B_SPLINE_CURVE_WITH_KNOTS('',2,(#80748,#80749,#80750),
 .UNSPECIFIED.,.F.,.F.,(3,3),(0.,1.),.UNSPECIFIED.);
#23529=B_SPLINE_CURVE_WITH_KNOTS('',2,(#80753,#80754,#80755),
 .UNSPECIFIED.,.F.,.F.,(3,3),(0.,1.),.UNSPECIFIED.);
#23530=B_SPLINE_CURVE_WITH_KNOTS('',2,(#80763,#80764,#80765),
 .UNSPECIFIED.,.F.,.F.,(3,3),(0.,1.),.UNSPECIFIED.);
#23531=B_SPLINE_CURVE_WITH_KNOTS('',2,(#80768,#80769,#80770),
 .UNSPECIFIED.,.F.,.F.,(3,3),(0.,1.),.UNSPECIFIED.);
#23532=B_SPLINE_CURVE_WITH_KNOTS('',2,(#80778,#80779,#80780),
 .UNSPECIFIED.,.F.,.F.,(3,3),(0.,1.),.UNSPECIFIED.);
#23533=B_SPLINE_CURVE_WITH_KNOTS('',2,(#80783,#80784,#80785),
 .UNSPECIFIED.,.F.,.F.,(3,3),(0.,1.),.UNSPECIFIED.);
#23534=B_SPLINE_CURVE_WITH_KNOTS('',2,(#80793,#80794,#80795),
 .UNSPECIFIED.,.F.,.F.,(3,3),(0.,1.),.UNSPECIFIED.);
#23535=B_SPLINE_CURVE_WITH_KNOTS('',2,(#80798,#80799,#80800),
 .UNSPECIFIED.,.F.,.F.,(3,3),(0.,1.),.UNSPECIFIED.);
#23536=B_SPLINE_CURVE_WITH_KNOTS('',2,(#80807,#80808,#80809),
 .UNSPECIFIED.,.F.,.F.,(3,3),(0.,1.),.UNSPECIFIED.);
#23537=B_SPLINE_CURVE_WITH_KNOTS('',2,(#80810,#80811,#80812),
 .UNSPECIFIED.,.F.,.F.,(3,3),(0.,1.),.UNSPECIFIED.);
#23538=B_SPLINE_CURVE_WITH_KNOTS('',2,(#80822,#80823,#80824),
 .UNSPECIFIED.,.F.,.F.,(3,3),(0.,1.),.UNSPECIFIED.);
#23539=B_SPLINE_CURVE_WITH_KNOTS('',2,(#80828,#80829,#80830),
 .UNSPECIFIED.,.F.,.F.,(3,3),(0.,1.),.UNSPECIFIED.);
#23540=B_SPLINE_CURVE_WITH_KNOTS('',2,(#80839,#80840,#80841),
 .UNSPECIFIED.,.F.,.F.,(3,3),(0.,1.),.UNSPECIFIED.);
#23541=B_SPLINE_CURVE_WITH_KNOTS('',2,(#80844,#80845,#80846),
 .UNSPECIFIED.,.F.,.F.,(3,3),(0.,1.),.UNSPECIFIED.);
#23542=B_SPLINE_CURVE_WITH_KNOTS('',2,(#80854,#80855,#80856),
 .UNSPECIFIED.,.F.,.F.,(3,3),(0.,1.),.UNSPECIFIED.);
#23543=B_SPLINE_CURVE_WITH_KNOTS('',2,(#80859,#80860,#80861),
 .UNSPECIFIED.,.F.,.F.,(3,3),(0.,1.),.UNSPECIFIED.);
#23544=B_SPLINE_CURVE_WITH_KNOTS('',2,(#80869,#80870,#80871),
 .UNSPECIFIED.,.F.,.F.,(3,3),(0.,1.),.UNSPECIFIED.);
#23545=B_SPLINE_CURVE_WITH_KNOTS('',2,(#80874,#80875,#80876),
 .UNSPECIFIED.,.F.,.F.,(3,3),(0.,1.),.UNSPECIFIED.);
#23546=B_SPLINE_CURVE_WITH_KNOTS('',2,(#80884,#80885,#80886),
 .UNSPECIFIED.,.F.,.F.,(3,3),(0.,1.),.UNSPECIFIED.);
#23547=B_SPLINE_CURVE_WITH_KNOTS('',2,(#80889,#80890,#80891),
 .UNSPECIFIED.,.F.,.F.,(3,3),(0.,1.),.UNSPECIFIED.);
#23548=B_SPLINE_CURVE_WITH_KNOTS('',2,(#80899,#80900,#80901),
 .UNSPECIFIED.,.F.,.F.,(3,3),(0.,1.),.UNSPECIFIED.);
#23549=B_SPLINE_CURVE_WITH_KNOTS('',2,(#80904,#80905,#80906),
 .UNSPECIFIED.,.F.,.F.,(3,3),(0.,1.),.UNSPECIFIED.);
#23550=B_SPLINE_CURVE_WITH_KNOTS('',2,(#80914,#80915,#80916),
 .UNSPECIFIED.,.F.,.F.,(3,3),(0.,1.),.UNSPECIFIED.);
#23551=B_SPLINE_CURVE_WITH_KNOTS('',2,(#80919,#80920,#80921),
 .UNSPECIFIED.,.F.,.F.,(3,3),(0.,1.),.UNSPECIFIED.);
#23552=B_SPLINE_CURVE_WITH_KNOTS('',2,(#80929,#80930,#80931),
 .UNSPECIFIED.,.F.,.F.,(3,3),(0.,1.),.UNSPECIFIED.);
#23553=B_SPLINE_CURVE_WITH_KNOTS('',2,(#80934,#80935,#80936),
 .UNSPECIFIED.,.F.,.F.,(3,3),(0.,1.),.UNSPECIFIED.);
#23554=B_SPLINE_CURVE_WITH_KNOTS('',2,(#80944,#80945,#80946),
 .UNSPECIFIED.,.F.,.F.,(3,3),(0.,1.),.UNSPECIFIED.);
#23555=B_SPLINE_CURVE_WITH_KNOTS('',2,(#80949,#80950,#80951),
 .UNSPECIFIED.,.F.,.F.,(3,3),(0.,1.),.UNSPECIFIED.);
#23556=B_SPLINE_CURVE_WITH_KNOTS('',2,(#80965,#80966,#80967),
 .UNSPECIFIED.,.F.,.F.,(3,3),(0.,1.),.UNSPECIFIED.);
#23557=B_SPLINE_CURVE_WITH_KNOTS('',2,(#80970,#80971,#80972),
 .UNSPECIFIED.,.F.,.F.,(3,3),(0.,1.),.UNSPECIFIED.);
#23558=B_SPLINE_CURVE_WITH_KNOTS('',2,(#80980,#80981,#80982),
 .UNSPECIFIED.,.F.,.F.,(3,3),(0.,1.),.UNSPECIFIED.);
#23559=B_SPLINE_CURVE_WITH_KNOTS('',2,(#80985,#80986,#80987),
 .UNSPECIFIED.,.F.,.F.,(3,3),(0.,1.),.UNSPECIFIED.);
#23560=B_SPLINE_CURVE_WITH_KNOTS('',2,(#80995,#80996,#80997),
 .UNSPECIFIED.,.F.,.F.,(3,3),(0.,1.),.UNSPECIFIED.);
#23561=B_SPLINE_CURVE_WITH_KNOTS('',2,(#81000,#81001,#81002),
 .UNSPECIFIED.,.F.,.F.,(3,3),(0.,1.),.UNSPECIFIED.);
#23562=B_SPLINE_CURVE_WITH_KNOTS('',2,(#81010,#81011,#81012),
 .UNSPECIFIED.,.F.,.F.,(3,3),(0.,1.),.UNSPECIFIED.);
#23563=B_SPLINE_CURVE_WITH_KNOTS('',2,(#81015,#81016,#81017),
 .UNSPECIFIED.,.F.,.F.,(3,3),(0.,1.),.UNSPECIFIED.);
#23564=B_SPLINE_CURVE_WITH_KNOTS('',2,(#81025,#81026,#81027),
 .UNSPECIFIED.,.F.,.F.,(3,3),(0.,1.),.UNSPECIFIED.);
#23565=B_SPLINE_CURVE_WITH_KNOTS('',2,(#81030,#81031,#81032),
 .UNSPECIFIED.,.F.,.F.,(3,3),(0.,1.),.UNSPECIFIED.);
#23566=B_SPLINE_CURVE_WITH_KNOTS('',2,(#81040,#81041,#81042),
 .UNSPECIFIED.,.F.,.F.,(3,3),(0.,1.),.UNSPECIFIED.);
#23567=B_SPLINE_CURVE_WITH_KNOTS('',2,(#81045,#81046,#81047),
 .UNSPECIFIED.,.F.,.F.,(3,3),(0.,1.),.UNSPECIFIED.);
#23568=B_SPLINE_CURVE_WITH_KNOTS('',2,(#81055,#81056,#81057),
 .UNSPECIFIED.,.F.,.F.,(3,3),(0.,1.),.UNSPECIFIED.);
#23569=B_SPLINE_CURVE_WITH_KNOTS('',2,(#81060,#81061,#81062),
 .UNSPECIFIED.,.F.,.F.,(3,3),(0.,1.),.UNSPECIFIED.);
#23570=B_SPLINE_CURVE_WITH_KNOTS('',2,(#81070,#81071,#81072),
 .UNSPECIFIED.,.F.,.F.,(3,3),(0.,1.),.UNSPECIFIED.);
#23571=B_SPLINE_CURVE_WITH_KNOTS('',2,(#81075,#81076,#81077),
 .UNSPECIFIED.,.F.,.F.,(3,3),(0.,1.),.UNSPECIFIED.);
#23572=B_SPLINE_CURVE_WITH_KNOTS('',2,(#81085,#81086,#81087),
 .UNSPECIFIED.,.F.,.F.,(3,3),(0.,1.),.UNSPECIFIED.);
#23573=B_SPLINE_CURVE_WITH_KNOTS('',2,(#81090,#81091,#81092),
 .UNSPECIFIED.,.F.,.F.,(3,3),(0.,1.),.UNSPECIFIED.);
#23574=B_SPLINE_CURVE_WITH_KNOTS('',2,(#81118,#81119,#81120),
 .UNSPECIFIED.,.F.,.F.,(3,3),(0.,1.),.UNSPECIFIED.);
#23575=B_SPLINE_CURVE_WITH_KNOTS('',2,(#81124,#81125,#81126),
 .UNSPECIFIED.,.F.,.F.,(3,3),(0.,1.),.UNSPECIFIED.);
#23576=B_SPLINE_CURVE_WITH_KNOTS('',2,(#81135,#81136,#81137),
 .UNSPECIFIED.,.F.,.F.,(3,3),(0.,1.),.UNSPECIFIED.);
#23577=B_SPLINE_CURVE_WITH_KNOTS('',2,(#81140,#81141,#81142),
 .UNSPECIFIED.,.F.,.F.,(3,3),(0.,1.),.UNSPECIFIED.);
#23578=B_SPLINE_CURVE_WITH_KNOTS('',2,(#81150,#81151,#81152),
 .UNSPECIFIED.,.F.,.F.,(3,3),(0.,1.),.UNSPECIFIED.);
#23579=B_SPLINE_CURVE_WITH_KNOTS('',2,(#81155,#81156,#81157),
 .UNSPECIFIED.,.F.,.F.,(3,3),(0.,1.),.UNSPECIFIED.);
#23580=B_SPLINE_CURVE_WITH_KNOTS('',2,(#81165,#81166,#81167),
 .UNSPECIFIED.,.F.,.F.,(3,3),(0.,1.),.UNSPECIFIED.);
#23581=B_SPLINE_CURVE_WITH_KNOTS('',2,(#81170,#81171,#81172),
 .UNSPECIFIED.,.F.,.F.,(3,3),(0.,1.),.UNSPECIFIED.);
#23582=B_SPLINE_CURVE_WITH_KNOTS('',2,(#81180,#81181,#81182),
 .UNSPECIFIED.,.F.,.F.,(3,3),(0.,1.),.UNSPECIFIED.);
#23583=B_SPLINE_CURVE_WITH_KNOTS('',2,(#81185,#81186,#81187),
 .UNSPECIFIED.,.F.,.F.,(3,3),(0.,1.),.UNSPECIFIED.);
#23584=B_SPLINE_CURVE_WITH_KNOTS('',2,(#81195,#81196,#81197),
 .UNSPECIFIED.,.F.,.F.,(3,3),(0.,1.),.UNSPECIFIED.);
#23585=B_SPLINE_CURVE_WITH_KNOTS('',2,(#81200,#81201,#81202),
 .UNSPECIFIED.,.F.,.F.,(3,3),(0.,1.),.UNSPECIFIED.);
#23586=B_SPLINE_CURVE_WITH_KNOTS('',2,(#81210,#81211,#81212),
 .UNSPECIFIED.,.F.,.F.,(3,3),(0.,1.),.UNSPECIFIED.);
#23587=B_SPLINE_CURVE_WITH_KNOTS('',2,(#81215,#81216,#81217),
 .UNSPECIFIED.,.F.,.F.,(3,3),(0.,1.),.UNSPECIFIED.);
#23588=B_SPLINE_CURVE_WITH_KNOTS('',2,(#81224,#81225,#81226),
 .UNSPECIFIED.,.F.,.F.,(3,3),(0.,1.),.UNSPECIFIED.);
#23589=B_SPLINE_CURVE_WITH_KNOTS('',2,(#81227,#81228,#81229),
 .UNSPECIFIED.,.F.,.F.,(3,3),(0.,1.),.UNSPECIFIED.);
#23590=B_SPLINE_CURVE_WITH_KNOTS('',2,(#81238,#81239,#81240),
 .UNSPECIFIED.,.F.,.F.,(3,3),(0.,1.),.UNSPECIFIED.);
#23591=B_SPLINE_CURVE_WITH_KNOTS('',2,(#81244,#81245,#81246),
 .UNSPECIFIED.,.F.,.F.,(3,3),(0.,1.),.UNSPECIFIED.);
#23592=B_SPLINE_CURVE_WITH_KNOTS('',2,(#81255,#81256,#81257),
 .UNSPECIFIED.,.F.,.F.,(3,3),(0.,1.),.UNSPECIFIED.);
#23593=B_SPLINE_CURVE_WITH_KNOTS('',2,(#81260,#81261,#81262),
 .UNSPECIFIED.,.F.,.F.,(3,3),(0.,1.),.UNSPECIFIED.);
#23594=B_SPLINE_CURVE_WITH_KNOTS('',2,(#81270,#81271,#81272),
 .UNSPECIFIED.,.F.,.F.,(3,3),(0.,1.),.UNSPECIFIED.);
#23595=B_SPLINE_CURVE_WITH_KNOTS('',2,(#81275,#81276,#81277),
 .UNSPECIFIED.,.F.,.F.,(3,3),(0.,1.),.UNSPECIFIED.);
#23596=B_SPLINE_CURVE_WITH_KNOTS('',2,(#81285,#81286,#81287),
 .UNSPECIFIED.,.F.,.F.,(3,3),(0.,1.),.UNSPECIFIED.);
#23597=B_SPLINE_CURVE_WITH_KNOTS('',2,(#81290,#81291,#81292),
 .UNSPECIFIED.,.F.,.F.,(3,3),(0.,1.),.UNSPECIFIED.);
#23598=B_SPLINE_CURVE_WITH_KNOTS('',2,(#81300,#81301,#81302),
 .UNSPECIFIED.,.F.,.F.,(3,3),(0.,1.),.UNSPECIFIED.);
#23599=B_SPLINE_CURVE_WITH_KNOTS('',2,(#81305,#81306,#81307),
 .UNSPECIFIED.,.F.,.F.,(3,3),(0.,1.),.UNSPECIFIED.);
#23600=B_SPLINE_CURVE_WITH_KNOTS('',2,(#81315,#81316,#81317),
 .UNSPECIFIED.,.F.,.F.,(3,3),(0.,1.),.UNSPECIFIED.);
#23601=B_SPLINE_CURVE_WITH_KNOTS('',2,(#81320,#81321,#81322),
 .UNSPECIFIED.,.F.,.F.,(3,3),(0.,1.),.UNSPECIFIED.);
#23602=B_SPLINE_CURVE_WITH_KNOTS('',2,(#81330,#81331,#81332),
 .UNSPECIFIED.,.F.,.F.,(3,3),(0.,1.),.UNSPECIFIED.);
#23603=B_SPLINE_CURVE_WITH_KNOTS('',2,(#81335,#81336,#81337),
 .UNSPECIFIED.,.F.,.F.,(3,3),(0.,1.),.UNSPECIFIED.);
#23604=B_SPLINE_CURVE_WITH_KNOTS('',2,(#81345,#81346,#81347),
 .UNSPECIFIED.,.F.,.F.,(3,3),(0.,1.),.UNSPECIFIED.);
#23605=B_SPLINE_CURVE_WITH_KNOTS('',2,(#81350,#81351,#81352),
 .UNSPECIFIED.,.F.,.F.,(3,3),(0.,1.),.UNSPECIFIED.);
#23606=B_SPLINE_CURVE_WITH_KNOTS('',2,(#81360,#81361,#81362),
 .UNSPECIFIED.,.F.,.F.,(3,3),(0.,1.),.UNSPECIFIED.);
#23607=B_SPLINE_CURVE_WITH_KNOTS('',2,(#81365,#81366,#81367),
 .UNSPECIFIED.,.F.,.F.,(3,3),(0.,1.),.UNSPECIFIED.);
#23608=B_SPLINE_CURVE_WITH_KNOTS('',2,(#81375,#81376,#81377),
 .UNSPECIFIED.,.F.,.F.,(3,3),(0.,1.),.UNSPECIFIED.);
#23609=B_SPLINE_CURVE_WITH_KNOTS('',2,(#81380,#81381,#81382),
 .UNSPECIFIED.,.F.,.F.,(3,3),(0.,1.),.UNSPECIFIED.);
#23610=B_SPLINE_CURVE_WITH_KNOTS('',2,(#81390,#81391,#81392),
 .UNSPECIFIED.,.F.,.F.,(3,3),(0.,1.),.UNSPECIFIED.);
#23611=B_SPLINE_CURVE_WITH_KNOTS('',2,(#81395,#81396,#81397),
 .UNSPECIFIED.,.F.,.F.,(3,3),(0.,1.),.UNSPECIFIED.);
#23612=B_SPLINE_CURVE_WITH_KNOTS('',2,(#81404,#81405,#81406),
 .UNSPECIFIED.,.F.,.F.,(3,3),(0.,1.),.UNSPECIFIED.);
#23613=B_SPLINE_CURVE_WITH_KNOTS('',2,(#81407,#81408,#81409),
 .UNSPECIFIED.,.F.,.F.,(3,3),(0.,1.),.UNSPECIFIED.);
#23614=B_SPLINE_CURVE_WITH_KNOTS('',2,(#81427,#81428,#81429),
 .UNSPECIFIED.,.F.,.F.,(3,3),(0.,1.),.UNSPECIFIED.);
#23615=B_SPLINE_CURVE_WITH_KNOTS('',2,(#81432,#81433,#81434),
 .UNSPECIFIED.,.F.,.F.,(3,3),(0.,1.),.UNSPECIFIED.);
#23616=B_SPLINE_CURVE_WITH_KNOTS('',2,(#81442,#81443,#81444),
 .UNSPECIFIED.,.F.,.F.,(3,3),(0.,1.),.UNSPECIFIED.);
#23617=B_SPLINE_CURVE_WITH_KNOTS('',2,(#81447,#81448,#81449),
 .UNSPECIFIED.,.F.,.F.,(3,3),(0.,1.),.UNSPECIFIED.);
#23618=B_SPLINE_CURVE_WITH_KNOTS('',2,(#81463,#81464,#81465),
 .UNSPECIFIED.,.F.,.F.,(3,3),(0.,1.),.UNSPECIFIED.);
#23619=B_SPLINE_CURVE_WITH_KNOTS('',2,(#81468,#81469,#81470),
 .UNSPECIFIED.,.F.,.F.,(3,3),(0.,1.),.UNSPECIFIED.);
#23620=B_SPLINE_CURVE_WITH_KNOTS('',2,(#81478,#81479,#81480),
 .UNSPECIFIED.,.F.,.F.,(3,3),(0.,1.),.UNSPECIFIED.);
#23621=B_SPLINE_CURVE_WITH_KNOTS('',2,(#81483,#81484,#81485),
 .UNSPECIFIED.,.F.,.F.,(3,3),(0.,1.),.UNSPECIFIED.);
#23622=B_SPLINE_CURVE_WITH_KNOTS('',2,(#81511,#81512,#81513),
 .UNSPECIFIED.,.F.,.F.,(3,3),(0.,1.),.UNSPECIFIED.);
#23623=B_SPLINE_CURVE_WITH_KNOTS('',2,(#81517,#81518,#81519),
 .UNSPECIFIED.,.F.,.F.,(3,3),(0.,1.),.UNSPECIFIED.);
#23624=B_SPLINE_CURVE_WITH_KNOTS('',2,(#81528,#81529,#81530),
 .UNSPECIFIED.,.F.,.F.,(3,3),(0.,1.),.UNSPECIFIED.);
#23625=B_SPLINE_CURVE_WITH_KNOTS('',2,(#81533,#81534,#81535),
 .UNSPECIFIED.,.F.,.F.,(3,3),(0.,1.),.UNSPECIFIED.);
#23626=B_SPLINE_CURVE_WITH_KNOTS('',2,(#81543,#81544,#81545),
 .UNSPECIFIED.,.F.,.F.,(3,3),(0.,1.),.UNSPECIFIED.);
#23627=B_SPLINE_CURVE_WITH_KNOTS('',2,(#81548,#81549,#81550),
 .UNSPECIFIED.,.F.,.F.,(3,3),(0.,1.),.UNSPECIFIED.);
#23628=B_SPLINE_CURVE_WITH_KNOTS('',2,(#81558,#81559,#81560),
 .UNSPECIFIED.,.F.,.F.,(3,3),(0.,1.),.UNSPECIFIED.);
#23629=B_SPLINE_CURVE_WITH_KNOTS('',2,(#81563,#81564,#81565),
 .UNSPECIFIED.,.F.,.F.,(3,3),(0.,1.),.UNSPECIFIED.);
#23630=B_SPLINE_CURVE_WITH_KNOTS('',2,(#81573,#81574,#81575),
 .UNSPECIFIED.,.F.,.F.,(3,3),(0.,1.),.UNSPECIFIED.);
#23631=B_SPLINE_CURVE_WITH_KNOTS('',2,(#81578,#81579,#81580),
 .UNSPECIFIED.,.F.,.F.,(3,3),(0.,1.),.UNSPECIFIED.);
#23632=B_SPLINE_CURVE_WITH_KNOTS('',2,(#81588,#81589,#81590),
 .UNSPECIFIED.,.F.,.F.,(3,3),(0.,1.),.UNSPECIFIED.);
#23633=B_SPLINE_CURVE_WITH_KNOTS('',2,(#81593,#81594,#81595),
 .UNSPECIFIED.,.F.,.F.,(3,3),(0.,1.),.UNSPECIFIED.);
#23634=B_SPLINE_CURVE_WITH_KNOTS('',2,(#81603,#81604,#81605),
 .UNSPECIFIED.,.F.,.F.,(3,3),(0.,1.),.UNSPECIFIED.);
#23635=B_SPLINE_CURVE_WITH_KNOTS('',2,(#81608,#81609,#81610),
 .UNSPECIFIED.,.F.,.F.,(3,3),(0.,1.),.UNSPECIFIED.);
#23636=B_SPLINE_CURVE_WITH_KNOTS('',2,(#81617,#81618,#81619),
 .UNSPECIFIED.,.F.,.F.,(3,3),(0.,1.),.UNSPECIFIED.);
#23637=B_SPLINE_CURVE_WITH_KNOTS('',2,(#81620,#81621,#81622),
 .UNSPECIFIED.,.F.,.F.,(3,3),(0.,1.),.UNSPECIFIED.);
#23638=B_SPLINE_CURVE_WITH_KNOTS('',2,(#81631,#81632,#81633),
 .UNSPECIFIED.,.F.,.F.,(3,3),(0.,1.),.UNSPECIFIED.);
#23639=B_SPLINE_CURVE_WITH_KNOTS('',2,(#81637,#81638,#81639),
 .UNSPECIFIED.,.F.,.F.,(3,3),(0.,1.),.UNSPECIFIED.);
#23640=B_SPLINE_CURVE_WITH_KNOTS('',2,(#81648,#81649,#81650),
 .UNSPECIFIED.,.F.,.F.,(3,3),(0.,1.),.UNSPECIFIED.);
#23641=B_SPLINE_CURVE_WITH_KNOTS('',2,(#81653,#81654,#81655),
 .UNSPECIFIED.,.F.,.F.,(3,3),(0.,1.),.UNSPECIFIED.);
#23642=B_SPLINE_CURVE_WITH_KNOTS('',2,(#81663,#81664,#81665),
 .UNSPECIFIED.,.F.,.F.,(3,3),(0.,1.),.UNSPECIFIED.);
#23643=B_SPLINE_CURVE_WITH_KNOTS('',2,(#81668,#81669,#81670),
 .UNSPECIFIED.,.F.,.F.,(3,3),(0.,1.),.UNSPECIFIED.);
#23644=B_SPLINE_CURVE_WITH_KNOTS('',2,(#81678,#81679,#81680),
 .UNSPECIFIED.,.F.,.F.,(3,3),(0.,1.),.UNSPECIFIED.);
#23645=B_SPLINE_CURVE_WITH_KNOTS('',2,(#81683,#81684,#81685),
 .UNSPECIFIED.,.F.,.F.,(3,3),(0.,1.),.UNSPECIFIED.);
#23646=B_SPLINE_CURVE_WITH_KNOTS('',2,(#81693,#81694,#81695),
 .UNSPECIFIED.,.F.,.F.,(3,3),(0.,1.),.UNSPECIFIED.);
#23647=B_SPLINE_CURVE_WITH_KNOTS('',2,(#81698,#81699,#81700),
 .UNSPECIFIED.,.F.,.F.,(3,3),(0.,1.),.UNSPECIFIED.);
#23648=B_SPLINE_CURVE_WITH_KNOTS('',2,(#81708,#81709,#81710),
 .UNSPECIFIED.,.F.,.F.,(3,3),(0.,1.),.UNSPECIFIED.);
#23649=B_SPLINE_CURVE_WITH_KNOTS('',2,(#81713,#81714,#81715),
 .UNSPECIFIED.,.F.,.F.,(3,3),(0.,1.),.UNSPECIFIED.);
#23650=B_SPLINE_CURVE_WITH_KNOTS('',2,(#81723,#81724,#81725),
 .UNSPECIFIED.,.F.,.F.,(3,3),(0.,1.),.UNSPECIFIED.);
#23651=B_SPLINE_CURVE_WITH_KNOTS('',2,(#81728,#81729,#81730),
 .UNSPECIFIED.,.F.,.F.,(3,3),(0.,1.),.UNSPECIFIED.);
#23652=B_SPLINE_CURVE_WITH_KNOTS('',2,(#81738,#81739,#81740),
 .UNSPECIFIED.,.F.,.F.,(3,3),(0.,1.),.UNSPECIFIED.);
#23653=B_SPLINE_CURVE_WITH_KNOTS('',2,(#81743,#81744,#81745),
 .UNSPECIFIED.,.F.,.F.,(3,3),(0.,1.),.UNSPECIFIED.);
#23654=B_SPLINE_CURVE_WITH_KNOTS('',2,(#81753,#81754,#81755),
 .UNSPECIFIED.,.F.,.F.,(3,3),(0.,1.),.UNSPECIFIED.);
#23655=B_SPLINE_CURVE_WITH_KNOTS('',2,(#81758,#81759,#81760),
 .UNSPECIFIED.,.F.,.F.,(3,3),(0.,1.),.UNSPECIFIED.);
#23656=B_SPLINE_CURVE_WITH_KNOTS('',2,(#81768,#81769,#81770),
 .UNSPECIFIED.,.F.,.F.,(3,3),(0.,1.),.UNSPECIFIED.);
#23657=B_SPLINE_CURVE_WITH_KNOTS('',2,(#81773,#81774,#81775),
 .UNSPECIFIED.,.F.,.F.,(3,3),(0.,1.),.UNSPECIFIED.);
#23658=B_SPLINE_CURVE_WITH_KNOTS('',2,(#81783,#81784,#81785),
 .UNSPECIFIED.,.F.,.F.,(3,3),(0.,1.),.UNSPECIFIED.);
#23659=B_SPLINE_CURVE_WITH_KNOTS('',2,(#81788,#81789,#81790),
 .UNSPECIFIED.,.F.,.F.,(3,3),(0.,1.),.UNSPECIFIED.);
#23660=B_SPLINE_CURVE_WITH_KNOTS('',2,(#81797,#81798,#81799),
 .UNSPECIFIED.,.F.,.F.,(3,3),(0.,1.),.UNSPECIFIED.);
#23661=B_SPLINE_CURVE_WITH_KNOTS('',2,(#81800,#81801,#81802),
 .UNSPECIFIED.,.F.,.F.,(3,3),(0.,1.),.UNSPECIFIED.);
#23662=B_SPLINE_CURVE_WITH_KNOTS('',2,(#81813,#81814,#81815),
 .UNSPECIFIED.,.F.,.F.,(3,3),(0.,1.),.UNSPECIFIED.);
#23663=B_SPLINE_CURVE_WITH_KNOTS('',2,(#81819,#81820,#81821),
 .UNSPECIFIED.,.F.,.F.,(3,3),(0.,1.),.UNSPECIFIED.);
#23664=B_SPLINE_CURVE_WITH_KNOTS('',2,(#81830,#81831,#81832),
 .UNSPECIFIED.,.F.,.F.,(3,3),(0.,1.),.UNSPECIFIED.);
#23665=B_SPLINE_CURVE_WITH_KNOTS('',2,(#81835,#81836,#81837),
 .UNSPECIFIED.,.F.,.F.,(3,3),(0.,1.),.UNSPECIFIED.);
#23666=B_SPLINE_CURVE_WITH_KNOTS('',2,(#81845,#81846,#81847),
 .UNSPECIFIED.,.F.,.F.,(3,3),(0.,1.),.UNSPECIFIED.);
#23667=B_SPLINE_CURVE_WITH_KNOTS('',2,(#81850,#81851,#81852),
 .UNSPECIFIED.,.F.,.F.,(3,3),(0.,1.),.UNSPECIFIED.);
#23668=B_SPLINE_CURVE_WITH_KNOTS('',2,(#81860,#81861,#81862),
 .UNSPECIFIED.,.F.,.F.,(3,3),(0.,1.),.UNSPECIFIED.);
#23669=B_SPLINE_CURVE_WITH_KNOTS('',2,(#81865,#81866,#81867),
 .UNSPECIFIED.,.F.,.F.,(3,3),(0.,1.),.UNSPECIFIED.);
#23670=B_SPLINE_CURVE_WITH_KNOTS('',2,(#81875,#81876,#81877),
 .UNSPECIFIED.,.F.,.F.,(3,3),(0.,1.),.UNSPECIFIED.);
#23671=B_SPLINE_CURVE_WITH_KNOTS('',2,(#81880,#81881,#81882),
 .UNSPECIFIED.,.F.,.F.,(3,3),(0.,1.),.UNSPECIFIED.);
#23672=B_SPLINE_CURVE_WITH_KNOTS('',2,(#81890,#81891,#81892),
 .UNSPECIFIED.,.F.,.F.,(3,3),(0.,1.),.UNSPECIFIED.);
#23673=B_SPLINE_CURVE_WITH_KNOTS('',2,(#81895,#81896,#81897),
 .UNSPECIFIED.,.F.,.F.,(3,3),(0.,1.),.UNSPECIFIED.);
#23674=B_SPLINE_CURVE_WITH_KNOTS('',2,(#81905,#81906,#81907),
 .UNSPECIFIED.,.F.,.F.,(3,3),(0.,1.),.UNSPECIFIED.);
#23675=B_SPLINE_CURVE_WITH_KNOTS('',2,(#81910,#81911,#81912),
 .UNSPECIFIED.,.F.,.F.,(3,3),(0.,1.),.UNSPECIFIED.);
#23676=B_SPLINE_CURVE_WITH_KNOTS('',2,(#81919,#81920,#81921),
 .UNSPECIFIED.,.F.,.F.,(3,3),(0.,1.),.UNSPECIFIED.);
#23677=B_SPLINE_CURVE_WITH_KNOTS('',2,(#81922,#81923,#81924),
 .UNSPECIFIED.,.F.,.F.,(3,3),(0.,1.),.UNSPECIFIED.);
#23678=B_SPLINE_CURVE_WITH_KNOTS('',2,(#81933,#81934,#81935),
 .UNSPECIFIED.,.F.,.F.,(3,3),(0.,1.),.UNSPECIFIED.);
#23679=B_SPLINE_CURVE_WITH_KNOTS('',2,(#81939,#81940,#81941),
 .UNSPECIFIED.,.F.,.F.,(3,3),(0.,1.),.UNSPECIFIED.);
#23680=B_SPLINE_CURVE_WITH_KNOTS('',2,(#81950,#81951,#81952),
 .UNSPECIFIED.,.F.,.F.,(3,3),(0.,1.),.UNSPECIFIED.);
#23681=B_SPLINE_CURVE_WITH_KNOTS('',2,(#81955,#81956,#81957),
 .UNSPECIFIED.,.F.,.F.,(3,3),(0.,1.),.UNSPECIFIED.);
#23682=B_SPLINE_CURVE_WITH_KNOTS('',2,(#81965,#81966,#81967),
 .UNSPECIFIED.,.F.,.F.,(3,3),(0.,1.),.UNSPECIFIED.);
#23683=B_SPLINE_CURVE_WITH_KNOTS('',2,(#81970,#81971,#81972),
 .UNSPECIFIED.,.F.,.F.,(3,3),(0.,1.),.UNSPECIFIED.);
#23684=B_SPLINE_CURVE_WITH_KNOTS('',2,(#81980,#81981,#81982),
 .UNSPECIFIED.,.F.,.F.,(3,3),(0.,1.),.UNSPECIFIED.);
#23685=B_SPLINE_CURVE_WITH_KNOTS('',2,(#81985,#81986,#81987),
 .UNSPECIFIED.,.F.,.F.,(3,3),(0.,1.),.UNSPECIFIED.);
#23686=B_SPLINE_CURVE_WITH_KNOTS('',2,(#81995,#81996,#81997),
 .UNSPECIFIED.,.F.,.F.,(3,3),(0.,1.),.UNSPECIFIED.);
#23687=B_SPLINE_CURVE_WITH_KNOTS('',2,(#82000,#82001,#82002),
 .UNSPECIFIED.,.F.,.F.,(3,3),(0.,1.),.UNSPECIFIED.);
#23688=B_SPLINE_CURVE_WITH_KNOTS('',2,(#82010,#82011,#82012),
 .UNSPECIFIED.,.F.,.F.,(3,3),(0.,1.),.UNSPECIFIED.);
#23689=B_SPLINE_CURVE_WITH_KNOTS('',2,(#82015,#82016,#82017),
 .UNSPECIFIED.,.F.,.F.,(3,3),(0.,1.),.UNSPECIFIED.);
#23690=B_SPLINE_CURVE_WITH_KNOTS('',2,(#82025,#82026,#82027),
 .UNSPECIFIED.,.F.,.F.,(3,3),(0.,1.),.UNSPECIFIED.);
#23691=B_SPLINE_CURVE_WITH_KNOTS('',2,(#82030,#82031,#82032),
 .UNSPECIFIED.,.F.,.F.,(3,3),(0.,1.),.UNSPECIFIED.);
#23692=B_SPLINE_CURVE_WITH_KNOTS('',2,(#82040,#82041,#82042),
 .UNSPECIFIED.,.F.,.F.,(3,3),(0.,1.),.UNSPECIFIED.);
#23693=B_SPLINE_CURVE_WITH_KNOTS('',2,(#82045,#82046,#82047),
 .UNSPECIFIED.,.F.,.F.,(3,3),(0.,1.),.UNSPECIFIED.);
#23694=B_SPLINE_CURVE_WITH_KNOTS('',2,(#82055,#82056,#82057),
 .UNSPECIFIED.,.F.,.F.,(3,3),(0.,1.),.UNSPECIFIED.);
#23695=B_SPLINE_CURVE_WITH_KNOTS('',2,(#82060,#82061,#82062),
 .UNSPECIFIED.,.F.,.F.,(3,3),(0.,1.),.UNSPECIFIED.);
#23696=B_SPLINE_CURVE_WITH_KNOTS('',2,(#82070,#82071,#82072),
 .UNSPECIFIED.,.F.,.F.,(3,3),(0.,1.),.UNSPECIFIED.);
#23697=B_SPLINE_CURVE_WITH_KNOTS('',2,(#82075,#82076,#82077),
 .UNSPECIFIED.,.F.,.F.,(3,3),(0.,1.),.UNSPECIFIED.);
#23698=B_SPLINE_CURVE_WITH_KNOTS('',2,(#82085,#82086,#82087),
 .UNSPECIFIED.,.F.,.F.,(3,3),(0.,1.),.UNSPECIFIED.);
#23699=B_SPLINE_CURVE_WITH_KNOTS('',2,(#82090,#82091,#82092),
 .UNSPECIFIED.,.F.,.F.,(3,3),(0.,1.),.UNSPECIFIED.);
#23700=B_SPLINE_CURVE_WITH_KNOTS('',2,(#82099,#82100,#82101),
 .UNSPECIFIED.,.F.,.F.,(3,3),(0.,1.),.UNSPECIFIED.);
#23701=B_SPLINE_CURVE_WITH_KNOTS('',2,(#82102,#82103,#82104),
 .UNSPECIFIED.,.F.,.F.,(3,3),(0.,1.),.UNSPECIFIED.);
#23702=B_SPLINE_CURVE_WITH_KNOTS('',2,(#82122,#82123,#82124),
 .UNSPECIFIED.,.F.,.F.,(3,3),(0.,1.),.UNSPECIFIED.);
#23703=B_SPLINE_CURVE_WITH_KNOTS('',2,(#82127,#82128,#82129),
 .UNSPECIFIED.,.F.,.F.,(3,3),(0.,1.),.UNSPECIFIED.);
#23704=B_SPLINE_CURVE_WITH_KNOTS('',2,(#82137,#82138,#82139),
 .UNSPECIFIED.,.F.,.F.,(3,3),(0.,1.),.UNSPECIFIED.);
#23705=B_SPLINE_CURVE_WITH_KNOTS('',2,(#82142,#82143,#82144),
 .UNSPECIFIED.,.F.,.F.,(3,3),(0.,1.),.UNSPECIFIED.);
#23706=B_SPLINE_CURVE_WITH_KNOTS('',2,(#82158,#82159,#82160),
 .UNSPECIFIED.,.F.,.F.,(3,3),(0.,1.),.UNSPECIFIED.);
#23707=B_SPLINE_CURVE_WITH_KNOTS('',2,(#82163,#82164,#82165),
 .UNSPECIFIED.,.F.,.F.,(3,3),(0.,1.),.UNSPECIFIED.);
#23708=B_SPLINE_CURVE_WITH_KNOTS('',2,(#82173,#82174,#82175),
 .UNSPECIFIED.,.F.,.F.,(3,3),(0.,1.),.UNSPECIFIED.);
#23709=B_SPLINE_CURVE_WITH_KNOTS('',2,(#82178,#82179,#82180),
 .UNSPECIFIED.,.F.,.F.,(3,3),(0.,1.),.UNSPECIFIED.);
#23710=B_SPLINE_CURVE_WITH_KNOTS('',2,(#82206,#82207,#82208),
 .UNSPECIFIED.,.F.,.F.,(3,3),(0.,1.),.UNSPECIFIED.);
#23711=B_SPLINE_CURVE_WITH_KNOTS('',2,(#82212,#82213,#82214),
 .UNSPECIFIED.,.F.,.F.,(3,3),(0.,1.),.UNSPECIFIED.);
#23712=B_SPLINE_CURVE_WITH_KNOTS('',2,(#82223,#82224,#82225),
 .UNSPECIFIED.,.F.,.F.,(3,3),(0.,1.),.UNSPECIFIED.);
#23713=B_SPLINE_CURVE_WITH_KNOTS('',2,(#82228,#82229,#82230),
 .UNSPECIFIED.,.F.,.F.,(3,3),(0.,1.),.UNSPECIFIED.);
#23714=B_SPLINE_CURVE_WITH_KNOTS('',2,(#82238,#82239,#82240),
 .UNSPECIFIED.,.F.,.F.,(3,3),(0.,1.),.UNSPECIFIED.);
#23715=B_SPLINE_CURVE_WITH_KNOTS('',2,(#82243,#82244,#82245),
 .UNSPECIFIED.,.F.,.F.,(3,3),(0.,1.),.UNSPECIFIED.);
#23716=B_SPLINE_CURVE_WITH_KNOTS('',2,(#82253,#82254,#82255),
 .UNSPECIFIED.,.F.,.F.,(3,3),(0.,1.),.UNSPECIFIED.);
#23717=B_SPLINE_CURVE_WITH_KNOTS('',2,(#82258,#82259,#82260),
 .UNSPECIFIED.,.F.,.F.,(3,3),(0.,1.),.UNSPECIFIED.);
#23718=B_SPLINE_CURVE_WITH_KNOTS('',2,(#82268,#82269,#82270),
 .UNSPECIFIED.,.F.,.F.,(3,3),(0.,1.),.UNSPECIFIED.);
#23719=B_SPLINE_CURVE_WITH_KNOTS('',2,(#82273,#82274,#82275),
 .UNSPECIFIED.,.F.,.F.,(3,3),(0.,1.),.UNSPECIFIED.);
#23720=B_SPLINE_CURVE_WITH_KNOTS('',2,(#82283,#82284,#82285),
 .UNSPECIFIED.,.F.,.F.,(3,3),(0.,1.),.UNSPECIFIED.);
#23721=B_SPLINE_CURVE_WITH_KNOTS('',2,(#82288,#82289,#82290),
 .UNSPECIFIED.,.F.,.F.,(3,3),(0.,1.),.UNSPECIFIED.);
#23722=B_SPLINE_CURVE_WITH_KNOTS('',2,(#82298,#82299,#82300),
 .UNSPECIFIED.,.F.,.F.,(3,3),(0.,1.),.UNSPECIFIED.);
#23723=B_SPLINE_CURVE_WITH_KNOTS('',2,(#82303,#82304,#82305),
 .UNSPECIFIED.,.F.,.F.,(3,3),(0.,1.),.UNSPECIFIED.);
#23724=B_SPLINE_CURVE_WITH_KNOTS('',2,(#82312,#82313,#82314),
 .UNSPECIFIED.,.F.,.F.,(3,3),(0.,1.),.UNSPECIFIED.);
#23725=B_SPLINE_CURVE_WITH_KNOTS('',2,(#82315,#82316,#82317),
 .UNSPECIFIED.,.F.,.F.,(3,3),(0.,1.),.UNSPECIFIED.);
#23726=B_SPLINE_CURVE_WITH_KNOTS('',2,(#82326,#82327,#82328),
 .UNSPECIFIED.,.F.,.F.,(3,3),(0.,1.),.UNSPECIFIED.);
#23727=B_SPLINE_CURVE_WITH_KNOTS('',2,(#82332,#82333,#82334),
 .UNSPECIFIED.,.F.,.F.,(3,3),(0.,1.),.UNSPECIFIED.);
#23728=B_SPLINE_CURVE_WITH_KNOTS('',2,(#82343,#82344,#82345),
 .UNSPECIFIED.,.F.,.F.,(3,3),(0.,1.),.UNSPECIFIED.);
#23729=B_SPLINE_CURVE_WITH_KNOTS('',2,(#82348,#82349,#82350),
 .UNSPECIFIED.,.F.,.F.,(3,3),(0.,1.),.UNSPECIFIED.);
#23730=B_SPLINE_CURVE_WITH_KNOTS('',2,(#82358,#82359,#82360),
 .UNSPECIFIED.,.F.,.F.,(3,3),(0.,1.),.UNSPECIFIED.);
#23731=B_SPLINE_CURVE_WITH_KNOTS('',2,(#82363,#82364,#82365),
 .UNSPECIFIED.,.F.,.F.,(3,3),(0.,1.),.UNSPECIFIED.);
#23732=B_SPLINE_CURVE_WITH_KNOTS('',2,(#82373,#82374,#82375),
 .UNSPECIFIED.,.F.,.F.,(3,3),(0.,1.),.UNSPECIFIED.);
#23733=B_SPLINE_CURVE_WITH_KNOTS('',2,(#82378,#82379,#82380),
 .UNSPECIFIED.,.F.,.F.,(3,3),(0.,1.),.UNSPECIFIED.);
#23734=B_SPLINE_CURVE_WITH_KNOTS('',2,(#82388,#82389,#82390),
 .UNSPECIFIED.,.F.,.F.,(3,3),(0.,1.),.UNSPECIFIED.);
#23735=B_SPLINE_CURVE_WITH_KNOTS('',2,(#82393,#82394,#82395),
 .UNSPECIFIED.,.F.,.F.,(3,3),(0.,1.),.UNSPECIFIED.);
#23736=B_SPLINE_CURVE_WITH_KNOTS('',2,(#82403,#82404,#82405),
 .UNSPECIFIED.,.F.,.F.,(3,3),(0.,1.),.UNSPECIFIED.);
#23737=B_SPLINE_CURVE_WITH_KNOTS('',2,(#82408,#82409,#82410),
 .UNSPECIFIED.,.F.,.F.,(3,3),(0.,1.),.UNSPECIFIED.);
#23738=B_SPLINE_CURVE_WITH_KNOTS('',2,(#82418,#82419,#82420),
 .UNSPECIFIED.,.F.,.F.,(3,3),(0.,1.),.UNSPECIFIED.);
#23739=B_SPLINE_CURVE_WITH_KNOTS('',2,(#82423,#82424,#82425),
 .UNSPECIFIED.,.F.,.F.,(3,3),(0.,1.),.UNSPECIFIED.);
#23740=B_SPLINE_CURVE_WITH_KNOTS('',2,(#82433,#82434,#82435),
 .UNSPECIFIED.,.F.,.F.,(3,3),(0.,1.),.UNSPECIFIED.);
#23741=B_SPLINE_CURVE_WITH_KNOTS('',2,(#82438,#82439,#82440),
 .UNSPECIFIED.,.F.,.F.,(3,3),(0.,1.),.UNSPECIFIED.);
#23742=B_SPLINE_CURVE_WITH_KNOTS('',2,(#82448,#82449,#82450),
 .UNSPECIFIED.,.F.,.F.,(3,3),(0.,1.),.UNSPECIFIED.);
#23743=B_SPLINE_CURVE_WITH_KNOTS('',2,(#82453,#82454,#82455),
 .UNSPECIFIED.,.F.,.F.,(3,3),(0.,1.),.UNSPECIFIED.);
#23744=B_SPLINE_CURVE_WITH_KNOTS('',2,(#82463,#82464,#82465),
 .UNSPECIFIED.,.F.,.F.,(3,3),(0.,1.),.UNSPECIFIED.);
#23745=B_SPLINE_CURVE_WITH_KNOTS('',2,(#82468,#82469,#82470),
 .UNSPECIFIED.,.F.,.F.,(3,3),(0.,1.),.UNSPECIFIED.);
#23746=B_SPLINE_CURVE_WITH_KNOTS('',2,(#82478,#82479,#82480),
 .UNSPECIFIED.,.F.,.F.,(3,3),(0.,1.),.UNSPECIFIED.);
#23747=B_SPLINE_CURVE_WITH_KNOTS('',2,(#82483,#82484,#82485),
 .UNSPECIFIED.,.F.,.F.,(3,3),(0.,1.),.UNSPECIFIED.);
#23748=B_SPLINE_CURVE_WITH_KNOTS('',2,(#82492,#82493,#82494),
 .UNSPECIFIED.,.F.,.F.,(3,3),(0.,1.),.UNSPECIFIED.);
#23749=B_SPLINE_CURVE_WITH_KNOTS('',2,(#82495,#82496,#82497),
 .UNSPECIFIED.,.F.,.F.,(3,3),(0.,1.),.UNSPECIFIED.);
#23750=B_SPLINE_CURVE_WITH_KNOTS('',2,(#82507,#82508,#82509),
 .UNSPECIFIED.,.F.,.F.,(3,3),(0.,1.),.UNSPECIFIED.);
#23751=B_SPLINE_CURVE_WITH_KNOTS('',2,(#82513,#82514,#82515),
 .UNSPECIFIED.,.F.,.F.,(3,3),(0.,1.),.UNSPECIFIED.);
#23752=B_SPLINE_CURVE_WITH_KNOTS('',2,(#82524,#82525,#82526),
 .UNSPECIFIED.,.F.,.F.,(3,3),(0.,1.),.UNSPECIFIED.);
#23753=B_SPLINE_CURVE_WITH_KNOTS('',2,(#82529,#82530,#82531),
 .UNSPECIFIED.,.F.,.F.,(3,3),(0.,1.),.UNSPECIFIED.);
#23754=B_SPLINE_CURVE_WITH_KNOTS('',2,(#82539,#82540,#82541),
 .UNSPECIFIED.,.F.,.F.,(3,3),(0.,1.),.UNSPECIFIED.);
#23755=B_SPLINE_CURVE_WITH_KNOTS('',2,(#82544,#82545,#82546),
 .UNSPECIFIED.,.F.,.F.,(3,3),(0.,1.),.UNSPECIFIED.);
#23756=B_SPLINE_CURVE_WITH_KNOTS('',2,(#82554,#82555,#82556),
 .UNSPECIFIED.,.F.,.F.,(3,3),(0.,1.),.UNSPECIFIED.);
#23757=B_SPLINE_CURVE_WITH_KNOTS('',2,(#82559,#82560,#82561),
 .UNSPECIFIED.,.F.,.F.,(3,3),(0.,1.),.UNSPECIFIED.);
#23758=B_SPLINE_CURVE_WITH_KNOTS('',2,(#82569,#82570,#82571),
 .UNSPECIFIED.,.F.,.F.,(3,3),(0.,1.),.UNSPECIFIED.);
#23759=B_SPLINE_CURVE_WITH_KNOTS('',2,(#82574,#82575,#82576),
 .UNSPECIFIED.,.F.,.F.,(3,3),(0.,1.),.UNSPECIFIED.);
#23760=B_SPLINE_CURVE_WITH_KNOTS('',2,(#82584,#82585,#82586),
 .UNSPECIFIED.,.F.,.F.,(3,3),(0.,1.),.UNSPECIFIED.);
#23761=B_SPLINE_CURVE_WITH_KNOTS('',2,(#82589,#82590,#82591),
 .UNSPECIFIED.,.F.,.F.,(3,3),(0.,1.),.UNSPECIFIED.);
#23762=B_SPLINE_CURVE_WITH_KNOTS('',2,(#82599,#82600,#82601),
 .UNSPECIFIED.,.F.,.F.,(3,3),(0.,1.),.UNSPECIFIED.);
#23763=B_SPLINE_CURVE_WITH_KNOTS('',2,(#82604,#82605,#82606),
 .UNSPECIFIED.,.F.,.F.,(3,3),(0.,1.),.UNSPECIFIED.);
#23764=B_SPLINE_CURVE_WITH_KNOTS('',2,(#82614,#82615,#82616),
 .UNSPECIFIED.,.F.,.F.,(3,3),(0.,1.),.UNSPECIFIED.);
#23765=B_SPLINE_CURVE_WITH_KNOTS('',2,(#82619,#82620,#82621),
 .UNSPECIFIED.,.F.,.F.,(3,3),(0.,1.),.UNSPECIFIED.);
#23766=B_SPLINE_CURVE_WITH_KNOTS('',2,(#82629,#82630,#82631),
 .UNSPECIFIED.,.F.,.F.,(3,3),(0.,1.),.UNSPECIFIED.);
#23767=B_SPLINE_CURVE_WITH_KNOTS('',2,(#82634,#82635,#82636),
 .UNSPECIFIED.,.F.,.F.,(3,3),(0.,1.),.UNSPECIFIED.);
#23768=B_SPLINE_CURVE_WITH_KNOTS('',2,(#82650,#82651,#82652),
 .UNSPECIFIED.,.F.,.F.,(3,3),(0.,1.),.UNSPECIFIED.);
#23769=B_SPLINE_CURVE_WITH_KNOTS('',2,(#82655,#82656,#82657),
 .UNSPECIFIED.,.F.,.F.,(3,3),(0.,1.),.UNSPECIFIED.);
#23770=B_SPLINE_CURVE_WITH_KNOTS('',2,(#82665,#82666,#82667),
 .UNSPECIFIED.,.F.,.F.,(3,3),(0.,1.),.UNSPECIFIED.);
#23771=B_SPLINE_CURVE_WITH_KNOTS('',2,(#82670,#82671,#82672),
 .UNSPECIFIED.,.F.,.F.,(3,3),(0.,1.),.UNSPECIFIED.);
#23772=B_SPLINE_CURVE_WITH_KNOTS('',2,(#82680,#82681,#82682),
 .UNSPECIFIED.,.F.,.F.,(3,3),(0.,1.),.UNSPECIFIED.);
#23773=B_SPLINE_CURVE_WITH_KNOTS('',2,(#82685,#82686,#82687),
 .UNSPECIFIED.,.F.,.F.,(3,3),(0.,1.),.UNSPECIFIED.);
#23774=B_SPLINE_CURVE_WITH_KNOTS('',2,(#82695,#82696,#82697),
 .UNSPECIFIED.,.F.,.F.,(3,3),(0.,1.),.UNSPECIFIED.);
#23775=B_SPLINE_CURVE_WITH_KNOTS('',2,(#82700,#82701,#82702),
 .UNSPECIFIED.,.F.,.F.,(3,3),(0.,1.),.UNSPECIFIED.);
#23776=B_SPLINE_CURVE_WITH_KNOTS('',2,(#82710,#82711,#82712),
 .UNSPECIFIED.,.F.,.F.,(3,3),(0.,1.),.UNSPECIFIED.);
#23777=B_SPLINE_CURVE_WITH_KNOTS('',2,(#82715,#82716,#82717),
 .UNSPECIFIED.,.F.,.F.,(3,3),(0.,1.),.UNSPECIFIED.);
#23778=B_SPLINE_CURVE_WITH_KNOTS('',2,(#82725,#82726,#82727),
 .UNSPECIFIED.,.F.,.F.,(3,3),(0.,1.),.UNSPECIFIED.);
#23779=B_SPLINE_CURVE_WITH_KNOTS('',2,(#82730,#82731,#82732),
 .UNSPECIFIED.,.F.,.F.,(3,3),(0.,1.),.UNSPECIFIED.);
#23780=B_SPLINE_CURVE_WITH_KNOTS('',2,(#82740,#82741,#82742),
 .UNSPECIFIED.,.F.,.F.,(3,3),(0.,1.),.UNSPECIFIED.);
#23781=B_SPLINE_CURVE_WITH_KNOTS('',2,(#82745,#82746,#82747),
 .UNSPECIFIED.,.F.,.F.,(3,3),(0.,1.),.UNSPECIFIED.);
#23782=B_SPLINE_CURVE_WITH_KNOTS('',2,(#82755,#82756,#82757),
 .UNSPECIFIED.,.F.,.F.,(3,3),(0.,1.),.UNSPECIFIED.);
#23783=B_SPLINE_CURVE_WITH_KNOTS('',2,(#82760,#82761,#82762),
 .UNSPECIFIED.,.F.,.F.,(3,3),(0.,1.),.UNSPECIFIED.);
#23784=B_SPLINE_CURVE_WITH_KNOTS('',2,(#82770,#82771,#82772),
 .UNSPECIFIED.,.F.,.F.,(3,3),(0.,1.),.UNSPECIFIED.);
#23785=B_SPLINE_CURVE_WITH_KNOTS('',2,(#82775,#82776,#82777),
 .UNSPECIFIED.,.F.,.F.,(3,3),(0.,1.),.UNSPECIFIED.);
#23786=B_SPLINE_CURVE_WITH_KNOTS('',2,(#82803,#82804,#82805),
 .UNSPECIFIED.,.F.,.F.,(3,3),(0.,1.),.UNSPECIFIED.);
#23787=B_SPLINE_CURVE_WITH_KNOTS('',2,(#82809,#82810,#82811),
 .UNSPECIFIED.,.F.,.F.,(3,3),(0.,1.),.UNSPECIFIED.);
#23788=B_SPLINE_CURVE_WITH_KNOTS('',2,(#82820,#82821,#82822),
 .UNSPECIFIED.,.F.,.F.,(3,3),(0.,1.),.UNSPECIFIED.);
#23789=B_SPLINE_CURVE_WITH_KNOTS('',2,(#82825,#82826,#82827),
 .UNSPECIFIED.,.F.,.F.,(3,3),(0.,1.),.UNSPECIFIED.);
#23790=B_SPLINE_CURVE_WITH_KNOTS('',2,(#82835,#82836,#82837),
 .UNSPECIFIED.,.F.,.F.,(3,3),(0.,1.),.UNSPECIFIED.);
#23791=B_SPLINE_CURVE_WITH_KNOTS('',2,(#82840,#82841,#82842),
 .UNSPECIFIED.,.F.,.F.,(3,3),(0.,1.),.UNSPECIFIED.);
#23792=B_SPLINE_CURVE_WITH_KNOTS('',2,(#82850,#82851,#82852),
 .UNSPECIFIED.,.F.,.F.,(3,3),(0.,1.),.UNSPECIFIED.);
#23793=B_SPLINE_CURVE_WITH_KNOTS('',2,(#82855,#82856,#82857),
 .UNSPECIFIED.,.F.,.F.,(3,3),(0.,1.),.UNSPECIFIED.);
#23794=B_SPLINE_CURVE_WITH_KNOTS('',2,(#82865,#82866,#82867),
 .UNSPECIFIED.,.F.,.F.,(3,3),(0.,1.),.UNSPECIFIED.);
#23795=B_SPLINE_CURVE_WITH_KNOTS('',2,(#82870,#82871,#82872),
 .UNSPECIFIED.,.F.,.F.,(3,3),(0.,1.),.UNSPECIFIED.);
#23796=B_SPLINE_CURVE_WITH_KNOTS('',2,(#82880,#82881,#82882),
 .UNSPECIFIED.,.F.,.F.,(3,3),(0.,1.),.UNSPECIFIED.);
#23797=B_SPLINE_CURVE_WITH_KNOTS('',2,(#82885,#82886,#82887),
 .UNSPECIFIED.,.F.,.F.,(3,3),(0.,1.),.UNSPECIFIED.);
#23798=B_SPLINE_CURVE_WITH_KNOTS('',2,(#82895,#82896,#82897),
 .UNSPECIFIED.,.F.,.F.,(3,3),(0.,1.),.UNSPECIFIED.);
#23799=B_SPLINE_CURVE_WITH_KNOTS('',2,(#82900,#82901,#82902),
 .UNSPECIFIED.,.F.,.F.,(3,3),(0.,1.),.UNSPECIFIED.);
#23800=B_SPLINE_CURVE_WITH_KNOTS('',2,(#82909,#82910,#82911),
 .UNSPECIFIED.,.F.,.F.,(3,3),(0.,1.),.UNSPECIFIED.);
#23801=B_SPLINE_CURVE_WITH_KNOTS('',2,(#82912,#82913,#82914),
 .UNSPECIFIED.,.F.,.F.,(3,3),(0.,1.),.UNSPECIFIED.);
#23802=B_SPLINE_CURVE_WITH_KNOTS('',2,(#82923,#82924,#82925),
 .UNSPECIFIED.,.F.,.F.,(3,3),(0.,1.),.UNSPECIFIED.);
#23803=B_SPLINE_CURVE_WITH_KNOTS('',2,(#82929,#82930,#82931),
 .UNSPECIFIED.,.F.,.F.,(3,3),(0.,1.),.UNSPECIFIED.);
#23804=B_SPLINE_CURVE_WITH_KNOTS('',2,(#82940,#82941,#82942),
 .UNSPECIFIED.,.F.,.F.,(3,3),(0.,1.),.UNSPECIFIED.);
#23805=B_SPLINE_CURVE_WITH_KNOTS('',2,(#82945,#82946,#82947),
 .UNSPECIFIED.,.F.,.F.,(3,3),(0.,1.),.UNSPECIFIED.);
#23806=B_SPLINE_CURVE_WITH_KNOTS('',2,(#82955,#82956,#82957),
 .UNSPECIFIED.,.F.,.F.,(3,3),(0.,1.),.UNSPECIFIED.);
#23807=B_SPLINE_CURVE_WITH_KNOTS('',2,(#82960,#82961,#82962),
 .UNSPECIFIED.,.F.,.F.,(3,3),(0.,1.),.UNSPECIFIED.);
#23808=B_SPLINE_CURVE_WITH_KNOTS('',2,(#82970,#82971,#82972),
 .UNSPECIFIED.,.F.,.F.,(3,3),(0.,1.),.UNSPECIFIED.);
#23809=B_SPLINE_CURVE_WITH_KNOTS('',2,(#82975,#82976,#82977),
 .UNSPECIFIED.,.F.,.F.,(3,3),(0.,1.),.UNSPECIFIED.);
#23810=B_SPLINE_CURVE_WITH_KNOTS('',2,(#82985,#82986,#82987),
 .UNSPECIFIED.,.F.,.F.,(3,3),(0.,1.),.UNSPECIFIED.);
#23811=B_SPLINE_CURVE_WITH_KNOTS('',2,(#82990,#82991,#82992),
 .UNSPECIFIED.,.F.,.F.,(3,3),(0.,1.),.UNSPECIFIED.);
#23812=B_SPLINE_CURVE_WITH_KNOTS('',2,(#83000,#83001,#83002),
 .UNSPECIFIED.,.F.,.F.,(3,3),(0.,1.),.UNSPECIFIED.);
#23813=B_SPLINE_CURVE_WITH_KNOTS('',2,(#83005,#83006,#83007),
 .UNSPECIFIED.,.F.,.F.,(3,3),(0.,1.),.UNSPECIFIED.);
#23814=B_SPLINE_CURVE_WITH_KNOTS('',2,(#83015,#83016,#83017),
 .UNSPECIFIED.,.F.,.F.,(3,3),(0.,1.),.UNSPECIFIED.);
#23815=B_SPLINE_CURVE_WITH_KNOTS('',2,(#83020,#83021,#83022),
 .UNSPECIFIED.,.F.,.F.,(3,3),(0.,1.),.UNSPECIFIED.);
#23816=B_SPLINE_CURVE_WITH_KNOTS('',2,(#83030,#83031,#83032),
 .UNSPECIFIED.,.F.,.F.,(3,3),(0.,1.),.UNSPECIFIED.);
#23817=B_SPLINE_CURVE_WITH_KNOTS('',2,(#83035,#83036,#83037),
 .UNSPECIFIED.,.F.,.F.,(3,3),(0.,1.),.UNSPECIFIED.);
#23818=B_SPLINE_CURVE_WITH_KNOTS('',2,(#83045,#83046,#83047),
 .UNSPECIFIED.,.F.,.F.,(3,3),(0.,1.),.UNSPECIFIED.);
#23819=B_SPLINE_CURVE_WITH_KNOTS('',2,(#83050,#83051,#83052),
 .UNSPECIFIED.,.F.,.F.,(3,3),(0.,1.),.UNSPECIFIED.);
#23820=B_SPLINE_CURVE_WITH_KNOTS('',2,(#83060,#83061,#83062),
 .UNSPECIFIED.,.F.,.F.,(3,3),(0.,1.),.UNSPECIFIED.);
#23821=B_SPLINE_CURVE_WITH_KNOTS('',2,(#83065,#83066,#83067),
 .UNSPECIFIED.,.F.,.F.,(3,3),(0.,1.),.UNSPECIFIED.);
#23822=B_SPLINE_CURVE_WITH_KNOTS('',2,(#83075,#83076,#83077),
 .UNSPECIFIED.,.F.,.F.,(3,3),(0.,1.),.UNSPECIFIED.);
#23823=B_SPLINE_CURVE_WITH_KNOTS('',2,(#83080,#83081,#83082),
 .UNSPECIFIED.,.F.,.F.,(3,3),(0.,1.),.UNSPECIFIED.);
#23824=B_SPLINE_CURVE_WITH_KNOTS('',2,(#83089,#83090,#83091),
 .UNSPECIFIED.,.F.,.F.,(3,3),(0.,1.),.UNSPECIFIED.);
#23825=B_SPLINE_CURVE_WITH_KNOTS('',2,(#83092,#83093,#83094),
 .UNSPECIFIED.,.F.,.F.,(3,3),(0.,1.),.UNSPECIFIED.);
#23826=B_SPLINE_CURVE_WITH_KNOTS('',2,(#83104,#83105,#83106),
 .UNSPECIFIED.,.F.,.F.,(3,3),(0.,1.),.UNSPECIFIED.);
#23827=B_SPLINE_CURVE_WITH_KNOTS('',2,(#83110,#83111,#83112),
 .UNSPECIFIED.,.F.,.F.,(3,3),(0.,1.),.UNSPECIFIED.);
#23828=B_SPLINE_CURVE_WITH_KNOTS('',2,(#83121,#83122,#83123),
 .UNSPECIFIED.,.F.,.F.,(3,3),(0.,1.),.UNSPECIFIED.);
#23829=B_SPLINE_CURVE_WITH_KNOTS('',2,(#83126,#83127,#83128),
 .UNSPECIFIED.,.F.,.F.,(3,3),(0.,1.),.UNSPECIFIED.);
#23830=B_SPLINE_CURVE_WITH_KNOTS('',2,(#83136,#83137,#83138),
 .UNSPECIFIED.,.F.,.F.,(3,3),(0.,1.),.UNSPECIFIED.);
#23831=B_SPLINE_CURVE_WITH_KNOTS('',2,(#83141,#83142,#83143),
 .UNSPECIFIED.,.F.,.F.,(3,3),(0.,1.),.UNSPECIFIED.);
#23832=B_SPLINE_CURVE_WITH_KNOTS('',2,(#83151,#83152,#83153),
 .UNSPECIFIED.,.F.,.F.,(3,3),(0.,1.),.UNSPECIFIED.);
#23833=B_SPLINE_CURVE_WITH_KNOTS('',2,(#83156,#83157,#83158),
 .UNSPECIFIED.,.F.,.F.,(3,3),(0.,1.),.UNSPECIFIED.);
#23834=B_SPLINE_CURVE_WITH_KNOTS('',2,(#83166,#83167,#83168),
 .UNSPECIFIED.,.F.,.F.,(3,3),(0.,1.),.UNSPECIFIED.);
#23835=B_SPLINE_CURVE_WITH_KNOTS('',2,(#83171,#83172,#83173),
 .UNSPECIFIED.,.F.,.F.,(3,3),(0.,1.),.UNSPECIFIED.);
#23836=B_SPLINE_CURVE_WITH_KNOTS('',2,(#83181,#83182,#83183),
 .UNSPECIFIED.,.F.,.F.,(3,3),(0.,1.),.UNSPECIFIED.);
#23837=B_SPLINE_CURVE_WITH_KNOTS('',2,(#83186,#83187,#83188),
 .UNSPECIFIED.,.F.,.F.,(3,3),(0.,1.),.UNSPECIFIED.);
#23838=B_SPLINE_CURVE_WITH_KNOTS('',2,(#83196,#83197,#83198),
 .UNSPECIFIED.,.F.,.F.,(3,3),(0.,1.),.UNSPECIFIED.);
#23839=B_SPLINE_CURVE_WITH_KNOTS('',2,(#83201,#83202,#83203),
 .UNSPECIFIED.,.F.,.F.,(3,3),(0.,1.),.UNSPECIFIED.);
#23840=B_SPLINE_CURVE_WITH_KNOTS('',2,(#83211,#83212,#83213),
 .UNSPECIFIED.,.F.,.F.,(3,3),(0.,1.),.UNSPECIFIED.);
#23841=B_SPLINE_CURVE_WITH_KNOTS('',2,(#83216,#83217,#83218),
 .UNSPECIFIED.,.F.,.F.,(3,3),(0.,1.),.UNSPECIFIED.);
#23842=B_SPLINE_CURVE_WITH_KNOTS('',2,(#83226,#83227,#83228),
 .UNSPECIFIED.,.F.,.F.,(3,3),(0.,1.),.UNSPECIFIED.);
#23843=B_SPLINE_CURVE_WITH_KNOTS('',2,(#83231,#83232,#83233),
 .UNSPECIFIED.,.F.,.F.,(3,3),(0.,1.),.UNSPECIFIED.);
#23844=B_SPLINE_CURVE_WITH_KNOTS('',2,(#83241,#83242,#83243),
 .UNSPECIFIED.,.F.,.F.,(3,3),(0.,1.),.UNSPECIFIED.);
#23845=B_SPLINE_CURVE_WITH_KNOTS('',2,(#83246,#83247,#83248),
 .UNSPECIFIED.,.F.,.F.,(3,3),(0.,1.),.UNSPECIFIED.);
#23846=B_SPLINE_CURVE_WITH_KNOTS('',2,(#83256,#83257,#83258),
 .UNSPECIFIED.,.F.,.F.,(3,3),(0.,1.),.UNSPECIFIED.);
#23847=B_SPLINE_CURVE_WITH_KNOTS('',2,(#83261,#83262,#83263),
 .UNSPECIFIED.,.F.,.F.,(3,3),(0.,1.),.UNSPECIFIED.);
#23848=B_SPLINE_CURVE_WITH_KNOTS('',2,(#83271,#83272,#83273),
 .UNSPECIFIED.,.F.,.F.,(3,3),(0.,1.),.UNSPECIFIED.);
#23849=B_SPLINE_CURVE_WITH_KNOTS('',2,(#83276,#83277,#83278),
 .UNSPECIFIED.,.F.,.F.,(3,3),(0.,1.),.UNSPECIFIED.);
#23850=B_SPLINE_CURVE_WITH_KNOTS('',2,(#83292,#83293,#83294),
 .UNSPECIFIED.,.F.,.F.,(3,3),(0.,1.),.UNSPECIFIED.);
#23851=B_SPLINE_CURVE_WITH_KNOTS('',2,(#83297,#83298,#83299),
 .UNSPECIFIED.,.F.,.F.,(3,3),(0.,1.),.UNSPECIFIED.);
#23852=B_SPLINE_CURVE_WITH_KNOTS('',2,(#83307,#83308,#83309),
 .UNSPECIFIED.,.F.,.F.,(3,3),(0.,1.),.UNSPECIFIED.);
#23853=B_SPLINE_CURVE_WITH_KNOTS('',2,(#83312,#83313,#83314),
 .UNSPECIFIED.,.F.,.F.,(3,3),(0.,1.),.UNSPECIFIED.);
#23854=B_SPLINE_CURVE_WITH_KNOTS('',2,(#83322,#83323,#83324),
 .UNSPECIFIED.,.F.,.F.,(3,3),(0.,1.),.UNSPECIFIED.);
#23855=B_SPLINE_CURVE_WITH_KNOTS('',2,(#83327,#83328,#83329),
 .UNSPECIFIED.,.F.,.F.,(3,3),(0.,1.),.UNSPECIFIED.);
#23856=B_SPLINE_CURVE_WITH_KNOTS('',2,(#83337,#83338,#83339),
 .UNSPECIFIED.,.F.,.F.,(3,3),(0.,1.),.UNSPECIFIED.);
#23857=B_SPLINE_CURVE_WITH_KNOTS('',2,(#83342,#83343,#83344),
 .UNSPECIFIED.,.F.,.F.,(3,3),(0.,1.),.UNSPECIFIED.);
#23858=B_SPLINE_CURVE_WITH_KNOTS('',2,(#83352,#83353,#83354),
 .UNSPECIFIED.,.F.,.F.,(3,3),(0.,1.),.UNSPECIFIED.);
#23859=B_SPLINE_CURVE_WITH_KNOTS('',2,(#83357,#83358,#83359),
 .UNSPECIFIED.,.F.,.F.,(3,3),(0.,1.),.UNSPECIFIED.);
#23860=B_SPLINE_CURVE_WITH_KNOTS('',2,(#83367,#83368,#83369),
 .UNSPECIFIED.,.F.,.F.,(3,3),(0.,1.),.UNSPECIFIED.);
#23861=B_SPLINE_CURVE_WITH_KNOTS('',2,(#83372,#83373,#83374),
 .UNSPECIFIED.,.F.,.F.,(3,3),(0.,1.),.UNSPECIFIED.);
#23862=B_SPLINE_CURVE_WITH_KNOTS('',2,(#83382,#83383,#83384),
 .UNSPECIFIED.,.F.,.F.,(3,3),(0.,1.),.UNSPECIFIED.);
#23863=B_SPLINE_CURVE_WITH_KNOTS('',2,(#83387,#83388,#83389),
 .UNSPECIFIED.,.F.,.F.,(3,3),(0.,1.),.UNSPECIFIED.);
#23864=B_SPLINE_CURVE_WITH_KNOTS('',2,(#83403,#83404,#83405),
 .UNSPECIFIED.,.F.,.F.,(3,3),(0.,1.),.UNSPECIFIED.);
#23865=B_SPLINE_CURVE_WITH_KNOTS('',2,(#83408,#83409,#83410),
 .UNSPECIFIED.,.F.,.F.,(3,3),(0.,1.),.UNSPECIFIED.);
#23866=B_SPLINE_CURVE_WITH_KNOTS('',2,(#83418,#83419,#83420),
 .UNSPECIFIED.,.F.,.F.,(3,3),(0.,1.),.UNSPECIFIED.);
#23867=B_SPLINE_CURVE_WITH_KNOTS('',2,(#83423,#83424,#83425),
 .UNSPECIFIED.,.F.,.F.,(3,3),(0.,1.),.UNSPECIFIED.);
#23868=B_SPLINE_CURVE_WITH_KNOTS('',2,(#83433,#83434,#83435),
 .UNSPECIFIED.,.F.,.F.,(3,3),(0.,1.),.UNSPECIFIED.);
#23869=B_SPLINE_CURVE_WITH_KNOTS('',2,(#83438,#83439,#83440),
 .UNSPECIFIED.,.F.,.F.,(3,3),(0.,1.),.UNSPECIFIED.);
#23870=B_SPLINE_CURVE_WITH_KNOTS('',2,(#83448,#83449,#83450),
 .UNSPECIFIED.,.F.,.F.,(3,3),(0.,1.),.UNSPECIFIED.);
#23871=B_SPLINE_CURVE_WITH_KNOTS('',2,(#83453,#83454,#83455),
 .UNSPECIFIED.,.F.,.F.,(3,3),(0.,1.),.UNSPECIFIED.);
#23872=B_SPLINE_CURVE_WITH_KNOTS('',2,(#83463,#83464,#83465),
 .UNSPECIFIED.,.F.,.F.,(3,3),(0.,1.),.UNSPECIFIED.);
#23873=B_SPLINE_CURVE_WITH_KNOTS('',2,(#83468,#83469,#83470),
 .UNSPECIFIED.,.F.,.F.,(3,3),(0.,1.),.UNSPECIFIED.);
#23874=B_SPLINE_CURVE_WITH_KNOTS('',2,(#83478,#83479,#83480),
 .UNSPECIFIED.,.F.,.F.,(3,3),(0.,1.),.UNSPECIFIED.);
#23875=B_SPLINE_CURVE_WITH_KNOTS('',2,(#83483,#83484,#83485),
 .UNSPECIFIED.,.F.,.F.,(3,3),(0.,1.),.UNSPECIFIED.);
#23876=B_SPLINE_CURVE_WITH_KNOTS('',2,(#83493,#83494,#83495),
 .UNSPECIFIED.,.F.,.F.,(3,3),(0.,1.),.UNSPECIFIED.);
#23877=B_SPLINE_CURVE_WITH_KNOTS('',2,(#83498,#83499,#83500),
 .UNSPECIFIED.,.F.,.F.,(3,3),(0.,1.),.UNSPECIFIED.);
#23878=B_SPLINE_CURVE_WITH_KNOTS('',2,(#83513,#83514,#83515),
 .UNSPECIFIED.,.F.,.F.,(3,3),(0.,1.),.UNSPECIFIED.);
#23879=B_SPLINE_CURVE_WITH_KNOTS('',2,(#83516,#83517,#83518),
 .UNSPECIFIED.,.F.,.F.,(3,3),(0.,1.),.UNSPECIFIED.);
#23880=B_SPLINE_CURVE_WITH_KNOTS('',2,(#83529,#83530,#83531),
 .UNSPECIFIED.,.F.,.F.,(3,3),(0.,1.),.UNSPECIFIED.);
#23881=B_SPLINE_CURVE_WITH_KNOTS('',2,(#83535,#83536,#83537),
 .UNSPECIFIED.,.F.,.F.,(3,3),(0.,1.),.UNSPECIFIED.);
#23882=B_SPLINE_CURVE_WITH_KNOTS('',2,(#83546,#83547,#83548),
 .UNSPECIFIED.,.F.,.F.,(3,3),(0.,1.),.UNSPECIFIED.);
#23883=B_SPLINE_CURVE_WITH_KNOTS('',2,(#83551,#83552,#83553),
 .UNSPECIFIED.,.F.,.F.,(3,3),(0.,1.),.UNSPECIFIED.);
#23884=B_SPLINE_CURVE_WITH_KNOTS('',2,(#83561,#83562,#83563),
 .UNSPECIFIED.,.F.,.F.,(3,3),(0.,1.),.UNSPECIFIED.);
#23885=B_SPLINE_CURVE_WITH_KNOTS('',2,(#83566,#83567,#83568),
 .UNSPECIFIED.,.F.,.F.,(3,3),(0.,1.),.UNSPECIFIED.);
#23886=B_SPLINE_CURVE_WITH_KNOTS('',2,(#83576,#83577,#83578),
 .UNSPECIFIED.,.F.,.F.,(3,3),(0.,1.),.UNSPECIFIED.);
#23887=B_SPLINE_CURVE_WITH_KNOTS('',2,(#83581,#83582,#83583),
 .UNSPECIFIED.,.F.,.F.,(3,3),(0.,1.),.UNSPECIFIED.);
#23888=B_SPLINE_CURVE_WITH_KNOTS('',2,(#83591,#83592,#83593),
 .UNSPECIFIED.,.F.,.F.,(3,3),(0.,1.),.UNSPECIFIED.);
#23889=B_SPLINE_CURVE_WITH_KNOTS('',2,(#83596,#83597,#83598),
 .UNSPECIFIED.,.F.,.F.,(3,3),(0.,1.),.UNSPECIFIED.);
#23890=B_SPLINE_CURVE_WITH_KNOTS('',2,(#83606,#83607,#83608),
 .UNSPECIFIED.,.F.,.F.,(3,3),(0.,1.),.UNSPECIFIED.);
#23891=B_SPLINE_CURVE_WITH_KNOTS('',2,(#83611,#83612,#83613),
 .UNSPECIFIED.,.F.,.F.,(3,3),(0.,1.),.UNSPECIFIED.);
#23892=B_SPLINE_CURVE_WITH_KNOTS('',2,(#83621,#83622,#83623),
 .UNSPECIFIED.,.F.,.F.,(3,3),(0.,1.),.UNSPECIFIED.);
#23893=B_SPLINE_CURVE_WITH_KNOTS('',2,(#83626,#83627,#83628),
 .UNSPECIFIED.,.F.,.F.,(3,3),(0.,1.),.UNSPECIFIED.);
#23894=B_SPLINE_CURVE_WITH_KNOTS('',2,(#83635,#83636,#83637),
 .UNSPECIFIED.,.F.,.F.,(3,3),(0.,1.),.UNSPECIFIED.);
#23895=B_SPLINE_CURVE_WITH_KNOTS('',2,(#83638,#83639,#83640),
 .UNSPECIFIED.,.F.,.F.,(3,3),(0.,1.),.UNSPECIFIED.);
#23896=B_SPLINE_CURVE_WITH_KNOTS('',2,(#83649,#83650,#83651),
 .UNSPECIFIED.,.F.,.F.,(3,3),(0.,1.),.UNSPECIFIED.);
#23897=B_SPLINE_CURVE_WITH_KNOTS('',2,(#83655,#83656,#83657),
 .UNSPECIFIED.,.F.,.F.,(3,3),(0.,1.),.UNSPECIFIED.);
#23898=B_SPLINE_CURVE_WITH_KNOTS('',2,(#83666,#83667,#83668),
 .UNSPECIFIED.,.F.,.F.,(3,3),(0.,1.),.UNSPECIFIED.);
#23899=B_SPLINE_CURVE_WITH_KNOTS('',2,(#83671,#83672,#83673),
 .UNSPECIFIED.,.F.,.F.,(3,3),(0.,1.),.UNSPECIFIED.);
#23900=B_SPLINE_CURVE_WITH_KNOTS('',2,(#83681,#83682,#83683),
 .UNSPECIFIED.,.F.,.F.,(3,3),(0.,1.),.UNSPECIFIED.);
#23901=B_SPLINE_CURVE_WITH_KNOTS('',2,(#83686,#83687,#83688),
 .UNSPECIFIED.,.F.,.F.,(3,3),(0.,1.),.UNSPECIFIED.);
#23902=B_SPLINE_CURVE_WITH_KNOTS('',2,(#83696,#83697,#83698),
 .UNSPECIFIED.,.F.,.F.,(3,3),(0.,1.),.UNSPECIFIED.);
#23903=B_SPLINE_CURVE_WITH_KNOTS('',2,(#83701,#83702,#83703),
 .UNSPECIFIED.,.F.,.F.,(3,3),(0.,1.),.UNSPECIFIED.);
#23904=B_SPLINE_CURVE_WITH_KNOTS('',2,(#83711,#83712,#83713),
 .UNSPECIFIED.,.F.,.F.,(3,3),(0.,1.),.UNSPECIFIED.);
#23905=B_SPLINE_CURVE_WITH_KNOTS('',2,(#83716,#83717,#83718),
 .UNSPECIFIED.,.F.,.F.,(3,3),(0.,1.),.UNSPECIFIED.);
#23906=B_SPLINE_CURVE_WITH_KNOTS('',2,(#83726,#83727,#83728),
 .UNSPECIFIED.,.F.,.F.,(3,3),(0.,1.),.UNSPECIFIED.);
#23907=B_SPLINE_CURVE_WITH_KNOTS('',2,(#83731,#83732,#83733),
 .UNSPECIFIED.,.F.,.F.,(3,3),(0.,1.),.UNSPECIFIED.);
#23908=B_SPLINE_CURVE_WITH_KNOTS('',2,(#83741,#83742,#83743),
 .UNSPECIFIED.,.F.,.F.,(3,3),(0.,1.),.UNSPECIFIED.);
#23909=B_SPLINE_CURVE_WITH_KNOTS('',2,(#83746,#83747,#83748),
 .UNSPECIFIED.,.F.,.F.,(3,3),(0.,1.),.UNSPECIFIED.);
#23910=B_SPLINE_CURVE_WITH_KNOTS('',2,(#83756,#83757,#83758),
 .UNSPECIFIED.,.F.,.F.,(3,3),(0.,1.),.UNSPECIFIED.);
#23911=B_SPLINE_CURVE_WITH_KNOTS('',2,(#83761,#83762,#83763),
 .UNSPECIFIED.,.F.,.F.,(3,3),(0.,1.),.UNSPECIFIED.);
#23912=B_SPLINE_CURVE_WITH_KNOTS('',2,(#83771,#83772,#83773),
 .UNSPECIFIED.,.F.,.F.,(3,3),(0.,1.),.UNSPECIFIED.);
#23913=B_SPLINE_CURVE_WITH_KNOTS('',2,(#83776,#83777,#83778),
 .UNSPECIFIED.,.F.,.F.,(3,3),(0.,1.),.UNSPECIFIED.);
#23914=B_SPLINE_CURVE_WITH_KNOTS('',2,(#83786,#83787,#83788),
 .UNSPECIFIED.,.F.,.F.,(3,3),(0.,1.),.UNSPECIFIED.);
#23915=B_SPLINE_CURVE_WITH_KNOTS('',2,(#83791,#83792,#83793),
 .UNSPECIFIED.,.F.,.F.,(3,3),(0.,1.),.UNSPECIFIED.);
#23916=B_SPLINE_CURVE_WITH_KNOTS('',2,(#83801,#83802,#83803),
 .UNSPECIFIED.,.F.,.F.,(3,3),(0.,1.),.UNSPECIFIED.);
#23917=B_SPLINE_CURVE_WITH_KNOTS('',2,(#83806,#83807,#83808),
 .UNSPECIFIED.,.F.,.F.,(3,3),(0.,1.),.UNSPECIFIED.);
#23918=B_SPLINE_CURVE_WITH_KNOTS('',2,(#83815,#83816,#83817),
 .UNSPECIFIED.,.F.,.F.,(3,3),(0.,1.),.UNSPECIFIED.);
#23919=B_SPLINE_CURVE_WITH_KNOTS('',2,(#83818,#83819,#83820),
 .UNSPECIFIED.,.F.,.F.,(3,3),(0.,1.),.UNSPECIFIED.);
#23920=B_SPLINE_CURVE_WITH_KNOTS('',2,(#83917,#83918,#83919),
 .UNSPECIFIED.,.F.,.F.,(3,3),(0.,1.),.UNSPECIFIED.);
#23921=B_SPLINE_CURVE_WITH_KNOTS('',2,(#83923,#83924,#83925),
 .UNSPECIFIED.,.F.,.F.,(3,3),(0.,1.),.UNSPECIFIED.);
#23922=B_SPLINE_CURVE_WITH_KNOTS('',2,(#83934,#83935,#83936),
 .UNSPECIFIED.,.F.,.F.,(3,3),(0.,1.),.UNSPECIFIED.);
#23923=B_SPLINE_CURVE_WITH_KNOTS('',2,(#83939,#83940,#83941),
 .UNSPECIFIED.,.F.,.F.,(3,3),(0.,1.),.UNSPECIFIED.);
#23924=B_SPLINE_CURVE_WITH_KNOTS('',2,(#83949,#83950,#83951),
 .UNSPECIFIED.,.F.,.F.,(3,3),(0.,1.),.UNSPECIFIED.);
#23925=B_SPLINE_CURVE_WITH_KNOTS('',2,(#83954,#83955,#83956),
 .UNSPECIFIED.,.F.,.F.,(3,3),(0.,1.),.UNSPECIFIED.);
#23926=B_SPLINE_CURVE_WITH_KNOTS('',2,(#83964,#83965,#83966),
 .UNSPECIFIED.,.F.,.F.,(3,3),(0.,1.),.UNSPECIFIED.);
#23927=B_SPLINE_CURVE_WITH_KNOTS('',2,(#83969,#83970,#83971),
 .UNSPECIFIED.,.F.,.F.,(3,3),(0.,1.),.UNSPECIFIED.);
#23928=B_SPLINE_CURVE_WITH_KNOTS('',2,(#83979,#83980,#83981),
 .UNSPECIFIED.,.F.,.F.,(3,3),(0.,1.),.UNSPECIFIED.);
#23929=B_SPLINE_CURVE_WITH_KNOTS('',2,(#83984,#83985,#83986),
 .UNSPECIFIED.,.F.,.F.,(3,3),(0.,1.),.UNSPECIFIED.);
#23930=B_SPLINE_CURVE_WITH_KNOTS('',2,(#83994,#83995,#83996),
 .UNSPECIFIED.,.F.,.F.,(3,3),(0.,1.),.UNSPECIFIED.);
#23931=B_SPLINE_CURVE_WITH_KNOTS('',2,(#83999,#84000,#84001),
 .UNSPECIFIED.,.F.,.F.,(3,3),(0.,1.),.UNSPECIFIED.);
#23932=B_SPLINE_CURVE_WITH_KNOTS('',2,(#84009,#84010,#84011),
 .UNSPECIFIED.,.F.,.F.,(3,3),(0.,1.),.UNSPECIFIED.);
#23933=B_SPLINE_CURVE_WITH_KNOTS('',2,(#84014,#84015,#84016),
 .UNSPECIFIED.,.F.,.F.,(3,3),(0.,1.),.UNSPECIFIED.);
#23934=B_SPLINE_CURVE_WITH_KNOTS('',2,(#84023,#84024,#84025),
 .UNSPECIFIED.,.F.,.F.,(3,3),(0.,1.),.UNSPECIFIED.);
#23935=B_SPLINE_CURVE_WITH_KNOTS('',2,(#84026,#84027,#84028),
 .UNSPECIFIED.,.F.,.F.,(3,3),(0.,1.),.UNSPECIFIED.);
#23936=B_SPLINE_CURVE_WITH_KNOTS('',2,(#84037,#84038,#84039),
 .UNSPECIFIED.,.F.,.F.,(3,3),(0.,1.),.UNSPECIFIED.);
#23937=B_SPLINE_CURVE_WITH_KNOTS('',2,(#84043,#84044,#84045),
 .UNSPECIFIED.,.F.,.F.,(3,3),(0.,1.),.UNSPECIFIED.);
#23938=B_SPLINE_CURVE_WITH_KNOTS('',2,(#84054,#84055,#84056),
 .UNSPECIFIED.,.F.,.F.,(3,3),(0.,1.),.UNSPECIFIED.);
#23939=B_SPLINE_CURVE_WITH_KNOTS('',2,(#84059,#84060,#84061),
 .UNSPECIFIED.,.F.,.F.,(3,3),(0.,1.),.UNSPECIFIED.);
#23940=B_SPLINE_CURVE_WITH_KNOTS('',2,(#84069,#84070,#84071),
 .UNSPECIFIED.,.F.,.F.,(3,3),(0.,1.),.UNSPECIFIED.);
#23941=B_SPLINE_CURVE_WITH_KNOTS('',2,(#84074,#84075,#84076),
 .UNSPECIFIED.,.F.,.F.,(3,3),(0.,1.),.UNSPECIFIED.);
#23942=B_SPLINE_CURVE_WITH_KNOTS('',2,(#84084,#84085,#84086),
 .UNSPECIFIED.,.F.,.F.,(3,3),(0.,1.),.UNSPECIFIED.);
#23943=B_SPLINE_CURVE_WITH_KNOTS('',2,(#84089,#84090,#84091),
 .UNSPECIFIED.,.F.,.F.,(3,3),(0.,1.),.UNSPECIFIED.);
#23944=B_SPLINE_CURVE_WITH_KNOTS('',2,(#84099,#84100,#84101),
 .UNSPECIFIED.,.F.,.F.,(3,3),(0.,1.),.UNSPECIFIED.);
#23945=B_SPLINE_CURVE_WITH_KNOTS('',2,(#84104,#84105,#84106),
 .UNSPECIFIED.,.F.,.F.,(3,3),(0.,1.),.UNSPECIFIED.);
#23946=B_SPLINE_CURVE_WITH_KNOTS('',2,(#84114,#84115,#84116),
 .UNSPECIFIED.,.F.,.F.,(3,3),(0.,1.),.UNSPECIFIED.);
#23947=B_SPLINE_CURVE_WITH_KNOTS('',2,(#84119,#84120,#84121),
 .UNSPECIFIED.,.F.,.F.,(3,3),(0.,1.),.UNSPECIFIED.);
#23948=B_SPLINE_CURVE_WITH_KNOTS('',2,(#84129,#84130,#84131),
 .UNSPECIFIED.,.F.,.F.,(3,3),(0.,1.),.UNSPECIFIED.);
#23949=B_SPLINE_CURVE_WITH_KNOTS('',2,(#84134,#84135,#84136),
 .UNSPECIFIED.,.F.,.F.,(3,3),(0.,1.),.UNSPECIFIED.);
#23950=B_SPLINE_CURVE_WITH_KNOTS('',2,(#84144,#84145,#84146),
 .UNSPECIFIED.,.F.,.F.,(3,3),(0.,1.),.UNSPECIFIED.);
#23951=B_SPLINE_CURVE_WITH_KNOTS('',2,(#84149,#84150,#84151),
 .UNSPECIFIED.,.F.,.F.,(3,3),(0.,1.),.UNSPECIFIED.);
#23952=B_SPLINE_CURVE_WITH_KNOTS('',2,(#84159,#84160,#84161),
 .UNSPECIFIED.,.F.,.F.,(3,3),(0.,1.),.UNSPECIFIED.);
#23953=B_SPLINE_CURVE_WITH_KNOTS('',2,(#84164,#84165,#84166),
 .UNSPECIFIED.,.F.,.F.,(3,3),(0.,1.),.UNSPECIFIED.);
#23954=B_SPLINE_CURVE_WITH_KNOTS('',2,(#84174,#84175,#84176),
 .UNSPECIFIED.,.F.,.F.,(3,3),(0.,1.),.UNSPECIFIED.);
#23955=B_SPLINE_CURVE_WITH_KNOTS('',2,(#84179,#84180,#84181),
 .UNSPECIFIED.,.F.,.F.,(3,3),(0.,1.),.UNSPECIFIED.);
#23956=B_SPLINE_CURVE_WITH_KNOTS('',2,(#84189,#84190,#84191),
 .UNSPECIFIED.,.F.,.F.,(3,3),(0.,1.),.UNSPECIFIED.);
#23957=B_SPLINE_CURVE_WITH_KNOTS('',2,(#84194,#84195,#84196),
 .UNSPECIFIED.,.F.,.F.,(3,3),(0.,1.),.UNSPECIFIED.);
#23958=B_SPLINE_CURVE_WITH_KNOTS('',2,(#84203,#84204,#84205),
 .UNSPECIFIED.,.F.,.F.,(3,3),(0.,1.),.UNSPECIFIED.);
#23959=B_SPLINE_CURVE_WITH_KNOTS('',2,(#84206,#84207,#84208),
 .UNSPECIFIED.,.F.,.F.,(3,3),(0.,1.),.UNSPECIFIED.);
#23960=B_SPLINE_CURVE_WITH_KNOTS('',2,(#84218,#84219,#84220),
 .UNSPECIFIED.,.F.,.F.,(3,3),(0.,1.),.UNSPECIFIED.);
#23961=B_SPLINE_CURVE_WITH_KNOTS('',2,(#84224,#84225,#84226),
 .UNSPECIFIED.,.F.,.F.,(3,3),(0.,1.),.UNSPECIFIED.);
#23962=B_SPLINE_CURVE_WITH_KNOTS('',2,(#84235,#84236,#84237),
 .UNSPECIFIED.,.F.,.F.,(3,3),(0.,1.),.UNSPECIFIED.);
#23963=B_SPLINE_CURVE_WITH_KNOTS('',2,(#84240,#84241,#84242),
 .UNSPECIFIED.,.F.,.F.,(3,3),(0.,1.),.UNSPECIFIED.);
#23964=B_SPLINE_CURVE_WITH_KNOTS('',2,(#84250,#84251,#84252),
 .UNSPECIFIED.,.F.,.F.,(3,3),(0.,1.),.UNSPECIFIED.);
#23965=B_SPLINE_CURVE_WITH_KNOTS('',2,(#84255,#84256,#84257),
 .UNSPECIFIED.,.F.,.F.,(3,3),(0.,1.),.UNSPECIFIED.);
#23966=B_SPLINE_CURVE_WITH_KNOTS('',2,(#84265,#84266,#84267),
 .UNSPECIFIED.,.F.,.F.,(3,3),(0.,1.),.UNSPECIFIED.);
#23967=B_SPLINE_CURVE_WITH_KNOTS('',2,(#84270,#84271,#84272),
 .UNSPECIFIED.,.F.,.F.,(3,3),(0.,1.),.UNSPECIFIED.);
#23968=B_SPLINE_CURVE_WITH_KNOTS('',2,(#84280,#84281,#84282),
 .UNSPECIFIED.,.F.,.F.,(3,3),(0.,1.),.UNSPECIFIED.);
#23969=B_SPLINE_CURVE_WITH_KNOTS('',2,(#84285,#84286,#84287),
 .UNSPECIFIED.,.F.,.F.,(3,3),(0.,1.),.UNSPECIFIED.);
#23970=B_SPLINE_CURVE_WITH_KNOTS('',2,(#84295,#84296,#84297),
 .UNSPECIFIED.,.F.,.F.,(3,3),(0.,1.),.UNSPECIFIED.);
#23971=B_SPLINE_CURVE_WITH_KNOTS('',2,(#84300,#84301,#84302),
 .UNSPECIFIED.,.F.,.F.,(3,3),(0.,1.),.UNSPECIFIED.);
#23972=B_SPLINE_CURVE_WITH_KNOTS('',2,(#84346,#84347,#84348),
 .UNSPECIFIED.,.F.,.F.,(3,3),(0.,1.),.UNSPECIFIED.);
#23973=B_SPLINE_CURVE_WITH_KNOTS('',2,(#84351,#84352,#84353),
 .UNSPECIFIED.,.F.,.F.,(3,3),(0.,1.),.UNSPECIFIED.);
#23974=B_SPLINE_CURVE_WITH_KNOTS('',2,(#84361,#84362,#84363),
 .UNSPECIFIED.,.F.,.F.,(3,3),(0.,1.),.UNSPECIFIED.);
#23975=B_SPLINE_CURVE_WITH_KNOTS('',2,(#84366,#84367,#84368),
 .UNSPECIFIED.,.F.,.F.,(3,3),(0.,1.),.UNSPECIFIED.);
#23976=B_SPLINE_CURVE_WITH_KNOTS('',2,(#84376,#84377,#84378),
 .UNSPECIFIED.,.F.,.F.,(3,3),(0.,1.),.UNSPECIFIED.);
#23977=B_SPLINE_CURVE_WITH_KNOTS('',2,(#84381,#84382,#84383),
 .UNSPECIFIED.,.F.,.F.,(3,3),(0.,1.),.UNSPECIFIED.);
#23978=B_SPLINE_CURVE_WITH_KNOTS('',2,(#84391,#84392,#84393),
 .UNSPECIFIED.,.F.,.F.,(3,3),(0.,1.),.UNSPECIFIED.);
#23979=B_SPLINE_CURVE_WITH_KNOTS('',2,(#84396,#84397,#84398),
 .UNSPECIFIED.,.F.,.F.,(3,3),(0.,1.),.UNSPECIFIED.);
#23980=B_SPLINE_CURVE_WITH_KNOTS('',2,(#84406,#84407,#84408),
 .UNSPECIFIED.,.F.,.F.,(3,3),(0.,1.),.UNSPECIFIED.);
#23981=B_SPLINE_CURVE_WITH_KNOTS('',2,(#84411,#84412,#84413),
 .UNSPECIFIED.,.F.,.F.,(3,3),(0.,1.),.UNSPECIFIED.);
#23982=B_SPLINE_CURVE_WITH_KNOTS('',2,(#84421,#84422,#84423),
 .UNSPECIFIED.,.F.,.F.,(3,3),(0.,1.),.UNSPECIFIED.);
#23983=B_SPLINE_CURVE_WITH_KNOTS('',2,(#84426,#84427,#84428),
 .UNSPECIFIED.,.F.,.F.,(3,3),(0.,1.),.UNSPECIFIED.);
#23984=B_SPLINE_CURVE_WITH_KNOTS('',2,(#84436,#84437,#84438),
 .UNSPECIFIED.,.F.,.F.,(3,3),(0.,1.),.UNSPECIFIED.);
#23985=B_SPLINE_CURVE_WITH_KNOTS('',2,(#84441,#84442,#84443),
 .UNSPECIFIED.,.F.,.F.,(3,3),(0.,1.),.UNSPECIFIED.);
#23986=B_SPLINE_CURVE_WITH_KNOTS('',2,(#84451,#84452,#84453),
 .UNSPECIFIED.,.F.,.F.,(3,3),(0.,1.),.UNSPECIFIED.);
#23987=B_SPLINE_CURVE_WITH_KNOTS('',2,(#84456,#84457,#84458),
 .UNSPECIFIED.,.F.,.F.,(3,3),(0.,1.),.UNSPECIFIED.);
#23988=B_SPLINE_CURVE_WITH_KNOTS('',2,(#84471,#84472,#84473),
 .UNSPECIFIED.,.F.,.F.,(3,3),(0.,1.),.UNSPECIFIED.);
#23989=B_SPLINE_CURVE_WITH_KNOTS('',2,(#84474,#84475,#84476),
 .UNSPECIFIED.,.F.,.F.,(3,3),(0.,1.),.UNSPECIFIED.);
#23990=B_SPLINE_CURVE_WITH_KNOTS('',2,(#84487,#84488,#84489),
 .UNSPECIFIED.,.F.,.F.,(3,3),(0.,1.),.UNSPECIFIED.);
#23991=B_SPLINE_CURVE_WITH_KNOTS('',2,(#84493,#84494,#84495),
 .UNSPECIFIED.,.F.,.F.,(3,3),(0.,1.),.UNSPECIFIED.);
#23992=B_SPLINE_CURVE_WITH_KNOTS('',2,(#84504,#84505,#84506),
 .UNSPECIFIED.,.F.,.F.,(3,3),(0.,1.),.UNSPECIFIED.);
#23993=B_SPLINE_CURVE_WITH_KNOTS('',2,(#84509,#84510,#84511),
 .UNSPECIFIED.,.F.,.F.,(3,3),(0.,1.),.UNSPECIFIED.);
#23994=B_SPLINE_CURVE_WITH_KNOTS('',2,(#84519,#84520,#84521),
 .UNSPECIFIED.,.F.,.F.,(3,3),(0.,1.),.UNSPECIFIED.);
#23995=B_SPLINE_CURVE_WITH_KNOTS('',2,(#84524,#84525,#84526),
 .UNSPECIFIED.,.F.,.F.,(3,3),(0.,1.),.UNSPECIFIED.);
#23996=B_SPLINE_CURVE_WITH_KNOTS('',2,(#84534,#84535,#84536),
 .UNSPECIFIED.,.F.,.F.,(3,3),(0.,1.),.UNSPECIFIED.);
#23997=B_SPLINE_CURVE_WITH_KNOTS('',2,(#84539,#84540,#84541),
 .UNSPECIFIED.,.F.,.F.,(3,3),(0.,1.),.UNSPECIFIED.);
#23998=B_SPLINE_CURVE_WITH_KNOTS('',2,(#84549,#84550,#84551),
 .UNSPECIFIED.,.F.,.F.,(3,3),(0.,1.),.UNSPECIFIED.);
#23999=B_SPLINE_CURVE_WITH_KNOTS('',2,(#84554,#84555,#84556),
 .UNSPECIFIED.,.F.,.F.,(3,3),(0.,1.),.UNSPECIFIED.);
#24000=B_SPLINE_CURVE_WITH_KNOTS('',2,(#84564,#84565,#84566),
 .UNSPECIFIED.,.F.,.F.,(3,3),(0.,1.),.UNSPECIFIED.);
#24001=B_SPLINE_CURVE_WITH_KNOTS('',2,(#84569,#84570,#84571),
 .UNSPECIFIED.,.F.,.F.,(3,3),(0.,1.),.UNSPECIFIED.);
#24002=B_SPLINE_CURVE_WITH_KNOTS('',2,(#84579,#84580,#84581),
 .UNSPECIFIED.,.F.,.F.,(3,3),(0.,1.),.UNSPECIFIED.);
#24003=B_SPLINE_CURVE_WITH_KNOTS('',2,(#84584,#84585,#84586),
 .UNSPECIFIED.,.F.,.F.,(3,3),(0.,1.),.UNSPECIFIED.);
#24004=B_SPLINE_CURVE_WITH_KNOTS('',2,(#84593,#84594,#84595),
 .UNSPECIFIED.,.F.,.F.,(3,3),(0.,1.),.UNSPECIFIED.);
#24005=B_SPLINE_CURVE_WITH_KNOTS('',2,(#84596,#84597,#84598),
 .UNSPECIFIED.,.F.,.F.,(3,3),(0.,1.),.UNSPECIFIED.);
#24006=B_SPLINE_CURVE_WITH_KNOTS('',2,(#84607,#84608,#84609),
 .UNSPECIFIED.,.F.,.F.,(3,3),(0.,1.),.UNSPECIFIED.);
#24007=B_SPLINE_CURVE_WITH_KNOTS('',2,(#84613,#84614,#84615),
 .UNSPECIFIED.,.F.,.F.,(3,3),(0.,1.),.UNSPECIFIED.);
#24008=B_SPLINE_CURVE_WITH_KNOTS('',2,(#84624,#84625,#84626),
 .UNSPECIFIED.,.F.,.F.,(3,3),(0.,1.),.UNSPECIFIED.);
#24009=B_SPLINE_CURVE_WITH_KNOTS('',2,(#84629,#84630,#84631),
 .UNSPECIFIED.,.F.,.F.,(3,3),(0.,1.),.UNSPECIFIED.);
#24010=B_SPLINE_CURVE_WITH_KNOTS('',2,(#84639,#84640,#84641),
 .UNSPECIFIED.,.F.,.F.,(3,3),(0.,1.),.UNSPECIFIED.);
#24011=B_SPLINE_CURVE_WITH_KNOTS('',2,(#84644,#84645,#84646),
 .UNSPECIFIED.,.F.,.F.,(3,3),(0.,1.),.UNSPECIFIED.);
#24012=B_SPLINE_CURVE_WITH_KNOTS('',2,(#84654,#84655,#84656),
 .UNSPECIFIED.,.F.,.F.,(3,3),(0.,1.),.UNSPECIFIED.);
#24013=B_SPLINE_CURVE_WITH_KNOTS('',2,(#84659,#84660,#84661),
 .UNSPECIFIED.,.F.,.F.,(3,3),(0.,1.),.UNSPECIFIED.);
#24014=B_SPLINE_CURVE_WITH_KNOTS('',2,(#84669,#84670,#84671),
 .UNSPECIFIED.,.F.,.F.,(3,3),(0.,1.),.UNSPECIFIED.);
#24015=B_SPLINE_CURVE_WITH_KNOTS('',2,(#84674,#84675,#84676),
 .UNSPECIFIED.,.F.,.F.,(3,3),(0.,1.),.UNSPECIFIED.);
#24016=B_SPLINE_CURVE_WITH_KNOTS('',2,(#84684,#84685,#84686),
 .UNSPECIFIED.,.F.,.F.,(3,3),(0.,1.),.UNSPECIFIED.);
#24017=B_SPLINE_CURVE_WITH_KNOTS('',2,(#84689,#84690,#84691),
 .UNSPECIFIED.,.F.,.F.,(3,3),(0.,1.),.UNSPECIFIED.);
#24018=B_SPLINE_CURVE_WITH_KNOTS('',2,(#84699,#84700,#84701),
 .UNSPECIFIED.,.F.,.F.,(3,3),(0.,1.),.UNSPECIFIED.);
#24019=B_SPLINE_CURVE_WITH_KNOTS('',2,(#84704,#84705,#84706),
 .UNSPECIFIED.,.F.,.F.,(3,3),(0.,1.),.UNSPECIFIED.);
#24020=B_SPLINE_CURVE_WITH_KNOTS('',2,(#84714,#84715,#84716),
 .UNSPECIFIED.,.F.,.F.,(3,3),(0.,1.),.UNSPECIFIED.);
#24021=B_SPLINE_CURVE_WITH_KNOTS('',2,(#84719,#84720,#84721),
 .UNSPECIFIED.,.F.,.F.,(3,3),(0.,1.),.UNSPECIFIED.);
#24022=B_SPLINE_CURVE_WITH_KNOTS('',2,(#84729,#84730,#84731),
 .UNSPECIFIED.,.F.,.F.,(3,3),(0.,1.),.UNSPECIFIED.);
#24023=B_SPLINE_CURVE_WITH_KNOTS('',2,(#84734,#84735,#84736),
 .UNSPECIFIED.,.F.,.F.,(3,3),(0.,1.),.UNSPECIFIED.);
#24024=B_SPLINE_CURVE_WITH_KNOTS('',2,(#84744,#84745,#84746),
 .UNSPECIFIED.,.F.,.F.,(3,3),(0.,1.),.UNSPECIFIED.);
#24025=B_SPLINE_CURVE_WITH_KNOTS('',2,(#84749,#84750,#84751),
 .UNSPECIFIED.,.F.,.F.,(3,3),(0.,1.),.UNSPECIFIED.);
#24026=B_SPLINE_CURVE_WITH_KNOTS('',2,(#84759,#84760,#84761),
 .UNSPECIFIED.,.F.,.F.,(3,3),(0.,1.),.UNSPECIFIED.);
#24027=B_SPLINE_CURVE_WITH_KNOTS('',2,(#84764,#84765,#84766),
 .UNSPECIFIED.,.F.,.F.,(3,3),(0.,1.),.UNSPECIFIED.);
#24028=B_SPLINE_CURVE_WITH_KNOTS('',2,(#84773,#84774,#84775),
 .UNSPECIFIED.,.F.,.F.,(3,3),(0.,1.),.UNSPECIFIED.);
#24029=B_SPLINE_CURVE_WITH_KNOTS('',2,(#84776,#84777,#84778),
 .UNSPECIFIED.,.F.,.F.,(3,3),(0.,1.),.UNSPECIFIED.);
#24030=B_SPLINE_CURVE_WITH_KNOTS('',2,(#84788,#84789,#84790),
 .UNSPECIFIED.,.F.,.F.,(3,3),(0.,1.),.UNSPECIFIED.);
#24031=B_SPLINE_CURVE_WITH_KNOTS('',2,(#84794,#84795,#84796),
 .UNSPECIFIED.,.F.,.F.,(3,3),(0.,1.),.UNSPECIFIED.);
#24032=B_SPLINE_CURVE_WITH_KNOTS('',2,(#84805,#84806,#84807),
 .UNSPECIFIED.,.F.,.F.,(3,3),(0.,1.),.UNSPECIFIED.);
#24033=B_SPLINE_CURVE_WITH_KNOTS('',2,(#84810,#84811,#84812),
 .UNSPECIFIED.,.F.,.F.,(3,3),(0.,1.),.UNSPECIFIED.);
#24034=B_SPLINE_CURVE_WITH_KNOTS('',2,(#84820,#84821,#84822),
 .UNSPECIFIED.,.F.,.F.,(3,3),(0.,1.),.UNSPECIFIED.);
#24035=B_SPLINE_CURVE_WITH_KNOTS('',2,(#84825,#84826,#84827),
 .UNSPECIFIED.,.F.,.F.,(3,3),(0.,1.),.UNSPECIFIED.);
#24036=B_SPLINE_CURVE_WITH_KNOTS('',2,(#84835,#84836,#84837),
 .UNSPECIFIED.,.F.,.F.,(3,3),(0.,1.),.UNSPECIFIED.);
#24037=B_SPLINE_CURVE_WITH_KNOTS('',2,(#84840,#84841,#84842),
 .UNSPECIFIED.,.F.,.F.,(3,3),(0.,1.),.UNSPECIFIED.);
#24038=B_SPLINE_CURVE_WITH_KNOTS('',2,(#84850,#84851,#84852),
 .UNSPECIFIED.,.F.,.F.,(3,3),(0.,1.),.UNSPECIFIED.);
#24039=B_SPLINE_CURVE_WITH_KNOTS('',2,(#84855,#84856,#84857),
 .UNSPECIFIED.,.F.,.F.,(3,3),(0.,1.),.UNSPECIFIED.);
#24040=B_SPLINE_CURVE_WITH_KNOTS('',2,(#84865,#84866,#84867),
 .UNSPECIFIED.,.F.,.F.,(3,3),(0.,1.),.UNSPECIFIED.);
#24041=B_SPLINE_CURVE_WITH_KNOTS('',2,(#84870,#84871,#84872),
 .UNSPECIFIED.,.F.,.F.,(3,3),(0.,1.),.UNSPECIFIED.);
#24042=B_SPLINE_CURVE_WITH_KNOTS('',2,(#84880,#84881,#84882),
 .UNSPECIFIED.,.F.,.F.,(3,3),(0.,1.),.UNSPECIFIED.);
#24043=B_SPLINE_CURVE_WITH_KNOTS('',2,(#84885,#84886,#84887),
 .UNSPECIFIED.,.F.,.F.,(3,3),(0.,1.),.UNSPECIFIED.);
#24044=B_SPLINE_CURVE_WITH_KNOTS('',2,(#84895,#84896,#84897),
 .UNSPECIFIED.,.F.,.F.,(3,3),(0.,1.),.UNSPECIFIED.);
#24045=B_SPLINE_CURVE_WITH_KNOTS('',2,(#84900,#84901,#84902),
 .UNSPECIFIED.,.F.,.F.,(3,3),(0.,1.),.UNSPECIFIED.);
#24046=B_SPLINE_CURVE_WITH_KNOTS('',2,(#84909,#84910,#84911),
 .UNSPECIFIED.,.F.,.F.,(3,3),(0.,1.),.UNSPECIFIED.);
#24047=B_SPLINE_CURVE_WITH_KNOTS('',2,(#84912,#84913,#84914),
 .UNSPECIFIED.,.F.,.F.,(3,3),(0.,1.),.UNSPECIFIED.);
#24048=B_SPLINE_CURVE_WITH_KNOTS('',2,(#84923,#84924,#84925),
 .UNSPECIFIED.,.F.,.F.,(3,3),(0.,1.),.UNSPECIFIED.);
#24049=B_SPLINE_CURVE_WITH_KNOTS('',2,(#84929,#84930,#84931),
 .UNSPECIFIED.,.F.,.F.,(3,3),(0.,1.),.UNSPECIFIED.);
#24050=B_SPLINE_CURVE_WITH_KNOTS('',2,(#84940,#84941,#84942),
 .UNSPECIFIED.,.F.,.F.,(3,3),(0.,1.),.UNSPECIFIED.);
#24051=B_SPLINE_CURVE_WITH_KNOTS('',2,(#84945,#84946,#84947),
 .UNSPECIFIED.,.F.,.F.,(3,3),(0.,1.),.UNSPECIFIED.);
#24052=B_SPLINE_CURVE_WITH_KNOTS('',2,(#84955,#84956,#84957),
 .UNSPECIFIED.,.F.,.F.,(3,3),(0.,1.),.UNSPECIFIED.);
#24053=B_SPLINE_CURVE_WITH_KNOTS('',2,(#84960,#84961,#84962),
 .UNSPECIFIED.,.F.,.F.,(3,3),(0.,1.),.UNSPECIFIED.);
#24054=B_SPLINE_CURVE_WITH_KNOTS('',2,(#84970,#84971,#84972),
 .UNSPECIFIED.,.F.,.F.,(3,3),(0.,1.),.UNSPECIFIED.);
#24055=B_SPLINE_CURVE_WITH_KNOTS('',2,(#84975,#84976,#84977),
 .UNSPECIFIED.,.F.,.F.,(3,3),(0.,1.),.UNSPECIFIED.);
#24056=B_SPLINE_CURVE_WITH_KNOTS('',2,(#84985,#84986,#84987),
 .UNSPECIFIED.,.F.,.F.,(3,3),(0.,1.),.UNSPECIFIED.);
#24057=B_SPLINE_CURVE_WITH_KNOTS('',2,(#84990,#84991,#84992),
 .UNSPECIFIED.,.F.,.F.,(3,3),(0.,1.),.UNSPECIFIED.);
#24058=B_SPLINE_CURVE_WITH_KNOTS('',2,(#85000,#85001,#85002),
 .UNSPECIFIED.,.F.,.F.,(3,3),(0.,1.),.UNSPECIFIED.);
#24059=B_SPLINE_CURVE_WITH_KNOTS('',2,(#85005,#85006,#85007),
 .UNSPECIFIED.,.F.,.F.,(3,3),(0.,1.),.UNSPECIFIED.);
#24060=B_SPLINE_CURVE_WITH_KNOTS('',2,(#85015,#85016,#85017),
 .UNSPECIFIED.,.F.,.F.,(3,3),(0.,1.),.UNSPECIFIED.);
#24061=B_SPLINE_CURVE_WITH_KNOTS('',2,(#85020,#85021,#85022),
 .UNSPECIFIED.,.F.,.F.,(3,3),(0.,1.),.UNSPECIFIED.);
#24062=B_SPLINE_CURVE_WITH_KNOTS('',2,(#85030,#85031,#85032),
 .UNSPECIFIED.,.F.,.F.,(3,3),(0.,1.),.UNSPECIFIED.);
#24063=B_SPLINE_CURVE_WITH_KNOTS('',2,(#85035,#85036,#85037),
 .UNSPECIFIED.,.F.,.F.,(3,3),(0.,1.),.UNSPECIFIED.);
#24064=B_SPLINE_CURVE_WITH_KNOTS('',2,(#85045,#85046,#85047),
 .UNSPECIFIED.,.F.,.F.,(3,3),(0.,1.),.UNSPECIFIED.);
#24065=B_SPLINE_CURVE_WITH_KNOTS('',2,(#85050,#85051,#85052),
 .UNSPECIFIED.,.F.,.F.,(3,3),(0.,1.),.UNSPECIFIED.);
#24066=B_SPLINE_CURVE_WITH_KNOTS('',2,(#85060,#85061,#85062),
 .UNSPECIFIED.,.F.,.F.,(3,3),(0.,1.),.UNSPECIFIED.);
#24067=B_SPLINE_CURVE_WITH_KNOTS('',2,(#85065,#85066,#85067),
 .UNSPECIFIED.,.F.,.F.,(3,3),(0.,1.),.UNSPECIFIED.);
#24068=B_SPLINE_CURVE_WITH_KNOTS('',2,(#85075,#85076,#85077),
 .UNSPECIFIED.,.F.,.F.,(3,3),(0.,1.),.UNSPECIFIED.);
#24069=B_SPLINE_CURVE_WITH_KNOTS('',2,(#85080,#85081,#85082),
 .UNSPECIFIED.,.F.,.F.,(3,3),(0.,1.),.UNSPECIFIED.);
#24070=B_SPLINE_CURVE_WITH_KNOTS('',2,(#85090,#85091,#85092),
 .UNSPECIFIED.,.F.,.F.,(3,3),(0.,1.),.UNSPECIFIED.);
#24071=B_SPLINE_CURVE_WITH_KNOTS('',2,(#85095,#85096,#85097),
 .UNSPECIFIED.,.F.,.F.,(3,3),(0.,1.),.UNSPECIFIED.);
#24072=B_SPLINE_CURVE_WITH_KNOTS('',2,(#85105,#85106,#85107),
 .UNSPECIFIED.,.F.,.F.,(3,3),(0.,1.),.UNSPECIFIED.);
#24073=B_SPLINE_CURVE_WITH_KNOTS('',2,(#85110,#85111,#85112),
 .UNSPECIFIED.,.F.,.F.,(3,3),(0.,1.),.UNSPECIFIED.);
#24074=B_SPLINE_CURVE_WITH_KNOTS('',2,(#85120,#85121,#85122),
 .UNSPECIFIED.,.F.,.F.,(3,3),(0.,1.),.UNSPECIFIED.);
#24075=B_SPLINE_CURVE_WITH_KNOTS('',2,(#85125,#85126,#85127),
 .UNSPECIFIED.,.F.,.F.,(3,3),(0.,1.),.UNSPECIFIED.);
#24076=B_SPLINE_CURVE_WITH_KNOTS('',2,(#85135,#85136,#85137),
 .UNSPECIFIED.,.F.,.F.,(3,3),(0.,1.),.UNSPECIFIED.);
#24077=B_SPLINE_CURVE_WITH_KNOTS('',2,(#85140,#85141,#85142),
 .UNSPECIFIED.,.F.,.F.,(3,3),(0.,1.),.UNSPECIFIED.);
#24078=B_SPLINE_CURVE_WITH_KNOTS('',2,(#85150,#85151,#85152),
 .UNSPECIFIED.,.F.,.F.,(3,3),(0.,1.),.UNSPECIFIED.);
#24079=B_SPLINE_CURVE_WITH_KNOTS('',2,(#85155,#85156,#85157),
 .UNSPECIFIED.,.F.,.F.,(3,3),(0.,1.),.UNSPECIFIED.);
#24080=B_SPLINE_CURVE_WITH_KNOTS('',2,(#85165,#85166,#85167),
 .UNSPECIFIED.,.F.,.F.,(3,3),(0.,1.),.UNSPECIFIED.);
#24081=B_SPLINE_CURVE_WITH_KNOTS('',2,(#85170,#85171,#85172),
 .UNSPECIFIED.,.F.,.F.,(3,3),(0.,1.),.UNSPECIFIED.);
#24082=B_SPLINE_CURVE_WITH_KNOTS('',2,(#85185,#85186,#85187),
 .UNSPECIFIED.,.F.,.F.,(3,3),(0.,1.),.UNSPECIFIED.);
#24083=B_SPLINE_CURVE_WITH_KNOTS('',2,(#85188,#85189,#85190),
 .UNSPECIFIED.,.F.,.F.,(3,3),(0.,1.),.UNSPECIFIED.);
#24084=B_SPLINE_CURVE_WITH_KNOTS('',2,(#85202,#85203,#85204),
 .UNSPECIFIED.,.F.,.F.,(3,3),(0.,1.),.UNSPECIFIED.);
#24085=B_SPLINE_CURVE_WITH_KNOTS('',2,(#85208,#85209,#85210),
 .UNSPECIFIED.,.F.,.F.,(3,3),(0.,1.),.UNSPECIFIED.);
#24086=B_SPLINE_CURVE_WITH_KNOTS('',2,(#85219,#85220,#85221),
 .UNSPECIFIED.,.F.,.F.,(3,3),(0.,1.),.UNSPECIFIED.);
#24087=B_SPLINE_CURVE_WITH_KNOTS('',2,(#85224,#85225,#85226),
 .UNSPECIFIED.,.F.,.F.,(3,3),(0.,1.),.UNSPECIFIED.);
#24088=B_SPLINE_CURVE_WITH_KNOTS('',2,(#85234,#85235,#85236),
 .UNSPECIFIED.,.F.,.F.,(3,3),(0.,1.),.UNSPECIFIED.);
#24089=B_SPLINE_CURVE_WITH_KNOTS('',2,(#85239,#85240,#85241),
 .UNSPECIFIED.,.F.,.F.,(3,3),(0.,1.),.UNSPECIFIED.);
#24090=B_SPLINE_CURVE_WITH_KNOTS('',2,(#85249,#85250,#85251),
 .UNSPECIFIED.,.F.,.F.,(3,3),(0.,1.),.UNSPECIFIED.);
#24091=B_SPLINE_CURVE_WITH_KNOTS('',2,(#85254,#85255,#85256),
 .UNSPECIFIED.,.F.,.F.,(3,3),(0.,1.),.UNSPECIFIED.);
#24092=B_SPLINE_CURVE_WITH_KNOTS('',2,(#85264,#85265,#85266),
 .UNSPECIFIED.,.F.,.F.,(3,3),(0.,1.),.UNSPECIFIED.);
#24093=B_SPLINE_CURVE_WITH_KNOTS('',2,(#85269,#85270,#85271),
 .UNSPECIFIED.,.F.,.F.,(3,3),(0.,1.),.UNSPECIFIED.);
#24094=B_SPLINE_CURVE_WITH_KNOTS('',2,(#85279,#85280,#85281),
 .UNSPECIFIED.,.F.,.F.,(3,3),(0.,1.),.UNSPECIFIED.);
#24095=B_SPLINE_CURVE_WITH_KNOTS('',2,(#85284,#85285,#85286),
 .UNSPECIFIED.,.F.,.F.,(3,3),(0.,1.),.UNSPECIFIED.);
#24096=B_SPLINE_CURVE_WITH_KNOTS('',2,(#85294,#85295,#85296),
 .UNSPECIFIED.,.F.,.F.,(3,3),(0.,1.),.UNSPECIFIED.);
#24097=B_SPLINE_CURVE_WITH_KNOTS('',2,(#85299,#85300,#85301),
 .UNSPECIFIED.,.F.,.F.,(3,3),(0.,1.),.UNSPECIFIED.);
#24098=B_SPLINE_CURVE_WITH_KNOTS('',2,(#85308,#85309,#85310),
 .UNSPECIFIED.,.F.,.F.,(3,3),(0.,1.),.UNSPECIFIED.);
#24099=B_SPLINE_CURVE_WITH_KNOTS('',2,(#85311,#85312,#85313),
 .UNSPECIFIED.,.F.,.F.,(3,3),(0.,1.),.UNSPECIFIED.);
#24100=B_SPLINE_CURVE_WITH_KNOTS('',2,(#85322,#85323,#85324),
 .UNSPECIFIED.,.F.,.F.,(3,3),(0.,1.),.UNSPECIFIED.);
#24101=B_SPLINE_CURVE_WITH_KNOTS('',2,(#85328,#85329,#85330),
 .UNSPECIFIED.,.F.,.F.,(3,3),(0.,1.),.UNSPECIFIED.);
#24102=B_SPLINE_CURVE_WITH_KNOTS('',2,(#85339,#85340,#85341),
 .UNSPECIFIED.,.F.,.F.,(3,3),(0.,1.),.UNSPECIFIED.);
#24103=B_SPLINE_CURVE_WITH_KNOTS('',2,(#85344,#85345,#85346),
 .UNSPECIFIED.,.F.,.F.,(3,3),(0.,1.),.UNSPECIFIED.);
#24104=B_SPLINE_CURVE_WITH_KNOTS('',2,(#85354,#85355,#85356),
 .UNSPECIFIED.,.F.,.F.,(3,3),(0.,1.),.UNSPECIFIED.);
#24105=B_SPLINE_CURVE_WITH_KNOTS('',2,(#85359,#85360,#85361),
 .UNSPECIFIED.,.F.,.F.,(3,3),(0.,1.),.UNSPECIFIED.);
#24106=B_SPLINE_CURVE_WITH_KNOTS('',2,(#85369,#85370,#85371),
 .UNSPECIFIED.,.F.,.F.,(3,3),(0.,1.),.UNSPECIFIED.);
#24107=B_SPLINE_CURVE_WITH_KNOTS('',2,(#85374,#85375,#85376),
 .UNSPECIFIED.,.F.,.F.,(3,3),(0.,1.),.UNSPECIFIED.);
#24108=B_SPLINE_CURVE_WITH_KNOTS('',2,(#85384,#85385,#85386),
 .UNSPECIFIED.,.F.,.F.,(3,3),(0.,1.),.UNSPECIFIED.);
#24109=B_SPLINE_CURVE_WITH_KNOTS('',2,(#85389,#85390,#85391),
 .UNSPECIFIED.,.F.,.F.,(3,3),(0.,1.),.UNSPECIFIED.);
#24110=B_SPLINE_CURVE_WITH_KNOTS('',2,(#85399,#85400,#85401),
 .UNSPECIFIED.,.F.,.F.,(3,3),(0.,1.),.UNSPECIFIED.);
#24111=B_SPLINE_CURVE_WITH_KNOTS('',2,(#85404,#85405,#85406),
 .UNSPECIFIED.,.F.,.F.,(3,3),(0.,1.),.UNSPECIFIED.);
#24112=B_SPLINE_CURVE_WITH_KNOTS('',2,(#85414,#85415,#85416),
 .UNSPECIFIED.,.F.,.F.,(3,3),(0.,1.),.UNSPECIFIED.);
#24113=B_SPLINE_CURVE_WITH_KNOTS('',2,(#85419,#85420,#85421),
 .UNSPECIFIED.,.F.,.F.,(3,3),(0.,1.),.UNSPECIFIED.);
#24114=B_SPLINE_CURVE_WITH_KNOTS('',2,(#85429,#85430,#85431),
 .UNSPECIFIED.,.F.,.F.,(3,3),(0.,1.),.UNSPECIFIED.);
#24115=B_SPLINE_CURVE_WITH_KNOTS('',2,(#85434,#85435,#85436),
 .UNSPECIFIED.,.F.,.F.,(3,3),(0.,1.),.UNSPECIFIED.);
#24116=B_SPLINE_CURVE_WITH_KNOTS('',2,(#85444,#85445,#85446),
 .UNSPECIFIED.,.F.,.F.,(3,3),(0.,1.),.UNSPECIFIED.);
#24117=B_SPLINE_CURVE_WITH_KNOTS('',2,(#85449,#85450,#85451),
 .UNSPECIFIED.,.F.,.F.,(3,3),(0.,1.),.UNSPECIFIED.);
#24118=B_SPLINE_CURVE_WITH_KNOTS('',2,(#85459,#85460,#85461),
 .UNSPECIFIED.,.F.,.F.,(3,3),(0.,1.),.UNSPECIFIED.);
#24119=B_SPLINE_CURVE_WITH_KNOTS('',2,(#85464,#85465,#85466),
 .UNSPECIFIED.,.F.,.F.,(3,3),(0.,1.),.UNSPECIFIED.);
#24120=B_SPLINE_CURVE_WITH_KNOTS('',2,(#85474,#85475,#85476),
 .UNSPECIFIED.,.F.,.F.,(3,3),(0.,1.),.UNSPECIFIED.);
#24121=B_SPLINE_CURVE_WITH_KNOTS('',2,(#85479,#85480,#85481),
 .UNSPECIFIED.,.F.,.F.,(3,3),(0.,1.),.UNSPECIFIED.);
#24122=B_SPLINE_CURVE_WITH_KNOTS('',2,(#85488,#85489,#85490),
 .UNSPECIFIED.,.F.,.F.,(3,3),(0.,1.),.UNSPECIFIED.);
#24123=B_SPLINE_CURVE_WITH_KNOTS('',2,(#85491,#85492,#85493),
 .UNSPECIFIED.,.F.,.F.,(3,3),(0.,1.),.UNSPECIFIED.);
#24124=B_SPLINE_CURVE_WITH_KNOTS('',2,(#85503,#85504,#85505),
 .UNSPECIFIED.,.F.,.F.,(3,3),(0.,1.),.UNSPECIFIED.);
#24125=B_SPLINE_CURVE_WITH_KNOTS('',2,(#85509,#85510,#85511),
 .UNSPECIFIED.,.F.,.F.,(3,3),(0.,1.),.UNSPECIFIED.);
#24126=B_SPLINE_CURVE_WITH_KNOTS('',2,(#85520,#85521,#85522),
 .UNSPECIFIED.,.F.,.F.,(3,3),(0.,1.),.UNSPECIFIED.);
#24127=B_SPLINE_CURVE_WITH_KNOTS('',2,(#85525,#85526,#85527),
 .UNSPECIFIED.,.F.,.F.,(3,3),(0.,1.),.UNSPECIFIED.);
#24128=B_SPLINE_CURVE_WITH_KNOTS('',2,(#85535,#85536,#85537),
 .UNSPECIFIED.,.F.,.F.,(3,3),(0.,1.),.UNSPECIFIED.);
#24129=B_SPLINE_CURVE_WITH_KNOTS('',2,(#85540,#85541,#85542),
 .UNSPECIFIED.,.F.,.F.,(3,3),(0.,1.),.UNSPECIFIED.);
#24130=B_SPLINE_CURVE_WITH_KNOTS('',2,(#85556,#85557,#85558),
 .UNSPECIFIED.,.F.,.F.,(3,3),(0.,1.),.UNSPECIFIED.);
#24131=B_SPLINE_CURVE_WITH_KNOTS('',2,(#85561,#85562,#85563),
 .UNSPECIFIED.,.F.,.F.,(3,3),(0.,1.),.UNSPECIFIED.);
#24132=B_SPLINE_CURVE_WITH_KNOTS('',2,(#85571,#85572,#85573),
 .UNSPECIFIED.,.F.,.F.,(3,3),(0.,1.),.UNSPECIFIED.);
#24133=B_SPLINE_CURVE_WITH_KNOTS('',2,(#85576,#85577,#85578),
 .UNSPECIFIED.,.F.,.F.,(3,3),(0.,1.),.UNSPECIFIED.);
#24134=B_SPLINE_CURVE_WITH_KNOTS('',2,(#85586,#85587,#85588),
 .UNSPECIFIED.,.F.,.F.,(3,3),(0.,1.),.UNSPECIFIED.);
#24135=B_SPLINE_CURVE_WITH_KNOTS('',2,(#85591,#85592,#85593),
 .UNSPECIFIED.,.F.,.F.,(3,3),(0.,1.),.UNSPECIFIED.);
#24136=B_SPLINE_CURVE_WITH_KNOTS('',2,(#85625,#85626,#85627),
 .UNSPECIFIED.,.F.,.F.,(3,3),(0.,1.),.UNSPECIFIED.);
#24137=B_SPLINE_CURVE_WITH_KNOTS('',2,(#85631,#85632,#85633),
 .UNSPECIFIED.,.F.,.F.,(3,3),(0.,1.),.UNSPECIFIED.);
#24138=B_SPLINE_CURVE_WITH_KNOTS('',2,(#85642,#85643,#85644),
 .UNSPECIFIED.,.F.,.F.,(3,3),(0.,1.),.UNSPECIFIED.);
#24139=B_SPLINE_CURVE_WITH_KNOTS('',2,(#85647,#85648,#85649),
 .UNSPECIFIED.,.F.,.F.,(3,3),(0.,1.),.UNSPECIFIED.);
#24140=B_SPLINE_CURVE_WITH_KNOTS('',2,(#85657,#85658,#85659),
 .UNSPECIFIED.,.F.,.F.,(3,3),(0.,1.),.UNSPECIFIED.);
#24141=B_SPLINE_CURVE_WITH_KNOTS('',2,(#85662,#85663,#85664),
 .UNSPECIFIED.,.F.,.F.,(3,3),(0.,1.),.UNSPECIFIED.);
#24142=B_SPLINE_CURVE_WITH_KNOTS('',2,(#85672,#85673,#85674),
 .UNSPECIFIED.,.F.,.F.,(3,3),(0.,1.),.UNSPECIFIED.);
#24143=B_SPLINE_CURVE_WITH_KNOTS('',2,(#85677,#85678,#85679),
 .UNSPECIFIED.,.F.,.F.,(3,3),(0.,1.),.UNSPECIFIED.);
#24144=B_SPLINE_CURVE_WITH_KNOTS('',2,(#85687,#85688,#85689),
 .UNSPECIFIED.,.F.,.F.,(3,3),(0.,1.),.UNSPECIFIED.);
#24145=B_SPLINE_CURVE_WITH_KNOTS('',2,(#85692,#85693,#85694),
 .UNSPECIFIED.,.F.,.F.,(3,3),(0.,1.),.UNSPECIFIED.);
#24146=B_SPLINE_CURVE_WITH_KNOTS('',2,(#85702,#85703,#85704),
 .UNSPECIFIED.,.F.,.F.,(3,3),(0.,1.),.UNSPECIFIED.);
#24147=B_SPLINE_CURVE_WITH_KNOTS('',2,(#85707,#85708,#85709),
 .UNSPECIFIED.,.F.,.F.,(3,3),(0.,1.),.UNSPECIFIED.);
#24148=B_SPLINE_CURVE_WITH_KNOTS('',2,(#85717,#85718,#85719),
 .UNSPECIFIED.,.F.,.F.,(3,3),(0.,1.),.UNSPECIFIED.);
#24149=B_SPLINE_CURVE_WITH_KNOTS('',2,(#85722,#85723,#85724),
 .UNSPECIFIED.,.F.,.F.,(3,3),(0.,1.),.UNSPECIFIED.);
#24150=B_SPLINE_CURVE_WITH_KNOTS('',2,(#85731,#85732,#85733),
 .UNSPECIFIED.,.F.,.F.,(3,3),(0.,1.),.UNSPECIFIED.);
#24151=B_SPLINE_CURVE_WITH_KNOTS('',2,(#85734,#85735,#85736),
 .UNSPECIFIED.,.F.,.F.,(3,3),(0.,1.),.UNSPECIFIED.);
#24152=B_SPLINE_CURVE_WITH_KNOTS('',2,(#85745,#85746,#85747),
 .UNSPECIFIED.,.F.,.F.,(3,3),(0.,1.),.UNSPECIFIED.);
#24153=B_SPLINE_CURVE_WITH_KNOTS('',2,(#85751,#85752,#85753),
 .UNSPECIFIED.,.F.,.F.,(3,3),(0.,1.),.UNSPECIFIED.);
#24154=B_SPLINE_CURVE_WITH_KNOTS('',2,(#85762,#85763,#85764),
 .UNSPECIFIED.,.F.,.F.,(3,3),(0.,1.),.UNSPECIFIED.);
#24155=B_SPLINE_CURVE_WITH_KNOTS('',2,(#85767,#85768,#85769),
 .UNSPECIFIED.,.F.,.F.,(3,3),(0.,1.),.UNSPECIFIED.);
#24156=B_SPLINE_CURVE_WITH_KNOTS('',2,(#85777,#85778,#85779),
 .UNSPECIFIED.,.F.,.F.,(3,3),(0.,1.),.UNSPECIFIED.);
#24157=B_SPLINE_CURVE_WITH_KNOTS('',2,(#85782,#85783,#85784),
 .UNSPECIFIED.,.F.,.F.,(3,3),(0.,1.),.UNSPECIFIED.);
#24158=B_SPLINE_CURVE_WITH_KNOTS('',2,(#85792,#85793,#85794),
 .UNSPECIFIED.,.F.,.F.,(3,3),(0.,1.),.UNSPECIFIED.);
#24159=B_SPLINE_CURVE_WITH_KNOTS('',2,(#85797,#85798,#85799),
 .UNSPECIFIED.,.F.,.F.,(3,3),(0.,1.),.UNSPECIFIED.);
#24160=B_SPLINE_CURVE_WITH_KNOTS('',2,(#85807,#85808,#85809),
 .UNSPECIFIED.,.F.,.F.,(3,3),(0.,1.),.UNSPECIFIED.);
#24161=B_SPLINE_CURVE_WITH_KNOTS('',2,(#85812,#85813,#85814),
 .UNSPECIFIED.,.F.,.F.,(3,3),(0.,1.),.UNSPECIFIED.);
#24162=B_SPLINE_CURVE_WITH_KNOTS('',2,(#85822,#85823,#85824),
 .UNSPECIFIED.,.F.,.F.,(3,3),(0.,1.),.UNSPECIFIED.);
#24163=B_SPLINE_CURVE_WITH_KNOTS('',2,(#85827,#85828,#85829),
 .UNSPECIFIED.,.F.,.F.,(3,3),(0.,1.),.UNSPECIFIED.);
#24164=B_SPLINE_CURVE_WITH_KNOTS('',2,(#85837,#85838,#85839),
 .UNSPECIFIED.,.F.,.F.,(3,3),(0.,1.),.UNSPECIFIED.);
#24165=B_SPLINE_CURVE_WITH_KNOTS('',2,(#85842,#85843,#85844),
 .UNSPECIFIED.,.F.,.F.,(3,3),(0.,1.),.UNSPECIFIED.);
#24166=B_SPLINE_CURVE_WITH_KNOTS('',2,(#85852,#85853,#85854),
 .UNSPECIFIED.,.F.,.F.,(3,3),(0.,1.),.UNSPECIFIED.);
#24167=B_SPLINE_CURVE_WITH_KNOTS('',2,(#85857,#85858,#85859),
 .UNSPECIFIED.,.F.,.F.,(3,3),(0.,1.),.UNSPECIFIED.);
#24168=B_SPLINE_CURVE_WITH_KNOTS('',2,(#85867,#85868,#85869),
 .UNSPECIFIED.,.F.,.F.,(3,3),(0.,1.),.UNSPECIFIED.);
#24169=B_SPLINE_CURVE_WITH_KNOTS('',2,(#85872,#85873,#85874),
 .UNSPECIFIED.,.F.,.F.,(3,3),(0.,1.),.UNSPECIFIED.);
#24170=B_SPLINE_CURVE_WITH_KNOTS('',2,(#85882,#85883,#85884),
 .UNSPECIFIED.,.F.,.F.,(3,3),(0.,1.),.UNSPECIFIED.);
#24171=B_SPLINE_CURVE_WITH_KNOTS('',2,(#85887,#85888,#85889),
 .UNSPECIFIED.,.F.,.F.,(3,3),(0.,1.),.UNSPECIFIED.);
#24172=B_SPLINE_CURVE_WITH_KNOTS('',2,(#85897,#85898,#85899),
 .UNSPECIFIED.,.F.,.F.,(3,3),(0.,1.),.UNSPECIFIED.);
#24173=B_SPLINE_CURVE_WITH_KNOTS('',2,(#85902,#85903,#85904),
 .UNSPECIFIED.,.F.,.F.,(3,3),(0.,1.),.UNSPECIFIED.);
#24174=B_SPLINE_CURVE_WITH_KNOTS('',2,(#85911,#85912,#85913),
 .UNSPECIFIED.,.F.,.F.,(3,3),(0.,1.),.UNSPECIFIED.);
#24175=B_SPLINE_CURVE_WITH_KNOTS('',2,(#85914,#85915,#85916),
 .UNSPECIFIED.,.F.,.F.,(3,3),(0.,1.),.UNSPECIFIED.);
#24176=B_SPLINE_CURVE_WITH_KNOTS('',2,(#85926,#85927,#85928),
 .UNSPECIFIED.,.F.,.F.,(3,3),(0.,1.),.UNSPECIFIED.);
#24177=B_SPLINE_CURVE_WITH_KNOTS('',2,(#85932,#85933,#85934),
 .UNSPECIFIED.,.F.,.F.,(3,3),(0.,1.),.UNSPECIFIED.);
#24178=B_SPLINE_CURVE_WITH_KNOTS('',2,(#85943,#85944,#85945),
 .UNSPECIFIED.,.F.,.F.,(3,3),(0.,1.),.UNSPECIFIED.);
#24179=B_SPLINE_CURVE_WITH_KNOTS('',2,(#85948,#85949,#85950),
 .UNSPECIFIED.,.F.,.F.,(3,3),(0.,1.),.UNSPECIFIED.);
#24180=B_SPLINE_CURVE_WITH_KNOTS('',2,(#85958,#85959,#85960),
 .UNSPECIFIED.,.F.,.F.,(3,3),(0.,1.),.UNSPECIFIED.);
#24181=B_SPLINE_CURVE_WITH_KNOTS('',2,(#85963,#85964,#85965),
 .UNSPECIFIED.,.F.,.F.,(3,3),(0.,1.),.UNSPECIFIED.);
#24182=B_SPLINE_CURVE_WITH_KNOTS('',2,(#85973,#85974,#85975),
 .UNSPECIFIED.,.F.,.F.,(3,3),(0.,1.),.UNSPECIFIED.);
#24183=B_SPLINE_CURVE_WITH_KNOTS('',2,(#85978,#85979,#85980),
 .UNSPECIFIED.,.F.,.F.,(3,3),(0.,1.),.UNSPECIFIED.);
#24184=B_SPLINE_CURVE_WITH_KNOTS('',2,(#85988,#85989,#85990),
 .UNSPECIFIED.,.F.,.F.,(3,3),(0.,1.),.UNSPECIFIED.);
#24185=B_SPLINE_CURVE_WITH_KNOTS('',2,(#85993,#85994,#85995),
 .UNSPECIFIED.,.F.,.F.,(3,3),(0.,1.),.UNSPECIFIED.);
#24186=B_SPLINE_CURVE_WITH_KNOTS('',2,(#86003,#86004,#86005),
 .UNSPECIFIED.,.F.,.F.,(3,3),(0.,1.),.UNSPECIFIED.);
#24187=B_SPLINE_CURVE_WITH_KNOTS('',2,(#86008,#86009,#86010),
 .UNSPECIFIED.,.F.,.F.,(3,3),(0.,1.),.UNSPECIFIED.);
#24188=B_SPLINE_CURVE_WITH_KNOTS('',2,(#86018,#86019,#86020),
 .UNSPECIFIED.,.F.,.F.,(3,3),(0.,1.),.UNSPECIFIED.);
#24189=B_SPLINE_CURVE_WITH_KNOTS('',2,(#86023,#86024,#86025),
 .UNSPECIFIED.,.F.,.F.,(3,3),(0.,1.),.UNSPECIFIED.);
#24190=B_SPLINE_CURVE_WITH_KNOTS('',2,(#86032,#86033,#86034),
 .UNSPECIFIED.,.F.,.F.,(3,3),(0.,1.),.UNSPECIFIED.);
#24191=B_SPLINE_CURVE_WITH_KNOTS('',2,(#86035,#86036,#86037),
 .UNSPECIFIED.,.F.,.F.,(3,3),(0.,1.),.UNSPECIFIED.);
#24192=B_SPLINE_CURVE_WITH_KNOTS('',2,(#86046,#86047,#86048),
 .UNSPECIFIED.,.F.,.F.,(3,3),(0.,1.),.UNSPECIFIED.);
#24193=B_SPLINE_CURVE_WITH_KNOTS('',2,(#86052,#86053,#86054),
 .UNSPECIFIED.,.F.,.F.,(3,3),(0.,1.),.UNSPECIFIED.);
#24194=B_SPLINE_CURVE_WITH_KNOTS('',2,(#86063,#86064,#86065),
 .UNSPECIFIED.,.F.,.F.,(3,3),(0.,1.),.UNSPECIFIED.);
#24195=B_SPLINE_CURVE_WITH_KNOTS('',2,(#86068,#86069,#86070),
 .UNSPECIFIED.,.F.,.F.,(3,3),(0.,1.),.UNSPECIFIED.);
#24196=B_SPLINE_CURVE_WITH_KNOTS('',2,(#86078,#86079,#86080),
 .UNSPECIFIED.,.F.,.F.,(3,3),(0.,1.),.UNSPECIFIED.);
#24197=B_SPLINE_CURVE_WITH_KNOTS('',2,(#86083,#86084,#86085),
 .UNSPECIFIED.,.F.,.F.,(3,3),(0.,1.),.UNSPECIFIED.);
#24198=B_SPLINE_CURVE_WITH_KNOTS('',2,(#86093,#86094,#86095),
 .UNSPECIFIED.,.F.,.F.,(3,3),(0.,1.),.UNSPECIFIED.);
#24199=B_SPLINE_CURVE_WITH_KNOTS('',2,(#86098,#86099,#86100),
 .UNSPECIFIED.,.F.,.F.,(3,3),(0.,1.),.UNSPECIFIED.);
#24200=B_SPLINE_CURVE_WITH_KNOTS('',2,(#86108,#86109,#86110),
 .UNSPECIFIED.,.F.,.F.,(3,3),(0.,1.),.UNSPECIFIED.);
#24201=B_SPLINE_CURVE_WITH_KNOTS('',2,(#86113,#86114,#86115),
 .UNSPECIFIED.,.F.,.F.,(3,3),(0.,1.),.UNSPECIFIED.);
#24202=B_SPLINE_CURVE_WITH_KNOTS('',2,(#86123,#86124,#86125),
 .UNSPECIFIED.,.F.,.F.,(3,3),(0.,1.),.UNSPECIFIED.);
#24203=B_SPLINE_CURVE_WITH_KNOTS('',2,(#86128,#86129,#86130),
 .UNSPECIFIED.,.F.,.F.,(3,3),(0.,1.),.UNSPECIFIED.);
#24204=B_SPLINE_CURVE_WITH_KNOTS('',2,(#86138,#86139,#86140),
 .UNSPECIFIED.,.F.,.F.,(3,3),(0.,1.),.UNSPECIFIED.);
#24205=B_SPLINE_CURVE_WITH_KNOTS('',2,(#86143,#86144,#86145),
 .UNSPECIFIED.,.F.,.F.,(3,3),(0.,1.),.UNSPECIFIED.);
#24206=B_SPLINE_CURVE_WITH_KNOTS('',2,(#86153,#86154,#86155),
 .UNSPECIFIED.,.F.,.F.,(3,3),(0.,1.),.UNSPECIFIED.);
#24207=B_SPLINE_CURVE_WITH_KNOTS('',2,(#86158,#86159,#86160),
 .UNSPECIFIED.,.F.,.F.,(3,3),(0.,1.),.UNSPECIFIED.);
#24208=B_SPLINE_CURVE_WITH_KNOTS('',2,(#86167,#86168,#86169),
 .UNSPECIFIED.,.F.,.F.,(3,3),(0.,1.),.UNSPECIFIED.);
#24209=B_SPLINE_CURVE_WITH_KNOTS('',2,(#86170,#86171,#86172),
 .UNSPECIFIED.,.F.,.F.,(3,3),(0.,1.),.UNSPECIFIED.);
#24210=B_SPLINE_CURVE_WITH_KNOTS('',2,(#86181,#86182,#86183),
 .UNSPECIFIED.,.F.,.F.,(3,3),(0.,1.),.UNSPECIFIED.);
#24211=B_SPLINE_CURVE_WITH_KNOTS('',2,(#86187,#86188,#86189),
 .UNSPECIFIED.,.F.,.F.,(3,3),(0.,1.),.UNSPECIFIED.);
#24212=B_SPLINE_CURVE_WITH_KNOTS('',2,(#86198,#86199,#86200),
 .UNSPECIFIED.,.F.,.F.,(3,3),(0.,1.),.UNSPECIFIED.);
#24213=B_SPLINE_CURVE_WITH_KNOTS('',2,(#86203,#86204,#86205),
 .UNSPECIFIED.,.F.,.F.,(3,3),(0.,1.),.UNSPECIFIED.);
#24214=B_SPLINE_CURVE_WITH_KNOTS('',2,(#86213,#86214,#86215),
 .UNSPECIFIED.,.F.,.F.,(3,3),(0.,1.),.UNSPECIFIED.);
#24215=B_SPLINE_CURVE_WITH_KNOTS('',2,(#86218,#86219,#86220),
 .UNSPECIFIED.,.F.,.F.,(3,3),(0.,1.),.UNSPECIFIED.);
#24216=B_SPLINE_CURVE_WITH_KNOTS('',2,(#86228,#86229,#86230),
 .UNSPECIFIED.,.F.,.F.,(3,3),(0.,1.),.UNSPECIFIED.);
#24217=B_SPLINE_CURVE_WITH_KNOTS('',2,(#86233,#86234,#86235),
 .UNSPECIFIED.,.F.,.F.,(3,3),(0.,1.),.UNSPECIFIED.);
#24218=B_SPLINE_CURVE_WITH_KNOTS('',2,(#86243,#86244,#86245),
 .UNSPECIFIED.,.F.,.F.,(3,3),(0.,1.),.UNSPECIFIED.);
#24219=B_SPLINE_CURVE_WITH_KNOTS('',2,(#86248,#86249,#86250),
 .UNSPECIFIED.,.F.,.F.,(3,3),(0.,1.),.UNSPECIFIED.);
#24220=B_SPLINE_CURVE_WITH_KNOTS('',2,(#86258,#86259,#86260),
 .UNSPECIFIED.,.F.,.F.,(3,3),(0.,1.),.UNSPECIFIED.);
#24221=B_SPLINE_CURVE_WITH_KNOTS('',2,(#86263,#86264,#86265),
 .UNSPECIFIED.,.F.,.F.,(3,3),(0.,1.),.UNSPECIFIED.);
#24222=B_SPLINE_CURVE_WITH_KNOTS('',2,(#86273,#86274,#86275),
 .UNSPECIFIED.,.F.,.F.,(3,3),(0.,1.),.UNSPECIFIED.);
#24223=B_SPLINE_CURVE_WITH_KNOTS('',2,(#86278,#86279,#86280),
 .UNSPECIFIED.,.F.,.F.,(3,3),(0.,1.),.UNSPECIFIED.);
#24224=B_SPLINE_CURVE_WITH_KNOTS('',2,(#86288,#86289,#86290),
 .UNSPECIFIED.,.F.,.F.,(3,3),(0.,1.),.UNSPECIFIED.);
#24225=B_SPLINE_CURVE_WITH_KNOTS('',2,(#86293,#86294,#86295),
 .UNSPECIFIED.,.F.,.F.,(3,3),(0.,1.),.UNSPECIFIED.);
#24226=B_SPLINE_CURVE_WITH_KNOTS('',2,(#86303,#86304,#86305),
 .UNSPECIFIED.,.F.,.F.,(3,3),(0.,1.),.UNSPECIFIED.);
#24227=B_SPLINE_CURVE_WITH_KNOTS('',2,(#86308,#86309,#86310),
 .UNSPECIFIED.,.F.,.F.,(3,3),(0.,1.),.UNSPECIFIED.);
#24228=B_SPLINE_CURVE_WITH_KNOTS('',2,(#86318,#86319,#86320),
 .UNSPECIFIED.,.F.,.F.,(3,3),(0.,1.),.UNSPECIFIED.);
#24229=B_SPLINE_CURVE_WITH_KNOTS('',2,(#86323,#86324,#86325),
 .UNSPECIFIED.,.F.,.F.,(3,3),(0.,1.),.UNSPECIFIED.);
#24230=B_SPLINE_CURVE_WITH_KNOTS('',2,(#86333,#86334,#86335),
 .UNSPECIFIED.,.F.,.F.,(3,3),(0.,1.),.UNSPECIFIED.);
#24231=B_SPLINE_CURVE_WITH_KNOTS('',2,(#86338,#86339,#86340),
 .UNSPECIFIED.,.F.,.F.,(3,3),(0.,1.),.UNSPECIFIED.);
#24232=B_SPLINE_CURVE_WITH_KNOTS('',2,(#86348,#86349,#86350),
 .UNSPECIFIED.,.F.,.F.,(3,3),(0.,1.),.UNSPECIFIED.);
#24233=B_SPLINE_CURVE_WITH_KNOTS('',2,(#86353,#86354,#86355),
 .UNSPECIFIED.,.F.,.F.,(3,3),(0.,1.),.UNSPECIFIED.);
#24234=B_SPLINE_CURVE_WITH_KNOTS('',2,(#86363,#86364,#86365),
 .UNSPECIFIED.,.F.,.F.,(3,3),(0.,1.),.UNSPECIFIED.);
#24235=B_SPLINE_CURVE_WITH_KNOTS('',2,(#86368,#86369,#86370),
 .UNSPECIFIED.,.F.,.F.,(3,3),(0.,1.),.UNSPECIFIED.);
#24236=B_SPLINE_CURVE_WITH_KNOTS('',2,(#86378,#86379,#86380),
 .UNSPECIFIED.,.F.,.F.,(3,3),(0.,1.),.UNSPECIFIED.);
#24237=B_SPLINE_CURVE_WITH_KNOTS('',2,(#86383,#86384,#86385),
 .UNSPECIFIED.,.F.,.F.,(3,3),(0.,1.),.UNSPECIFIED.);
#24238=B_SPLINE_CURVE_WITH_KNOTS('',2,(#86393,#86394,#86395),
 .UNSPECIFIED.,.F.,.F.,(3,3),(0.,1.),.UNSPECIFIED.);
#24239=B_SPLINE_CURVE_WITH_KNOTS('',2,(#86398,#86399,#86400),
 .UNSPECIFIED.,.F.,.F.,(3,3),(0.,1.),.UNSPECIFIED.);
#24240=B_SPLINE_CURVE_WITH_KNOTS('',2,(#86407,#86408,#86409),
 .UNSPECIFIED.,.F.,.F.,(3,3),(0.,1.),.UNSPECIFIED.);
#24241=B_SPLINE_CURVE_WITH_KNOTS('',2,(#86410,#86411,#86412),
 .UNSPECIFIED.,.F.,.F.,(3,3),(0.,1.),.UNSPECIFIED.);
#24242=B_SPLINE_CURVE_WITH_KNOTS('',2,(#86425,#86426,#86427),
 .UNSPECIFIED.,.F.,.F.,(3,3),(0.,1.),.UNSPECIFIED.);
#24243=B_SPLINE_CURVE_WITH_KNOTS('',2,(#86431,#86432,#86433),
 .UNSPECIFIED.,.F.,.F.,(3,3),(0.,1.),.UNSPECIFIED.);
#24244=B_SPLINE_CURVE_WITH_KNOTS('',2,(#86442,#86443,#86444),
 .UNSPECIFIED.,.F.,.F.,(3,3),(0.,1.),.UNSPECIFIED.);
#24245=B_SPLINE_CURVE_WITH_KNOTS('',2,(#86447,#86448,#86449),
 .UNSPECIFIED.,.F.,.F.,(3,3),(0.,1.),.UNSPECIFIED.);
#24246=B_SPLINE_CURVE_WITH_KNOTS('',2,(#86457,#86458,#86459),
 .UNSPECIFIED.,.F.,.F.,(3,3),(0.,1.),.UNSPECIFIED.);
#24247=B_SPLINE_CURVE_WITH_KNOTS('',2,(#86462,#86463,#86464),
 .UNSPECIFIED.,.F.,.F.,(3,3),(0.,1.),.UNSPECIFIED.);
#24248=B_SPLINE_CURVE_WITH_KNOTS('',2,(#86472,#86473,#86474),
 .UNSPECIFIED.,.F.,.F.,(3,3),(0.,1.),.UNSPECIFIED.);
#24249=B_SPLINE_CURVE_WITH_KNOTS('',2,(#86477,#86478,#86479),
 .UNSPECIFIED.,.F.,.F.,(3,3),(0.,1.),.UNSPECIFIED.);
#24250=B_SPLINE_CURVE_WITH_KNOTS('',2,(#86487,#86488,#86489),
 .UNSPECIFIED.,.F.,.F.,(3,3),(0.,1.),.UNSPECIFIED.);
#24251=B_SPLINE_CURVE_WITH_KNOTS('',2,(#86492,#86493,#86494),
 .UNSPECIFIED.,.F.,.F.,(3,3),(0.,1.),.UNSPECIFIED.);
#24252=B_SPLINE_CURVE_WITH_KNOTS('',2,(#86502,#86503,#86504),
 .UNSPECIFIED.,.F.,.F.,(3,3),(0.,1.),.UNSPECIFIED.);
#24253=B_SPLINE_CURVE_WITH_KNOTS('',2,(#86507,#86508,#86509),
 .UNSPECIFIED.,.F.,.F.,(3,3),(0.,1.),.UNSPECIFIED.);
#24254=B_SPLINE_CURVE_WITH_KNOTS('',2,(#86517,#86518,#86519),
 .UNSPECIFIED.,.F.,.F.,(3,3),(0.,1.),.UNSPECIFIED.);
#24255=B_SPLINE_CURVE_WITH_KNOTS('',2,(#86522,#86523,#86524),
 .UNSPECIFIED.,.F.,.F.,(3,3),(0.,1.),.UNSPECIFIED.);
#24256=B_SPLINE_CURVE_WITH_KNOTS('',2,(#86531,#86532,#86533),
 .UNSPECIFIED.,.F.,.F.,(3,3),(0.,1.),.UNSPECIFIED.);
#24257=B_SPLINE_CURVE_WITH_KNOTS('',2,(#86534,#86535,#86536),
 .UNSPECIFIED.,.F.,.F.,(3,3),(0.,1.),.UNSPECIFIED.);
#24258=B_SPLINE_CURVE_WITH_KNOTS('',2,(#86545,#86546,#86547),
 .UNSPECIFIED.,.F.,.F.,(3,3),(0.,1.),.UNSPECIFIED.);
#24259=B_SPLINE_CURVE_WITH_KNOTS('',2,(#86551,#86552,#86553),
 .UNSPECIFIED.,.F.,.F.,(3,3),(0.,1.),.UNSPECIFIED.);
#24260=B_SPLINE_CURVE_WITH_KNOTS('',2,(#86562,#86563,#86564),
 .UNSPECIFIED.,.F.,.F.,(3,3),(0.,1.),.UNSPECIFIED.);
#24261=B_SPLINE_CURVE_WITH_KNOTS('',2,(#86567,#86568,#86569),
 .UNSPECIFIED.,.F.,.F.,(3,3),(0.,1.),.UNSPECIFIED.);
#24262=B_SPLINE_CURVE_WITH_KNOTS('',2,(#86577,#86578,#86579),
 .UNSPECIFIED.,.F.,.F.,(3,3),(0.,1.),.UNSPECIFIED.);
#24263=B_SPLINE_CURVE_WITH_KNOTS('',2,(#86582,#86583,#86584),
 .UNSPECIFIED.,.F.,.F.,(3,3),(0.,1.),.UNSPECIFIED.);
#24264=B_SPLINE_CURVE_WITH_KNOTS('',2,(#86592,#86593,#86594),
 .UNSPECIFIED.,.F.,.F.,(3,3),(0.,1.),.UNSPECIFIED.);
#24265=B_SPLINE_CURVE_WITH_KNOTS('',2,(#86597,#86598,#86599),
 .UNSPECIFIED.,.F.,.F.,(3,3),(0.,1.),.UNSPECIFIED.);
#24266=B_SPLINE_CURVE_WITH_KNOTS('',2,(#86607,#86608,#86609),
 .UNSPECIFIED.,.F.,.F.,(3,3),(0.,1.),.UNSPECIFIED.);
#24267=B_SPLINE_CURVE_WITH_KNOTS('',2,(#86612,#86613,#86614),
 .UNSPECIFIED.,.F.,.F.,(3,3),(0.,1.),.UNSPECIFIED.);
#24268=B_SPLINE_CURVE_WITH_KNOTS('',2,(#86622,#86623,#86624),
 .UNSPECIFIED.,.F.,.F.,(3,3),(0.,1.),.UNSPECIFIED.);
#24269=B_SPLINE_CURVE_WITH_KNOTS('',2,(#86627,#86628,#86629),
 .UNSPECIFIED.,.F.,.F.,(3,3),(0.,1.),.UNSPECIFIED.);
#24270=B_SPLINE_CURVE_WITH_KNOTS('',2,(#86637,#86638,#86639),
 .UNSPECIFIED.,.F.,.F.,(3,3),(0.,1.),.UNSPECIFIED.);
#24271=B_SPLINE_CURVE_WITH_KNOTS('',2,(#86642,#86643,#86644),
 .UNSPECIFIED.,.F.,.F.,(3,3),(0.,1.),.UNSPECIFIED.);
#24272=B_SPLINE_CURVE_WITH_KNOTS('',2,(#86652,#86653,#86654),
 .UNSPECIFIED.,.F.,.F.,(3,3),(0.,1.),.UNSPECIFIED.);
#24273=B_SPLINE_CURVE_WITH_KNOTS('',2,(#86657,#86658,#86659),
 .UNSPECIFIED.,.F.,.F.,(3,3),(0.,1.),.UNSPECIFIED.);
#24274=B_SPLINE_CURVE_WITH_KNOTS('',2,(#86667,#86668,#86669),
 .UNSPECIFIED.,.F.,.F.,(3,3),(0.,1.),.UNSPECIFIED.);
#24275=B_SPLINE_CURVE_WITH_KNOTS('',2,(#86672,#86673,#86674),
 .UNSPECIFIED.,.F.,.F.,(3,3),(0.,1.),.UNSPECIFIED.);
#24276=B_SPLINE_CURVE_WITH_KNOTS('',2,(#86682,#86683,#86684),
 .UNSPECIFIED.,.F.,.F.,(3,3),(0.,1.),.UNSPECIFIED.);
#24277=B_SPLINE_CURVE_WITH_KNOTS('',2,(#86687,#86688,#86689),
 .UNSPECIFIED.,.F.,.F.,(3,3),(0.,1.),.UNSPECIFIED.);
#24278=B_SPLINE_CURVE_WITH_KNOTS('',2,(#86697,#86698,#86699),
 .UNSPECIFIED.,.F.,.F.,(3,3),(0.,1.),.UNSPECIFIED.);
#24279=B_SPLINE_CURVE_WITH_KNOTS('',2,(#86702,#86703,#86704),
 .UNSPECIFIED.,.F.,.F.,(3,3),(0.,1.),.UNSPECIFIED.);
#24280=B_SPLINE_CURVE_WITH_KNOTS('',2,(#86711,#86712,#86713),
 .UNSPECIFIED.,.F.,.F.,(3,3),(0.,1.),.UNSPECIFIED.);
#24281=B_SPLINE_CURVE_WITH_KNOTS('',2,(#86714,#86715,#86716),
 .UNSPECIFIED.,.F.,.F.,(3,3),(0.,1.),.UNSPECIFIED.);
#24282=B_SPLINE_CURVE_WITH_KNOTS('',2,(#86726,#86727,#86728),
 .UNSPECIFIED.,.F.,.F.,(3,3),(0.,1.),.UNSPECIFIED.);
#24283=B_SPLINE_CURVE_WITH_KNOTS('',2,(#86732,#86733,#86734),
 .UNSPECIFIED.,.F.,.F.,(3,3),(0.,1.),.UNSPECIFIED.);
#24284=B_SPLINE_CURVE_WITH_KNOTS('',2,(#86743,#86744,#86745),
 .UNSPECIFIED.,.F.,.F.,(3,3),(0.,1.),.UNSPECIFIED.);
#24285=B_SPLINE_CURVE_WITH_KNOTS('',2,(#86748,#86749,#86750),
 .UNSPECIFIED.,.F.,.F.,(3,3),(0.,1.),.UNSPECIFIED.);
#24286=B_SPLINE_CURVE_WITH_KNOTS('',2,(#86758,#86759,#86760),
 .UNSPECIFIED.,.F.,.F.,(3,3),(0.,1.),.UNSPECIFIED.);
#24287=B_SPLINE_CURVE_WITH_KNOTS('',2,(#86763,#86764,#86765),
 .UNSPECIFIED.,.F.,.F.,(3,3),(0.,1.),.UNSPECIFIED.);
#24288=B_SPLINE_CURVE_WITH_KNOTS('',2,(#86773,#86774,#86775),
 .UNSPECIFIED.,.F.,.F.,(3,3),(0.,1.),.UNSPECIFIED.);
#24289=B_SPLINE_CURVE_WITH_KNOTS('',2,(#86778,#86779,#86780),
 .UNSPECIFIED.,.F.,.F.,(3,3),(0.,1.),.UNSPECIFIED.);
#24290=B_SPLINE_CURVE_WITH_KNOTS('',2,(#86788,#86789,#86790),
 .UNSPECIFIED.,.F.,.F.,(3,3),(0.,1.),.UNSPECIFIED.);
#24291=B_SPLINE_CURVE_WITH_KNOTS('',2,(#86793,#86794,#86795),
 .UNSPECIFIED.,.F.,.F.,(3,3),(0.,1.),.UNSPECIFIED.);
#24292=B_SPLINE_CURVE_WITH_KNOTS('',2,(#86803,#86804,#86805),
 .UNSPECIFIED.,.F.,.F.,(3,3),(0.,1.),.UNSPECIFIED.);
#24293=B_SPLINE_CURVE_WITH_KNOTS('',2,(#86808,#86809,#86810),
 .UNSPECIFIED.,.F.,.F.,(3,3),(0.,1.),.UNSPECIFIED.);
#24294=B_SPLINE_CURVE_WITH_KNOTS('',2,(#86818,#86819,#86820),
 .UNSPECIFIED.,.F.,.F.,(3,3),(0.,1.),.UNSPECIFIED.);
#24295=B_SPLINE_CURVE_WITH_KNOTS('',2,(#86823,#86824,#86825),
 .UNSPECIFIED.,.F.,.F.,(3,3),(0.,1.),.UNSPECIFIED.);
#24296=B_SPLINE_CURVE_WITH_KNOTS('',2,(#86832,#86833,#86834),
 .UNSPECIFIED.,.F.,.F.,(3,3),(0.,1.),.UNSPECIFIED.);
#24297=B_SPLINE_CURVE_WITH_KNOTS('',2,(#86835,#86836,#86837),
 .UNSPECIFIED.,.F.,.F.,(3,3),(0.,1.),.UNSPECIFIED.);
#24298=B_SPLINE_CURVE_WITH_KNOTS('',2,(#86846,#86847,#86848),
 .UNSPECIFIED.,.F.,.F.,(3,3),(0.,1.),.UNSPECIFIED.);
#24299=B_SPLINE_CURVE_WITH_KNOTS('',2,(#86852,#86853,#86854),
 .UNSPECIFIED.,.F.,.F.,(3,3),(0.,1.),.UNSPECIFIED.);
#24300=B_SPLINE_CURVE_WITH_KNOTS('',2,(#86863,#86864,#86865),
 .UNSPECIFIED.,.F.,.F.,(3,3),(0.,1.),.UNSPECIFIED.);
#24301=B_SPLINE_CURVE_WITH_KNOTS('',2,(#86868,#86869,#86870),
 .UNSPECIFIED.,.F.,.F.,(3,3),(0.,1.),.UNSPECIFIED.);
#24302=B_SPLINE_CURVE_WITH_KNOTS('',2,(#86878,#86879,#86880),
 .UNSPECIFIED.,.F.,.F.,(3,3),(0.,1.),.UNSPECIFIED.);
#24303=B_SPLINE_CURVE_WITH_KNOTS('',2,(#86883,#86884,#86885),
 .UNSPECIFIED.,.F.,.F.,(3,3),(0.,1.),.UNSPECIFIED.);
#24304=B_SPLINE_CURVE_WITH_KNOTS('',2,(#86893,#86894,#86895),
 .UNSPECIFIED.,.F.,.F.,(3,3),(0.,1.),.UNSPECIFIED.);
#24305=B_SPLINE_CURVE_WITH_KNOTS('',2,(#86898,#86899,#86900),
 .UNSPECIFIED.,.F.,.F.,(3,3),(0.,1.),.UNSPECIFIED.);
#24306=B_SPLINE_CURVE_WITH_KNOTS('',2,(#86908,#86909,#86910),
 .UNSPECIFIED.,.F.,.F.,(3,3),(0.,1.),.UNSPECIFIED.);
#24307=B_SPLINE_CURVE_WITH_KNOTS('',2,(#86913,#86914,#86915),
 .UNSPECIFIED.,.F.,.F.,(3,3),(0.,1.),.UNSPECIFIED.);
#24308=B_SPLINE_CURVE_WITH_KNOTS('',2,(#86923,#86924,#86925),
 .UNSPECIFIED.,.F.,.F.,(3,3),(0.,1.),.UNSPECIFIED.);
#24309=B_SPLINE_CURVE_WITH_KNOTS('',2,(#86928,#86929,#86930),
 .UNSPECIFIED.,.F.,.F.,(3,3),(0.,1.),.UNSPECIFIED.);
#24310=B_SPLINE_CURVE_WITH_KNOTS('',2,(#86938,#86939,#86940),
 .UNSPECIFIED.,.F.,.F.,(3,3),(0.,1.),.UNSPECIFIED.);
#24311=B_SPLINE_CURVE_WITH_KNOTS('',2,(#86943,#86944,#86945),
 .UNSPECIFIED.,.F.,.F.,(3,3),(0.,1.),.UNSPECIFIED.);
#24312=B_SPLINE_CURVE_WITH_KNOTS('',2,(#86953,#86954,#86955),
 .UNSPECIFIED.,.F.,.F.,(3,3),(0.,1.),.UNSPECIFIED.);
#24313=B_SPLINE_CURVE_WITH_KNOTS('',2,(#86958,#86959,#86960),
 .UNSPECIFIED.,.F.,.F.,(3,3),(0.,1.),.UNSPECIFIED.);
#24314=B_SPLINE_CURVE_WITH_KNOTS('',2,(#86968,#86969,#86970),
 .UNSPECIFIED.,.F.,.F.,(3,3),(0.,1.),.UNSPECIFIED.);
#24315=B_SPLINE_CURVE_WITH_KNOTS('',2,(#86973,#86974,#86975),
 .UNSPECIFIED.,.F.,.F.,(3,3),(0.,1.),.UNSPECIFIED.);
#24316=B_SPLINE_CURVE_WITH_KNOTS('',2,(#86983,#86984,#86985),
 .UNSPECIFIED.,.F.,.F.,(3,3),(0.,1.),.UNSPECIFIED.);
#24317=B_SPLINE_CURVE_WITH_KNOTS('',2,(#86988,#86989,#86990),
 .UNSPECIFIED.,.F.,.F.,(3,3),(0.,1.),.UNSPECIFIED.);
#24318=B_SPLINE_CURVE_WITH_KNOTS('',2,(#86998,#86999,#87000),
 .UNSPECIFIED.,.F.,.F.,(3,3),(0.,1.),.UNSPECIFIED.);
#24319=B_SPLINE_CURVE_WITH_KNOTS('',2,(#87003,#87004,#87005),
 .UNSPECIFIED.,.F.,.F.,(3,3),(0.,1.),.UNSPECIFIED.);
#24320=B_SPLINE_CURVE_WITH_KNOTS('',2,(#87013,#87014,#87015),
 .UNSPECIFIED.,.F.,.F.,(3,3),(0.,1.),.UNSPECIFIED.);
#24321=B_SPLINE_CURVE_WITH_KNOTS('',2,(#87018,#87019,#87020),
 .UNSPECIFIED.,.F.,.F.,(3,3),(0.,1.),.UNSPECIFIED.);
#24322=B_SPLINE_CURVE_WITH_KNOTS('',2,(#87028,#87029,#87030),
 .UNSPECIFIED.,.F.,.F.,(3,3),(0.,1.),.UNSPECIFIED.);
#24323=B_SPLINE_CURVE_WITH_KNOTS('',2,(#87033,#87034,#87035),
 .UNSPECIFIED.,.F.,.F.,(3,3),(0.,1.),.UNSPECIFIED.);
#24324=B_SPLINE_CURVE_WITH_KNOTS('',2,(#87043,#87044,#87045),
 .UNSPECIFIED.,.F.,.F.,(3,3),(0.,1.),.UNSPECIFIED.);
#24325=B_SPLINE_CURVE_WITH_KNOTS('',2,(#87048,#87049,#87050),
 .UNSPECIFIED.,.F.,.F.,(3,3),(0.,1.),.UNSPECIFIED.);
#24326=B_SPLINE_CURVE_WITH_KNOTS('',2,(#87058,#87059,#87060),
 .UNSPECIFIED.,.F.,.F.,(3,3),(0.,1.),.UNSPECIFIED.);
#24327=B_SPLINE_CURVE_WITH_KNOTS('',2,(#87063,#87064,#87065),
 .UNSPECIFIED.,.F.,.F.,(3,3),(0.,1.),.UNSPECIFIED.);
#24328=B_SPLINE_CURVE_WITH_KNOTS('',2,(#87073,#87074,#87075),
 .UNSPECIFIED.,.F.,.F.,(3,3),(0.,1.),.UNSPECIFIED.);
#24329=B_SPLINE_CURVE_WITH_KNOTS('',2,(#87078,#87079,#87080),
 .UNSPECIFIED.,.F.,.F.,(3,3),(0.,1.),.UNSPECIFIED.);
#24330=B_SPLINE_CURVE_WITH_KNOTS('',2,(#87088,#87089,#87090),
 .UNSPECIFIED.,.F.,.F.,(3,3),(0.,1.),.UNSPECIFIED.);
#24331=B_SPLINE_CURVE_WITH_KNOTS('',2,(#87093,#87094,#87095),
 .UNSPECIFIED.,.F.,.F.,(3,3),(0.,1.),.UNSPECIFIED.);
#24332=B_SPLINE_CURVE_WITH_KNOTS('',2,(#87103,#87104,#87105),
 .UNSPECIFIED.,.F.,.F.,(3,3),(0.,1.),.UNSPECIFIED.);
#24333=B_SPLINE_CURVE_WITH_KNOTS('',2,(#87108,#87109,#87110),
 .UNSPECIFIED.,.F.,.F.,(3,3),(0.,1.),.UNSPECIFIED.);
#24334=B_SPLINE_CURVE_WITH_KNOTS('',2,(#87118,#87119,#87120),
 .UNSPECIFIED.,.F.,.F.,(3,3),(0.,1.),.UNSPECIFIED.);
#24335=B_SPLINE_CURVE_WITH_KNOTS('',2,(#87123,#87124,#87125),
 .UNSPECIFIED.,.F.,.F.,(3,3),(0.,1.),.UNSPECIFIED.);
#24336=B_SPLINE_CURVE_WITH_KNOTS('',2,(#87133,#87134,#87135),
 .UNSPECIFIED.,.F.,.F.,(3,3),(0.,1.),.UNSPECIFIED.);
#24337=B_SPLINE_CURVE_WITH_KNOTS('',2,(#87138,#87139,#87140),
 .UNSPECIFIED.,.F.,.F.,(3,3),(0.,1.),.UNSPECIFIED.);
#24338=B_SPLINE_CURVE_WITH_KNOTS('',2,(#87153,#87154,#87155),
 .UNSPECIFIED.,.F.,.F.,(3,3),(0.,1.),.UNSPECIFIED.);
#24339=B_SPLINE_CURVE_WITH_KNOTS('',2,(#87156,#87157,#87158),
 .UNSPECIFIED.,.F.,.F.,(3,3),(0.,1.),.UNSPECIFIED.);
#24623=VERTEX_POINT('',#76152);
#24624=VERTEX_POINT('',#76153);
#24625=VERTEX_POINT('',#76157);
#24626=VERTEX_POINT('',#76159);
#24627=VERTEX_POINT('',#76170);
#24628=VERTEX_POINT('',#76174);
#24629=VERTEX_POINT('',#76185);
#24630=VERTEX_POINT('',#76189);
#24631=VERTEX_POINT('',#76200);
#24632=VERTEX_POINT('',#76204);
#24633=VERTEX_POINT('',#76215);
#24634=VERTEX_POINT('',#76219);
#24635=VERTEX_POINT('',#76230);
#24636=VERTEX_POINT('',#76234);
#24637=VERTEX_POINT('',#76245);
#24638=VERTEX_POINT('',#76249);
#24639=VERTEX_POINT('',#76272);
#24640=VERTEX_POINT('',#76273);
#24641=VERTEX_POINT('',#76277);
#24642=VERTEX_POINT('',#76279);
#24643=VERTEX_POINT('',#76290);
#24644=VERTEX_POINT('',#76294);
#24645=VERTEX_POINT('',#76305);
#24646=VERTEX_POINT('',#76309);
#24647=VERTEX_POINT('',#76320);
#24648=VERTEX_POINT('',#76324);
#24649=VERTEX_POINT('',#76335);
#24650=VERTEX_POINT('',#76339);
#24651=VERTEX_POINT('',#76350);
#24652=VERTEX_POINT('',#76354);
#24653=VERTEX_POINT('',#76365);
#24654=VERTEX_POINT('',#76369);
#24655=VERTEX_POINT('',#76380);
#24656=VERTEX_POINT('',#76384);
#24657=VERTEX_POINT('',#76395);
#24658=VERTEX_POINT('',#76399);
#24659=VERTEX_POINT('',#76410);
#24660=VERTEX_POINT('',#76414);
#24661=VERTEX_POINT('',#76425);
#24662=VERTEX_POINT('',#76429);
#24663=VERTEX_POINT('',#76453);
#24664=VERTEX_POINT('',#76454);
#24665=VERTEX_POINT('',#76458);
#24666=VERTEX_POINT('',#76460);
#24667=VERTEX_POINT('',#76471);
#24668=VERTEX_POINT('',#76475);
#24669=VERTEX_POINT('',#76486);
#24670=VERTEX_POINT('',#76490);
#24671=VERTEX_POINT('',#76501);
#24672=VERTEX_POINT('',#76505);
#24673=VERTEX_POINT('',#76516);
#24674=VERTEX_POINT('',#76520);
#24675=VERTEX_POINT('',#76531);
#24676=VERTEX_POINT('',#76535);
#24677=VERTEX_POINT('',#76546);
#24678=VERTEX_POINT('',#76550);
#24679=VERTEX_POINT('',#76573);
#24680=VERTEX_POINT('',#76574);
#24681=VERTEX_POINT('',#76578);
#24682=VERTEX_POINT('',#76580);
#24683=VERTEX_POINT('',#76591);
#24684=VERTEX_POINT('',#76595);
#24685=VERTEX_POINT('',#76606);
#24686=VERTEX_POINT('',#76610);
#24687=VERTEX_POINT('',#76621);
#24688=VERTEX_POINT('',#76625);
#24689=VERTEX_POINT('',#76636);
#24690=VERTEX_POINT('',#76640);
#24691=VERTEX_POINT('',#76651);
#24692=VERTEX_POINT('',#76655);
#24693=VERTEX_POINT('',#76666);
#24694=VERTEX_POINT('',#76670);
#24695=VERTEX_POINT('',#76681);
#24696=VERTEX_POINT('',#76685);
#24697=VERTEX_POINT('',#76696);
#24698=VERTEX_POINT('',#76700);
#24699=VERTEX_POINT('',#76711);
#24700=VERTEX_POINT('',#76715);
#24701=VERTEX_POINT('',#76726);
#24702=VERTEX_POINT('',#76730);
#24703=VERTEX_POINT('',#76741);
#24704=VERTEX_POINT('',#76745);
#24705=VERTEX_POINT('',#76756);
#24706=VERTEX_POINT('',#76760);
#24707=VERTEX_POINT('',#76771);
#24708=VERTEX_POINT('',#76775);
#24709=VERTEX_POINT('',#76786);
#24710=VERTEX_POINT('',#76790);
#24711=VERTEX_POINT('',#76801);
#24712=VERTEX_POINT('',#76805);
#24713=VERTEX_POINT('',#76816);
#24714=VERTEX_POINT('',#76820);
#24715=VERTEX_POINT('',#76831);
#24716=VERTEX_POINT('',#76835);
#24717=VERTEX_POINT('',#76846);
#24718=VERTEX_POINT('',#76850);
#24719=VERTEX_POINT('',#76861);
#24720=VERTEX_POINT('',#76865);
#24721=VERTEX_POINT('',#76871);
#24722=VERTEX_POINT('',#76873);
#24723=VERTEX_POINT('',#76897);
#24724=VERTEX_POINT('',#76898);
#24725=VERTEX_POINT('',#76902);
#24726=VERTEX_POINT('',#76904);
#24727=VERTEX_POINT('',#76915);
#24728=VERTEX_POINT('',#76919);
#24729=VERTEX_POINT('',#76930);
#24730=VERTEX_POINT('',#76934);
#24731=VERTEX_POINT('',#76945);
#24732=VERTEX_POINT('',#76949);
#24733=VERTEX_POINT('',#76960);
#24734=VERTEX_POINT('',#76964);
#24735=VERTEX_POINT('',#76975);
#24736=VERTEX_POINT('',#76979);
#24737=VERTEX_POINT('',#76990);
#24738=VERTEX_POINT('',#76994);
#24739=VERTEX_POINT('',#77017);
#24740=VERTEX_POINT('',#77018);
#24741=VERTEX_POINT('',#77022);
#24742=VERTEX_POINT('',#77024);
#24743=VERTEX_POINT('',#77035);
#24744=VERTEX_POINT('',#77039);
#24745=VERTEX_POINT('',#77050);
#24746=VERTEX_POINT('',#77054);
#24747=VERTEX_POINT('',#77065);
#24748=VERTEX_POINT('',#77069);
#24749=VERTEX_POINT('',#77080);
#24750=VERTEX_POINT('',#77084);
#24751=VERTEX_POINT('',#77095);
#24752=VERTEX_POINT('',#77099);
#24753=VERTEX_POINT('',#77110);
#24754=VERTEX_POINT('',#77114);
#24755=VERTEX_POINT('',#77125);
#24756=VERTEX_POINT('',#77129);
#24757=VERTEX_POINT('',#77140);
#24758=VERTEX_POINT('',#77144);
#24759=VERTEX_POINT('',#77155);
#24760=VERTEX_POINT('',#77159);
#24761=VERTEX_POINT('',#77170);
#24762=VERTEX_POINT('',#77174);
#24763=VERTEX_POINT('',#77198);
#24764=VERTEX_POINT('',#77199);
#24765=VERTEX_POINT('',#77203);
#24766=VERTEX_POINT('',#77205);
#24767=VERTEX_POINT('',#77216);
#24768=VERTEX_POINT('',#77220);
#24769=VERTEX_POINT('',#77231);
#24770=VERTEX_POINT('',#77235);
#24771=VERTEX_POINT('',#77246);
#24772=VERTEX_POINT('',#77250);
#24773=VERTEX_POINT('',#77261);
#24774=VERTEX_POINT('',#77265);
#24775=VERTEX_POINT('',#77276);
#24776=VERTEX_POINT('',#77280);
#24777=VERTEX_POINT('',#77291);
#24778=VERTEX_POINT('',#77295);
#24779=VERTEX_POINT('',#77318);
#24780=VERTEX_POINT('',#77319);
#24781=VERTEX_POINT('',#77323);
#24782=VERTEX_POINT('',#77325);
#24783=VERTEX_POINT('',#77336);
#24784=VERTEX_POINT('',#77340);
#24785=VERTEX_POINT('',#77351);
#24786=VERTEX_POINT('',#77355);
#24787=VERTEX_POINT('',#77366);
#24788=VERTEX_POINT('',#77370);
#24789=VERTEX_POINT('',#77381);
#24790=VERTEX_POINT('',#77385);
#24791=VERTEX_POINT('',#77396);
#24792=VERTEX_POINT('',#77400);
#24793=VERTEX_POINT('',#77411);
#24794=VERTEX_POINT('',#77415);
#24795=VERTEX_POINT('',#77426);
#24796=VERTEX_POINT('',#77430);
#24797=VERTEX_POINT('',#77453);
#24798=VERTEX_POINT('',#77454);
#24799=VERTEX_POINT('',#77458);
#24800=VERTEX_POINT('',#77460);
#24801=VERTEX_POINT('',#77471);
#24802=VERTEX_POINT('',#77475);
#24803=VERTEX_POINT('',#77486);
#24804=VERTEX_POINT('',#77490);
#24805=VERTEX_POINT('',#77501);
#24806=VERTEX_POINT('',#77505);
#24807=VERTEX_POINT('',#77516);
#24808=VERTEX_POINT('',#77520);
#24809=VERTEX_POINT('',#77531);
#24810=VERTEX_POINT('',#77535);
#24811=VERTEX_POINT('',#77546);
#24812=VERTEX_POINT('',#77550);
#24813=VERTEX_POINT('',#77561);
#24814=VERTEX_POINT('',#77565);
#24815=VERTEX_POINT('',#77576);
#24816=VERTEX_POINT('',#77580);
#24817=VERTEX_POINT('',#77591);
#24818=VERTEX_POINT('',#77595);
#24819=VERTEX_POINT('',#77606);
#24820=VERTEX_POINT('',#77610);
#24821=VERTEX_POINT('',#77621);
#24822=VERTEX_POINT('',#77625);
#24823=VERTEX_POINT('',#77636);
#24824=VERTEX_POINT('',#77640);
#24825=VERTEX_POINT('',#77651);
#24826=VERTEX_POINT('',#77655);
#24827=VERTEX_POINT('',#77666);
#24828=VERTEX_POINT('',#77670);
#24829=VERTEX_POINT('',#77697);
#24830=VERTEX_POINT('',#77698);
#24831=VERTEX_POINT('',#77702);
#24832=VERTEX_POINT('',#77704);
#24833=VERTEX_POINT('',#77715);
#24834=VERTEX_POINT('',#77719);
#24835=VERTEX_POINT('',#77730);
#24836=VERTEX_POINT('',#77734);
#24837=VERTEX_POINT('',#77745);
#24838=VERTEX_POINT('',#77749);
#24839=VERTEX_POINT('',#77760);
#24840=VERTEX_POINT('',#77764);
#24841=VERTEX_POINT('',#77775);
#24842=VERTEX_POINT('',#77779);
#24843=VERTEX_POINT('',#77790);
#24844=VERTEX_POINT('',#77794);
#24845=VERTEX_POINT('',#77817);
#24846=VERTEX_POINT('',#77818);
#24847=VERTEX_POINT('',#77822);
#24848=VERTEX_POINT('',#77824);
#24849=VERTEX_POINT('',#77835);
#24850=VERTEX_POINT('',#77839);
#24851=VERTEX_POINT('',#77850);
#24852=VERTEX_POINT('',#77854);
#24853=VERTEX_POINT('',#77865);
#24854=VERTEX_POINT('',#77869);
#24855=VERTEX_POINT('',#77880);
#24856=VERTEX_POINT('',#77884);
#24857=VERTEX_POINT('',#77895);
#24858=VERTEX_POINT('',#77899);
#24859=VERTEX_POINT('',#77910);
#24860=VERTEX_POINT('',#77914);
#24861=VERTEX_POINT('',#77925);
#24862=VERTEX_POINT('',#77929);
#24863=VERTEX_POINT('',#77940);
#24864=VERTEX_POINT('',#77944);
#24865=VERTEX_POINT('',#77955);
#24866=VERTEX_POINT('',#77959);
#24867=VERTEX_POINT('',#77970);
#24868=VERTEX_POINT('',#77974);
#24869=VERTEX_POINT('',#77998);
#24870=VERTEX_POINT('',#77999);
#24871=VERTEX_POINT('',#78003);
#24872=VERTEX_POINT('',#78005);
#24873=VERTEX_POINT('',#78016);
#24874=VERTEX_POINT('',#78020);
#24875=VERTEX_POINT('',#78031);
#24876=VERTEX_POINT('',#78035);
#24877=VERTEX_POINT('',#78041);
#24878=VERTEX_POINT('',#78043);
#24879=VERTEX_POINT('',#78052);
#24880=VERTEX_POINT('',#78056);
#24881=VERTEX_POINT('',#78067);
#24882=VERTEX_POINT('',#78071);
#24883=VERTEX_POINT('',#78082);
#24884=VERTEX_POINT('',#78086);
#24885=VERTEX_POINT('',#78092);
#24886=VERTEX_POINT('',#78094);
#24887=VERTEX_POINT('',#78098);
#24888=VERTEX_POINT('',#78100);
#24889=VERTEX_POINT('',#78104);
#24890=VERTEX_POINT('',#78106);
#24891=VERTEX_POINT('',#78120);
#24892=VERTEX_POINT('',#78121);
#24893=VERTEX_POINT('',#78125);
#24894=VERTEX_POINT('',#78127);
#24895=VERTEX_POINT('',#78138);
#24896=VERTEX_POINT('',#78142);
#24897=VERTEX_POINT('',#78153);
#24898=VERTEX_POINT('',#78157);
#24899=VERTEX_POINT('',#78168);
#24900=VERTEX_POINT('',#78172);
#24901=VERTEX_POINT('',#78183);
#24902=VERTEX_POINT('',#78187);
#24903=VERTEX_POINT('',#78198);
#24904=VERTEX_POINT('',#78202);
#24905=VERTEX_POINT('',#78213);
#24906=VERTEX_POINT('',#78217);
#24907=VERTEX_POINT('',#78240);
#24908=VERTEX_POINT('',#78241);
#24909=VERTEX_POINT('',#78245);
#24910=VERTEX_POINT('',#78247);
#24911=VERTEX_POINT('',#78258);
#24912=VERTEX_POINT('',#78262);
#24913=VERTEX_POINT('',#78273);
#24914=VERTEX_POINT('',#78277);
#24915=VERTEX_POINT('',#78288);
#24916=VERTEX_POINT('',#78292);
#24917=VERTEX_POINT('',#78303);
#24918=VERTEX_POINT('',#78307);
#24919=VERTEX_POINT('',#78318);
#24920=VERTEX_POINT('',#78322);
#24921=VERTEX_POINT('',#78333);
#24922=VERTEX_POINT('',#78337);
#24923=VERTEX_POINT('',#78348);
#24924=VERTEX_POINT('',#78352);
#24925=VERTEX_POINT('',#78363);
#24926=VERTEX_POINT('',#78367);
#24927=VERTEX_POINT('',#78378);
#24928=VERTEX_POINT('',#78382);
#24929=VERTEX_POINT('',#78393);
#24930=VERTEX_POINT('',#78397);
#24931=VERTEX_POINT('',#78421);
#24932=VERTEX_POINT('',#78422);
#24933=VERTEX_POINT('',#78426);
#24934=VERTEX_POINT('',#78428);
#24935=VERTEX_POINT('',#78439);
#24936=VERTEX_POINT('',#78443);
#24937=VERTEX_POINT('',#78454);
#24938=VERTEX_POINT('',#78458);
#24939=VERTEX_POINT('',#78469);
#24940=VERTEX_POINT('',#78473);
#24941=VERTEX_POINT('',#78484);
#24942=VERTEX_POINT('',#78488);
#24943=VERTEX_POINT('',#78499);
#24944=VERTEX_POINT('',#78503);
#24945=VERTEX_POINT('',#78514);
#24946=VERTEX_POINT('',#78518);
#24947=VERTEX_POINT('',#78529);
#24948=VERTEX_POINT('',#78533);
#24949=VERTEX_POINT('',#78556);
#24950=VERTEX_POINT('',#78557);
#24951=VERTEX_POINT('',#78561);
#24952=VERTEX_POINT('',#78563);
#24953=VERTEX_POINT('',#78574);
#24954=VERTEX_POINT('',#78578);
#24955=VERTEX_POINT('',#78589);
#24956=VERTEX_POINT('',#78593);
#24957=VERTEX_POINT('',#78604);
#24958=VERTEX_POINT('',#78608);
#24959=VERTEX_POINT('',#78619);
#24960=VERTEX_POINT('',#78623);
#24961=VERTEX_POINT('',#78634);
#24962=VERTEX_POINT('',#78638);
#24963=VERTEX_POINT('',#78649);
#24964=VERTEX_POINT('',#78653);
#24965=VERTEX_POINT('',#78664);
#24966=VERTEX_POINT('',#78668);
#24967=VERTEX_POINT('',#78679);
#24968=VERTEX_POINT('',#78683);
#24969=VERTEX_POINT('',#78694);
#24970=VERTEX_POINT('',#78698);
#24971=VERTEX_POINT('',#78709);
#24972=VERTEX_POINT('',#78713);
#24973=VERTEX_POINT('',#78724);
#24974=VERTEX_POINT('',#78728);
#24975=VERTEX_POINT('',#78739);
#24976=VERTEX_POINT('',#78743);
#24977=VERTEX_POINT('',#78754);
#24978=VERTEX_POINT('',#78758);
#24979=VERTEX_POINT('',#78769);
#24980=VERTEX_POINT('',#78773);
#24981=VERTEX_POINT('',#78784);
#24982=VERTEX_POINT('',#78788);
#24983=VERTEX_POINT('',#78799);
#24984=VERTEX_POINT('',#78803);
#24985=VERTEX_POINT('',#78809);
#24986=VERTEX_POINT('',#78811);
#24987=VERTEX_POINT('',#78835);
#24988=VERTEX_POINT('',#78836);
#24989=VERTEX_POINT('',#78840);
#24990=VERTEX_POINT('',#78842);
#24991=VERTEX_POINT('',#78853);
#24992=VERTEX_POINT('',#78857);
#24993=VERTEX_POINT('',#78868);
#24994=VERTEX_POINT('',#78872);
#24995=VERTEX_POINT('',#78883);
#24996=VERTEX_POINT('',#78887);
#24997=VERTEX_POINT('',#78898);
#24998=VERTEX_POINT('',#78902);
#24999=VERTEX_POINT('',#78913);
#25000=VERTEX_POINT('',#78917);
#25001=VERTEX_POINT('',#78928);
#25002=VERTEX_POINT('',#78932);
#25003=VERTEX_POINT('',#78955);
#25004=VERTEX_POINT('',#78956);
#25005=VERTEX_POINT('',#78960);
#25006=VERTEX_POINT('',#78962);
#25007=VERTEX_POINT('',#78973);
#25008=VERTEX_POINT('',#78977);
#25009=VERTEX_POINT('',#78988);
#25010=VERTEX_POINT('',#78992);
#25011=VERTEX_POINT('',#79003);
#25012=VERTEX_POINT('',#79007);
#25013=VERTEX_POINT('',#79018);
#25014=VERTEX_POINT('',#79022);
#25015=VERTEX_POINT('',#79033);
#25016=VERTEX_POINT('',#79037);
#25017=VERTEX_POINT('',#79048);
#25018=VERTEX_POINT('',#79052);
#25019=VERTEX_POINT('',#79063);
#25020=VERTEX_POINT('',#79067);
#25021=VERTEX_POINT('',#79078);
#25022=VERTEX_POINT('',#79082);
#25023=VERTEX_POINT('',#79093);
#25024=VERTEX_POINT('',#79097);
#25025=VERTEX_POINT('',#79108);
#25026=VERTEX_POINT('',#79112);
#25027=VERTEX_POINT('',#79136);
#25028=VERTEX_POINT('',#79137);
#25029=VERTEX_POINT('',#79141);
#25030=VERTEX_POINT('',#79143);
#25031=VERTEX_POINT('',#79154);
#25032=VERTEX_POINT('',#79158);
#25033=VERTEX_POINT('',#79169);
#25034=VERTEX_POINT('',#79173);
#25035=VERTEX_POINT('',#79184);
#25036=VERTEX_POINT('',#79188);
#25037=VERTEX_POINT('',#79199);
#25038=VERTEX_POINT('',#79203);
#25039=VERTEX_POINT('',#79214);
#25040=VERTEX_POINT('',#79218);
#25041=VERTEX_POINT('',#79224);
#25042=VERTEX_POINT('',#79226);
#25043=VERTEX_POINT('',#79230);
#25044=VERTEX_POINT('',#79232);
#25045=VERTEX_POINT('',#79236);
#25046=VERTEX_POINT('',#79238);
#25047=VERTEX_POINT('',#79242);
#25048=VERTEX_POINT('',#79244);
#25049=VERTEX_POINT('',#79248);
#25050=VERTEX_POINT('',#79250);
#25051=VERTEX_POINT('',#79254);
#25052=VERTEX_POINT('',#79256);
#25053=VERTEX_POINT('',#79265);
#25054=VERTEX_POINT('',#79269);
#25055=VERTEX_POINT('',#79280);
#25056=VERTEX_POINT('',#79284);
#25057=VERTEX_POINT('',#79295);
#25058=VERTEX_POINT('',#79299);
#25059=VERTEX_POINT('',#79310);
#25060=VERTEX_POINT('',#79314);
#25061=VERTEX_POINT('',#79325);
#25062=VERTEX_POINT('',#79329);
#25063=VERTEX_POINT('',#79340);
#25064=VERTEX_POINT('',#79344);
#25065=VERTEX_POINT('',#79355);
#25066=VERTEX_POINT('',#79359);
#25067=VERTEX_POINT('',#79370);
#25068=VERTEX_POINT('',#79374);
#25069=VERTEX_POINT('',#79380);
#25070=VERTEX_POINT('',#79382);
#25071=VERTEX_POINT('',#79405);
#25072=VERTEX_POINT('',#79406);
#25073=VERTEX_POINT('',#79410);
#25074=VERTEX_POINT('',#79412);
#25075=VERTEX_POINT('',#79423);
#25076=VERTEX_POINT('',#79427);
#25077=VERTEX_POINT('',#79438);
#25078=VERTEX_POINT('',#79442);
#25079=VERTEX_POINT('',#79453);
#25080=VERTEX_POINT('',#79457);
#25081=VERTEX_POINT('',#79468);
#25082=VERTEX_POINT('',#79472);
#25083=VERTEX_POINT('',#79483);
#25084=VERTEX_POINT('',#79487);
#25085=VERTEX_POINT('',#79498);
#25086=VERTEX_POINT('',#79502);
#25087=VERTEX_POINT('',#79525);
#25088=VERTEX_POINT('',#79526);
#25089=VERTEX_POINT('',#79530);
#25090=VERTEX_POINT('',#79532);
#25091=VERTEX_POINT('',#79543);
#25092=VERTEX_POINT('',#79547);
#25093=VERTEX_POINT('',#79558);
#25094=VERTEX_POINT('',#79562);
#25095=VERTEX_POINT('',#79573);
#25096=VERTEX_POINT('',#79577);
#25097=VERTEX_POINT('',#79588);
#25098=VERTEX_POINT('',#79592);
#25099=VERTEX_POINT('',#79603);
#25100=VERTEX_POINT('',#79607);
#25101=VERTEX_POINT('',#79618);
#25102=VERTEX_POINT('',#79622);
#25103=VERTEX_POINT('',#79633);
#25104=VERTEX_POINT('',#79637);
#25105=VERTEX_POINT('',#79648);
#25106=VERTEX_POINT('',#79652);
#25107=VERTEX_POINT('',#79663);
#25108=VERTEX_POINT('',#79667);
#25109=VERTEX_POINT('',#79678);
#25110=VERTEX_POINT('',#79682);
#25111=VERTEX_POINT('',#79701);
#25112=VERTEX_POINT('',#79702);
#25113=VERTEX_POINT('',#79704);
#25114=VERTEX_POINT('',#79706);
#25115=VERTEX_POINT('',#79710);
#25116=VERTEX_POINT('',#79712);
#25117=VERTEX_POINT('',#79719);
#25118=VERTEX_POINT('',#79720);
#25119=VERTEX_POINT('',#79722);
#25120=VERTEX_POINT('',#79724);
#25121=VERTEX_POINT('',#79728);
#25122=VERTEX_POINT('',#79730);
#25123=VERTEX_POINT('',#79734);
#25124=VERTEX_POINT('',#79736);
#25125=VERTEX_POINT('',#79740);
#25126=VERTEX_POINT('',#79742);
#25127=VERTEX_POINT('',#79746);
#25128=VERTEX_POINT('',#79748);
#25129=VERTEX_POINT('',#79752);
#25130=VERTEX_POINT('',#79754);
#25131=VERTEX_POINT('',#79758);
#25132=VERTEX_POINT('',#79760);
#25133=VERTEX_POINT('',#79764);
#25134=VERTEX_POINT('',#79766);
#25135=VERTEX_POINT('',#79770);
#25136=VERTEX_POINT('',#79772);
#25137=VERTEX_POINT('',#79776);
#25138=VERTEX_POINT('',#79778);
#25139=VERTEX_POINT('',#79793);
#25140=VERTEX_POINT('',#79794);
#25141=VERTEX_POINT('',#79798);
#25142=VERTEX_POINT('',#79800);
#25143=VERTEX_POINT('',#79811);
#25144=VERTEX_POINT('',#79815);
#25145=VERTEX_POINT('',#79826);
#25146=VERTEX_POINT('',#79830);
#25147=VERTEX_POINT('',#79841);
#25148=VERTEX_POINT('',#79845);
#25149=VERTEX_POINT('',#79856);
#25150=VERTEX_POINT('',#79860);
#25151=VERTEX_POINT('',#79871);
#25152=VERTEX_POINT('',#79875);
#25153=VERTEX_POINT('',#79886);
#25154=VERTEX_POINT('',#79890);
#25155=VERTEX_POINT('',#79913);
#25156=VERTEX_POINT('',#79914);
#25157=VERTEX_POINT('',#79918);
#25158=VERTEX_POINT('',#79920);
#25159=VERTEX_POINT('',#79931);
#25160=VERTEX_POINT('',#79935);
#25161=VERTEX_POINT('',#79946);
#25162=VERTEX_POINT('',#79950);
#25163=VERTEX_POINT('',#79961);
#25164=VERTEX_POINT('',#79965);
#25165=VERTEX_POINT('',#79976);
#25166=VERTEX_POINT('',#79980);
#25167=VERTEX_POINT('',#79991);
#25168=VERTEX_POINT('',#79995);
#25169=VERTEX_POINT('',#80006);
#25170=VERTEX_POINT('',#80010);
#25171=VERTEX_POINT('',#80021);
#25172=VERTEX_POINT('',#80025);
#25173=VERTEX_POINT('',#80036);
#25174=VERTEX_POINT('',#80040);
#25175=VERTEX_POINT('',#80051);
#25176=VERTEX_POINT('',#80055);
#25177=VERTEX_POINT('',#80066);
#25178=VERTEX_POINT('',#80070);
#25179=VERTEX_POINT('',#80094);
#25180=VERTEX_POINT('',#80095);
#25181=VERTEX_POINT('',#80099);
#25182=VERTEX_POINT('',#80101);
#25183=VERTEX_POINT('',#80112);
#25184=VERTEX_POINT('',#80116);
#25185=VERTEX_POINT('',#80127);
#25186=VERTEX_POINT('',#80131);
#25187=VERTEX_POINT('',#80142);
#25188=VERTEX_POINT('',#80146);
#25189=VERTEX_POINT('',#80157);
#25190=VERTEX_POINT('',#80161);
#25191=VERTEX_POINT('',#80172);
#25192=VERTEX_POINT('',#80176);
#25193=VERTEX_POINT('',#80187);
#25194=VERTEX_POINT('',#80191);
#25195=VERTEX_POINT('',#80202);
#25196=VERTEX_POINT('',#80206);
#25197=VERTEX_POINT('',#80217);
#25198=VERTEX_POINT('',#80221);
#25199=VERTEX_POINT('',#80232);
#25200=VERTEX_POINT('',#80236);
#25201=VERTEX_POINT('',#80247);
#25202=VERTEX_POINT('',#80251);
#25203=VERTEX_POINT('',#80262);
#25204=VERTEX_POINT('',#80266);
#25205=VERTEX_POINT('',#80272);
#25206=VERTEX_POINT('',#80274);
#25207=VERTEX_POINT('',#80283);
#25208=VERTEX_POINT('',#80287);
#25209=VERTEX_POINT('',#80298);
#25210=VERTEX_POINT('',#80302);
#25211=VERTEX_POINT('',#80313);
#25212=VERTEX_POINT('',#80317);
#25213=VERTEX_POINT('',#80328);
#25214=VERTEX_POINT('',#80332);
#25215=VERTEX_POINT('',#80343);
#25216=VERTEX_POINT('',#80347);
#25217=VERTEX_POINT('',#80358);
#25218=VERTEX_POINT('',#80362);
#25219=VERTEX_POINT('',#80373);
#25220=VERTEX_POINT('',#80377);
#25221=VERTEX_POINT('',#80383);
#25222=VERTEX_POINT('',#80385);
#25223=VERTEX_POINT('',#80394);
#25224=VERTEX_POINT('',#80398);
#25225=VERTEX_POINT('',#80409);
#25226=VERTEX_POINT('',#80413);
#25227=VERTEX_POINT('',#80424);
#25228=VERTEX_POINT('',#80428);
#25229=VERTEX_POINT('',#80439);
#25230=VERTEX_POINT('',#80443);
#25231=VERTEX_POINT('',#80454);
#25232=VERTEX_POINT('',#80458);
#25233=VERTEX_POINT('',#80469);
#25234=VERTEX_POINT('',#80473);
#25235=VERTEX_POINT('',#80484);
#25236=VERTEX_POINT('',#80488);
#25237=VERTEX_POINT('',#80494);
#25238=VERTEX_POINT('',#80496);
#25239=VERTEX_POINT('',#80519);
#25240=VERTEX_POINT('',#80520);
#25241=VERTEX_POINT('',#80524);
#25242=VERTEX_POINT('',#80526);
#25243=VERTEX_POINT('',#80537);
#25244=VERTEX_POINT('',#80541);
#25245=VERTEX_POINT('',#80552);
#25246=VERTEX_POINT('',#80556);
#25247=VERTEX_POINT('',#80567);
#25248=VERTEX_POINT('',#80571);
#25249=VERTEX_POINT('',#80582);
#25250=VERTEX_POINT('',#80586);
#25251=VERTEX_POINT('',#80597);
#25252=VERTEX_POINT('',#80601);
#25253=VERTEX_POINT('',#80612);
#25254=VERTEX_POINT('',#80616);
#25255=VERTEX_POINT('',#80639);
#25256=VERTEX_POINT('',#80640);
#25257=VERTEX_POINT('',#80644);
#25258=VERTEX_POINT('',#80646);
#25259=VERTEX_POINT('',#80657);
#25260=VERTEX_POINT('',#80661);
#25261=VERTEX_POINT('',#80672);
#25262=VERTEX_POINT('',#80676);
#25263=VERTEX_POINT('',#80687);
#25264=VERTEX_POINT('',#80691);
#25265=VERTEX_POINT('',#80702);
#25266=VERTEX_POINT('',#80706);
#25267=VERTEX_POINT('',#80717);
#25268=VERTEX_POINT('',#80721);
#25269=VERTEX_POINT('',#80732);
#25270=VERTEX_POINT('',#80736);
#25271=VERTEX_POINT('',#80747);
#25272=VERTEX_POINT('',#80751);
#25273=VERTEX_POINT('',#80762);
#25274=VERTEX_POINT('',#80766);
#25275=VERTEX_POINT('',#80777);
#25276=VERTEX_POINT('',#80781);
#25277=VERTEX_POINT('',#80792);
#25278=VERTEX_POINT('',#80796);
#25279=VERTEX_POINT('',#80820);
#25280=VERTEX_POINT('',#80821);
#25281=VERTEX_POINT('',#80825);
#25282=VERTEX_POINT('',#80827);
#25283=VERTEX_POINT('',#80838);
#25284=VERTEX_POINT('',#80842);
#25285=VERTEX_POINT('',#80853);
#25286=VERTEX_POINT('',#80857);
#25287=VERTEX_POINT('',#80868);
#25288=VERTEX_POINT('',#80872);
#25289=VERTEX_POINT('',#80883);
#25290=VERTEX_POINT('',#80887);
#25291=VERTEX_POINT('',#80898);
#25292=VERTEX_POINT('',#80902);
#25293=VERTEX_POINT('',#80913);
#25294=VERTEX_POINT('',#80917);
#25295=VERTEX_POINT('',#80928);
#25296=VERTEX_POINT('',#80932);
#25297=VERTEX_POINT('',#80943);
#25298=VERTEX_POINT('',#80947);
#25299=VERTEX_POINT('',#80953);
#25300=VERTEX_POINT('',#80955);
#25301=VERTEX_POINT('',#80964);
#25302=VERTEX_POINT('',#80968);
#25303=VERTEX_POINT('',#80979);
#25304=VERTEX_POINT('',#80983);
#25305=VERTEX_POINT('',#80994);
#25306=VERTEX_POINT('',#80998);
#25307=VERTEX_POINT('',#81009);
#25308=VERTEX_POINT('',#81013);
#25309=VERTEX_POINT('',#81024);
#25310=VERTEX_POINT('',#81028);
#25311=VERTEX_POINT('',#81039);
#25312=VERTEX_POINT('',#81043);
#25313=VERTEX_POINT('',#81054);
#25314=VERTEX_POINT('',#81058);
#25315=VERTEX_POINT('',#81069);
#25316=VERTEX_POINT('',#81073);
#25317=VERTEX_POINT('',#81084);
#25318=VERTEX_POINT('',#81088);
#25319=VERTEX_POINT('',#81094);
#25320=VERTEX_POINT('',#81096);
#25321=VERTEX_POINT('',#81100);
#25322=VERTEX_POINT('',#81102);
#25323=VERTEX_POINT('',#81116);
#25324=VERTEX_POINT('',#81117);
#25325=VERTEX_POINT('',#81121);
#25326=VERTEX_POINT('',#81123);
#25327=VERTEX_POINT('',#81134);
#25328=VERTEX_POINT('',#81138);
#25329=VERTEX_POINT('',#81149);
#25330=VERTEX_POINT('',#81153);
#25331=VERTEX_POINT('',#81164);
#25332=VERTEX_POINT('',#81168);
#25333=VERTEX_POINT('',#81179);
#25334=VERTEX_POINT('',#81183);
#25335=VERTEX_POINT('',#81194);
#25336=VERTEX_POINT('',#81198);
#25337=VERTEX_POINT('',#81209);
#25338=VERTEX_POINT('',#81213);
#25339=VERTEX_POINT('',#81236);
#25340=VERTEX_POINT('',#81237);
#25341=VERTEX_POINT('',#81241);
#25342=VERTEX_POINT('',#81243);
#25343=VERTEX_POINT('',#81254);
#25344=VERTEX_POINT('',#81258);
#25345=VERTEX_POINT('',#81269);
#25346=VERTEX_POINT('',#81273);
#25347=VERTEX_POINT('',#81284);
#25348=VERTEX_POINT('',#81288);
#25349=VERTEX_POINT('',#81299);
#25350=VERTEX_POINT('',#81303);
#25351=VERTEX_POINT('',#81314);
#25352=VERTEX_POINT('',#81318);
#25353=VERTEX_POINT('',#81329);
#25354=VERTEX_POINT('',#81333);
#25355=VERTEX_POINT('',#81344);
#25356=VERTEX_POINT('',#81348);
#25357=VERTEX_POINT('',#81359);
#25358=VERTEX_POINT('',#81363);
#25359=VERTEX_POINT('',#81374);
#25360=VERTEX_POINT('',#81378);
#25361=VERTEX_POINT('',#81389);
#25362=VERTEX_POINT('',#81393);
#25363=VERTEX_POINT('',#81412);
#25364=VERTEX_POINT('',#81413);
#25365=VERTEX_POINT('',#81415);
#25366=VERTEX_POINT('',#81417);
#25367=VERTEX_POINT('',#81426);
#25368=VERTEX_POINT('',#81430);
#25369=VERTEX_POINT('',#81441);
#25370=VERTEX_POINT('',#81445);
#25371=VERTEX_POINT('',#81451);
#25372=VERTEX_POINT('',#81453);
#25373=VERTEX_POINT('',#81462);
#25374=VERTEX_POINT('',#81466);
#25375=VERTEX_POINT('',#81477);
#25376=VERTEX_POINT('',#81481);
#25377=VERTEX_POINT('',#81487);
#25378=VERTEX_POINT('',#81489);
#25379=VERTEX_POINT('',#81493);
#25380=VERTEX_POINT('',#81495);
#25381=VERTEX_POINT('',#81509);
#25382=VERTEX_POINT('',#81510);
#25383=VERTEX_POINT('',#81514);
#25384=VERTEX_POINT('',#81516);
#25385=VERTEX_POINT('',#81527);
#25386=VERTEX_POINT('',#81531);
#25387=VERTEX_POINT('',#81542);
#25388=VERTEX_POINT('',#81546);
#25389=VERTEX_POINT('',#81557);
#25390=VERTEX_POINT('',#81561);
#25391=VERTEX_POINT('',#81572);
#25392=VERTEX_POINT('',#81576);
#25393=VERTEX_POINT('',#81587);
#25394=VERTEX_POINT('',#81591);
#25395=VERTEX_POINT('',#81602);
#25396=VERTEX_POINT('',#81606);
#25397=VERTEX_POINT('',#81629);
#25398=VERTEX_POINT('',#81630);
#25399=VERTEX_POINT('',#81634);
#25400=VERTEX_POINT('',#81636);
#25401=VERTEX_POINT('',#81647);
#25402=VERTEX_POINT('',#81651);
#25403=VERTEX_POINT('',#81662);
#25404=VERTEX_POINT('',#81666);
#25405=VERTEX_POINT('',#81677);
#25406=VERTEX_POINT('',#81681);
#25407=VERTEX_POINT('',#81692);
#25408=VERTEX_POINT('',#81696);
#25409=VERTEX_POINT('',#81707);
#25410=VERTEX_POINT('',#81711);
#25411=VERTEX_POINT('',#81722);
#25412=VERTEX_POINT('',#81726);
#25413=VERTEX_POINT('',#81737);
#25414=VERTEX_POINT('',#81741);
#25415=VERTEX_POINT('',#81752);
#25416=VERTEX_POINT('',#81756);
#25417=VERTEX_POINT('',#81767);
#25418=VERTEX_POINT('',#81771);
#25419=VERTEX_POINT('',#81782);
#25420=VERTEX_POINT('',#81786);
#25421=VERTEX_POINT('',#81811);
#25422=VERTEX_POINT('',#81812);
#25423=VERTEX_POINT('',#81816);
#25424=VERTEX_POINT('',#81818);
#25425=VERTEX_POINT('',#81829);
#25426=VERTEX_POINT('',#81833);
#25427=VERTEX_POINT('',#81844);
#25428=VERTEX_POINT('',#81848);
#25429=VERTEX_POINT('',#81859);
#25430=VERTEX_POINT('',#81863);
#25431=VERTEX_POINT('',#81874);
#25432=VERTEX_POINT('',#81878);
#25433=VERTEX_POINT('',#81889);
#25434=VERTEX_POINT('',#81893);
#25435=VERTEX_POINT('',#81904);
#25436=VERTEX_POINT('',#81908);
#25437=VERTEX_POINT('',#81931);
#25438=VERTEX_POINT('',#81932);
#25439=VERTEX_POINT('',#81936);
#25440=VERTEX_POINT('',#81938);
#25441=VERTEX_POINT('',#81949);
#25442=VERTEX_POINT('',#81953);
#25443=VERTEX_POINT('',#81964);
#25444=VERTEX_POINT('',#81968);
#25445=VERTEX_POINT('',#81979);
#25446=VERTEX_POINT('',#81983);
#25447=VERTEX_POINT('',#81994);
#25448=VERTEX_POINT('',#81998);
#25449=VERTEX_POINT('',#82009);
#25450=VERTEX_POINT('',#82013);
#25451=VERTEX_POINT('',#82024);
#25452=VERTEX_POINT('',#82028);
#25453=VERTEX_POINT('',#82039);
#25454=VERTEX_POINT('',#82043);
#25455=VERTEX_POINT('',#82054);
#25456=VERTEX_POINT('',#82058);
#25457=VERTEX_POINT('',#82069);
#25458=VERTEX_POINT('',#82073);
#25459=VERTEX_POINT('',#82084);
#25460=VERTEX_POINT('',#82088);
#25461=VERTEX_POINT('',#82107);
#25462=VERTEX_POINT('',#82108);
#25463=VERTEX_POINT('',#82110);
#25464=VERTEX_POINT('',#82112);
#25465=VERTEX_POINT('',#82121);
#25466=VERTEX_POINT('',#82125);
#25467=VERTEX_POINT('',#82136);
#25468=VERTEX_POINT('',#82140);
#25469=VERTEX_POINT('',#82146);
#25470=VERTEX_POINT('',#82148);
#25471=VERTEX_POINT('',#82157);
#25472=VERTEX_POINT('',#82161);
#25473=VERTEX_POINT('',#82172);
#25474=VERTEX_POINT('',#82176);
#25475=VERTEX_POINT('',#82182);
#25476=VERTEX_POINT('',#82184);
#25477=VERTEX_POINT('',#82188);
#25478=VERTEX_POINT('',#82190);
#25479=VERTEX_POINT('',#82204);
#25480=VERTEX_POINT('',#82205);
#25481=VERTEX_POINT('',#82209);
#25482=VERTEX_POINT('',#82211);
#25483=VERTEX_POINT('',#82222);
#25484=VERTEX_POINT('',#82226);
#25485=VERTEX_POINT('',#82237);
#25486=VERTEX_POINT('',#82241);
#25487=VERTEX_POINT('',#82252);
#25488=VERTEX_POINT('',#82256);
#25489=VERTEX_POINT('',#82267);
#25490=VERTEX_POINT('',#82271);
#25491=VERTEX_POINT('',#82282);
#25492=VERTEX_POINT('',#82286);
#25493=VERTEX_POINT('',#82297);
#25494=VERTEX_POINT('',#82301);
#25495=VERTEX_POINT('',#82324);
#25496=VERTEX_POINT('',#82325);
#25497=VERTEX_POINT('',#82329);
#25498=VERTEX_POINT('',#82331);
#25499=VERTEX_POINT('',#82342);
#25500=VERTEX_POINT('',#82346);
#25501=VERTEX_POINT('',#82357);
#25502=VERTEX_POINT('',#82361);
#25503=VERTEX_POINT('',#82372);
#25504=VERTEX_POINT('',#82376);
#25505=VERTEX_POINT('',#82387);
#25506=VERTEX_POINT('',#82391);
#25507=VERTEX_POINT('',#82402);
#25508=VERTEX_POINT('',#82406);
#25509=VERTEX_POINT('',#82417);
#25510=VERTEX_POINT('',#82421);
#25511=VERTEX_POINT('',#82432);
#25512=VERTEX_POINT('',#82436);
#25513=VERTEX_POINT('',#82447);
#25514=VERTEX_POINT('',#82451);
#25515=VERTEX_POINT('',#82462);
#25516=VERTEX_POINT('',#82466);
#25517=VERTEX_POINT('',#82477);
#25518=VERTEX_POINT('',#82481);
#25519=VERTEX_POINT('',#82505);
#25520=VERTEX_POINT('',#82506);
#25521=VERTEX_POINT('',#82510);
#25522=VERTEX_POINT('',#82512);
#25523=VERTEX_POINT('',#82523);
#25524=VERTEX_POINT('',#82527);
#25525=VERTEX_POINT('',#82538);
#25526=VERTEX_POINT('',#82542);
#25527=VERTEX_POINT('',#82553);
#25528=VERTEX_POINT('',#82557);
#25529=VERTEX_POINT('',#82568);
#25530=VERTEX_POINT('',#82572);
#25531=VERTEX_POINT('',#82583);
#25532=VERTEX_POINT('',#82587);
#25533=VERTEX_POINT('',#82598);
#25534=VERTEX_POINT('',#82602);
#25535=VERTEX_POINT('',#82613);
#25536=VERTEX_POINT('',#82617);
#25537=VERTEX_POINT('',#82628);
#25538=VERTEX_POINT('',#82632);
#25539=VERTEX_POINT('',#82638);
#25540=VERTEX_POINT('',#82640);
#25541=VERTEX_POINT('',#82649);
#25542=VERTEX_POINT('',#82653);
#25543=VERTEX_POINT('',#82664);
#25544=VERTEX_POINT('',#82668);
#25545=VERTEX_POINT('',#82679);
#25546=VERTEX_POINT('',#82683);
#25547=VERTEX_POINT('',#82694);
#25548=VERTEX_POINT('',#82698);
#25549=VERTEX_POINT('',#82709);
#25550=VERTEX_POINT('',#82713);
#25551=VERTEX_POINT('',#82724);
#25552=VERTEX_POINT('',#82728);
#25553=VERTEX_POINT('',#82739);
#25554=VERTEX_POINT('',#82743);
#25555=VERTEX_POINT('',#82754);
#25556=VERTEX_POINT('',#82758);
#25557=VERTEX_POINT('',#82769);
#25558=VERTEX_POINT('',#82773);
#25559=VERTEX_POINT('',#82779);
#25560=VERTEX_POINT('',#82781);
#25561=VERTEX_POINT('',#82785);
#25562=VERTEX_POINT('',#82787);
#25563=VERTEX_POINT('',#82801);
#25564=VERTEX_POINT('',#82802);
#25565=VERTEX_POINT('',#82806);
#25566=VERTEX_POINT('',#82808);
#25567=VERTEX_POINT('',#82819);
#25568=VERTEX_POINT('',#82823);
#25569=VERTEX_POINT('',#82834);
#25570=VERTEX_POINT('',#82838);
#25571=VERTEX_POINT('',#82849);
#25572=VERTEX_POINT('',#82853);
#25573=VERTEX_POINT('',#82864);
#25574=VERTEX_POINT('',#82868);
#25575=VERTEX_POINT('',#82879);
#25576=VERTEX_POINT('',#82883);
#25577=VERTEX_POINT('',#82894);
#25578=VERTEX_POINT('',#82898);
#25579=VERTEX_POINT('',#82921);
#25580=VERTEX_POINT('',#82922);
#25581=VERTEX_POINT('',#82926);
#25582=VERTEX_POINT('',#82928);
#25583=VERTEX_POINT('',#82939);
#25584=VERTEX_POINT('',#82943);
#25585=VERTEX_POINT('',#82954);
#25586=VERTEX_POINT('',#82958);
#25587=VERTEX_POINT('',#82969);
#25588=VERTEX_POINT('',#82973);
#25589=VERTEX_POINT('',#82984);
#25590=VERTEX_POINT('',#82988);
#25591=VERTEX_POINT('',#82999);
#25592=VERTEX_POINT('',#83003);
#25593=VERTEX_POINT('',#83014);
#25594=VERTEX_POINT('',#83018);
#25595=VERTEX_POINT('',#83029);
#25596=VERTEX_POINT('',#83033);
#25597=VERTEX_POINT('',#83044);
#25598=VERTEX_POINT('',#83048);
#25599=VERTEX_POINT('',#83059);
#25600=VERTEX_POINT('',#83063);
#25601=VERTEX_POINT('',#83074);
#25602=VERTEX_POINT('',#83078);
#25603=VERTEX_POINT('',#83102);
#25604=VERTEX_POINT('',#83103);
#25605=VERTEX_POINT('',#83107);
#25606=VERTEX_POINT('',#83109);
#25607=VERTEX_POINT('',#83120);
#25608=VERTEX_POINT('',#83124);
#25609=VERTEX_POINT('',#83135);
#25610=VERTEX_POINT('',#83139);
#25611=VERTEX_POINT('',#83150);
#25612=VERTEX_POINT('',#83154);
#25613=VERTEX_POINT('',#83165);
#25614=VERTEX_POINT('',#83169);
#25615=VERTEX_POINT('',#83180);
#25616=VERTEX_POINT('',#83184);
#25617=VERTEX_POINT('',#83195);
#25618=VERTEX_POINT('',#83199);
#25619=VERTEX_POINT('',#83210);
#25620=VERTEX_POINT('',#83214);
#25621=VERTEX_POINT('',#83225);
#25622=VERTEX_POINT('',#83229);
#25623=VERTEX_POINT('',#83240);
#25624=VERTEX_POINT('',#83244);
#25625=VERTEX_POINT('',#83255);
#25626=VERTEX_POINT('',#83259);
#25627=VERTEX_POINT('',#83270);
#25628=VERTEX_POINT('',#83274);
#25629=VERTEX_POINT('',#83280);
#25630=VERTEX_POINT('',#83282);
#25631=VERTEX_POINT('',#83291);
#25632=VERTEX_POINT('',#83295);
#25633=VERTEX_POINT('',#83306);
#25634=VERTEX_POINT('',#83310);
#25635=VERTEX_POINT('',#83321);
#25636=VERTEX_POINT('',#83325);
#25637=VERTEX_POINT('',#83336);
#25638=VERTEX_POINT('',#83340);
#25639=VERTEX_POINT('',#83351);
#25640=VERTEX_POINT('',#83355);
#25641=VERTEX_POINT('',#83366);
#25642=VERTEX_POINT('',#83370);
#25643=VERTEX_POINT('',#83381);
#25644=VERTEX_POINT('',#83385);
#25645=VERTEX_POINT('',#83391);
#25646=VERTEX_POINT('',#83393);
#25647=VERTEX_POINT('',#83402);
#25648=VERTEX_POINT('',#83406);
#25649=VERTEX_POINT('',#83417);
#25650=VERTEX_POINT('',#83421);
#25651=VERTEX_POINT('',#83432);
#25652=VERTEX_POINT('',#83436);
#25653=VERTEX_POINT('',#83447);
#25654=VERTEX_POINT('',#83451);
#25655=VERTEX_POINT('',#83462);
#25656=VERTEX_POINT('',#83466);
#25657=VERTEX_POINT('',#83477);
#25658=VERTEX_POINT('',#83481);
#25659=VERTEX_POINT('',#83492);
#25660=VERTEX_POINT('',#83496);
#25661=VERTEX_POINT('',#83502);
#25662=VERTEX_POINT('',#83504);
#25663=VERTEX_POINT('',#83527);
#25664=VERTEX_POINT('',#83528);
#25665=VERTEX_POINT('',#83532);
#25666=VERTEX_POINT('',#83534);
#25667=VERTEX_POINT('',#83545);
#25668=VERTEX_POINT('',#83549);
#25669=VERTEX_POINT('',#83560);
#25670=VERTEX_POINT('',#83564);
#25671=VERTEX_POINT('',#83575);
#25672=VERTEX_POINT('',#83579);
#25673=VERTEX_POINT('',#83590);
#25674=VERTEX_POINT('',#83594);
#25675=VERTEX_POINT('',#83605);
#25676=VERTEX_POINT('',#83609);
#25677=VERTEX_POINT('',#83620);
#25678=VERTEX_POINT('',#83624);
#25679=VERTEX_POINT('',#83647);
#25680=VERTEX_POINT('',#83648);
#25681=VERTEX_POINT('',#83652);
#25682=VERTEX_POINT('',#83654);
#25683=VERTEX_POINT('',#83665);
#25684=VERTEX_POINT('',#83669);
#25685=VERTEX_POINT('',#83680);
#25686=VERTEX_POINT('',#83684);
#25687=VERTEX_POINT('',#83695);
#25688=VERTEX_POINT('',#83699);
#25689=VERTEX_POINT('',#83710);
#25690=VERTEX_POINT('',#83714);
#25691=VERTEX_POINT('',#83725);
#25692=VERTEX_POINT('',#83729);
#25693=VERTEX_POINT('',#83740);
#25694=VERTEX_POINT('',#83744);
#25695=VERTEX_POINT('',#83755);
#25696=VERTEX_POINT('',#83759);
#25697=VERTEX_POINT('',#83770);
#25698=VERTEX_POINT('',#83774);
#25699=VERTEX_POINT('',#83785);
#25700=VERTEX_POINT('',#83789);
#25701=VERTEX_POINT('',#83800);
#25702=VERTEX_POINT('',#83804);
#25703=VERTEX_POINT('',#83823);
#25704=VERTEX_POINT('',#83824);
#25705=VERTEX_POINT('',#83826);
#25706=VERTEX_POINT('',#83828);
#25707=VERTEX_POINT('',#83832);
#25708=VERTEX_POINT('',#83834);
#25709=VERTEX_POINT('',#83841);
#25710=VERTEX_POINT('',#83842);
#25711=VERTEX_POINT('',#83844);
#25712=VERTEX_POINT('',#83846);
#25713=VERTEX_POINT('',#83850);
#25714=VERTEX_POINT('',#83852);
#25715=VERTEX_POINT('',#83856);
#25716=VERTEX_POINT('',#83858);
#25717=VERTEX_POINT('',#83862);
#25718=VERTEX_POINT('',#83864);
#25719=VERTEX_POINT('',#83868);
#25720=VERTEX_POINT('',#83870);
#25721=VERTEX_POINT('',#83874);
#25722=VERTEX_POINT('',#83876);
#25723=VERTEX_POINT('',#83880);
#25724=VERTEX_POINT('',#83882);
#25725=VERTEX_POINT('',#83886);
#25726=VERTEX_POINT('',#83888);
#25727=VERTEX_POINT('',#83892);
#25728=VERTEX_POINT('',#83894);
#25729=VERTEX_POINT('',#83898);
#25730=VERTEX_POINT('',#83900);
#25731=VERTEX_POINT('',#83915);
#25732=VERTEX_POINT('',#83916);
#25733=VERTEX_POINT('',#83920);
#25734=VERTEX_POINT('',#83922);
#25735=VERTEX_POINT('',#83933);
#25736=VERTEX_POINT('',#83937);
#25737=VERTEX_POINT('',#83948);
#25738=VERTEX_POINT('',#83952);
#25739=VERTEX_POINT('',#83963);
#25740=VERTEX_POINT('',#83967);
#25741=VERTEX_POINT('',#83978);
#25742=VERTEX_POINT('',#83982);
#25743=VERTEX_POINT('',#83993);
#25744=VERTEX_POINT('',#83997);
#25745=VERTEX_POINT('',#84008);
#25746=VERTEX_POINT('',#84012);
#25747=VERTEX_POINT('',#84035);
#25748=VERTEX_POINT('',#84036);
#25749=VERTEX_POINT('',#84040);
#25750=VERTEX_POINT('',#84042);
#25751=VERTEX_POINT('',#84053);
#25752=VERTEX_POINT('',#84057);
#25753=VERTEX_POINT('',#84068);
#25754=VERTEX_POINT('',#84072);
#25755=VERTEX_POINT('',#84083);
#25756=VERTEX_POINT('',#84087);
#25757=VERTEX_POINT('',#84098);
#25758=VERTEX_POINT('',#84102);
#25759=VERTEX_POINT('',#84113);
#25760=VERTEX_POINT('',#84117);
#25761=VERTEX_POINT('',#84128);
#25762=VERTEX_POINT('',#84132);
#25763=VERTEX_POINT('',#84143);
#25764=VERTEX_POINT('',#84147);
#25765=VERTEX_POINT('',#84158);
#25766=VERTEX_POINT('',#84162);
#25767=VERTEX_POINT('',#84173);
#25768=VERTEX_POINT('',#84177);
#25769=VERTEX_POINT('',#84188);
#25770=VERTEX_POINT('',#84192);
#25771=VERTEX_POINT('',#84216);
#25772=VERTEX_POINT('',#84217);
#25773=VERTEX_POINT('',#84221);
#25774=VERTEX_POINT('',#84223);
#25775=VERTEX_POINT('',#84234);
#25776=VERTEX_POINT('',#84238);
#25777=VERTEX_POINT('',#84249);
#25778=VERTEX_POINT('',#84253);
#25779=VERTEX_POINT('',#84264);
#25780=VERTEX_POINT('',#84268);
#25781=VERTEX_POINT('',#84279);
#25782=VERTEX_POINT('',#84283);
#25783=VERTEX_POINT('',#84294);
#25784=VERTEX_POINT('',#84298);
#25785=VERTEX_POINT('',#84304);
#25786=VERTEX_POINT('',#84306);
#25787=VERTEX_POINT('',#84310);
#25788=VERTEX_POINT('',#84312);
#25789=VERTEX_POINT('',#84316);
#25790=VERTEX_POINT('',#84318);
#25791=VERTEX_POINT('',#84322);
#25792=VERTEX_POINT('',#84324);
#25793=VERTEX_POINT('',#84328);
#25794=VERTEX_POINT('',#84330);
#25795=VERTEX_POINT('',#84334);
#25796=VERTEX_POINT('',#84336);
#25797=VERTEX_POINT('',#84345);
#25798=VERTEX_POINT('',#84349);
#25799=VERTEX_POINT('',#84360);
#25800=VERTEX_POINT('',#84364);
#25801=VERTEX_POINT('',#84375);
#25802=VERTEX_POINT('',#84379);
#25803=VERTEX_POINT('',#84390);
#25804=VERTEX_POINT('',#84394);
#25805=VERTEX_POINT('',#84405);
#25806=VERTEX_POINT('',#84409);
#25807=VERTEX_POINT('',#84420);
#25808=VERTEX_POINT('',#84424);
#25809=VERTEX_POINT('',#84435);
#25810=VERTEX_POINT('',#84439);
#25811=VERTEX_POINT('',#84450);
#25812=VERTEX_POINT('',#84454);
#25813=VERTEX_POINT('',#84460);
#25814=VERTEX_POINT('',#84462);
#25815=VERTEX_POINT('',#84485);
#25816=VERTEX_POINT('',#84486);
#25817=VERTEX_POINT('',#84490);
#25818=VERTEX_POINT('',#84492);
#25819=VERTEX_POINT('',#84503);
#25820=VERTEX_POINT('',#84507);
#25821=VERTEX_POINT('',#84518);
#25822=VERTEX_POINT('',#84522);
#25823=VERTEX_POINT('',#84533);
#25824=VERTEX_POINT('',#84537);
#25825=VERTEX_POINT('',#84548);
#25826=VERTEX_POINT('',#84552);
#25827=VERTEX_POINT('',#84563);
#25828=VERTEX_POINT('',#84567);
#25829=VERTEX_POINT('',#84578);
#25830=VERTEX_POINT('',#84582);
#25831=VERTEX_POINT('',#84605);
#25832=VERTEX_POINT('',#84606);
#25833=VERTEX_POINT('',#84610);
#25834=VERTEX_POINT('',#84612);
#25835=VERTEX_POINT('',#84623);
#25836=VERTEX_POINT('',#84627);
#25837=VERTEX_POINT('',#84638);
#25838=VERTEX_POINT('',#84642);
#25839=VERTEX_POINT('',#84653);
#25840=VERTEX_POINT('',#84657);
#25841=VERTEX_POINT('',#84668);
#25842=VERTEX_POINT('',#84672);
#25843=VERTEX_POINT('',#84683);
#25844=VERTEX_POINT('',#84687);
#25845=VERTEX_POINT('',#84698);
#25846=VERTEX_POINT('',#84702);
#25847=VERTEX_POINT('',#84713);
#25848=VERTEX_POINT('',#84717);
#25849=VERTEX_POINT('',#84728);
#25850=VERTEX_POINT('',#84732);
#25851=VERTEX_POINT('',#84743);
#25852=VERTEX_POINT('',#84747);
#25853=VERTEX_POINT('',#84758);
#25854=VERTEX_POINT('',#84762);
#25855=VERTEX_POINT('',#84786);
#25856=VERTEX_POINT('',#84787);
#25857=VERTEX_POINT('',#84791);
#25858=VERTEX_POINT('',#84793);
#25859=VERTEX_POINT('',#84804);
#25860=VERTEX_POINT('',#84808);
#25861=VERTEX_POINT('',#84819);
#25862=VERTEX_POINT('',#84823);
#25863=VERTEX_POINT('',#84834);
#25864=VERTEX_POINT('',#84838);
#25865=VERTEX_POINT('',#84849);
#25866=VERTEX_POINT('',#84853);
#25867=VERTEX_POINT('',#84864);
#25868=VERTEX_POINT('',#84868);
#25869=VERTEX_POINT('',#84879);
#25870=VERTEX_POINT('',#84883);
#25871=VERTEX_POINT('',#84894);
#25872=VERTEX_POINT('',#84898);
#25873=VERTEX_POINT('',#84921);
#25874=VERTEX_POINT('',#84922);
#25875=VERTEX_POINT('',#84926);
#25876=VERTEX_POINT('',#84928);
#25877=VERTEX_POINT('',#84939);
#25878=VERTEX_POINT('',#84943);
#25879=VERTEX_POINT('',#84954);
#25880=VERTEX_POINT('',#84958);
#25881=VERTEX_POINT('',#84969);
#25882=VERTEX_POINT('',#84973);
#25883=VERTEX_POINT('',#84984);
#25884=VERTEX_POINT('',#84988);
#25885=VERTEX_POINT('',#84999);
#25886=VERTEX_POINT('',#85003);
#25887=VERTEX_POINT('',#85014);
#25888=VERTEX_POINT('',#85018);
#25889=VERTEX_POINT('',#85029);
#25890=VERTEX_POINT('',#85033);
#25891=VERTEX_POINT('',#85044);
#25892=VERTEX_POINT('',#85048);
#25893=VERTEX_POINT('',#85059);
#25894=VERTEX_POINT('',#85063);
#25895=VERTEX_POINT('',#85074);
#25896=VERTEX_POINT('',#85078);
#25897=VERTEX_POINT('',#85089);
#25898=VERTEX_POINT('',#85093);
#25899=VERTEX_POINT('',#85104);
#25900=VERTEX_POINT('',#85108);
#25901=VERTEX_POINT('',#85119);
#25902=VERTEX_POINT('',#85123);
#25903=VERTEX_POINT('',#85134);
#25904=VERTEX_POINT('',#85138);
#25905=VERTEX_POINT('',#85149);
#25906=VERTEX_POINT('',#85153);
#25907=VERTEX_POINT('',#85164);
#25908=VERTEX_POINT('',#85168);
#25909=VERTEX_POINT('',#85174);
#25910=VERTEX_POINT('',#85176);
#25911=VERTEX_POINT('',#85200);
#25912=VERTEX_POINT('',#85201);
#25913=VERTEX_POINT('',#85205);
#25914=VERTEX_POINT('',#85207);
#25915=VERTEX_POINT('',#85218);
#25916=VERTEX_POINT('',#85222);
#25917=VERTEX_POINT('',#85233);
#25918=VERTEX_POINT('',#85237);
#25919=VERTEX_POINT('',#85248);
#25920=VERTEX_POINT('',#85252);
#25921=VERTEX_POINT('',#85263);
#25922=VERTEX_POINT('',#85267);
#25923=VERTEX_POINT('',#85278);
#25924=VERTEX_POINT('',#85282);
#25925=VERTEX_POINT('',#85293);
#25926=VERTEX_POINT('',#85297);
#25927=VERTEX_POINT('',#85320);
#25928=VERTEX_POINT('',#85321);
#25929=VERTEX_POINT('',#85325);
#25930=VERTEX_POINT('',#85327);
#25931=VERTEX_POINT('',#85338);
#25932=VERTEX_POINT('',#85342);
#25933=VERTEX_POINT('',#85353);
#25934=VERTEX_POINT('',#85357);
#25935=VERTEX_POINT('',#85368);
#25936=VERTEX_POINT('',#85372);
#25937=VERTEX_POINT('',#85383);
#25938=VERTEX_POINT('',#85387);
#25939=VERTEX_POINT('',#85398);
#25940=VERTEX_POINT('',#85402);
#25941=VERTEX_POINT('',#85413);
#25942=VERTEX_POINT('',#85417);
#25943=VERTEX_POINT('',#85428);
#25944=VERTEX_POINT('',#85432);
#25945=VERTEX_POINT('',#85443);
#25946=VERTEX_POINT('',#85447);
#25947=VERTEX_POINT('',#85458);
#25948=VERTEX_POINT('',#85462);
#25949=VERTEX_POINT('',#85473);
#25950=VERTEX_POINT('',#85477);
#25951=VERTEX_POINT('',#85501);
#25952=VERTEX_POINT('',#85502);
#25953=VERTEX_POINT('',#85506);
#25954=VERTEX_POINT('',#85508);
#25955=VERTEX_POINT('',#85519);
#25956=VERTEX_POINT('',#85523);
#25957=VERTEX_POINT('',#85534);
#25958=VERTEX_POINT('',#85538);
#25959=VERTEX_POINT('',#85544);
#25960=VERTEX_POINT('',#85546);
#25961=VERTEX_POINT('',#85555);
#25962=VERTEX_POINT('',#85559);
#25963=VERTEX_POINT('',#85570);
#25964=VERTEX_POINT('',#85574);
#25965=VERTEX_POINT('',#85585);
#25966=VERTEX_POINT('',#85589);
#25967=VERTEX_POINT('',#85595);
#25968=VERTEX_POINT('',#85597);
#25969=VERTEX_POINT('',#85601);
#25970=VERTEX_POINT('',#85603);
#25971=VERTEX_POINT('',#85607);
#25972=VERTEX_POINT('',#85609);
#25973=VERTEX_POINT('',#85623);
#25974=VERTEX_POINT('',#85624);
#25975=VERTEX_POINT('',#85628);
#25976=VERTEX_POINT('',#85630);
#25977=VERTEX_POINT('',#85641);
#25978=VERTEX_POINT('',#85645);
#25979=VERTEX_POINT('',#85656);
#25980=VERTEX_POINT('',#85660);
#25981=VERTEX_POINT('',#85671);
#25982=VERTEX_POINT('',#85675);
#25983=VERTEX_POINT('',#85686);
#25984=VERTEX_POINT('',#85690);
#25985=VERTEX_POINT('',#85701);
#25986=VERTEX_POINT('',#85705);
#25987=VERTEX_POINT('',#85716);
#25988=VERTEX_POINT('',#85720);
#25989=VERTEX_POINT('',#85743);
#25990=VERTEX_POINT('',#85744);
#25991=VERTEX_POINT('',#85748);
#25992=VERTEX_POINT('',#85750);
#25993=VERTEX_POINT('',#85761);
#25994=VERTEX_POINT('',#85765);
#25995=VERTEX_POINT('',#85776);
#25996=VERTEX_POINT('',#85780);
#25997=VERTEX_POINT('',#85791);
#25998=VERTEX_POINT('',#85795);
#25999=VERTEX_POINT('',#85806);
#26000=VERTEX_POINT('',#85810);
#26001=VERTEX_POINT('',#85821);
#26002=VERTEX_POINT('',#85825);
#26003=VERTEX_POINT('',#85836);
#26004=VERTEX_POINT('',#85840);
#26005=VERTEX_POINT('',#85851);
#26006=VERTEX_POINT('',#85855);
#26007=VERTEX_POINT('',#85866);
#26008=VERTEX_POINT('',#85870);
#26009=VERTEX_POINT('',#85881);
#26010=VERTEX_POINT('',#85885);
#26011=VERTEX_POINT('',#85896);
#26012=VERTEX_POINT('',#85900);
#26013=VERTEX_POINT('',#85924);
#26014=VERTEX_POINT('',#85925);
#26015=VERTEX_POINT('',#85929);
#26016=VERTEX_POINT('',#85931);
#26017=VERTEX_POINT('',#85942);
#26018=VERTEX_POINT('',#85946);
#26019=VERTEX_POINT('',#85957);
#26020=VERTEX_POINT('',#85961);
#26021=VERTEX_POINT('',#85972);
#26022=VERTEX_POINT('',#85976);
#26023=VERTEX_POINT('',#85987);
#26024=VERTEX_POINT('',#85991);
#26025=VERTEX_POINT('',#86002);
#26026=VERTEX_POINT('',#86006);
#26027=VERTEX_POINT('',#86017);
#26028=VERTEX_POINT('',#86021);
#26029=VERTEX_POINT('',#86044);
#26030=VERTEX_POINT('',#86045);
#26031=VERTEX_POINT('',#86049);
#26032=VERTEX_POINT('',#86051);
#26033=VERTEX_POINT('',#86062);
#26034=VERTEX_POINT('',#86066);
#26035=VERTEX_POINT('',#86077);
#26036=VERTEX_POINT('',#86081);
#26037=VERTEX_POINT('',#86092);
#26038=VERTEX_POINT('',#86096);
#26039=VERTEX_POINT('',#86107);
#26040=VERTEX_POINT('',#86111);
#26041=VERTEX_POINT('',#86122);
#26042=VERTEX_POINT('',#86126);
#26043=VERTEX_POINT('',#86137);
#26044=VERTEX_POINT('',#86141);
#26045=VERTEX_POINT('',#86152);
#26046=VERTEX_POINT('',#86156);
#26047=VERTEX_POINT('',#86179);
#26048=VERTEX_POINT('',#86180);
#26049=VERTEX_POINT('',#86184);
#26050=VERTEX_POINT('',#86186);
#26051=VERTEX_POINT('',#86197);
#26052=VERTEX_POINT('',#86201);
#26053=VERTEX_POINT('',#86212);
#26054=VERTEX_POINT('',#86216);
#26055=VERTEX_POINT('',#86227);
#26056=VERTEX_POINT('',#86231);
#26057=VERTEX_POINT('',#86242);
#26058=VERTEX_POINT('',#86246);
#26059=VERTEX_POINT('',#86257);
#26060=VERTEX_POINT('',#86261);
#26061=VERTEX_POINT('',#86272);
#26062=VERTEX_POINT('',#86276);
#26063=VERTEX_POINT('',#86287);
#26064=VERTEX_POINT('',#86291);
#26065=VERTEX_POINT('',#86302);
#26066=VERTEX_POINT('',#86306);
#26067=VERTEX_POINT('',#86317);
#26068=VERTEX_POINT('',#86321);
#26069=VERTEX_POINT('',#86332);
#26070=VERTEX_POINT('',#86336);
#26071=VERTEX_POINT('',#86347);
#26072=VERTEX_POINT('',#86351);
#26073=VERTEX_POINT('',#86362);
#26074=VERTEX_POINT('',#86366);
#26075=VERTEX_POINT('',#86377);
#26076=VERTEX_POINT('',#86381);
#26077=VERTEX_POINT('',#86392);
#26078=VERTEX_POINT('',#86396);
#26079=VERTEX_POINT('',#86423);
#26080=VERTEX_POINT('',#86424);
#26081=VERTEX_POINT('',#86428);
#26082=VERTEX_POINT('',#86430);
#26083=VERTEX_POINT('',#86441);
#26084=VERTEX_POINT('',#86445);
#26085=VERTEX_POINT('',#86456);
#26086=VERTEX_POINT('',#86460);
#26087=VERTEX_POINT('',#86471);
#26088=VERTEX_POINT('',#86475);
#26089=VERTEX_POINT('',#86486);
#26090=VERTEX_POINT('',#86490);
#26091=VERTEX_POINT('',#86501);
#26092=VERTEX_POINT('',#86505);
#26093=VERTEX_POINT('',#86516);
#26094=VERTEX_POINT('',#86520);
#26095=VERTEX_POINT('',#86543);
#26096=VERTEX_POINT('',#86544);
#26097=VERTEX_POINT('',#86548);
#26098=VERTEX_POINT('',#86550);
#26099=VERTEX_POINT('',#86561);
#26100=VERTEX_POINT('',#86565);
#26101=VERTEX_POINT('',#86576);
#26102=VERTEX_POINT('',#86580);
#26103=VERTEX_POINT('',#86591);
#26104=VERTEX_POINT('',#86595);
#26105=VERTEX_POINT('',#86606);
#26106=VERTEX_POINT('',#86610);
#26107=VERTEX_POINT('',#86621);
#26108=VERTEX_POINT('',#86625);
#26109=VERTEX_POINT('',#86636);
#26110=VERTEX_POINT('',#86640);
#26111=VERTEX_POINT('',#86651);
#26112=VERTEX_POINT('',#86655);
#26113=VERTEX_POINT('',#86666);
#26114=VERTEX_POINT('',#86670);
#26115=VERTEX_POINT('',#86681);
#26116=VERTEX_POINT('',#86685);
#26117=VERTEX_POINT('',#86696);
#26118=VERTEX_POINT('',#86700);
#26119=VERTEX_POINT('',#86724);
#26120=VERTEX_POINT('',#86725);
#26121=VERTEX_POINT('',#86729);
#26122=VERTEX_POINT('',#86731);
#26123=VERTEX_POINT('',#86742);
#26124=VERTEX_POINT('',#86746);
#26125=VERTEX_POINT('',#86757);
#26126=VERTEX_POINT('',#86761);
#26127=VERTEX_POINT('',#86772);
#26128=VERTEX_POINT('',#86776);
#26129=VERTEX_POINT('',#86787);
#26130=VERTEX_POINT('',#86791);
#26131=VERTEX_POINT('',#86802);
#26132=VERTEX_POINT('',#86806);
#26133=VERTEX_POINT('',#86817);
#26134=VERTEX_POINT('',#86821);
#26135=VERTEX_POINT('',#86844);
#26136=VERTEX_POINT('',#86845);
#26137=VERTEX_POINT('',#86849);
#26138=VERTEX_POINT('',#86851);
#26139=VERTEX_POINT('',#86862);
#26140=VERTEX_POINT('',#86866);
#26141=VERTEX_POINT('',#86877);
#26142=VERTEX_POINT('',#86881);
#26143=VERTEX_POINT('',#86892);
#26144=VERTEX_POINT('',#86896);
#26145=VERTEX_POINT('',#86907);
#26146=VERTEX_POINT('',#86911);
#26147=VERTEX_POINT('',#86922);
#26148=VERTEX_POINT('',#86926);
#26149=VERTEX_POINT('',#86937);
#26150=VERTEX_POINT('',#86941);
#26151=VERTEX_POINT('',#86952);
#26152=VERTEX_POINT('',#86956);
#26153=VERTEX_POINT('',#86967);
#26154=VERTEX_POINT('',#86971);
#26155=VERTEX_POINT('',#86982);
#26156=VERTEX_POINT('',#86986);
#26157=VERTEX_POINT('',#86997);
#26158=VERTEX_POINT('',#87001);
#26159=VERTEX_POINT('',#87012);
#26160=VERTEX_POINT('',#87016);
#26161=VERTEX_POINT('',#87027);
#26162=VERTEX_POINT('',#87031);
#26163=VERTEX_POINT('',#87042);
#26164=VERTEX_POINT('',#87046);
#26165=VERTEX_POINT('',#87057);
#26166=VERTEX_POINT('',#87061);
#26167=VERTEX_POINT('',#87072);
#26168=VERTEX_POINT('',#87076);
#26169=VERTEX_POINT('',#87087);
#26170=VERTEX_POINT('',#87091);
#26171=VERTEX_POINT('',#87102);
#26172=VERTEX_POINT('',#87106);
#26173=VERTEX_POINT('',#87117);
#26174=VERTEX_POINT('',#87121);
#26175=VERTEX_POINT('',#87132);
#26176=VERTEX_POINT('',#87136);
#26177=VERTEX_POINT('',#87142);
#26178=VERTEX_POINT('',#87144);
#26179=VERTEX_POINT('',#87163);
#26180=VERTEX_POINT('',#87164);
#26181=VERTEX_POINT('',#87166);
#26182=VERTEX_POINT('',#87168);
#26183=VERTEX_POINT('',#87172);
#26184=VERTEX_POINT('',#87174);
#26185=VERTEX_POINT('',#87178);
#26186=VERTEX_POINT('',#87180);
#26187=VERTEX_POINT('',#87188);
#26188=VERTEX_POINT('',#87189);
#26189=VERTEX_POINT('',#87191);
#26190=VERTEX_POINT('',#87193);
#26191=VERTEX_POINT('',#87197);
#26192=VERTEX_POINT('',#87199);
#26193=VERTEX_POINT('',#87203);
#26194=VERTEX_POINT('',#87205);
#26195=VERTEX_POINT('',#87213);
#26196=VERTEX_POINT('',#87214);
#26197=VERTEX_POINT('',#87216);
#26198=VERTEX_POINT('',#87218);
#26199=VERTEX_POINT('',#87222);
#26200=VERTEX_POINT('',#87224);
#26201=VERTEX_POINT('',#87228);
#26202=VERTEX_POINT('',#87230);
#26203=VERTEX_POINT('',#87238);
#26204=VERTEX_POINT('',#87239);
#26205=VERTEX_POINT('',#87241);
#26206=VERTEX_POINT('',#87243);
#26207=VERTEX_POINT('',#87247);
#26208=VERTEX_POINT('',#87249);
#26209=VERTEX_POINT('',#87253);
#26210=VERTEX_POINT('',#87255);
#26211=VERTEX_POINT('',#87263);
#26212=VERTEX_POINT('',#87264);
#26213=VERTEX_POINT('',#87266);
#26214=VERTEX_POINT('',#87268);
#26215=VERTEX_POINT('',#87272);
#26216=VERTEX_POINT('',#87274);
#26217=VERTEX_POINT('',#87278);
#26218=VERTEX_POINT('',#87280);
#26219=VERTEX_POINT('',#87288);
#26220=VERTEX_POINT('',#87289);
#26221=VERTEX_POINT('',#87291);
#26222=VERTEX_POINT('',#87293);
#26223=VERTEX_POINT('',#87297);
#26224=VERTEX_POINT('',#87299);
#26225=VERTEX_POINT('',#87303);
#26226=VERTEX_POINT('',#87305);
#26227=VERTEX_POINT('',#87313);
#26228=VERTEX_POINT('',#87314);
#26229=VERTEX_POINT('',#87316);
#26230=VERTEX_POINT('',#87318);
#26231=VERTEX_POINT('',#87322);
#26232=VERTEX_POINT('',#87324);
#26233=VERTEX_POINT('',#87328);
#26234=VERTEX_POINT('',#87330);
#26235=VERTEX_POINT('',#87338);
#26236=VERTEX_POINT('',#87339);
#26237=VERTEX_POINT('',#87341);
#26238=VERTEX_POINT('',#87343);
#26239=VERTEX_POINT('',#87347);
#26240=VERTEX_POINT('',#87349);
#26241=VERTEX_POINT('',#87353);
#26242=VERTEX_POINT('',#87355);
#26243=VERTEX_POINT('',#87363);
#26244=VERTEX_POINT('',#87364);
#26245=VERTEX_POINT('',#87366);
#26246=VERTEX_POINT('',#87368);
#26247=VERTEX_POINT('',#87372);
#26248=VERTEX_POINT('',#87374);
#26249=VERTEX_POINT('',#87378);
#26250=VERTEX_POINT('',#87380);
#26251=VERTEX_POINT('',#87388);
#26252=VERTEX_POINT('',#87389);
#26253=VERTEX_POINT('',#87391);
#26254=VERTEX_POINT('',#87393);
#26255=VERTEX_POINT('',#87397);
#26256=VERTEX_POINT('',#87399);
#26257=VERTEX_POINT('',#87403);
#26258=VERTEX_POINT('',#87405);
#26259=VERTEX_POINT('',#87413);
#26260=VERTEX_POINT('',#87414);
#26261=VERTEX_POINT('',#87416);
#26262=VERTEX_POINT('',#87418);
#26263=VERTEX_POINT('',#87422);
#26264=VERTEX_POINT('',#87424);
#26265=VERTEX_POINT('',#87428);
#26266=VERTEX_POINT('',#87430);
#26267=VERTEX_POINT('',#87438);
#26268=VERTEX_POINT('',#87439);
#26269=VERTEX_POINT('',#87441);
#26270=VERTEX_POINT('',#87443);
#26271=VERTEX_POINT('',#87447);
#26272=VERTEX_POINT('',#87449);
#26273=VERTEX_POINT('',#87453);
#26274=VERTEX_POINT('',#87455);
#26275=VERTEX_POINT('',#87463);
#26276=VERTEX_POINT('',#87464);
#26277=VERTEX_POINT('',#87466);
#26278=VERTEX_POINT('',#87468);
#26279=VERTEX_POINT('',#87472);
#26280=VERTEX_POINT('',#87474);
#26281=VERTEX_POINT('',#87478);
#26282=VERTEX_POINT('',#87480);
#26283=VERTEX_POINT('',#87488);
#26284=VERTEX_POINT('',#87489);
#26285=VERTEX_POINT('',#87491);
#26286=VERTEX_POINT('',#87493);
#26287=VERTEX_POINT('',#87497);
#26288=VERTEX_POINT('',#87499);
#26289=VERTEX_POINT('',#87503);
#26290=VERTEX_POINT('',#87505);
#26291=VERTEX_POINT('',#87513);
#26292=VERTEX_POINT('',#87514);
#26293=VERTEX_POINT('',#87516);
#26294=VERTEX_POINT('',#87518);
#26295=VERTEX_POINT('',#87522);
#26296=VERTEX_POINT('',#87524);
#26297=VERTEX_POINT('',#87528);
#26298=VERTEX_POINT('',#87530);
#26299=VERTEX_POINT('',#87538);
#26300=VERTEX_POINT('',#87539);
#26301=VERTEX_POINT('',#87541);
#26302=VERTEX_POINT('',#87543);
#26303=VERTEX_POINT('',#87547);
#26304=VERTEX_POINT('',#87549);
#26305=VERTEX_POINT('',#87553);
#26306=VERTEX_POINT('',#87555);
#26307=VERTEX_POINT('',#87563);
#26308=VERTEX_POINT('',#87564);
#26309=VERTEX_POINT('',#87566);
#26310=VERTEX_POINT('',#87568);
#26311=VERTEX_POINT('',#87572);
#26312=VERTEX_POINT('',#87574);
#26313=VERTEX_POINT('',#87578);
#26314=VERTEX_POINT('',#87580);
#26315=VERTEX_POINT('',#87588);
#26316=VERTEX_POINT('',#87589);
#26317=VERTEX_POINT('',#87591);
#26318=VERTEX_POINT('',#87593);
#26319=VERTEX_POINT('',#87597);
#26320=VERTEX_POINT('',#87599);
#26321=VERTEX_POINT('',#87603);
#26322=VERTEX_POINT('',#87605);
#26323=VERTEX_POINT('',#87613);
#26324=VERTEX_POINT('',#87614);
#26325=VERTEX_POINT('',#87616);
#26326=VERTEX_POINT('',#87618);
#26327=VERTEX_POINT('',#87622);
#26328=VERTEX_POINT('',#87624);
#26329=VERTEX_POINT('',#87628);
#26330=VERTEX_POINT('',#87630);
#26331=VERTEX_POINT('',#87638);
#26332=VERTEX_POINT('',#87639);
#26333=VERTEX_POINT('',#87641);
#26334=VERTEX_POINT('',#87643);
#26335=VERTEX_POINT('',#87647);
#26336=VERTEX_POINT('',#87649);
#26337=VERTEX_POINT('',#87653);
#26338=VERTEX_POINT('',#87655);
#26339=VERTEX_POINT('',#87663);
#26340=VERTEX_POINT('',#87664);
#26341=VERTEX_POINT('',#87666);
#26342=VERTEX_POINT('',#87668);
#26343=VERTEX_POINT('',#87672);
#26344=VERTEX_POINT('',#87674);
#26345=VERTEX_POINT('',#87678);
#26346=VERTEX_POINT('',#87680);
#26347=VERTEX_POINT('',#87688);
#26348=VERTEX_POINT('',#87689);
#26349=VERTEX_POINT('',#87691);
#26350=VERTEX_POINT('',#87693);
#26351=VERTEX_POINT('',#87697);
#26352=VERTEX_POINT('',#87699);
#26353=VERTEX_POINT('',#87703);
#26354=VERTEX_POINT('',#87705);
#26355=VERTEX_POINT('',#87713);
#26356=VERTEX_POINT('',#87714);
#26357=VERTEX_POINT('',#87716);
#26358=VERTEX_POINT('',#87718);
#26359=VERTEX_POINT('',#87722);
#26360=VERTEX_POINT('',#87724);
#26361=VERTEX_POINT('',#87728);
#26362=VERTEX_POINT('',#87730);
#26363=VERTEX_POINT('',#87738);
#26364=VERTEX_POINT('',#87739);
#26365=VERTEX_POINT('',#87741);
#26366=VERTEX_POINT('',#87743);
#26367=VERTEX_POINT('',#87747);
#26368=VERTEX_POINT('',#87749);
#26369=VERTEX_POINT('',#87753);
#26370=VERTEX_POINT('',#87755);
#26371=VERTEX_POINT('',#87763);
#26372=VERTEX_POINT('',#87764);
#26373=VERTEX_POINT('',#87766);
#26374=VERTEX_POINT('',#87768);
#26375=VERTEX_POINT('',#87772);
#26376=VERTEX_POINT('',#87774);
#26377=VERTEX_POINT('',#87778);
#26378=VERTEX_POINT('',#87780);
#26379=VERTEX_POINT('',#87788);
#26380=VERTEX_POINT('',#87789);
#26381=VERTEX_POINT('',#87791);
#26382=VERTEX_POINT('',#87793);
#26383=VERTEX_POINT('',#87797);
#26384=VERTEX_POINT('',#87799);
#26385=VERTEX_POINT('',#87803);
#26386=VERTEX_POINT('',#87805);
#26387=VERTEX_POINT('',#87813);
#26388=VERTEX_POINT('',#87814);
#26389=VERTEX_POINT('',#87816);
#26390=VERTEX_POINT('',#87818);
#26391=VERTEX_POINT('',#87822);
#26392=VERTEX_POINT('',#87824);
#26393=VERTEX_POINT('',#87828);
#26394=VERTEX_POINT('',#87830);
#26395=VERTEX_POINT('',#87838);
#26396=VERTEX_POINT('',#87839);
#26397=VERTEX_POINT('',#87841);
#26398=VERTEX_POINT('',#87843);
#26399=VERTEX_POINT('',#87847);
#26400=VERTEX_POINT('',#87849);
#26401=VERTEX_POINT('',#87853);
#26402=VERTEX_POINT('',#87855);
#26403=VERTEX_POINT('',#87863);
#26404=VERTEX_POINT('',#87864);
#26405=VERTEX_POINT('',#87866);
#26406=VERTEX_POINT('',#87868);
#26407=VERTEX_POINT('',#87872);
#26408=VERTEX_POINT('',#87874);
#26409=VERTEX_POINT('',#87878);
#26410=VERTEX_POINT('',#87880);
#26411=VERTEX_POINT('',#87888);
#26412=VERTEX_POINT('',#87889);
#26413=VERTEX_POINT('',#87891);
#26414=VERTEX_POINT('',#87893);
#26415=VERTEX_POINT('',#87897);
#26416=VERTEX_POINT('',#87899);
#26417=VERTEX_POINT('',#87903);
#26418=VERTEX_POINT('',#87905);
#26419=VERTEX_POINT('',#87913);
#26420=VERTEX_POINT('',#87914);
#26421=VERTEX_POINT('',#87916);
#26422=VERTEX_POINT('',#87918);
#26423=VERTEX_POINT('',#87922);
#26424=VERTEX_POINT('',#87924);
#26425=VERTEX_POINT('',#87928);
#26426=VERTEX_POINT('',#87930);
#26427=VERTEX_POINT('',#87938);
#26428=VERTEX_POINT('',#87939);
#26429=VERTEX_POINT('',#87941);
#26430=VERTEX_POINT('',#87943);
#26431=VERTEX_POINT('',#87947);
#26432=VERTEX_POINT('',#87949);
#26433=VERTEX_POINT('',#87953);
#26434=VERTEX_POINT('',#87955);
#26435=VERTEX_POINT('',#87963);
#26436=VERTEX_POINT('',#87964);
#26437=VERTEX_POINT('',#87966);
#26438=VERTEX_POINT('',#87968);
#26439=VERTEX_POINT('',#87972);
#26440=VERTEX_POINT('',#87974);
#26441=VERTEX_POINT('',#87978);
#26442=VERTEX_POINT('',#87980);
#26443=VERTEX_POINT('',#87988);
#26444=VERTEX_POINT('',#87989);
#26445=VERTEX_POINT('',#87991);
#26446=VERTEX_POINT('',#87993);
#26447=VERTEX_POINT('',#87997);
#26448=VERTEX_POINT('',#87999);
#26449=VERTEX_POINT('',#88003);
#26450=VERTEX_POINT('',#88005);
#26451=VERTEX_POINT('',#88013);
#26452=VERTEX_POINT('',#88014);
#26453=VERTEX_POINT('',#88016);
#26454=VERTEX_POINT('',#88018);
#26455=VERTEX_POINT('',#88022);
#26456=VERTEX_POINT('',#88024);
#26457=VERTEX_POINT('',#88028);
#26458=VERTEX_POINT('',#88030);
#26459=VERTEX_POINT('',#88038);
#26460=VERTEX_POINT('',#88039);
#26461=VERTEX_POINT('',#88041);
#26462=VERTEX_POINT('',#88043);
#26463=VERTEX_POINT('',#88047);
#26464=VERTEX_POINT('',#88049);
#26465=VERTEX_POINT('',#88053);
#26466=VERTEX_POINT('',#88055);
#26467=VERTEX_POINT('',#88063);
#26468=VERTEX_POINT('',#88064);
#26469=VERTEX_POINT('',#88066);
#26470=VERTEX_POINT('',#88068);
#26471=VERTEX_POINT('',#88072);
#26472=VERTEX_POINT('',#88074);
#26473=VERTEX_POINT('',#88078);
#26474=VERTEX_POINT('',#88080);
#26475=VERTEX_POINT('',#88088);
#26476=VERTEX_POINT('',#88089);
#26477=VERTEX_POINT('',#88091);
#26478=VERTEX_POINT('',#88093);
#26479=VERTEX_POINT('',#88097);
#26480=VERTEX_POINT('',#88099);
#26481=VERTEX_POINT('',#88103);
#26482=VERTEX_POINT('',#88105);
#26483=VERTEX_POINT('',#88113);
#26484=VERTEX_POINT('',#88114);
#26485=VERTEX_POINT('',#88116);
#26486=VERTEX_POINT('',#88118);
#26487=VERTEX_POINT('',#88122);
#26488=VERTEX_POINT('',#88124);
#26489=VERTEX_POINT('',#88128);
#26490=VERTEX_POINT('',#88130);
#26491=VERTEX_POINT('',#88138);
#26492=VERTEX_POINT('',#88139);
#26493=VERTEX_POINT('',#88141);
#26494=VERTEX_POINT('',#88143);
#26495=VERTEX_POINT('',#88147);
#26496=VERTEX_POINT('',#88149);
#26497=VERTEX_POINT('',#88153);
#26498=VERTEX_POINT('',#88155);
#26499=VERTEX_POINT('',#88163);
#26500=VERTEX_POINT('',#88164);
#26501=VERTEX_POINT('',#88166);
#26502=VERTEX_POINT('',#88168);
#26503=VERTEX_POINT('',#88172);
#26504=VERTEX_POINT('',#88174);
#26505=VERTEX_POINT('',#88178);
#26506=VERTEX_POINT('',#88180);
#26507=VERTEX_POINT('',#88188);
#26508=VERTEX_POINT('',#88189);
#26509=VERTEX_POINT('',#88191);
#26510=VERTEX_POINT('',#88193);
#26511=VERTEX_POINT('',#88197);
#26512=VERTEX_POINT('',#88199);
#26513=VERTEX_POINT('',#88203);
#26514=VERTEX_POINT('',#88205);
#26515=VERTEX_POINT('',#88213);
#26516=VERTEX_POINT('',#88214);
#26517=VERTEX_POINT('',#88216);
#26518=VERTEX_POINT('',#88218);
#26519=VERTEX_POINT('',#88222);
#26520=VERTEX_POINT('',#88224);
#26521=VERTEX_POINT('',#88228);
#26522=VERTEX_POINT('',#88230);
#26523=VERTEX_POINT('',#88238);
#26524=VERTEX_POINT('',#88239);
#26525=VERTEX_POINT('',#88241);
#26526=VERTEX_POINT('',#88243);
#26527=VERTEX_POINT('',#88247);
#26528=VERTEX_POINT('',#88249);
#26529=VERTEX_POINT('',#88253);
#26530=VERTEX_POINT('',#88255);
#26531=VERTEX_POINT('',#88263);
#26532=VERTEX_POINT('',#88264);
#26533=VERTEX_POINT('',#88266);
#26534=VERTEX_POINT('',#88268);
#26535=VERTEX_POINT('',#88272);
#26536=VERTEX_POINT('',#88274);
#26537=VERTEX_POINT('',#88278);
#26538=VERTEX_POINT('',#88280);
#26539=VERTEX_POINT('',#88288);
#26540=VERTEX_POINT('',#88289);
#26541=VERTEX_POINT('',#88291);
#26542=VERTEX_POINT('',#88293);
#26543=VERTEX_POINT('',#88297);
#26544=VERTEX_POINT('',#88299);
#26545=VERTEX_POINT('',#88303);
#26546=VERTEX_POINT('',#88305);
#26547=VERTEX_POINT('',#88313);
#26548=VERTEX_POINT('',#88314);
#26549=VERTEX_POINT('',#88316);
#26550=VERTEX_POINT('',#88318);
#26551=VERTEX_POINT('',#88322);
#26552=VERTEX_POINT('',#88324);
#26553=VERTEX_POINT('',#88328);
#26554=VERTEX_POINT('',#88330);
#26555=VERTEX_POINT('',#88338);
#26556=VERTEX_POINT('',#88339);
#26557=VERTEX_POINT('',#88341);
#26558=VERTEX_POINT('',#88343);
#26559=VERTEX_POINT('',#88347);
#26560=VERTEX_POINT('',#88349);
#26561=VERTEX_POINT('',#88353);
#26562=VERTEX_POINT('',#88355);
#26563=VERTEX_POINT('',#88363);
#26564=VERTEX_POINT('',#88364);
#26565=VERTEX_POINT('',#88366);
#26566=VERTEX_POINT('',#88368);
#26567=VERTEX_POINT('',#88372);
#26568=VERTEX_POINT('',#88374);
#26569=VERTEX_POINT('',#88378);
#26570=VERTEX_POINT('',#88380);
#26571=VERTEX_POINT('',#88388);
#26572=VERTEX_POINT('',#88389);
#26573=VERTEX_POINT('',#88391);
#26574=VERTEX_POINT('',#88393);
#26575=VERTEX_POINT('',#88397);
#26576=VERTEX_POINT('',#88399);
#26577=VERTEX_POINT('',#88403);
#26578=VERTEX_POINT('',#88405);
#26579=VERTEX_POINT('',#88413);
#26580=VERTEX_POINT('',#88414);
#26581=VERTEX_POINT('',#88416);
#26582=VERTEX_POINT('',#88418);
#26583=VERTEX_POINT('',#88422);
#26584=VERTEX_POINT('',#88424);
#26585=VERTEX_POINT('',#88428);
#26586=VERTEX_POINT('',#88430);
#26587=VERTEX_POINT('',#88438);
#26588=VERTEX_POINT('',#88439);
#26589=VERTEX_POINT('',#88441);
#26590=VERTEX_POINT('',#88443);
#26591=VERTEX_POINT('',#88447);
#26592=VERTEX_POINT('',#88449);
#26593=VERTEX_POINT('',#88453);
#26594=VERTEX_POINT('',#88455);
#26595=VERTEX_POINT('',#88463);
#26596=VERTEX_POINT('',#88464);
#26597=VERTEX_POINT('',#88466);
#26598=VERTEX_POINT('',#88468);
#26599=VERTEX_POINT('',#88472);
#26600=VERTEX_POINT('',#88474);
#26601=VERTEX_POINT('',#88478);
#26602=VERTEX_POINT('',#88480);
#26603=VERTEX_POINT('',#88488);
#26604=VERTEX_POINT('',#88489);
#26605=VERTEX_POINT('',#88491);
#26606=VERTEX_POINT('',#88493);
#26607=VERTEX_POINT('',#88497);
#26608=VERTEX_POINT('',#88499);
#26609=VERTEX_POINT('',#88503);
#26610=VERTEX_POINT('',#88505);
#26611=VERTEX_POINT('',#88513);
#26612=VERTEX_POINT('',#88514);
#26613=VERTEX_POINT('',#88516);
#26614=VERTEX_POINT('',#88518);
#26615=VERTEX_POINT('',#88522);
#26616=VERTEX_POINT('',#88524);
#26617=VERTEX_POINT('',#88528);
#26618=VERTEX_POINT('',#88530);
#26619=VERTEX_POINT('',#88538);
#26620=VERTEX_POINT('',#88539);
#26621=VERTEX_POINT('',#88541);
#26622=VERTEX_POINT('',#88543);
#26623=VERTEX_POINT('',#88547);
#26624=VERTEX_POINT('',#88549);
#26625=VERTEX_POINT('',#88553);
#26626=VERTEX_POINT('',#88555);
#26627=VERTEX_POINT('',#88563);
#26628=VERTEX_POINT('',#88564);
#26629=VERTEX_POINT('',#88566);
#26630=VERTEX_POINT('',#88568);
#26631=VERTEX_POINT('',#88572);
#26632=VERTEX_POINT('',#88574);
#26633=VERTEX_POINT('',#88578);
#26634=VERTEX_POINT('',#88580);
#26635=VERTEX_POINT('',#88588);
#26636=VERTEX_POINT('',#88589);
#26637=VERTEX_POINT('',#88591);
#26638=VERTEX_POINT('',#88593);
#26639=VERTEX_POINT('',#88597);
#26640=VERTEX_POINT('',#88599);
#26641=VERTEX_POINT('',#88603);
#26642=VERTEX_POINT('',#88605);
#26643=VERTEX_POINT('',#88613);
#26644=VERTEX_POINT('',#88614);
#26645=VERTEX_POINT('',#88616);
#26646=VERTEX_POINT('',#88618);
#26647=VERTEX_POINT('',#88622);
#26648=VERTEX_POINT('',#88624);
#26649=VERTEX_POINT('',#88628);
#26650=VERTEX_POINT('',#88630);
#26651=VERTEX_POINT('',#88638);
#26652=VERTEX_POINT('',#88639);
#26653=VERTEX_POINT('',#88641);
#26654=VERTEX_POINT('',#88643);
#26655=VERTEX_POINT('',#88647);
#26656=VERTEX_POINT('',#88649);
#26657=VERTEX_POINT('',#88653);
#26658=VERTEX_POINT('',#88655);
#26659=VERTEX_POINT('',#88663);
#26660=VERTEX_POINT('',#88664);
#26661=VERTEX_POINT('',#88666);
#26662=VERTEX_POINT('',#88668);
#26663=VERTEX_POINT('',#88672);
#26664=VERTEX_POINT('',#88674);
#26665=VERTEX_POINT('',#88678);
#26666=VERTEX_POINT('',#88680);
#26667=VERTEX_POINT('',#88688);
#26668=VERTEX_POINT('',#88689);
#26669=VERTEX_POINT('',#88691);
#26670=VERTEX_POINT('',#88693);
#26671=VERTEX_POINT('',#88697);
#26672=VERTEX_POINT('',#88699);
#26673=VERTEX_POINT('',#88703);
#26674=VERTEX_POINT('',#88705);
#26675=VERTEX_POINT('',#88713);
#26676=VERTEX_POINT('',#88714);
#26677=VERTEX_POINT('',#88716);
#26678=VERTEX_POINT('',#88718);
#26679=VERTEX_POINT('',#88722);
#26680=VERTEX_POINT('',#88724);
#26681=VERTEX_POINT('',#88728);
#26682=VERTEX_POINT('',#88730);
#26683=VERTEX_POINT('',#88738);
#26684=VERTEX_POINT('',#88739);
#26685=VERTEX_POINT('',#88741);
#26686=VERTEX_POINT('',#88743);
#26687=VERTEX_POINT('',#88747);
#26688=VERTEX_POINT('',#88749);
#26689=VERTEX_POINT('',#88753);
#26690=VERTEX_POINT('',#88755);
#26691=VERTEX_POINT('',#88763);
#26692=VERTEX_POINT('',#88764);
#26693=VERTEX_POINT('',#88766);
#26694=VERTEX_POINT('',#88768);
#26695=VERTEX_POINT('',#88772);
#26696=VERTEX_POINT('',#88774);
#26697=VERTEX_POINT('',#88778);
#26698=VERTEX_POINT('',#88780);
#26699=VERTEX_POINT('',#88788);
#26700=VERTEX_POINT('',#88789);
#26701=VERTEX_POINT('',#88791);
#26702=VERTEX_POINT('',#88793);
#26703=VERTEX_POINT('',#88797);
#26704=VERTEX_POINT('',#88799);
#26705=VERTEX_POINT('',#88803);
#26706=VERTEX_POINT('',#88805);
#26707=VERTEX_POINT('',#88813);
#26708=VERTEX_POINT('',#88814);
#26709=VERTEX_POINT('',#88816);
#26710=VERTEX_POINT('',#88818);
#26711=VERTEX_POINT('',#88822);
#26712=VERTEX_POINT('',#88824);
#26713=VERTEX_POINT('',#88828);
#26714=VERTEX_POINT('',#88830);
#26715=VERTEX_POINT('',#88838);
#26716=VERTEX_POINT('',#88839);
#26717=VERTEX_POINT('',#88841);
#26718=VERTEX_POINT('',#88843);
#26719=VERTEX_POINT('',#88847);
#26720=VERTEX_POINT('',#88849);
#26721=VERTEX_POINT('',#88853);
#26722=VERTEX_POINT('',#88855);
#26723=VERTEX_POINT('',#88863);
#26724=VERTEX_POINT('',#88864);
#26725=VERTEX_POINT('',#88866);
#26726=VERTEX_POINT('',#88868);
#26727=VERTEX_POINT('',#88872);
#26728=VERTEX_POINT('',#88874);
#26729=VERTEX_POINT('',#88878);
#26730=VERTEX_POINT('',#88880);
#26731=VERTEX_POINT('',#88888);
#26732=VERTEX_POINT('',#88889);
#26733=VERTEX_POINT('',#88891);
#26734=VERTEX_POINT('',#88893);
#26735=VERTEX_POINT('',#88897);
#26736=VERTEX_POINT('',#88899);
#26737=VERTEX_POINT('',#88903);
#26738=VERTEX_POINT('',#88905);
#26739=VERTEX_POINT('',#88913);
#26740=VERTEX_POINT('',#88914);
#26741=VERTEX_POINT('',#88916);
#26742=VERTEX_POINT('',#88918);
#26743=VERTEX_POINT('',#88922);
#26744=VERTEX_POINT('',#88924);
#26745=VERTEX_POINT('',#88928);
#26746=VERTEX_POINT('',#88930);
#26747=VERTEX_POINT('',#88938);
#26748=VERTEX_POINT('',#88939);
#26749=VERTEX_POINT('',#88941);
#26750=VERTEX_POINT('',#88943);
#26751=VERTEX_POINT('',#88947);
#26752=VERTEX_POINT('',#88949);
#26753=VERTEX_POINT('',#88953);
#26754=VERTEX_POINT('',#88955);
#26755=VERTEX_POINT('',#88963);
#26756=VERTEX_POINT('',#88964);
#26757=VERTEX_POINT('',#88966);
#26758=VERTEX_POINT('',#88968);
#26759=VERTEX_POINT('',#88972);
#26760=VERTEX_POINT('',#88974);
#26761=VERTEX_POINT('',#88978);
#26762=VERTEX_POINT('',#88980);
#26763=VERTEX_POINT('',#88988);
#26764=VERTEX_POINT('',#88989);
#26765=VERTEX_POINT('',#88991);
#26766=VERTEX_POINT('',#88993);
#26767=VERTEX_POINT('',#88997);
#26768=VERTEX_POINT('',#88999);
#26769=VERTEX_POINT('',#89003);
#26770=VERTEX_POINT('',#89005);
#26771=VERTEX_POINT('',#89013);
#26772=VERTEX_POINT('',#89014);
#26773=VERTEX_POINT('',#89016);
#26774=VERTEX_POINT('',#89018);
#26775=VERTEX_POINT('',#89022);
#26776=VERTEX_POINT('',#89024);
#26777=VERTEX_POINT('',#89028);
#26778=VERTEX_POINT('',#89030);
#26779=VERTEX_POINT('',#89038);
#26780=VERTEX_POINT('',#89039);
#26781=VERTEX_POINT('',#89041);
#26782=VERTEX_POINT('',#89043);
#26783=VERTEX_POINT('',#89047);
#26784=VERTEX_POINT('',#89049);
#26785=VERTEX_POINT('',#89053);
#26786=VERTEX_POINT('',#89055);
#26787=VERTEX_POINT('',#89063);
#26788=VERTEX_POINT('',#89064);
#26789=VERTEX_POINT('',#89066);
#26790=VERTEX_POINT('',#89068);
#26791=VERTEX_POINT('',#89072);
#26792=VERTEX_POINT('',#89074);
#26793=VERTEX_POINT('',#89078);
#26794=VERTEX_POINT('',#89080);
#26795=VERTEX_POINT('',#89088);
#26796=VERTEX_POINT('',#89089);
#26797=VERTEX_POINT('',#89091);
#26798=VERTEX_POINT('',#89093);
#26799=VERTEX_POINT('',#89097);
#26800=VERTEX_POINT('',#89099);
#26801=VERTEX_POINT('',#89103);
#26802=VERTEX_POINT('',#89105);
#26803=VERTEX_POINT('',#89113);
#26804=VERTEX_POINT('',#89114);
#26805=VERTEX_POINT('',#89116);
#26806=VERTEX_POINT('',#89118);
#26807=VERTEX_POINT('',#89122);
#26808=VERTEX_POINT('',#89124);
#26809=VERTEX_POINT('',#89128);
#26810=VERTEX_POINT('',#89130);
#26811=VERTEX_POINT('',#89138);
#26812=VERTEX_POINT('',#89139);
#26813=VERTEX_POINT('',#89141);
#26814=VERTEX_POINT('',#89143);
#26815=VERTEX_POINT('',#89147);
#26816=VERTEX_POINT('',#89149);
#26817=VERTEX_POINT('',#89153);
#26818=VERTEX_POINT('',#89155);
#26819=VERTEX_POINT('',#89163);
#26820=VERTEX_POINT('',#89164);
#26821=VERTEX_POINT('',#89166);
#26822=VERTEX_POINT('',#89168);
#26823=VERTEX_POINT('',#89172);
#26824=VERTEX_POINT('',#89174);
#26825=VERTEX_POINT('',#89178);
#26826=VERTEX_POINT('',#89180);
#26827=VERTEX_POINT('',#89188);
#26828=VERTEX_POINT('',#89189);
#26829=VERTEX_POINT('',#89191);
#26830=VERTEX_POINT('',#89193);
#26831=VERTEX_POINT('',#89197);
#26832=VERTEX_POINT('',#89199);
#26833=VERTEX_POINT('',#89203);
#26834=VERTEX_POINT('',#89205);
#26835=VERTEX_POINT('',#89213);
#26836=VERTEX_POINT('',#89214);
#26837=VERTEX_POINT('',#89216);
#26838=VERTEX_POINT('',#89218);
#26839=VERTEX_POINT('',#89222);
#26840=VERTEX_POINT('',#89224);
#26841=VERTEX_POINT('',#89228);
#26842=VERTEX_POINT('',#89230);
#26843=VERTEX_POINT('',#89238);
#26844=VERTEX_POINT('',#89239);
#26845=VERTEX_POINT('',#89241);
#26846=VERTEX_POINT('',#89243);
#26847=VERTEX_POINT('',#89247);
#26848=VERTEX_POINT('',#89249);
#26849=VERTEX_POINT('',#89253);
#26850=VERTEX_POINT('',#89255);
#26851=VERTEX_POINT('',#89263);
#26852=VERTEX_POINT('',#89264);
#26853=VERTEX_POINT('',#89266);
#26854=VERTEX_POINT('',#89268);
#26855=VERTEX_POINT('',#89272);
#26856=VERTEX_POINT('',#89274);
#26857=VERTEX_POINT('',#89278);
#26858=VERTEX_POINT('',#89280);
#26859=VERTEX_POINT('',#89288);
#26860=VERTEX_POINT('',#89289);
#26861=VERTEX_POINT('',#89291);
#26862=VERTEX_POINT('',#89293);
#26863=VERTEX_POINT('',#89297);
#26864=VERTEX_POINT('',#89299);
#26865=VERTEX_POINT('',#89303);
#26866=VERTEX_POINT('',#89305);
#26867=VERTEX_POINT('',#89313);
#26868=VERTEX_POINT('',#89314);
#26869=VERTEX_POINT('',#89316);
#26870=VERTEX_POINT('',#89318);
#26871=VERTEX_POINT('',#89322);
#26872=VERTEX_POINT('',#89324);
#26873=VERTEX_POINT('',#89328);
#26874=VERTEX_POINT('',#89330);
#26875=VERTEX_POINT('',#89338);
#26876=VERTEX_POINT('',#89339);
#26877=VERTEX_POINT('',#89341);
#26878=VERTEX_POINT('',#89343);
#26879=VERTEX_POINT('',#89347);
#26880=VERTEX_POINT('',#89349);
#26881=VERTEX_POINT('',#89353);
#26882=VERTEX_POINT('',#89355);
#26883=VERTEX_POINT('',#89363);
#26884=VERTEX_POINT('',#89364);
#26885=VERTEX_POINT('',#89366);
#26886=VERTEX_POINT('',#89368);
#26887=VERTEX_POINT('',#89372);
#26888=VERTEX_POINT('',#89374);
#26889=VERTEX_POINT('',#89378);
#26890=VERTEX_POINT('',#89380);
#26891=VERTEX_POINT('',#89388);
#26892=VERTEX_POINT('',#89389);
#26893=VERTEX_POINT('',#89391);
#26894=VERTEX_POINT('',#89393);
#26895=VERTEX_POINT('',#89397);
#26896=VERTEX_POINT('',#89399);
#26897=VERTEX_POINT('',#89403);
#26898=VERTEX_POINT('',#89405);
#26899=VERTEX_POINT('',#89413);
#26900=VERTEX_POINT('',#89414);
#26901=VERTEX_POINT('',#89416);
#26902=VERTEX_POINT('',#89418);
#26903=VERTEX_POINT('',#89422);
#26904=VERTEX_POINT('',#89424);
#26905=VERTEX_POINT('',#89428);
#26906=VERTEX_POINT('',#89430);
#26907=VERTEX_POINT('',#89438);
#26908=VERTEX_POINT('',#89439);
#26909=VERTEX_POINT('',#89441);
#26910=VERTEX_POINT('',#89443);
#26911=VERTEX_POINT('',#89447);
#26912=VERTEX_POINT('',#89449);
#26913=VERTEX_POINT('',#89453);
#26914=VERTEX_POINT('',#89455);
#26915=VERTEX_POINT('',#89463);
#26916=VERTEX_POINT('',#89464);
#26917=VERTEX_POINT('',#89466);
#26918=VERTEX_POINT('',#89468);
#26919=VERTEX_POINT('',#89472);
#26920=VERTEX_POINT('',#89474);
#26921=VERTEX_POINT('',#89478);
#26922=VERTEX_POINT('',#89480);
#26923=VERTEX_POINT('',#89488);
#26924=VERTEX_POINT('',#89489);
#26925=VERTEX_POINT('',#89491);
#26926=VERTEX_POINT('',#89493);
#26927=VERTEX_POINT('',#89497);
#26928=VERTEX_POINT('',#89499);
#26929=VERTEX_POINT('',#89503);
#26930=VERTEX_POINT('',#89505);
#26931=VERTEX_POINT('',#89513);
#26932=VERTEX_POINT('',#89514);
#26933=VERTEX_POINT('',#89516);
#26934=VERTEX_POINT('',#89518);
#26935=VERTEX_POINT('',#89522);
#26936=VERTEX_POINT('',#89524);
#26937=VERTEX_POINT('',#89528);
#26938=VERTEX_POINT('',#89530);
#26939=VERTEX_POINT('',#89538);
#26940=VERTEX_POINT('',#89539);
#26941=VERTEX_POINT('',#89541);
#26942=VERTEX_POINT('',#89543);
#26943=VERTEX_POINT('',#89547);
#26944=VERTEX_POINT('',#89549);
#26945=VERTEX_POINT('',#89553);
#26946=VERTEX_POINT('',#89555);
#26947=VERTEX_POINT('',#89563);
#26948=VERTEX_POINT('',#89564);
#26949=VERTEX_POINT('',#89566);
#26950=VERTEX_POINT('',#89568);
#26951=VERTEX_POINT('',#89572);
#26952=VERTEX_POINT('',#89574);
#26953=VERTEX_POINT('',#89578);
#26954=VERTEX_POINT('',#89580);
#26955=VERTEX_POINT('',#89588);
#26956=VERTEX_POINT('',#89589);
#26957=VERTEX_POINT('',#89591);
#26958=VERTEX_POINT('',#89593);
#26959=VERTEX_POINT('',#89597);
#26960=VERTEX_POINT('',#89599);
#26961=VERTEX_POINT('',#89603);
#26962=VERTEX_POINT('',#89605);
#26963=VERTEX_POINT('',#89613);
#26964=VERTEX_POINT('',#89614);
#26965=VERTEX_POINT('',#89616);
#26966=VERTEX_POINT('',#89618);
#26967=VERTEX_POINT('',#89622);
#26968=VERTEX_POINT('',#89624);
#26969=VERTEX_POINT('',#89628);
#26970=VERTEX_POINT('',#89630);
#26971=VERTEX_POINT('',#89638);
#26972=VERTEX_POINT('',#89639);
#26973=VERTEX_POINT('',#89641);
#26974=VERTEX_POINT('',#89643);
#26975=VERTEX_POINT('',#89647);
#26976=VERTEX_POINT('',#89649);
#26977=VERTEX_POINT('',#89653);
#26978=VERTEX_POINT('',#89655);
#26979=VERTEX_POINT('',#89663);
#26980=VERTEX_POINT('',#89664);
#26981=VERTEX_POINT('',#89666);
#26982=VERTEX_POINT('',#89668);
#26983=VERTEX_POINT('',#89672);
#26984=VERTEX_POINT('',#89674);
#26985=VERTEX_POINT('',#89678);
#26986=VERTEX_POINT('',#89680);
#26987=VERTEX_POINT('',#89688);
#26988=VERTEX_POINT('',#89689);
#26989=VERTEX_POINT('',#89691);
#26990=VERTEX_POINT('',#89693);
#26991=VERTEX_POINT('',#89697);
#26992=VERTEX_POINT('',#89699);
#26993=VERTEX_POINT('',#89703);
#26994=VERTEX_POINT('',#89705);
#26995=VERTEX_POINT('',#89713);
#26996=VERTEX_POINT('',#89714);
#26997=VERTEX_POINT('',#89716);
#26998=VERTEX_POINT('',#89718);
#26999=VERTEX_POINT('',#89722);
#27000=VERTEX_POINT('',#89724);
#27001=VERTEX_POINT('',#89728);
#27002=VERTEX_POINT('',#89730);
#27003=VERTEX_POINT('',#89738);
#27004=VERTEX_POINT('',#89739);
#27005=VERTEX_POINT('',#89741);
#27006=VERTEX_POINT('',#89743);
#27007=VERTEX_POINT('',#89747);
#27008=VERTEX_POINT('',#89749);
#27009=VERTEX_POINT('',#89753);
#27010=VERTEX_POINT('',#89755);
#27011=VERTEX_POINT('',#89763);
#27012=VERTEX_POINT('',#89764);
#27013=VERTEX_POINT('',#89766);
#27014=VERTEX_POINT('',#89768);
#27015=VERTEX_POINT('',#89772);
#27016=VERTEX_POINT('',#89774);
#27017=VERTEX_POINT('',#89778);
#27018=VERTEX_POINT('',#89780);
#27019=VERTEX_POINT('',#89788);
#27020=VERTEX_POINT('',#89789);
#27021=VERTEX_POINT('',#89791);
#27022=VERTEX_POINT('',#89793);
#27023=VERTEX_POINT('',#89797);
#27024=VERTEX_POINT('',#89799);
#27025=VERTEX_POINT('',#89803);
#27026=VERTEX_POINT('',#89805);
#27027=VERTEX_POINT('',#89813);
#27028=VERTEX_POINT('',#89814);
#27029=VERTEX_POINT('',#89816);
#27030=VERTEX_POINT('',#89818);
#27031=VERTEX_POINT('',#89822);
#27032=VERTEX_POINT('',#89824);
#27033=VERTEX_POINT('',#89828);
#27034=VERTEX_POINT('',#89830);
#27035=VERTEX_POINT('',#89838);
#27036=VERTEX_POINT('',#89839);
#27037=VERTEX_POINT('',#89841);
#27038=VERTEX_POINT('',#89843);
#27039=VERTEX_POINT('',#89847);
#27040=VERTEX_POINT('',#89849);
#27041=VERTEX_POINT('',#89853);
#27042=VERTEX_POINT('',#89855);
#27043=VERTEX_POINT('',#89863);
#27044=VERTEX_POINT('',#89864);
#27045=VERTEX_POINT('',#89866);
#27046=VERTEX_POINT('',#89868);
#27047=VERTEX_POINT('',#89872);
#27048=VERTEX_POINT('',#89874);
#27049=VERTEX_POINT('',#89878);
#27050=VERTEX_POINT('',#89880);
#27051=VERTEX_POINT('',#89888);
#27052=VERTEX_POINT('',#89889);
#27053=VERTEX_POINT('',#89891);
#27054=VERTEX_POINT('',#89893);
#27055=VERTEX_POINT('',#89897);
#27056=VERTEX_POINT('',#89899);
#27057=VERTEX_POINT('',#89903);
#27058=VERTEX_POINT('',#89905);
#27059=VERTEX_POINT('',#89913);
#27060=VERTEX_POINT('',#89914);
#27061=VERTEX_POINT('',#89916);
#27062=VERTEX_POINT('',#89918);
#27063=VERTEX_POINT('',#89922);
#27064=VERTEX_POINT('',#89924);
#27065=VERTEX_POINT('',#89928);
#27066=VERTEX_POINT('',#89930);
#27067=VERTEX_POINT('',#89938);
#27068=VERTEX_POINT('',#89939);
#27069=VERTEX_POINT('',#89941);
#27070=VERTEX_POINT('',#89943);
#27071=VERTEX_POINT('',#89947);
#27072=VERTEX_POINT('',#89949);
#27073=VERTEX_POINT('',#89953);
#27074=VERTEX_POINT('',#89955);
#27075=VERTEX_POINT('',#89963);
#27076=VERTEX_POINT('',#89964);
#27077=VERTEX_POINT('',#89966);
#27078=VERTEX_POINT('',#89968);
#27079=VERTEX_POINT('',#89972);
#27080=VERTEX_POINT('',#89974);
#27081=VERTEX_POINT('',#89978);
#27082=VERTEX_POINT('',#89980);
#27083=VERTEX_POINT('',#89988);
#27084=VERTEX_POINT('',#89989);
#27085=VERTEX_POINT('',#89991);
#27086=VERTEX_POINT('',#89993);
#27087=VERTEX_POINT('',#89997);
#27088=VERTEX_POINT('',#89999);
#27089=VERTEX_POINT('',#90003);
#27090=VERTEX_POINT('',#90005);
#27091=VERTEX_POINT('',#90013);
#27092=VERTEX_POINT('',#90014);
#27093=VERTEX_POINT('',#90016);
#27094=VERTEX_POINT('',#90018);
#27095=VERTEX_POINT('',#90022);
#27096=VERTEX_POINT('',#90024);
#27097=VERTEX_POINT('',#90028);
#27098=VERTEX_POINT('',#90030);
#27099=VERTEX_POINT('',#90038);
#27100=VERTEX_POINT('',#90039);
#27101=VERTEX_POINT('',#90041);
#27102=VERTEX_POINT('',#90043);
#27103=VERTEX_POINT('',#90047);
#27104=VERTEX_POINT('',#90049);
#27105=VERTEX_POINT('',#90053);
#27106=VERTEX_POINT('',#90055);
#27107=VERTEX_POINT('',#90063);
#27108=VERTEX_POINT('',#90064);
#27109=VERTEX_POINT('',#90066);
#27110=VERTEX_POINT('',#90068);
#27111=VERTEX_POINT('',#90072);
#27112=VERTEX_POINT('',#90074);
#27113=VERTEX_POINT('',#90078);
#27114=VERTEX_POINT('',#90080);
#27115=VERTEX_POINT('',#90088);
#27116=VERTEX_POINT('',#90089);
#27117=VERTEX_POINT('',#90091);
#27118=VERTEX_POINT('',#90093);
#27119=VERTEX_POINT('',#90097);
#27120=VERTEX_POINT('',#90099);
#27121=VERTEX_POINT('',#90103);
#27122=VERTEX_POINT('',#90105);
#27123=VERTEX_POINT('',#90113);
#27124=VERTEX_POINT('',#90114);
#27125=VERTEX_POINT('',#90116);
#27126=VERTEX_POINT('',#90118);
#27127=VERTEX_POINT('',#90122);
#27128=VERTEX_POINT('',#90124);
#27129=VERTEX_POINT('',#90128);
#27130=VERTEX_POINT('',#90130);
#27131=VERTEX_POINT('',#90138);
#27132=VERTEX_POINT('',#90139);
#27133=VERTEX_POINT('',#90141);
#27134=VERTEX_POINT('',#90143);
#27135=VERTEX_POINT('',#90147);
#27136=VERTEX_POINT('',#90149);
#27137=VERTEX_POINT('',#90153);
#27138=VERTEX_POINT('',#90155);
#27139=VERTEX_POINT('',#90163);
#27140=VERTEX_POINT('',#90164);
#27141=VERTEX_POINT('',#90166);
#27142=VERTEX_POINT('',#90168);
#27143=VERTEX_POINT('',#90172);
#27144=VERTEX_POINT('',#90174);
#27145=VERTEX_POINT('',#90178);
#27146=VERTEX_POINT('',#90180);
#27147=VERTEX_POINT('',#90188);
#27148=VERTEX_POINT('',#90189);
#27149=VERTEX_POINT('',#90191);
#27150=VERTEX_POINT('',#90193);
#27151=VERTEX_POINT('',#90197);
#27152=VERTEX_POINT('',#90199);
#27153=VERTEX_POINT('',#90203);
#27154=VERTEX_POINT('',#90205);
#27155=VERTEX_POINT('',#90213);
#27156=VERTEX_POINT('',#90214);
#27157=VERTEX_POINT('',#90216);
#27158=VERTEX_POINT('',#90218);
#27159=VERTEX_POINT('',#90222);
#27160=VERTEX_POINT('',#90224);
#27161=VERTEX_POINT('',#90228);
#27162=VERTEX_POINT('',#90230);
#27163=VERTEX_POINT('',#90238);
#27164=VERTEX_POINT('',#90239);
#27165=VERTEX_POINT('',#90241);
#27166=VERTEX_POINT('',#90243);
#27167=VERTEX_POINT('',#90247);
#27168=VERTEX_POINT('',#90249);
#27169=VERTEX_POINT('',#90253);
#27170=VERTEX_POINT('',#90255);
#27171=VERTEX_POINT('',#90263);
#27172=VERTEX_POINT('',#90264);
#27173=VERTEX_POINT('',#90266);
#27174=VERTEX_POINT('',#90268);
#27175=VERTEX_POINT('',#90272);
#27176=VERTEX_POINT('',#90274);
#27177=VERTEX_POINT('',#90278);
#27178=VERTEX_POINT('',#90280);
#27179=VERTEX_POINT('',#90288);
#27180=VERTEX_POINT('',#90289);
#27181=VERTEX_POINT('',#90291);
#27182=VERTEX_POINT('',#90293);
#27183=VERTEX_POINT('',#90297);
#27184=VERTEX_POINT('',#90299);
#27185=VERTEX_POINT('',#90303);
#27186=VERTEX_POINT('',#90305);
#27187=VERTEX_POINT('',#90313);
#27188=VERTEX_POINT('',#90314);
#27189=VERTEX_POINT('',#90316);
#27190=VERTEX_POINT('',#90318);
#27191=VERTEX_POINT('',#90322);
#27192=VERTEX_POINT('',#90324);
#27193=VERTEX_POINT('',#90328);
#27194=VERTEX_POINT('',#90330);
#27195=VERTEX_POINT('',#90338);
#27196=VERTEX_POINT('',#90339);
#27197=VERTEX_POINT('',#90341);
#27198=VERTEX_POINT('',#90343);
#27199=VERTEX_POINT('',#90347);
#27200=VERTEX_POINT('',#90349);
#27201=VERTEX_POINT('',#90353);
#27202=VERTEX_POINT('',#90355);
#27203=VERTEX_POINT('',#90363);
#27204=VERTEX_POINT('',#90364);
#27205=VERTEX_POINT('',#90366);
#27206=VERTEX_POINT('',#90368);
#27207=VERTEX_POINT('',#90372);
#27208=VERTEX_POINT('',#90374);
#27209=VERTEX_POINT('',#90378);
#27210=VERTEX_POINT('',#90380);
#27211=VERTEX_POINT('',#90388);
#27212=VERTEX_POINT('',#90389);
#27213=VERTEX_POINT('',#90391);
#27214=VERTEX_POINT('',#90393);
#27215=VERTEX_POINT('',#90397);
#27216=VERTEX_POINT('',#90399);
#27217=VERTEX_POINT('',#90403);
#27218=VERTEX_POINT('',#90405);
#27219=VERTEX_POINT('',#90413);
#27220=VERTEX_POINT('',#90414);
#27221=VERTEX_POINT('',#90416);
#27222=VERTEX_POINT('',#90418);
#27223=VERTEX_POINT('',#90422);
#27224=VERTEX_POINT('',#90424);
#27225=VERTEX_POINT('',#90428);
#27226=VERTEX_POINT('',#90430);
#27227=VERTEX_POINT('',#90438);
#27228=VERTEX_POINT('',#90439);
#27229=VERTEX_POINT('',#90441);
#27230=VERTEX_POINT('',#90443);
#27231=VERTEX_POINT('',#90447);
#27232=VERTEX_POINT('',#90449);
#27233=VERTEX_POINT('',#90453);
#27234=VERTEX_POINT('',#90455);
#27235=VERTEX_POINT('',#90463);
#27236=VERTEX_POINT('',#90464);
#27237=VERTEX_POINT('',#90466);
#27238=VERTEX_POINT('',#90468);
#27239=VERTEX_POINT('',#90472);
#27240=VERTEX_POINT('',#90474);
#27241=VERTEX_POINT('',#90478);
#27242=VERTEX_POINT('',#90480);
#27243=VERTEX_POINT('',#90488);
#27244=VERTEX_POINT('',#90489);
#27245=VERTEX_POINT('',#90491);
#27246=VERTEX_POINT('',#90493);
#27247=VERTEX_POINT('',#90497);
#27248=VERTEX_POINT('',#90499);
#27249=VERTEX_POINT('',#90503);
#27250=VERTEX_POINT('',#90505);
#27251=VERTEX_POINT('',#90513);
#27252=VERTEX_POINT('',#90514);
#27253=VERTEX_POINT('',#90516);
#27254=VERTEX_POINT('',#90518);
#27255=VERTEX_POINT('',#90522);
#27256=VERTEX_POINT('',#90524);
#27257=VERTEX_POINT('',#90528);
#27258=VERTEX_POINT('',#90530);
#27259=VERTEX_POINT('',#90538);
#27260=VERTEX_POINT('',#90539);
#27261=VERTEX_POINT('',#90541);
#27262=VERTEX_POINT('',#90543);
#27263=VERTEX_POINT('',#90547);
#27264=VERTEX_POINT('',#90549);
#27265=VERTEX_POINT('',#90553);
#27266=VERTEX_POINT('',#90555);
#27267=VERTEX_POINT('',#90563);
#27268=VERTEX_POINT('',#90564);
#27269=VERTEX_POINT('',#90566);
#27270=VERTEX_POINT('',#90568);
#27271=VERTEX_POINT('',#90572);
#27272=VERTEX_POINT('',#90574);
#27273=VERTEX_POINT('',#90578);
#27274=VERTEX_POINT('',#90580);
#27275=VERTEX_POINT('',#90588);
#27276=VERTEX_POINT('',#90589);
#27277=VERTEX_POINT('',#90591);
#27278=VERTEX_POINT('',#90593);
#27279=VERTEX_POINT('',#90597);
#27280=VERTEX_POINT('',#90599);
#27281=VERTEX_POINT('',#90603);
#27282=VERTEX_POINT('',#90605);
#27283=VERTEX_POINT('',#90613);
#27284=VERTEX_POINT('',#90614);
#27285=VERTEX_POINT('',#90616);
#27286=VERTEX_POINT('',#90618);
#27287=VERTEX_POINT('',#90622);
#27288=VERTEX_POINT('',#90624);
#27289=VERTEX_POINT('',#90628);
#27290=VERTEX_POINT('',#90630);
#27291=VERTEX_POINT('',#90638);
#27292=VERTEX_POINT('',#90639);
#27293=VERTEX_POINT('',#90641);
#27294=VERTEX_POINT('',#90643);
#27295=VERTEX_POINT('',#90647);
#27296=VERTEX_POINT('',#90649);
#27297=VERTEX_POINT('',#90653);
#27298=VERTEX_POINT('',#90655);
#27299=VERTEX_POINT('',#90663);
#27300=VERTEX_POINT('',#90664);
#27301=VERTEX_POINT('',#90666);
#27302=VERTEX_POINT('',#90668);
#27303=VERTEX_POINT('',#90672);
#27304=VERTEX_POINT('',#90674);
#27305=VERTEX_POINT('',#90678);
#27306=VERTEX_POINT('',#90680);
#27307=VERTEX_POINT('',#90688);
#27308=VERTEX_POINT('',#90689);
#27309=VERTEX_POINT('',#90691);
#27310=VERTEX_POINT('',#90693);
#27311=VERTEX_POINT('',#90697);
#27312=VERTEX_POINT('',#90699);
#27313=VERTEX_POINT('',#90703);
#27314=VERTEX_POINT('',#90705);
#27315=VERTEX_POINT('',#90713);
#27316=VERTEX_POINT('',#90714);
#27317=VERTEX_POINT('',#90716);
#27318=VERTEX_POINT('',#90718);
#27319=VERTEX_POINT('',#90722);
#27320=VERTEX_POINT('',#90724);
#27321=VERTEX_POINT('',#90728);
#27322=VERTEX_POINT('',#90730);
#27323=VERTEX_POINT('',#90738);
#27324=VERTEX_POINT('',#90739);
#27325=VERTEX_POINT('',#90741);
#27326=VERTEX_POINT('',#90743);
#27327=VERTEX_POINT('',#90747);
#27328=VERTEX_POINT('',#90749);
#27329=VERTEX_POINT('',#90753);
#27330=VERTEX_POINT('',#90755);
#27331=VERTEX_POINT('',#90763);
#27332=VERTEX_POINT('',#90764);
#27333=VERTEX_POINT('',#90766);
#27334=VERTEX_POINT('',#90768);
#27335=VERTEX_POINT('',#90772);
#27336=VERTEX_POINT('',#90774);
#27337=VERTEX_POINT('',#90778);
#27338=VERTEX_POINT('',#90780);
#27339=VERTEX_POINT('',#90788);
#27340=VERTEX_POINT('',#90789);
#27341=VERTEX_POINT('',#90791);
#27342=VERTEX_POINT('',#90793);
#27343=VERTEX_POINT('',#90797);
#27344=VERTEX_POINT('',#90799);
#27345=VERTEX_POINT('',#90803);
#27346=VERTEX_POINT('',#90805);
#27347=VERTEX_POINT('',#90813);
#27348=VERTEX_POINT('',#90814);
#27349=VERTEX_POINT('',#90816);
#27350=VERTEX_POINT('',#90818);
#27351=VERTEX_POINT('',#90822);
#27352=VERTEX_POINT('',#90824);
#27353=VERTEX_POINT('',#90828);
#27354=VERTEX_POINT('',#90830);
#27355=VERTEX_POINT('',#90838);
#27356=VERTEX_POINT('',#90839);
#27357=VERTEX_POINT('',#90841);
#27358=VERTEX_POINT('',#90843);
#27359=VERTEX_POINT('',#90847);
#27360=VERTEX_POINT('',#90849);
#27361=VERTEX_POINT('',#90853);
#27362=VERTEX_POINT('',#90855);
#27363=VERTEX_POINT('',#90863);
#27364=VERTEX_POINT('',#90864);
#27365=VERTEX_POINT('',#90866);
#27366=VERTEX_POINT('',#90868);
#27367=VERTEX_POINT('',#90872);
#27368=VERTEX_POINT('',#90874);
#27369=VERTEX_POINT('',#90878);
#27370=VERTEX_POINT('',#90880);
#27371=VERTEX_POINT('',#90888);
#27372=VERTEX_POINT('',#90889);
#27373=VERTEX_POINT('',#90891);
#27374=VERTEX_POINT('',#90893);
#27375=VERTEX_POINT('',#90897);
#27376=VERTEX_POINT('',#90899);
#27377=VERTEX_POINT('',#90903);
#27378=VERTEX_POINT('',#90905);
#27379=VERTEX_POINT('',#90913);
#27380=VERTEX_POINT('',#90914);
#27381=VERTEX_POINT('',#90916);
#27382=VERTEX_POINT('',#90918);
#27383=VERTEX_POINT('',#90922);
#27384=VERTEX_POINT('',#90924);
#27385=VERTEX_POINT('',#90928);
#27386=VERTEX_POINT('',#90930);
#27387=VERTEX_POINT('',#90938);
#27388=VERTEX_POINT('',#90939);
#27389=VERTEX_POINT('',#90941);
#27390=VERTEX_POINT('',#90943);
#27391=VERTEX_POINT('',#90947);
#27392=VERTEX_POINT('',#90949);
#27393=VERTEX_POINT('',#90953);
#27394=VERTEX_POINT('',#90955);
#27395=VERTEX_POINT('',#90963);
#27396=VERTEX_POINT('',#90964);
#27397=VERTEX_POINT('',#90966);
#27398=VERTEX_POINT('',#90968);
#27399=VERTEX_POINT('',#90972);
#27400=VERTEX_POINT('',#90974);
#27401=VERTEX_POINT('',#90978);
#27402=VERTEX_POINT('',#90980);
#27403=VERTEX_POINT('',#90988);
#27404=VERTEX_POINT('',#90989);
#27405=VERTEX_POINT('',#90991);
#27406=VERTEX_POINT('',#90993);
#27407=VERTEX_POINT('',#90997);
#27408=VERTEX_POINT('',#90999);
#27409=VERTEX_POINT('',#91003);
#27410=VERTEX_POINT('',#91005);
#27411=VERTEX_POINT('',#91013);
#27412=VERTEX_POINT('',#91014);
#27413=VERTEX_POINT('',#91016);
#27414=VERTEX_POINT('',#91018);
#27415=VERTEX_POINT('',#91022);
#27416=VERTEX_POINT('',#91024);
#27417=VERTEX_POINT('',#91028);
#27418=VERTEX_POINT('',#91030);
#27419=VERTEX_POINT('',#91038);
#27420=VERTEX_POINT('',#91039);
#27421=VERTEX_POINT('',#91041);
#27422=VERTEX_POINT('',#91043);
#27423=VERTEX_POINT('',#91047);
#27424=VERTEX_POINT('',#91049);
#27425=VERTEX_POINT('',#91053);
#27426=VERTEX_POINT('',#91055);
#27427=VERTEX_POINT('',#91063);
#27428=VERTEX_POINT('',#91064);
#27429=VERTEX_POINT('',#91066);
#27430=VERTEX_POINT('',#91068);
#27431=VERTEX_POINT('',#91072);
#27432=VERTEX_POINT('',#91074);
#27433=VERTEX_POINT('',#91078);
#27434=VERTEX_POINT('',#91080);
#27435=VERTEX_POINT('',#91088);
#27436=VERTEX_POINT('',#91089);
#27437=VERTEX_POINT('',#91091);
#27438=VERTEX_POINT('',#91093);
#27439=VERTEX_POINT('',#91097);
#27440=VERTEX_POINT('',#91099);
#27441=VERTEX_POINT('',#91103);
#27442=VERTEX_POINT('',#91105);
#27443=VERTEX_POINT('',#91113);
#27444=VERTEX_POINT('',#91114);
#27445=VERTEX_POINT('',#91116);
#27446=VERTEX_POINT('',#91118);
#27447=VERTEX_POINT('',#91122);
#27448=VERTEX_POINT('',#91124);
#27449=VERTEX_POINT('',#91128);
#27450=VERTEX_POINT('',#91130);
#27451=VERTEX_POINT('',#91138);
#27452=VERTEX_POINT('',#91139);
#27453=VERTEX_POINT('',#91141);
#27454=VERTEX_POINT('',#91143);
#27455=VERTEX_POINT('',#91147);
#27456=VERTEX_POINT('',#91149);
#27457=VERTEX_POINT('',#91153);
#27458=VERTEX_POINT('',#91155);
#27459=VERTEX_POINT('',#91163);
#27460=VERTEX_POINT('',#91164);
#27461=VERTEX_POINT('',#91166);
#27462=VERTEX_POINT('',#91168);
#27463=VERTEX_POINT('',#91172);
#27464=VERTEX_POINT('',#91174);
#27465=VERTEX_POINT('',#91178);
#27466=VERTEX_POINT('',#91180);
#27467=VERTEX_POINT('',#91188);
#27468=VERTEX_POINT('',#91189);
#27469=VERTEX_POINT('',#91191);
#27470=VERTEX_POINT('',#91193);
#27471=VERTEX_POINT('',#91197);
#27472=VERTEX_POINT('',#91199);
#27473=VERTEX_POINT('',#91203);
#27474=VERTEX_POINT('',#91205);
#27475=VERTEX_POINT('',#91213);
#27476=VERTEX_POINT('',#91214);
#27477=VERTEX_POINT('',#91216);
#27478=VERTEX_POINT('',#91218);
#27479=VERTEX_POINT('',#91222);
#27480=VERTEX_POINT('',#91224);
#27481=VERTEX_POINT('',#91228);
#27482=VERTEX_POINT('',#91230);
#27483=VERTEX_POINT('',#91238);
#27484=VERTEX_POINT('',#91239);
#27485=VERTEX_POINT('',#91241);
#27486=VERTEX_POINT('',#91243);
#27487=VERTEX_POINT('',#91247);
#27488=VERTEX_POINT('',#91249);
#27489=VERTEX_POINT('',#91253);
#27490=VERTEX_POINT('',#91255);
#27491=VERTEX_POINT('',#91263);
#27492=VERTEX_POINT('',#91264);
#27493=VERTEX_POINT('',#91266);
#27494=VERTEX_POINT('',#91268);
#27495=VERTEX_POINT('',#91272);
#27496=VERTEX_POINT('',#91274);
#27497=VERTEX_POINT('',#91278);
#27498=VERTEX_POINT('',#91280);
#27499=VERTEX_POINT('',#91288);
#27500=VERTEX_POINT('',#91289);
#27501=VERTEX_POINT('',#91291);
#27502=VERTEX_POINT('',#91293);
#27503=VERTEX_POINT('',#91297);
#27504=VERTEX_POINT('',#91299);
#27505=VERTEX_POINT('',#91303);
#27506=VERTEX_POINT('',#91305);
#27507=VERTEX_POINT('',#91313);
#27508=VERTEX_POINT('',#91314);
#27509=VERTEX_POINT('',#91316);
#27510=VERTEX_POINT('',#91318);
#27511=VERTEX_POINT('',#91322);
#27512=VERTEX_POINT('',#91324);
#27513=VERTEX_POINT('',#91328);
#27514=VERTEX_POINT('',#91330);
#27515=VERTEX_POINT('',#91338);
#27516=VERTEX_POINT('',#91339);
#27517=VERTEX_POINT('',#91341);
#27518=VERTEX_POINT('',#91343);
#27519=VERTEX_POINT('',#91347);
#27520=VERTEX_POINT('',#91349);
#27521=VERTEX_POINT('',#91353);
#27522=VERTEX_POINT('',#91355);
#27523=VERTEX_POINT('',#91363);
#27524=VERTEX_POINT('',#91364);
#27525=VERTEX_POINT('',#91366);
#27526=VERTEX_POINT('',#91368);
#27527=VERTEX_POINT('',#91372);
#27528=VERTEX_POINT('',#91374);
#27529=VERTEX_POINT('',#91378);
#27530=VERTEX_POINT('',#91380);
#27531=VERTEX_POINT('',#91388);
#27532=VERTEX_POINT('',#91389);
#27533=VERTEX_POINT('',#91391);
#27534=VERTEX_POINT('',#91393);
#27535=VERTEX_POINT('',#91397);
#27536=VERTEX_POINT('',#91399);
#27537=VERTEX_POINT('',#91403);
#27538=VERTEX_POINT('',#91405);
#27539=VERTEX_POINT('',#91413);
#27540=VERTEX_POINT('',#91414);
#27541=VERTEX_POINT('',#91416);
#27542=VERTEX_POINT('',#91418);
#27543=VERTEX_POINT('',#91422);
#27544=VERTEX_POINT('',#91424);
#27545=VERTEX_POINT('',#91428);
#27546=VERTEX_POINT('',#91430);
#27547=VERTEX_POINT('',#91438);
#27548=VERTEX_POINT('',#91439);
#27549=VERTEX_POINT('',#91441);
#27550=VERTEX_POINT('',#91443);
#27551=VERTEX_POINT('',#91447);
#27552=VERTEX_POINT('',#91449);
#27553=VERTEX_POINT('',#91453);
#27554=VERTEX_POINT('',#91455);
#27555=VERTEX_POINT('',#91463);
#27556=VERTEX_POINT('',#91464);
#27557=VERTEX_POINT('',#91466);
#27558=VERTEX_POINT('',#91468);
#27559=VERTEX_POINT('',#91472);
#27560=VERTEX_POINT('',#91474);
#27561=VERTEX_POINT('',#91478);
#27562=VERTEX_POINT('',#91480);
#27563=VERTEX_POINT('',#91488);
#27564=VERTEX_POINT('',#91489);
#27565=VERTEX_POINT('',#91491);
#27566=VERTEX_POINT('',#91493);
#27567=VERTEX_POINT('',#91497);
#27568=VERTEX_POINT('',#91499);
#27569=VERTEX_POINT('',#91503);
#27570=VERTEX_POINT('',#91505);
#27571=VERTEX_POINT('',#91513);
#27572=VERTEX_POINT('',#91514);
#27573=VERTEX_POINT('',#91516);
#27574=VERTEX_POINT('',#91518);
#27575=VERTEX_POINT('',#91522);
#27576=VERTEX_POINT('',#91524);
#27577=VERTEX_POINT('',#91528);
#27578=VERTEX_POINT('',#91530);
#27579=VERTEX_POINT('',#91538);
#27580=VERTEX_POINT('',#91539);
#27581=VERTEX_POINT('',#91541);
#27582=VERTEX_POINT('',#91543);
#27583=VERTEX_POINT('',#91547);
#27584=VERTEX_POINT('',#91549);
#27585=VERTEX_POINT('',#91553);
#27586=VERTEX_POINT('',#91555);
#27587=VERTEX_POINT('',#91563);
#27588=VERTEX_POINT('',#91564);
#27589=VERTEX_POINT('',#91566);
#27590=VERTEX_POINT('',#91568);
#27591=VERTEX_POINT('',#91572);
#27592=VERTEX_POINT('',#91574);
#27593=VERTEX_POINT('',#91578);
#27594=VERTEX_POINT('',#91580);
#27595=VERTEX_POINT('',#91588);
#27596=VERTEX_POINT('',#91589);
#27597=VERTEX_POINT('',#91591);
#27598=VERTEX_POINT('',#91593);
#27599=VERTEX_POINT('',#91597);
#27600=VERTEX_POINT('',#91599);
#27601=VERTEX_POINT('',#91603);
#27602=VERTEX_POINT('',#91605);
#27603=VERTEX_POINT('',#91613);
#27604=VERTEX_POINT('',#91614);
#27605=VERTEX_POINT('',#91616);
#27606=VERTEX_POINT('',#91618);
#27607=VERTEX_POINT('',#91622);
#27608=VERTEX_POINT('',#91624);
#27609=VERTEX_POINT('',#91628);
#27610=VERTEX_POINT('',#91630);
#27611=VERTEX_POINT('',#91638);
#27612=VERTEX_POINT('',#91639);
#27613=VERTEX_POINT('',#91641);
#27614=VERTEX_POINT('',#91643);
#27615=VERTEX_POINT('',#91647);
#27616=VERTEX_POINT('',#91649);
#27617=VERTEX_POINT('',#91653);
#27618=VERTEX_POINT('',#91655);
#27619=VERTEX_POINT('',#91663);
#27620=VERTEX_POINT('',#91664);
#27621=VERTEX_POINT('',#91666);
#27622=VERTEX_POINT('',#91668);
#27623=VERTEX_POINT('',#91672);
#27624=VERTEX_POINT('',#91674);
#27625=VERTEX_POINT('',#91678);
#27626=VERTEX_POINT('',#91680);
#27627=VERTEX_POINT('',#91688);
#27628=VERTEX_POINT('',#91689);
#27629=VERTEX_POINT('',#91691);
#27630=VERTEX_POINT('',#91693);
#27631=VERTEX_POINT('',#91695);
#27632=VERTEX_POINT('',#91697);
#27633=VERTEX_POINT('',#91701);
#27634=VERTEX_POINT('',#91702);
#27635=VERTEX_POINT('',#91704);
#27636=VERTEX_POINT('',#91706);
#27637=VERTEX_POINT('',#91708);
#27638=VERTEX_POINT('',#91710);
#27639=VERTEX_POINT('',#91717);
#27640=VERTEX_POINT('',#91719);
#27641=VERTEX_POINT('',#91721);
#27642=VERTEX_POINT('',#91723);
#27643=VERTEX_POINT('',#91725);
#27644=VERTEX_POINT('',#91727);
#27645=VERTEX_POINT('',#91729);
#27646=VERTEX_POINT('',#91731);
#27647=VERTEX_POINT('',#91733);
#27648=VERTEX_POINT('',#91735);
#27649=VERTEX_POINT('',#91737);
#27650=VERTEX_POINT('',#91739);
#27651=VERTEX_POINT('',#91741);
#27652=VERTEX_POINT('',#91743);
#27653=VERTEX_POINT('',#91745);
#27654=VERTEX_POINT('',#91747);
#27655=VERTEX_POINT('',#91749);
#27656=VERTEX_POINT('',#91751);
#27657=VERTEX_POINT('',#91753);
#27658=VERTEX_POINT('',#91755);
#27659=VERTEX_POINT('',#91759);
#27660=VERTEX_POINT('',#91761);
#27661=VERTEX_POINT('',#91765);
#27662=VERTEX_POINT('',#91767);
#27663=VERTEX_POINT('',#91771);
#27664=VERTEX_POINT('',#91776);
#27665=VERTEX_POINT('',#91778);
#27666=VERTEX_POINT('',#91780);
#27667=VERTEX_POINT('',#91783);
#27668=VERTEX_POINT('',#91785);
#27669=VERTEX_POINT('',#91788);
#27670=VERTEX_POINT('',#91790);
#27671=VERTEX_POINT('',#91793);
#27672=VERTEX_POINT('',#91797);
#27673=VERTEX_POINT('',#91801);
#27674=VERTEX_POINT('',#91803);
#27675=VERTEX_POINT('',#91807);
#27676=VERTEX_POINT('',#91811);
#27677=VERTEX_POINT('',#91812);
#27678=VERTEX_POINT('',#91814);
#27679=VERTEX_POINT('',#91816);
#27680=VERTEX_POINT('',#91819);
#27681=VERTEX_POINT('',#91822);
#27682=VERTEX_POINT('',#91825);
#27683=VERTEX_POINT('',#91829);
#27684=VERTEX_POINT('',#91833);
#27685=VERTEX_POINT('',#91836);
#27686=VERTEX_POINT('',#91838);
#27687=VERTEX_POINT('',#91842);
#27688=VERTEX_POINT('',#91845);
#27689=VERTEX_POINT('',#91847);
#27690=VERTEX_POINT('',#91851);
#27691=VERTEX_POINT('',#91854);
#27692=VERTEX_POINT('',#91856);
#27693=VERTEX_POINT('',#91860);
#27694=VERTEX_POINT('',#91863);
#27695=VERTEX_POINT('',#91865);
#27696=VERTEX_POINT('',#91869);
#27697=VERTEX_POINT('',#91872);
#27698=VERTEX_POINT('',#91874);
#27699=VERTEX_POINT('',#91878);
#27700=VERTEX_POINT('',#91881);
#27701=VERTEX_POINT('',#91883);
#27702=VERTEX_POINT('',#91887);
#27703=VERTEX_POINT('',#91890);
#27704=VERTEX_POINT('',#91894);
#27705=VERTEX_POINT('',#91897);
#27706=VERTEX_POINT('',#91899);
#27707=VERTEX_POINT('',#91901);
#27708=VERTEX_POINT('',#91906);
#27709=VERTEX_POINT('',#91912);
#27710=VERTEX_POINT('',#91918);
#27711=VERTEX_POINT('',#91924);
#27712=VERTEX_POINT('',#91930);
#27713=VERTEX_POINT('',#91936);
#27714=VERTEX_POINT('',#91937);
#27715=VERTEX_POINT('',#91939);
#27716=VERTEX_POINT('',#91941);
#27717=VERTEX_POINT('',#91945);
#27718=VERTEX_POINT('',#91947);
#27719=VERTEX_POINT('',#91951);
#27720=VERTEX_POINT('',#91953);
#27721=VERTEX_POINT('',#91957);
#27722=VERTEX_POINT('',#91958);
#27723=VERTEX_POINT('',#91960);
#27724=VERTEX_POINT('',#91965);
#27725=VERTEX_POINT('',#91967);
#27726=VERTEX_POINT('',#91971);
#27727=VERTEX_POINT('',#91973);
#27728=VERTEX_POINT('',#91977);
#27729=VERTEX_POINT('',#91979);
#27730=VERTEX_POINT('',#91983);
#27731=VERTEX_POINT('',#91990);
#27732=VERTEX_POINT('',#91993);
#27733=VERTEX_POINT('',#91995);
#27734=VERTEX_POINT('',#91997);
#27735=VERTEX_POINT('',#92001);
#27736=VERTEX_POINT('',#92005);
#27737=VERTEX_POINT('',#92009);
#27738=VERTEX_POINT('',#92015);
#27739=VERTEX_POINT('',#92019);
#27740=VERTEX_POINT('',#92020);
#27741=VERTEX_POINT('',#92022);
#27742=VERTEX_POINT('',#92024);
#27743=VERTEX_POINT('',#92028);
#27744=VERTEX_POINT('',#92030);
#27745=VERTEX_POINT('',#92034);
#27746=VERTEX_POINT('',#92036);
#27747=VERTEX_POINT('',#92043);
#27748=VERTEX_POINT('',#92045);
#27749=VERTEX_POINT('',#92049);
#27750=VERTEX_POINT('',#92051);
#27751=VERTEX_POINT('',#92055);
#27752=VERTEX_POINT('',#92057);
#27753=VERTEX_POINT('',#92064);
#27754=VERTEX_POINT('',#92066);
#27755=VERTEX_POINT('',#92070);
#27756=VERTEX_POINT('',#92074);
#27757=VERTEX_POINT('',#92080);
#27758=VERTEX_POINT('',#92084);
#27759=VERTEX_POINT('',#92088);
#27760=VERTEX_POINT('',#92094);
#27761=VERTEX_POINT('',#92095);
#27762=VERTEX_POINT('',#92100);
#30352=EDGE_CURVE('',#24623,#24624,#22944,.T.);
#30353=EDGE_CURVE('',#24623,#24625,#10876,.T.);
#30354=EDGE_CURVE('',#24625,#24626,#22945,.T.);
#30355=EDGE_CURVE('',#24624,#24626,#10877,.T.);
#30356=EDGE_CURVE('',#24627,#24623,#22946,.T.);
#30357=EDGE_CURVE('',#24627,#24628,#10878,.T.);
#30358=EDGE_CURVE('',#24628,#24625,#22947,.T.);
#30359=EDGE_CURVE('',#24629,#24627,#22948,.T.);
#30360=EDGE_CURVE('',#24629,#24630,#10879,.T.);
#30361=EDGE_CURVE('',#24630,#24628,#22949,.T.);
#30362=EDGE_CURVE('',#24631,#24629,#22950,.T.);
#30363=EDGE_CURVE('',#24631,#24632,#10880,.T.);
#30364=EDGE_CURVE('',#24632,#24630,#22951,.T.);
#30365=EDGE_CURVE('',#24633,#24631,#22952,.T.);
#30366=EDGE_CURVE('',#24633,#24634,#10881,.T.);
#30367=EDGE_CURVE('',#24634,#24632,#22953,.T.);
#30368=EDGE_CURVE('',#24635,#24633,#22954,.T.);
#30369=EDGE_CURVE('',#24635,#24636,#10882,.T.);
#30370=EDGE_CURVE('',#24636,#24634,#22955,.T.);
#30371=EDGE_CURVE('',#24637,#24635,#22956,.T.);
#30372=EDGE_CURVE('',#24637,#24638,#10883,.T.);
#30373=EDGE_CURVE('',#24638,#24636,#22957,.T.);
#30374=EDGE_CURVE('',#24624,#24637,#22958,.T.);
#30375=EDGE_CURVE('',#24626,#24638,#22959,.T.);
#30376=EDGE_CURVE('',#24639,#24640,#22960,.T.);
#30377=EDGE_CURVE('',#24639,#24641,#10884,.T.);
#30378=EDGE_CURVE('',#24641,#24642,#22961,.T.);
#30379=EDGE_CURVE('',#24640,#24642,#10885,.T.);
#30380=EDGE_CURVE('',#24643,#24639,#22962,.T.);
#30381=EDGE_CURVE('',#24643,#24644,#10886,.T.);
#30382=EDGE_CURVE('',#24644,#24641,#22963,.T.);
#30383=EDGE_CURVE('',#24645,#24643,#22964,.T.);
#30384=EDGE_CURVE('',#24645,#24646,#10887,.T.);
#30385=EDGE_CURVE('',#24646,#24644,#22965,.T.);
#30386=EDGE_CURVE('',#24647,#24645,#22966,.T.);
#30387=EDGE_CURVE('',#24647,#24648,#10888,.T.);
#30388=EDGE_CURVE('',#24648,#24646,#22967,.T.);
#30389=EDGE_CURVE('',#24649,#24647,#22968,.T.);
#30390=EDGE_CURVE('',#24649,#24650,#10889,.T.);
#30391=EDGE_CURVE('',#24650,#24648,#22969,.T.);
#30392=EDGE_CURVE('',#24651,#24649,#22970,.T.);
#30393=EDGE_CURVE('',#24651,#24652,#10890,.T.);
#30394=EDGE_CURVE('',#24652,#24650,#22971,.T.);
#30395=EDGE_CURVE('',#24653,#24651,#22972,.T.);
#30396=EDGE_CURVE('',#24653,#24654,#10891,.T.);
#30397=EDGE_CURVE('',#24654,#24652,#22973,.T.);
#30398=EDGE_CURVE('',#24655,#24653,#22974,.T.);
#30399=EDGE_CURVE('',#24655,#24656,#10892,.T.);
#30400=EDGE_CURVE('',#24656,#24654,#22975,.T.);
#30401=EDGE_CURVE('',#24657,#24655,#22976,.T.);
#30402=EDGE_CURVE('',#24657,#24658,#10893,.T.);
#30403=EDGE_CURVE('',#24658,#24656,#22977,.T.);
#30404=EDGE_CURVE('',#24659,#24657,#22978,.T.);
#30405=EDGE_CURVE('',#24659,#24660,#10894,.T.);
#30406=EDGE_CURVE('',#24660,#24658,#22979,.T.);
#30407=EDGE_CURVE('',#24661,#24659,#22980,.T.);
#30408=EDGE_CURVE('',#24661,#24662,#10895,.T.);
#30409=EDGE_CURVE('',#24662,#24660,#22981,.T.);
#30410=EDGE_CURVE('',#24640,#24661,#22982,.T.);
#30411=EDGE_CURVE('',#24642,#24662,#22983,.T.);
#30412=EDGE_CURVE('',#24663,#24664,#22984,.T.);
#30413=EDGE_CURVE('',#24663,#24665,#10896,.T.);
#30414=EDGE_CURVE('',#24665,#24666,#22985,.T.);
#30415=EDGE_CURVE('',#24664,#24666,#10897,.T.);
#30416=EDGE_CURVE('',#24667,#24663,#22986,.T.);
#30417=EDGE_CURVE('',#24667,#24668,#10898,.T.);
#30418=EDGE_CURVE('',#24668,#24665,#22987,.T.);
#30419=EDGE_CURVE('',#24669,#24667,#22988,.T.);
#30420=EDGE_CURVE('',#24669,#24670,#10899,.T.);
#30421=EDGE_CURVE('',#24670,#24668,#22989,.T.);
#30422=EDGE_CURVE('',#24671,#24669,#22990,.T.);
#30423=EDGE_CURVE('',#24671,#24672,#10900,.T.);
#30424=EDGE_CURVE('',#24672,#24670,#22991,.T.);
#30425=EDGE_CURVE('',#24673,#24671,#22992,.T.);
#30426=EDGE_CURVE('',#24673,#24674,#10901,.T.);
#30427=EDGE_CURVE('',#24674,#24672,#22993,.T.);
#30428=EDGE_CURVE('',#24675,#24673,#22994,.T.);
#30429=EDGE_CURVE('',#24675,#24676,#10902,.T.);
#30430=EDGE_CURVE('',#24676,#24674,#22995,.T.);
#30431=EDGE_CURVE('',#24677,#24675,#22996,.T.);
#30432=EDGE_CURVE('',#24677,#24678,#10903,.T.);
#30433=EDGE_CURVE('',#24678,#24676,#22997,.T.);
#30434=EDGE_CURVE('',#24664,#24677,#22998,.T.);
#30435=EDGE_CURVE('',#24666,#24678,#22999,.T.);
#30436=EDGE_CURVE('',#24679,#24680,#23000,.T.);
#30437=EDGE_CURVE('',#24679,#24681,#10904,.T.);
#30438=EDGE_CURVE('',#24681,#24682,#23001,.T.);
#30439=EDGE_CURVE('',#24680,#24682,#10905,.T.);
#30440=EDGE_CURVE('',#24683,#24679,#23002,.T.);
#30441=EDGE_CURVE('',#24683,#24684,#10906,.T.);
#30442=EDGE_CURVE('',#24684,#24681,#23003,.T.);
#30443=EDGE_CURVE('',#24685,#24683,#23004,.T.);
#30444=EDGE_CURVE('',#24685,#24686,#10907,.T.);
#30445=EDGE_CURVE('',#24686,#24684,#23005,.T.);
#30446=EDGE_CURVE('',#24687,#24685,#23006,.T.);
#30447=EDGE_CURVE('',#24687,#24688,#10908,.T.);
#30448=EDGE_CURVE('',#24688,#24686,#23007,.T.);
#30449=EDGE_CURVE('',#24689,#24687,#23008,.T.);
#30450=EDGE_CURVE('',#24689,#24690,#10909,.T.);
#30451=EDGE_CURVE('',#24690,#24688,#23009,.T.);
#30452=EDGE_CURVE('',#24691,#24689,#23010,.T.);
#30453=EDGE_CURVE('',#24691,#24692,#10910,.T.);
#30454=EDGE_CURVE('',#24692,#24690,#23011,.T.);
#30455=EDGE_CURVE('',#24693,#24691,#23012,.T.);
#30456=EDGE_CURVE('',#24693,#24694,#10911,.T.);
#30457=EDGE_CURVE('',#24694,#24692,#23013,.T.);
#30458=EDGE_CURVE('',#24695,#24693,#23014,.T.);
#30459=EDGE_CURVE('',#24695,#24696,#10912,.T.);
#30460=EDGE_CURVE('',#24696,#24694,#23015,.T.);
#30461=EDGE_CURVE('',#24697,#24695,#23016,.T.);
#30462=EDGE_CURVE('',#24697,#24698,#10913,.T.);
#30463=EDGE_CURVE('',#24698,#24696,#23017,.T.);
#30464=EDGE_CURVE('',#24699,#24697,#23018,.T.);
#30465=EDGE_CURVE('',#24699,#24700,#10914,.T.);
#30466=EDGE_CURVE('',#24700,#24698,#23019,.T.);
#30467=EDGE_CURVE('',#24701,#24699,#23020,.T.);
#30468=EDGE_CURVE('',#24701,#24702,#10915,.T.);
#30469=EDGE_CURVE('',#24702,#24700,#23021,.T.);
#30470=EDGE_CURVE('',#24703,#24701,#23022,.T.);
#30471=EDGE_CURVE('',#24703,#24704,#10916,.T.);
#30472=EDGE_CURVE('',#24704,#24702,#23023,.T.);
#30473=EDGE_CURVE('',#24705,#24703,#23024,.T.);
#30474=EDGE_CURVE('',#24705,#24706,#10917,.T.);
#30475=EDGE_CURVE('',#24706,#24704,#23025,.T.);
#30476=EDGE_CURVE('',#24707,#24705,#23026,.T.);
#30477=EDGE_CURVE('',#24707,#24708,#10918,.T.);
#30478=EDGE_CURVE('',#24708,#24706,#23027,.T.);
#30479=EDGE_CURVE('',#24709,#24707,#23028,.T.);
#30480=EDGE_CURVE('',#24709,#24710,#10919,.T.);
#30481=EDGE_CURVE('',#24710,#24708,#23029,.T.);
#30482=EDGE_CURVE('',#24711,#24709,#23030,.T.);
#30483=EDGE_CURVE('',#24711,#24712,#10920,.T.);
#30484=EDGE_CURVE('',#24712,#24710,#23031,.T.);
#30485=EDGE_CURVE('',#24713,#24711,#23032,.T.);
#30486=EDGE_CURVE('',#24713,#24714,#10921,.T.);
#30487=EDGE_CURVE('',#24714,#24712,#23033,.T.);
#30488=EDGE_CURVE('',#24715,#24713,#23034,.T.);
#30489=EDGE_CURVE('',#24715,#24716,#10922,.T.);
#30490=EDGE_CURVE('',#24716,#24714,#23035,.T.);
#30491=EDGE_CURVE('',#24717,#24715,#23036,.T.);
#30492=EDGE_CURVE('',#24717,#24718,#10923,.T.);
#30493=EDGE_CURVE('',#24718,#24716,#23037,.T.);
#30494=EDGE_CURVE('',#24719,#24717,#23038,.T.);
#30495=EDGE_CURVE('',#24719,#24720,#10924,.T.);
#30496=EDGE_CURVE('',#24720,#24718,#23039,.T.);
#30497=EDGE_CURVE('',#24721,#24719,#10925,.T.);
#30498=EDGE_CURVE('',#24721,#24722,#10926,.T.);
#30499=EDGE_CURVE('',#24722,#24720,#10927,.T.);
#30500=EDGE_CURVE('',#24680,#24721,#23040,.T.);
#30501=EDGE_CURVE('',#24682,#24722,#23041,.T.);
#30502=EDGE_CURVE('',#24723,#24724,#23042,.T.);
#30503=EDGE_CURVE('',#24723,#24725,#10928,.T.);
#30504=EDGE_CURVE('',#24725,#24726,#23043,.T.);
#30505=EDGE_CURVE('',#24724,#24726,#10929,.T.);
#30506=EDGE_CURVE('',#24727,#24723,#23044,.T.);
#30507=EDGE_CURVE('',#24727,#24728,#10930,.T.);
#30508=EDGE_CURVE('',#24728,#24725,#23045,.T.);
#30509=EDGE_CURVE('',#24729,#24727,#23046,.T.);
#30510=EDGE_CURVE('',#24729,#24730,#10931,.T.);
#30511=EDGE_CURVE('',#24730,#24728,#23047,.T.);
#30512=EDGE_CURVE('',#24731,#24729,#23048,.T.);
#30513=EDGE_CURVE('',#24731,#24732,#10932,.T.);
#30514=EDGE_CURVE('',#24732,#24730,#23049,.T.);
#30515=EDGE_CURVE('',#24733,#24731,#23050,.T.);
#30516=EDGE_CURVE('',#24733,#24734,#10933,.T.);
#30517=EDGE_CURVE('',#24734,#24732,#23051,.T.);
#30518=EDGE_CURVE('',#24735,#24733,#23052,.T.);
#30519=EDGE_CURVE('',#24735,#24736,#10934,.T.);
#30520=EDGE_CURVE('',#24736,#24734,#23053,.T.);
#30521=EDGE_CURVE('',#24737,#24735,#23054,.T.);
#30522=EDGE_CURVE('',#24737,#24738,#10935,.T.);
#30523=EDGE_CURVE('',#24738,#24736,#23055,.T.);
#30524=EDGE_CURVE('',#24724,#24737,#23056,.T.);
#30525=EDGE_CURVE('',#24726,#24738,#23057,.T.);
#30526=EDGE_CURVE('',#24739,#24740,#23058,.T.);
#30527=EDGE_CURVE('',#24739,#24741,#10936,.T.);
#30528=EDGE_CURVE('',#24741,#24742,#23059,.T.);
#30529=EDGE_CURVE('',#24740,#24742,#10937,.T.);
#30530=EDGE_CURVE('',#24743,#24739,#23060,.T.);
#30531=EDGE_CURVE('',#24743,#24744,#10938,.T.);
#30532=EDGE_CURVE('',#24744,#24741,#23061,.T.);
#30533=EDGE_CURVE('',#24745,#24743,#23062,.T.);
#30534=EDGE_CURVE('',#24745,#24746,#10939,.T.);
#30535=EDGE_CURVE('',#24746,#24744,#23063,.T.);
#30536=EDGE_CURVE('',#24747,#24745,#23064,.T.);
#30537=EDGE_CURVE('',#24747,#24748,#10940,.T.);
#30538=EDGE_CURVE('',#24748,#24746,#23065,.T.);
#30539=EDGE_CURVE('',#24749,#24747,#23066,.T.);
#30540=EDGE_CURVE('',#24749,#24750,#10941,.T.);
#30541=EDGE_CURVE('',#24750,#24748,#23067,.T.);
#30542=EDGE_CURVE('',#24751,#24749,#23068,.T.);
#30543=EDGE_CURVE('',#24751,#24752,#10942,.T.);
#30544=EDGE_CURVE('',#24752,#24750,#23069,.T.);
#30545=EDGE_CURVE('',#24753,#24751,#23070,.T.);
#30546=EDGE_CURVE('',#24753,#24754,#10943,.T.);
#30547=EDGE_CURVE('',#24754,#24752,#23071,.T.);
#30548=EDGE_CURVE('',#24755,#24753,#23072,.T.);
#30549=EDGE_CURVE('',#24755,#24756,#10944,.T.);
#30550=EDGE_CURVE('',#24756,#24754,#23073,.T.);
#30551=EDGE_CURVE('',#24757,#24755,#23074,.T.);
#30552=EDGE_CURVE('',#24757,#24758,#10945,.T.);
#30553=EDGE_CURVE('',#24758,#24756,#23075,.T.);
#30554=EDGE_CURVE('',#24759,#24757,#23076,.T.);
#30555=EDGE_CURVE('',#24759,#24760,#10946,.T.);
#30556=EDGE_CURVE('',#24760,#24758,#23077,.T.);
#30557=EDGE_CURVE('',#24761,#24759,#23078,.T.);
#30558=EDGE_CURVE('',#24761,#24762,#10947,.T.);
#30559=EDGE_CURVE('',#24762,#24760,#23079,.T.);
#30560=EDGE_CURVE('',#24740,#24761,#23080,.T.);
#30561=EDGE_CURVE('',#24742,#24762,#23081,.T.);
#30562=EDGE_CURVE('',#24763,#24764,#23082,.T.);
#30563=EDGE_CURVE('',#24763,#24765,#10948,.T.);
#30564=EDGE_CURVE('',#24765,#24766,#23083,.T.);
#30565=EDGE_CURVE('',#24764,#24766,#10949,.T.);
#30566=EDGE_CURVE('',#24767,#24763,#23084,.T.);
#30567=EDGE_CURVE('',#24767,#24768,#10950,.T.);
#30568=EDGE_CURVE('',#24768,#24765,#23085,.T.);
#30569=EDGE_CURVE('',#24769,#24767,#23086,.T.);
#30570=EDGE_CURVE('',#24769,#24770,#10951,.T.);
#30571=EDGE_CURVE('',#24770,#24768,#23087,.T.);
#30572=EDGE_CURVE('',#24771,#24769,#23088,.T.);
#30573=EDGE_CURVE('',#24771,#24772,#10952,.T.);
#30574=EDGE_CURVE('',#24772,#24770,#23089,.T.);
#30575=EDGE_CURVE('',#24773,#24771,#23090,.T.);
#30576=EDGE_CURVE('',#24773,#24774,#10953,.T.);
#30577=EDGE_CURVE('',#24774,#24772,#23091,.T.);
#30578=EDGE_CURVE('',#24775,#24773,#23092,.T.);
#30579=EDGE_CURVE('',#24775,#24776,#10954,.T.);
#30580=EDGE_CURVE('',#24776,#24774,#23093,.T.);
#30581=EDGE_CURVE('',#24777,#24775,#23094,.T.);
#30582=EDGE_CURVE('',#24777,#24778,#10955,.T.);
#30583=EDGE_CURVE('',#24778,#24776,#23095,.T.);
#30584=EDGE_CURVE('',#24764,#24777,#23096,.T.);
#30585=EDGE_CURVE('',#24766,#24778,#23097,.T.);
#30586=EDGE_CURVE('',#24779,#24780,#23098,.T.);
#30587=EDGE_CURVE('',#24779,#24781,#10956,.T.);
#30588=EDGE_CURVE('',#24781,#24782,#23099,.T.);
#30589=EDGE_CURVE('',#24780,#24782,#10957,.T.);
#30590=EDGE_CURVE('',#24783,#24779,#23100,.T.);
#30591=EDGE_CURVE('',#24783,#24784,#10958,.T.);
#30592=EDGE_CURVE('',#24784,#24781,#23101,.T.);
#30593=EDGE_CURVE('',#24785,#24783,#23102,.T.);
#30594=EDGE_CURVE('',#24785,#24786,#10959,.T.);
#30595=EDGE_CURVE('',#24786,#24784,#23103,.T.);
#30596=EDGE_CURVE('',#24787,#24785,#23104,.T.);
#30597=EDGE_CURVE('',#24787,#24788,#10960,.T.);
#30598=EDGE_CURVE('',#24788,#24786,#23105,.T.);
#30599=EDGE_CURVE('',#24789,#24787,#23106,.T.);
#30600=EDGE_CURVE('',#24789,#24790,#10961,.T.);
#30601=EDGE_CURVE('',#24790,#24788,#23107,.T.);
#30602=EDGE_CURVE('',#24791,#24789,#23108,.T.);
#30603=EDGE_CURVE('',#24791,#24792,#10962,.T.);
#30604=EDGE_CURVE('',#24792,#24790,#23109,.T.);
#30605=EDGE_CURVE('',#24793,#24791,#23110,.T.);
#30606=EDGE_CURVE('',#24793,#24794,#10963,.T.);
#30607=EDGE_CURVE('',#24794,#24792,#23111,.T.);
#30608=EDGE_CURVE('',#24795,#24793,#23112,.T.);
#30609=EDGE_CURVE('',#24795,#24796,#10964,.T.);
#30610=EDGE_CURVE('',#24796,#24794,#23113,.T.);
#30611=EDGE_CURVE('',#24780,#24795,#23114,.T.);
#30612=EDGE_CURVE('',#24782,#24796,#23115,.T.);
#30613=EDGE_CURVE('',#24797,#24798,#23116,.T.);
#30614=EDGE_CURVE('',#24797,#24799,#10965,.T.);
#30615=EDGE_CURVE('',#24799,#24800,#23117,.T.);
#30616=EDGE_CURVE('',#24798,#24800,#10966,.T.);
#30617=EDGE_CURVE('',#24801,#24797,#23118,.T.);
#30618=EDGE_CURVE('',#24801,#24802,#10967,.T.);
#30619=EDGE_CURVE('',#24802,#24799,#23119,.T.);
#30620=EDGE_CURVE('',#24803,#24801,#23120,.T.);
#30621=EDGE_CURVE('',#24803,#24804,#10968,.T.);
#30622=EDGE_CURVE('',#24804,#24802,#23121,.T.);
#30623=EDGE_CURVE('',#24805,#24803,#23122,.T.);
#30624=EDGE_CURVE('',#24805,#24806,#10969,.T.);
#30625=EDGE_CURVE('',#24806,#24804,#23123,.T.);
#30626=EDGE_CURVE('',#24807,#24805,#23124,.T.);
#30627=EDGE_CURVE('',#24807,#24808,#10970,.T.);
#30628=EDGE_CURVE('',#24808,#24806,#23125,.T.);
#30629=EDGE_CURVE('',#24809,#24807,#23126,.T.);
#30630=EDGE_CURVE('',#24809,#24810,#10971,.T.);
#30631=EDGE_CURVE('',#24810,#24808,#23127,.T.);
#30632=EDGE_CURVE('',#24811,#24809,#23128,.T.);
#30633=EDGE_CURVE('',#24811,#24812,#10972,.T.);
#30634=EDGE_CURVE('',#24812,#24810,#23129,.T.);
#30635=EDGE_CURVE('',#24813,#24811,#23130,.T.);
#30636=EDGE_CURVE('',#24813,#24814,#10973,.T.);
#30637=EDGE_CURVE('',#24814,#24812,#23131,.T.);
#30638=EDGE_CURVE('',#24815,#24813,#23132,.T.);
#30639=EDGE_CURVE('',#24815,#24816,#10974,.T.);
#30640=EDGE_CURVE('',#24816,#24814,#23133,.T.);
#30641=EDGE_CURVE('',#24817,#24815,#23134,.T.);
#30642=EDGE_CURVE('',#24817,#24818,#10975,.T.);
#30643=EDGE_CURVE('',#24818,#24816,#23135,.T.);
#30644=EDGE_CURVE('',#24819,#24817,#23136,.T.);
#30645=EDGE_CURVE('',#24819,#24820,#10976,.T.);
#30646=EDGE_CURVE('',#24820,#24818,#23137,.T.);
#30647=EDGE_CURVE('',#24821,#24819,#23138,.T.);
#30648=EDGE_CURVE('',#24821,#24822,#10977,.T.);
#30649=EDGE_CURVE('',#24822,#24820,#23139,.T.);
#30650=EDGE_CURVE('',#24823,#24821,#23140,.T.);
#30651=EDGE_CURVE('',#24823,#24824,#10978,.T.);
#30652=EDGE_CURVE('',#24824,#24822,#23141,.T.);
#30653=EDGE_CURVE('',#24825,#24823,#23142,.T.);
#30654=EDGE_CURVE('',#24825,#24826,#10979,.T.);
#30655=EDGE_CURVE('',#24826,#24824,#23143,.T.);
#30656=EDGE_CURVE('',#24827,#24825,#23144,.T.);
#30657=EDGE_CURVE('',#24827,#24828,#10980,.T.);
#30658=EDGE_CURVE('',#24828,#24826,#23145,.T.);
#30659=EDGE_CURVE('',#24798,#24827,#23146,.T.);
#30660=EDGE_CURVE('',#24800,#24828,#23147,.T.);
#30661=EDGE_CURVE('',#24829,#24830,#23148,.T.);
#30662=EDGE_CURVE('',#24829,#24831,#10981,.T.);
#30663=EDGE_CURVE('',#24831,#24832,#23149,.T.);
#30664=EDGE_CURVE('',#24830,#24832,#10982,.T.);
#30665=EDGE_CURVE('',#24833,#24829,#23150,.T.);
#30666=EDGE_CURVE('',#24833,#24834,#10983,.T.);
#30667=EDGE_CURVE('',#24834,#24831,#23151,.T.);
#30668=EDGE_CURVE('',#24835,#24833,#23152,.T.);
#30669=EDGE_CURVE('',#24835,#24836,#10984,.T.);
#30670=EDGE_CURVE('',#24836,#24834,#23153,.T.);
#30671=EDGE_CURVE('',#24837,#24835,#23154,.T.);
#30672=EDGE_CURVE('',#24837,#24838,#10985,.T.);
#30673=EDGE_CURVE('',#24838,#24836,#23155,.T.);
#30674=EDGE_CURVE('',#24839,#24837,#23156,.T.);
#30675=EDGE_CURVE('',#24839,#24840,#10986,.T.);
#30676=EDGE_CURVE('',#24840,#24838,#23157,.T.);
#30677=EDGE_CURVE('',#24841,#24839,#23158,.T.);
#30678=EDGE_CURVE('',#24841,#24842,#10987,.T.);
#30679=EDGE_CURVE('',#24842,#24840,#23159,.T.);
#30680=EDGE_CURVE('',#24843,#24841,#23160,.T.);
#30681=EDGE_CURVE('',#24843,#24844,#10988,.T.);
#30682=EDGE_CURVE('',#24844,#24842,#23161,.T.);
#30683=EDGE_CURVE('',#24830,#24843,#23162,.T.);
#30684=EDGE_CURVE('',#24832,#24844,#23163,.T.);
#30685=EDGE_CURVE('',#24845,#24846,#23164,.T.);
#30686=EDGE_CURVE('',#24845,#24847,#10989,.T.);
#30687=EDGE_CURVE('',#24847,#24848,#23165,.T.);
#30688=EDGE_CURVE('',#24846,#24848,#10990,.T.);
#30689=EDGE_CURVE('',#24849,#24845,#23166,.T.);
#30690=EDGE_CURVE('',#24849,#24850,#10991,.T.);
#30691=EDGE_CURVE('',#24850,#24847,#23167,.T.);
#30692=EDGE_CURVE('',#24851,#24849,#23168,.T.);
#30693=EDGE_CURVE('',#24851,#24852,#10992,.T.);
#30694=EDGE_CURVE('',#24852,#24850,#23169,.T.);
#30695=EDGE_CURVE('',#24853,#24851,#23170,.T.);
#30696=EDGE_CURVE('',#24853,#24854,#10993,.T.);
#30697=EDGE_CURVE('',#24854,#24852,#23171,.T.);
#30698=EDGE_CURVE('',#24855,#24853,#23172,.T.);
#30699=EDGE_CURVE('',#24855,#24856,#10994,.T.);
#30700=EDGE_CURVE('',#24856,#24854,#23173,.T.);
#30701=EDGE_CURVE('',#24857,#24855,#23174,.T.);
#30702=EDGE_CURVE('',#24857,#24858,#10995,.T.);
#30703=EDGE_CURVE('',#24858,#24856,#23175,.T.);
#30704=EDGE_CURVE('',#24859,#24857,#23176,.T.);
#30705=EDGE_CURVE('',#24859,#24860,#10996,.T.);
#30706=EDGE_CURVE('',#24860,#24858,#23177,.T.);
#30707=EDGE_CURVE('',#24861,#24859,#23178,.T.);
#30708=EDGE_CURVE('',#24861,#24862,#10997,.T.);
#30709=EDGE_CURVE('',#24862,#24860,#23179,.T.);
#30710=EDGE_CURVE('',#24863,#24861,#23180,.T.);
#30711=EDGE_CURVE('',#24863,#24864,#10998,.T.);
#30712=EDGE_CURVE('',#24864,#24862,#23181,.T.);
#30713=EDGE_CURVE('',#24865,#24863,#23182,.T.);
#30714=EDGE_CURVE('',#24865,#24866,#10999,.T.);
#30715=EDGE_CURVE('',#24866,#24864,#23183,.T.);
#30716=EDGE_CURVE('',#24867,#24865,#23184,.T.);
#30717=EDGE_CURVE('',#24867,#24868,#11000,.T.);
#30718=EDGE_CURVE('',#24868,#24866,#23185,.T.);
#30719=EDGE_CURVE('',#24846,#24867,#23186,.T.);
#30720=EDGE_CURVE('',#24848,#24868,#23187,.T.);
#30721=EDGE_CURVE('',#24869,#24870,#23188,.T.);
#30722=EDGE_CURVE('',#24869,#24871,#11001,.T.);
#30723=EDGE_CURVE('',#24871,#24872,#23189,.T.);
#30724=EDGE_CURVE('',#24870,#24872,#11002,.T.);
#30725=EDGE_CURVE('',#24873,#24869,#23190,.T.);
#30726=EDGE_CURVE('',#24873,#24874,#11003,.T.);
#30727=EDGE_CURVE('',#24874,#24871,#23191,.T.);
#30728=EDGE_CURVE('',#24875,#24873,#23192,.T.);
#30729=EDGE_CURVE('',#24875,#24876,#11004,.T.);
#30730=EDGE_CURVE('',#24876,#24874,#23193,.T.);
#30731=EDGE_CURVE('',#24877,#24875,#11005,.T.);
#30732=EDGE_CURVE('',#24877,#24878,#11006,.T.);
#30733=EDGE_CURVE('',#24878,#24876,#11007,.T.);
#30734=EDGE_CURVE('',#24879,#24877,#23194,.T.);
#30735=EDGE_CURVE('',#24879,#24880,#11008,.T.);
#30736=EDGE_CURVE('',#24880,#24878,#23195,.T.);
#30737=EDGE_CURVE('',#24881,#24879,#23196,.T.);
#30738=EDGE_CURVE('',#24881,#24882,#11009,.T.);
#30739=EDGE_CURVE('',#24882,#24880,#23197,.T.);
#30740=EDGE_CURVE('',#24883,#24881,#23198,.T.);
#30741=EDGE_CURVE('',#24883,#24884,#11010,.T.);
#30742=EDGE_CURVE('',#24884,#24882,#23199,.T.);
#30743=EDGE_CURVE('',#24885,#24883,#11011,.T.);
#30744=EDGE_CURVE('',#24885,#24886,#11012,.T.);
#30745=EDGE_CURVE('',#24886,#24884,#11013,.T.);
#30746=EDGE_CURVE('',#24887,#24885,#11014,.T.);
#30747=EDGE_CURVE('',#24887,#24888,#11015,.T.);
#30748=EDGE_CURVE('',#24888,#24886,#11016,.T.);
#30749=EDGE_CURVE('',#24889,#24887,#11017,.T.);
#30750=EDGE_CURVE('',#24889,#24890,#11018,.T.);
#30751=EDGE_CURVE('',#24890,#24888,#11019,.T.);
#30752=EDGE_CURVE('',#24870,#24889,#11020,.T.);
#30753=EDGE_CURVE('',#24872,#24890,#11021,.T.);
#30754=EDGE_CURVE('',#24891,#24892,#23200,.T.);
#30755=EDGE_CURVE('',#24891,#24893,#11022,.T.);
#30756=EDGE_CURVE('',#24893,#24894,#23201,.T.);
#30757=EDGE_CURVE('',#24892,#24894,#11023,.T.);
#30758=EDGE_CURVE('',#24895,#24891,#23202,.T.);
#30759=EDGE_CURVE('',#24895,#24896,#11024,.T.);
#30760=EDGE_CURVE('',#24896,#24893,#23203,.T.);
#30761=EDGE_CURVE('',#24897,#24895,#23204,.T.);
#30762=EDGE_CURVE('',#24897,#24898,#11025,.T.);
#30763=EDGE_CURVE('',#24898,#24896,#23205,.T.);
#30764=EDGE_CURVE('',#24899,#24897,#23206,.T.);
#30765=EDGE_CURVE('',#24899,#24900,#11026,.T.);
#30766=EDGE_CURVE('',#24900,#24898,#23207,.T.);
#30767=EDGE_CURVE('',#24901,#24899,#23208,.T.);
#30768=EDGE_CURVE('',#24901,#24902,#11027,.T.);
#30769=EDGE_CURVE('',#24902,#24900,#23209,.T.);
#30770=EDGE_CURVE('',#24903,#24901,#23210,.T.);
#30771=EDGE_CURVE('',#24903,#24904,#11028,.T.);
#30772=EDGE_CURVE('',#24904,#24902,#23211,.T.);
#30773=EDGE_CURVE('',#24905,#24903,#23212,.T.);
#30774=EDGE_CURVE('',#24905,#24906,#11029,.T.);
#30775=EDGE_CURVE('',#24906,#24904,#23213,.T.);
#30776=EDGE_CURVE('',#24892,#24905,#23214,.T.);
#30777=EDGE_CURVE('',#24894,#24906,#23215,.T.);
#30778=EDGE_CURVE('',#24907,#24908,#23216,.T.);
#30779=EDGE_CURVE('',#24907,#24909,#11030,.T.);
#30780=EDGE_CURVE('',#24909,#24910,#23217,.T.);
#30781=EDGE_CURVE('',#24908,#24910,#11031,.T.);
#30782=EDGE_CURVE('',#24911,#24907,#23218,.T.);
#30783=EDGE_CURVE('',#24911,#24912,#11032,.T.);
#30784=EDGE_CURVE('',#24912,#24909,#23219,.T.);
#30785=EDGE_CURVE('',#24913,#24911,#23220,.T.);
#30786=EDGE_CURVE('',#24913,#24914,#11033,.T.);
#30787=EDGE_CURVE('',#24914,#24912,#23221,.T.);
#30788=EDGE_CURVE('',#24915,#24913,#23222,.T.);
#30789=EDGE_CURVE('',#24915,#24916,#11034,.T.);
#30790=EDGE_CURVE('',#24916,#24914,#23223,.T.);
#30791=EDGE_CURVE('',#24917,#24915,#23224,.T.);
#30792=EDGE_CURVE('',#24917,#24918,#11035,.T.);
#30793=EDGE_CURVE('',#24918,#24916,#23225,.T.);
#30794=EDGE_CURVE('',#24919,#24917,#23226,.T.);
#30795=EDGE_CURVE('',#24919,#24920,#11036,.T.);
#30796=EDGE_CURVE('',#24920,#24918,#23227,.T.);
#30797=EDGE_CURVE('',#24921,#24919,#23228,.T.);
#30798=EDGE_CURVE('',#24921,#24922,#11037,.T.);
#30799=EDGE_CURVE('',#24922,#24920,#23229,.T.);
#30800=EDGE_CURVE('',#24923,#24921,#23230,.T.);
#30801=EDGE_CURVE('',#24923,#24924,#11038,.T.);
#30802=EDGE_CURVE('',#24924,#24922,#23231,.T.);
#30803=EDGE_CURVE('',#24925,#24923,#23232,.T.);
#30804=EDGE_CURVE('',#24925,#24926,#11039,.T.);
#30805=EDGE_CURVE('',#24926,#24924,#23233,.T.);
#30806=EDGE_CURVE('',#24927,#24925,#23234,.T.);
#30807=EDGE_CURVE('',#24927,#24928,#11040,.T.);
#30808=EDGE_CURVE('',#24928,#24926,#23235,.T.);
#30809=EDGE_CURVE('',#24929,#24927,#23236,.T.);
#30810=EDGE_CURVE('',#24929,#24930,#11041,.T.);
#30811=EDGE_CURVE('',#24930,#24928,#23237,.T.);
#30812=EDGE_CURVE('',#24908,#24929,#23238,.T.);
#30813=EDGE_CURVE('',#24910,#24930,#23239,.T.);
#30814=EDGE_CURVE('',#24931,#24932,#23240,.T.);
#30815=EDGE_CURVE('',#24931,#24933,#11042,.T.);
#30816=EDGE_CURVE('',#24933,#24934,#23241,.T.);
#30817=EDGE_CURVE('',#24932,#24934,#11043,.T.);
#30818=EDGE_CURVE('',#24935,#24931,#23242,.T.);
#30819=EDGE_CURVE('',#24935,#24936,#11044,.T.);
#30820=EDGE_CURVE('',#24936,#24933,#23243,.T.);
#30821=EDGE_CURVE('',#24937,#24935,#23244,.T.);
#30822=EDGE_CURVE('',#24937,#24938,#11045,.T.);
#30823=EDGE_CURVE('',#24938,#24936,#23245,.T.);
#30824=EDGE_CURVE('',#24939,#24937,#23246,.T.);
#30825=EDGE_CURVE('',#24939,#24940,#11046,.T.);
#30826=EDGE_CURVE('',#24940,#24938,#23247,.T.);
#30827=EDGE_CURVE('',#24941,#24939,#23248,.T.);
#30828=EDGE_CURVE('',#24941,#24942,#11047,.T.);
#30829=EDGE_CURVE('',#24942,#24940,#23249,.T.);
#30830=EDGE_CURVE('',#24943,#24941,#23250,.T.);
#30831=EDGE_CURVE('',#24943,#24944,#11048,.T.);
#30832=EDGE_CURVE('',#24944,#24942,#23251,.T.);
#30833=EDGE_CURVE('',#24945,#24943,#23252,.T.);
#30834=EDGE_CURVE('',#24945,#24946,#11049,.T.);
#30835=EDGE_CURVE('',#24946,#24944,#23253,.T.);
#30836=EDGE_CURVE('',#24947,#24945,#23254,.T.);
#30837=EDGE_CURVE('',#24947,#24948,#11050,.T.);
#30838=EDGE_CURVE('',#24948,#24946,#23255,.T.);
#30839=EDGE_CURVE('',#24932,#24947,#23256,.T.);
#30840=EDGE_CURVE('',#24934,#24948,#23257,.T.);
#30841=EDGE_CURVE('',#24949,#24950,#23258,.T.);
#30842=EDGE_CURVE('',#24949,#24951,#11051,.T.);
#30843=EDGE_CURVE('',#24951,#24952,#23259,.T.);
#30844=EDGE_CURVE('',#24950,#24952,#11052,.T.);
#30845=EDGE_CURVE('',#24953,#24949,#23260,.T.);
#30846=EDGE_CURVE('',#24953,#24954,#11053,.T.);
#30847=EDGE_CURVE('',#24954,#24951,#23261,.T.);
#30848=EDGE_CURVE('',#24955,#24953,#23262,.T.);
#30849=EDGE_CURVE('',#24955,#24956,#11054,.T.);
#30850=EDGE_CURVE('',#24956,#24954,#23263,.T.);
#30851=EDGE_CURVE('',#24957,#24955,#23264,.T.);
#30852=EDGE_CURVE('',#24957,#24958,#11055,.T.);
#30853=EDGE_CURVE('',#24958,#24956,#23265,.T.);
#30854=EDGE_CURVE('',#24959,#24957,#23266,.T.);
#30855=EDGE_CURVE('',#24959,#24960,#11056,.T.);
#30856=EDGE_CURVE('',#24960,#24958,#23267,.T.);
#30857=EDGE_CURVE('',#24961,#24959,#23268,.T.);
#30858=EDGE_CURVE('',#24961,#24962,#11057,.T.);
#30859=EDGE_CURVE('',#24962,#24960,#23269,.T.);
#30860=EDGE_CURVE('',#24963,#24961,#23270,.T.);
#30861=EDGE_CURVE('',#24963,#24964,#11058,.T.);
#30862=EDGE_CURVE('',#24964,#24962,#23271,.T.);
#30863=EDGE_CURVE('',#24965,#24963,#23272,.T.);
#30864=EDGE_CURVE('',#24965,#24966,#11059,.T.);
#30865=EDGE_CURVE('',#24966,#24964,#23273,.T.);
#30866=EDGE_CURVE('',#24967,#24965,#23274,.T.);
#30867=EDGE_CURVE('',#24967,#24968,#11060,.T.);
#30868=EDGE_CURVE('',#24968,#24966,#23275,.T.);
#30869=EDGE_CURVE('',#24969,#24967,#23276,.T.);
#30870=EDGE_CURVE('',#24969,#24970,#11061,.T.);
#30871=EDGE_CURVE('',#24970,#24968,#23277,.T.);
#30872=EDGE_CURVE('',#24971,#24969,#23278,.T.);
#30873=EDGE_CURVE('',#24971,#24972,#11062,.T.);
#30874=EDGE_CURVE('',#24972,#24970,#23279,.T.);
#30875=EDGE_CURVE('',#24973,#24971,#23280,.T.);
#30876=EDGE_CURVE('',#24973,#24974,#11063,.T.);
#30877=EDGE_CURVE('',#24974,#24972,#23281,.T.);
#30878=EDGE_CURVE('',#24975,#24973,#23282,.T.);
#30879=EDGE_CURVE('',#24975,#24976,#11064,.T.);
#30880=EDGE_CURVE('',#24976,#24974,#23283,.T.);
#30881=EDGE_CURVE('',#24977,#24975,#23284,.T.);
#30882=EDGE_CURVE('',#24977,#24978,#11065,.T.);
#30883=EDGE_CURVE('',#24978,#24976,#23285,.T.);
#30884=EDGE_CURVE('',#24979,#24977,#23286,.T.);
#30885=EDGE_CURVE('',#24979,#24980,#11066,.T.);
#30886=EDGE_CURVE('',#24980,#24978,#23287,.T.);
#30887=EDGE_CURVE('',#24981,#24979,#23288,.T.);
#30888=EDGE_CURVE('',#24981,#24982,#11067,.T.);
#30889=EDGE_CURVE('',#24982,#24980,#23289,.T.);
#30890=EDGE_CURVE('',#24983,#24981,#23290,.T.);
#30891=EDGE_CURVE('',#24983,#24984,#11068,.T.);
#30892=EDGE_CURVE('',#24984,#24982,#23291,.T.);
#30893=EDGE_CURVE('',#24985,#24983,#11069,.T.);
#30894=EDGE_CURVE('',#24985,#24986,#11070,.T.);
#30895=EDGE_CURVE('',#24986,#24984,#11071,.T.);
#30896=EDGE_CURVE('',#24950,#24985,#23292,.T.);
#30897=EDGE_CURVE('',#24952,#24986,#23293,.T.);
#30898=EDGE_CURVE('',#24987,#24988,#23294,.T.);
#30899=EDGE_CURVE('',#24987,#24989,#11072,.T.);
#30900=EDGE_CURVE('',#24989,#24990,#23295,.T.);
#30901=EDGE_CURVE('',#24988,#24990,#11073,.T.);
#30902=EDGE_CURVE('',#24991,#24987,#23296,.T.);
#30903=EDGE_CURVE('',#24991,#24992,#11074,.T.);
#30904=EDGE_CURVE('',#24992,#24989,#23297,.T.);
#30905=EDGE_CURVE('',#24993,#24991,#23298,.T.);
#30906=EDGE_CURVE('',#24993,#24994,#11075,.T.);
#30907=EDGE_CURVE('',#24994,#24992,#23299,.T.);
#30908=EDGE_CURVE('',#24995,#24993,#23300,.T.);
#30909=EDGE_CURVE('',#24995,#24996,#11076,.T.);
#30910=EDGE_CURVE('',#24996,#24994,#23301,.T.);
#30911=EDGE_CURVE('',#24997,#24995,#23302,.T.);
#30912=EDGE_CURVE('',#24997,#24998,#11077,.T.);
#30913=EDGE_CURVE('',#24998,#24996,#23303,.T.);
#30914=EDGE_CURVE('',#24999,#24997,#23304,.T.);
#30915=EDGE_CURVE('',#24999,#25000,#11078,.T.);
#30916=EDGE_CURVE('',#25000,#24998,#23305,.T.);
#30917=EDGE_CURVE('',#25001,#24999,#23306,.T.);
#30918=EDGE_CURVE('',#25001,#25002,#11079,.T.);
#30919=EDGE_CURVE('',#25002,#25000,#23307,.T.);
#30920=EDGE_CURVE('',#24988,#25001,#23308,.T.);
#30921=EDGE_CURVE('',#24990,#25002,#23309,.T.);
#30922=EDGE_CURVE('',#25003,#25004,#23310,.T.);
#30923=EDGE_CURVE('',#25003,#25005,#11080,.T.);
#30924=EDGE_CURVE('',#25005,#25006,#23311,.T.);
#30925=EDGE_CURVE('',#25004,#25006,#11081,.T.);
#30926=EDGE_CURVE('',#25007,#25003,#23312,.T.);
#30927=EDGE_CURVE('',#25007,#25008,#11082,.T.);
#30928=EDGE_CURVE('',#25008,#25005,#23313,.T.);
#30929=EDGE_CURVE('',#25009,#25007,#23314,.T.);
#30930=EDGE_CURVE('',#25009,#25010,#11083,.T.);
#30931=EDGE_CURVE('',#25010,#25008,#23315,.T.);
#30932=EDGE_CURVE('',#25011,#25009,#23316,.T.);
#30933=EDGE_CURVE('',#25011,#25012,#11084,.T.);
#30934=EDGE_CURVE('',#25012,#25010,#23317,.T.);
#30935=EDGE_CURVE('',#25013,#25011,#23318,.T.);
#30936=EDGE_CURVE('',#25013,#25014,#11085,.T.);
#30937=EDGE_CURVE('',#25014,#25012,#23319,.T.);
#30938=EDGE_CURVE('',#25015,#25013,#23320,.T.);
#30939=EDGE_CURVE('',#25015,#25016,#11086,.T.);
#30940=EDGE_CURVE('',#25016,#25014,#23321,.T.);
#30941=EDGE_CURVE('',#25017,#25015,#23322,.T.);
#30942=EDGE_CURVE('',#25017,#25018,#11087,.T.);
#30943=EDGE_CURVE('',#25018,#25016,#23323,.T.);
#30944=EDGE_CURVE('',#25019,#25017,#23324,.T.);
#30945=EDGE_CURVE('',#25019,#25020,#11088,.T.);
#30946=EDGE_CURVE('',#25020,#25018,#23325,.T.);
#30947=EDGE_CURVE('',#25021,#25019,#23326,.T.);
#30948=EDGE_CURVE('',#25021,#25022,#11089,.T.);
#30949=EDGE_CURVE('',#25022,#25020,#23327,.T.);
#30950=EDGE_CURVE('',#25023,#25021,#23328,.T.);
#30951=EDGE_CURVE('',#25023,#25024,#11090,.T.);
#30952=EDGE_CURVE('',#25024,#25022,#23329,.T.);
#30953=EDGE_CURVE('',#25025,#25023,#23330,.T.);
#30954=EDGE_CURVE('',#25025,#25026,#11091,.T.);
#30955=EDGE_CURVE('',#25026,#25024,#23331,.T.);
#30956=EDGE_CURVE('',#25004,#25025,#23332,.T.);
#30957=EDGE_CURVE('',#25006,#25026,#23333,.T.);
#30958=EDGE_CURVE('',#25027,#25028,#23334,.T.);
#30959=EDGE_CURVE('',#25027,#25029,#11092,.T.);
#30960=EDGE_CURVE('',#25029,#25030,#23335,.T.);
#30961=EDGE_CURVE('',#25028,#25030,#11093,.T.);
#30962=EDGE_CURVE('',#25031,#25027,#23336,.T.);
#30963=EDGE_CURVE('',#25031,#25032,#11094,.T.);
#30964=EDGE_CURVE('',#25032,#25029,#23337,.T.);
#30965=EDGE_CURVE('',#25033,#25031,#23338,.T.);
#30966=EDGE_CURVE('',#25033,#25034,#11095,.T.);
#30967=EDGE_CURVE('',#25034,#25032,#23339,.T.);
#30968=EDGE_CURVE('',#25035,#25033,#23340,.T.);
#30969=EDGE_CURVE('',#25035,#25036,#11096,.T.);
#30970=EDGE_CURVE('',#25036,#25034,#23341,.T.);
#30971=EDGE_CURVE('',#25037,#25035,#23342,.T.);
#30972=EDGE_CURVE('',#25037,#25038,#11097,.T.);
#30973=EDGE_CURVE('',#25038,#25036,#23343,.T.);
#30974=EDGE_CURVE('',#25039,#25037,#23344,.T.);
#30975=EDGE_CURVE('',#25039,#25040,#11098,.T.);
#30976=EDGE_CURVE('',#25040,#25038,#23345,.T.);
#30977=EDGE_CURVE('',#25041,#25039,#11099,.T.);
#30978=EDGE_CURVE('',#25041,#25042,#11100,.T.);
#30979=EDGE_CURVE('',#25042,#25040,#11101,.T.);
#30980=EDGE_CURVE('',#25043,#25041,#11102,.T.);
#30981=EDGE_CURVE('',#25043,#25044,#11103,.T.);
#30982=EDGE_CURVE('',#25044,#25042,#11104,.T.);
#30983=EDGE_CURVE('',#25045,#25043,#11105,.T.);
#30984=EDGE_CURVE('',#25045,#25046,#11106,.T.);
#30985=EDGE_CURVE('',#25046,#25044,#11107,.T.);
#30986=EDGE_CURVE('',#25047,#25045,#11108,.T.);
#30987=EDGE_CURVE('',#25047,#25048,#11109,.T.);
#30988=EDGE_CURVE('',#25048,#25046,#11110,.T.);
#30989=EDGE_CURVE('',#25049,#25047,#11111,.T.);
#30990=EDGE_CURVE('',#25049,#25050,#11112,.T.);
#30991=EDGE_CURVE('',#25050,#25048,#11113,.T.);
#30992=EDGE_CURVE('',#25051,#25049,#11114,.T.);
#30993=EDGE_CURVE('',#25051,#25052,#11115,.T.);
#30994=EDGE_CURVE('',#25052,#25050,#11116,.T.);
#30995=EDGE_CURVE('',#25053,#25051,#23346,.T.);
#30996=EDGE_CURVE('',#25053,#25054,#11117,.T.);
#30997=EDGE_CURVE('',#25054,#25052,#23347,.T.);
#30998=EDGE_CURVE('',#25055,#25053,#23348,.T.);
#30999=EDGE_CURVE('',#25055,#25056,#11118,.T.);
#31000=EDGE_CURVE('',#25056,#25054,#23349,.T.);
#31001=EDGE_CURVE('',#25057,#25055,#23350,.T.);
#31002=EDGE_CURVE('',#25057,#25058,#11119,.T.);
#31003=EDGE_CURVE('',#25058,#25056,#23351,.T.);
#31004=EDGE_CURVE('',#25059,#25057,#23352,.T.);
#31005=EDGE_CURVE('',#25059,#25060,#11120,.T.);
#31006=EDGE_CURVE('',#25060,#25058,#23353,.T.);
#31007=EDGE_CURVE('',#25061,#25059,#23354,.T.);
#31008=EDGE_CURVE('',#25061,#25062,#11121,.T.);
#31009=EDGE_CURVE('',#25062,#25060,#23355,.T.);
#31010=EDGE_CURVE('',#25063,#25061,#23356,.T.);
#31011=EDGE_CURVE('',#25063,#25064,#11122,.T.);
#31012=EDGE_CURVE('',#25064,#25062,#23357,.T.);
#31013=EDGE_CURVE('',#25065,#25063,#23358,.T.);
#31014=EDGE_CURVE('',#25065,#25066,#11123,.T.);
#31015=EDGE_CURVE('',#25066,#25064,#23359,.T.);
#31016=EDGE_CURVE('',#25067,#25065,#23360,.T.);
#31017=EDGE_CURVE('',#25067,#25068,#11124,.T.);
#31018=EDGE_CURVE('',#25068,#25066,#23361,.T.);
#31019=EDGE_CURVE('',#25069,#25067,#11125,.T.);
#31020=EDGE_CURVE('',#25069,#25070,#11126,.T.);
#31021=EDGE_CURVE('',#25070,#25068,#11127,.T.);
#31022=EDGE_CURVE('',#25028,#25069,#23362,.T.);
#31023=EDGE_CURVE('',#25030,#25070,#23363,.T.);
#31024=EDGE_CURVE('',#25071,#25072,#23364,.T.);
#31025=EDGE_CURVE('',#25071,#25073,#11128,.T.);
#31026=EDGE_CURVE('',#25073,#25074,#23365,.T.);
#31027=EDGE_CURVE('',#25072,#25074,#11129,.T.);
#31028=EDGE_CURVE('',#25075,#25071,#23366,.T.);
#31029=EDGE_CURVE('',#25075,#25076,#11130,.T.);
#31030=EDGE_CURVE('',#25076,#25073,#23367,.T.);
#31031=EDGE_CURVE('',#25077,#25075,#23368,.T.);
#31032=EDGE_CURVE('',#25077,#25078,#11131,.T.);
#31033=EDGE_CURVE('',#25078,#25076,#23369,.T.);
#31034=EDGE_CURVE('',#25079,#25077,#23370,.T.);
#31035=EDGE_CURVE('',#25079,#25080,#11132,.T.);
#31036=EDGE_CURVE('',#25080,#25078,#23371,.T.);
#31037=EDGE_CURVE('',#25081,#25079,#23372,.T.);
#31038=EDGE_CURVE('',#25081,#25082,#11133,.T.);
#31039=EDGE_CURVE('',#25082,#25080,#23373,.T.);
#31040=EDGE_CURVE('',#25083,#25081,#23374,.T.);
#31041=EDGE_CURVE('',#25083,#25084,#11134,.T.);
#31042=EDGE_CURVE('',#25084,#25082,#23375,.T.);
#31043=EDGE_CURVE('',#25085,#25083,#23376,.T.);
#31044=EDGE_CURVE('',#25085,#25086,#11135,.T.);
#31045=EDGE_CURVE('',#25086,#25084,#23377,.T.);
#31046=EDGE_CURVE('',#25072,#25085,#23378,.T.);
#31047=EDGE_CURVE('',#25074,#25086,#23379,.T.);
#31048=EDGE_CURVE('',#25087,#25088,#23380,.T.);
#31049=EDGE_CURVE('',#25087,#25089,#11136,.T.);
#31050=EDGE_CURVE('',#25089,#25090,#23381,.T.);
#31051=EDGE_CURVE('',#25088,#25090,#11137,.T.);
#31052=EDGE_CURVE('',#25091,#25087,#23382,.T.);
#31053=EDGE_CURVE('',#25091,#25092,#11138,.T.);
#31054=EDGE_CURVE('',#25092,#25089,#23383,.T.);
#31055=EDGE_CURVE('',#25093,#25091,#23384,.T.);
#31056=EDGE_CURVE('',#25093,#25094,#11139,.T.);
#31057=EDGE_CURVE('',#25094,#25092,#23385,.T.);
#31058=EDGE_CURVE('',#25095,#25093,#23386,.T.);
#31059=EDGE_CURVE('',#25095,#25096,#11140,.T.);
#31060=EDGE_CURVE('',#25096,#25094,#23387,.T.);
#31061=EDGE_CURVE('',#25097,#25095,#23388,.T.);
#31062=EDGE_CURVE('',#25097,#25098,#11141,.T.);
#31063=EDGE_CURVE('',#25098,#25096,#23389,.T.);
#31064=EDGE_CURVE('',#25099,#25097,#23390,.T.);
#31065=EDGE_CURVE('',#25099,#25100,#11142,.T.);
#31066=EDGE_CURVE('',#25100,#25098,#23391,.T.);
#31067=EDGE_CURVE('',#25101,#25099,#23392,.T.);
#31068=EDGE_CURVE('',#25101,#25102,#11143,.T.);
#31069=EDGE_CURVE('',#25102,#25100,#23393,.T.);
#31070=EDGE_CURVE('',#25103,#25101,#23394,.T.);
#31071=EDGE_CURVE('',#25103,#25104,#11144,.T.);
#31072=EDGE_CURVE('',#25104,#25102,#23395,.T.);
#31073=EDGE_CURVE('',#25105,#25103,#23396,.T.);
#31074=EDGE_CURVE('',#25105,#25106,#11145,.T.);
#31075=EDGE_CURVE('',#25106,#25104,#23397,.T.);
#31076=EDGE_CURVE('',#25107,#25105,#23398,.T.);
#31077=EDGE_CURVE('',#25107,#25108,#11146,.T.);
#31078=EDGE_CURVE('',#25108,#25106,#23399,.T.);
#31079=EDGE_CURVE('',#25109,#25107,#23400,.T.);
#31080=EDGE_CURVE('',#25109,#25110,#11147,.T.);
#31081=EDGE_CURVE('',#25110,#25108,#23401,.T.);
#31082=EDGE_CURVE('',#25088,#25109,#23402,.T.);
#31083=EDGE_CURVE('',#25090,#25110,#23403,.T.);
#31084=EDGE_CURVE('',#25111,#25112,#11148,.T.);
#31085=EDGE_CURVE('',#25111,#25113,#11149,.T.);
#31086=EDGE_CURVE('',#25113,#25114,#11150,.T.);
#31087=EDGE_CURVE('',#25112,#25114,#11151,.T.);
#31088=EDGE_CURVE('',#25115,#25111,#11152,.T.);
#31089=EDGE_CURVE('',#25115,#25116,#11153,.T.);
#31090=EDGE_CURVE('',#25116,#25113,#11154,.T.);
#31091=EDGE_CURVE('',#25112,#25115,#11155,.T.);
#31092=EDGE_CURVE('',#25114,#25116,#11156,.T.);
#31093=EDGE_CURVE('',#25117,#25118,#11157,.T.);
#31094=EDGE_CURVE('',#25117,#25119,#11158,.T.);
#31095=EDGE_CURVE('',#25119,#25120,#11159,.T.);
#31096=EDGE_CURVE('',#25118,#25120,#11160,.T.);
#31097=EDGE_CURVE('',#25121,#25117,#11161,.T.);
#31098=EDGE_CURVE('',#25121,#25122,#11162,.T.);
#31099=EDGE_CURVE('',#25122,#25119,#11163,.T.);
#31100=EDGE_CURVE('',#25123,#25121,#11164,.T.);
#31101=EDGE_CURVE('',#25123,#25124,#11165,.T.);
#31102=EDGE_CURVE('',#25124,#25122,#11166,.T.);
#31103=EDGE_CURVE('',#25125,#25123,#11167,.T.);
#31104=EDGE_CURVE('',#25125,#25126,#11168,.T.);
#31105=EDGE_CURVE('',#25126,#25124,#11169,.T.);
#31106=EDGE_CURVE('',#25127,#25125,#11170,.T.);
#31107=EDGE_CURVE('',#25127,#25128,#11171,.T.);
#31108=EDGE_CURVE('',#25128,#25126,#11172,.T.);
#31109=EDGE_CURVE('',#25129,#25127,#11173,.T.);
#31110=EDGE_CURVE('',#25129,#25130,#11174,.T.);
#31111=EDGE_CURVE('',#25130,#25128,#11175,.T.);
#31112=EDGE_CURVE('',#25131,#25129,#11176,.T.);
#31113=EDGE_CURVE('',#25131,#25132,#11177,.T.);
#31114=EDGE_CURVE('',#25132,#25130,#11178,.T.);
#31115=EDGE_CURVE('',#25133,#25131,#11179,.T.);
#31116=EDGE_CURVE('',#25133,#25134,#11180,.T.);
#31117=EDGE_CURVE('',#25134,#25132,#11181,.T.);
#31118=EDGE_CURVE('',#25135,#25133,#11182,.T.);
#31119=EDGE_CURVE('',#25135,#25136,#11183,.T.);
#31120=EDGE_CURVE('',#25136,#25134,#11184,.T.);
#31121=EDGE_CURVE('',#25137,#25135,#11185,.T.);
#31122=EDGE_CURVE('',#25137,#25138,#11186,.T.);
#31123=EDGE_CURVE('',#25138,#25136,#11187,.T.);
#31124=EDGE_CURVE('',#25118,#25137,#11188,.T.);
#31125=EDGE_CURVE('',#25120,#25138,#11189,.T.);
#31126=EDGE_CURVE('',#25139,#25140,#23404,.T.);
#31127=EDGE_CURVE('',#25139,#25141,#11190,.T.);
#31128=EDGE_CURVE('',#25141,#25142,#23405,.T.);
#31129=EDGE_CURVE('',#25140,#25142,#11191,.T.);
#31130=EDGE_CURVE('',#25143,#25139,#23406,.T.);
#31131=EDGE_CURVE('',#25143,#25144,#11192,.T.);
#31132=EDGE_CURVE('',#25144,#25141,#23407,.T.);
#31133=EDGE_CURVE('',#25145,#25143,#23408,.T.);
#31134=EDGE_CURVE('',#25145,#25146,#11193,.T.);
#31135=EDGE_CURVE('',#25146,#25144,#23409,.T.);
#31136=EDGE_CURVE('',#25147,#25145,#23410,.T.);
#31137=EDGE_CURVE('',#25147,#25148,#11194,.T.);
#31138=EDGE_CURVE('',#25148,#25146,#23411,.T.);
#31139=EDGE_CURVE('',#25149,#25147,#23412,.T.);
#31140=EDGE_CURVE('',#25149,#25150,#11195,.T.);
#31141=EDGE_CURVE('',#25150,#25148,#23413,.T.);
#31142=EDGE_CURVE('',#25151,#25149,#23414,.T.);
#31143=EDGE_CURVE('',#25151,#25152,#11196,.T.);
#31144=EDGE_CURVE('',#25152,#25150,#23415,.T.);
#31145=EDGE_CURVE('',#25153,#25151,#23416,.T.);
#31146=EDGE_CURVE('',#25153,#25154,#11197,.T.);
#31147=EDGE_CURVE('',#25154,#25152,#23417,.T.);
#31148=EDGE_CURVE('',#25140,#25153,#23418,.T.);
#31149=EDGE_CURVE('',#25142,#25154,#23419,.T.);
#31150=EDGE_CURVE('',#25155,#25156,#23420,.T.);
#31151=EDGE_CURVE('',#25155,#25157,#11198,.T.);
#31152=EDGE_CURVE('',#25157,#25158,#23421,.T.);
#31153=EDGE_CURVE('',#25156,#25158,#11199,.T.);
#31154=EDGE_CURVE('',#25159,#25155,#23422,.T.);
#31155=EDGE_CURVE('',#25159,#25160,#11200,.T.);
#31156=EDGE_CURVE('',#25160,#25157,#23423,.T.);
#31157=EDGE_CURVE('',#25161,#25159,#23424,.T.);
#31158=EDGE_CURVE('',#25161,#25162,#11201,.T.);
#31159=EDGE_CURVE('',#25162,#25160,#23425,.T.);
#31160=EDGE_CURVE('',#25163,#25161,#23426,.T.);
#31161=EDGE_CURVE('',#25163,#25164,#11202,.T.);
#31162=EDGE_CURVE('',#25164,#25162,#23427,.T.);
#31163=EDGE_CURVE('',#25165,#25163,#23428,.T.);
#31164=EDGE_CURVE('',#25165,#25166,#11203,.T.);
#31165=EDGE_CURVE('',#25166,#25164,#23429,.T.);
#31166=EDGE_CURVE('',#25167,#25165,#23430,.T.);
#31167=EDGE_CURVE('',#25167,#25168,#11204,.T.);
#31168=EDGE_CURVE('',#25168,#25166,#23431,.T.);
#31169=EDGE_CURVE('',#25169,#25167,#23432,.T.);
#31170=EDGE_CURVE('',#25169,#25170,#11205,.T.);
#31171=EDGE_CURVE('',#25170,#25168,#23433,.T.);
#31172=EDGE_CURVE('',#25171,#25169,#23434,.T.);
#31173=EDGE_CURVE('',#25171,#25172,#11206,.T.);
#31174=EDGE_CURVE('',#25172,#25170,#23435,.T.);
#31175=EDGE_CURVE('',#25173,#25171,#23436,.T.);
#31176=EDGE_CURVE('',#25173,#25174,#11207,.T.);
#31177=EDGE_CURVE('',#25174,#25172,#23437,.T.);
#31178=EDGE_CURVE('',#25175,#25173,#23438,.T.);
#31179=EDGE_CURVE('',#25175,#25176,#11208,.T.);
#31180=EDGE_CURVE('',#25176,#25174,#23439,.T.);
#31181=EDGE_CURVE('',#25177,#25175,#23440,.T.);
#31182=EDGE_CURVE('',#25177,#25178,#11209,.T.);
#31183=EDGE_CURVE('',#25178,#25176,#23441,.T.);
#31184=EDGE_CURVE('',#25156,#25177,#23442,.T.);
#31185=EDGE_CURVE('',#25158,#25178,#23443,.T.);
#31186=EDGE_CURVE('',#25179,#25180,#23444,.T.);
#31187=EDGE_CURVE('',#25179,#25181,#11210,.T.);
#31188=EDGE_CURVE('',#25181,#25182,#23445,.T.);
#31189=EDGE_CURVE('',#25180,#25182,#11211,.T.);
#31190=EDGE_CURVE('',#25183,#25179,#23446,.T.);
#31191=EDGE_CURVE('',#25183,#25184,#11212,.T.);
#31192=EDGE_CURVE('',#25184,#25181,#23447,.T.);
#31193=EDGE_CURVE('',#25185,#25183,#23448,.T.);
#31194=EDGE_CURVE('',#25185,#25186,#11213,.T.);
#31195=EDGE_CURVE('',#25186,#25184,#23449,.T.);
#31196=EDGE_CURVE('',#25187,#25185,#23450,.T.);
#31197=EDGE_CURVE('',#25187,#25188,#11214,.T.);
#31198=EDGE_CURVE('',#25188,#25186,#23451,.T.);
#31199=EDGE_CURVE('',#25189,#25187,#23452,.T.);
#31200=EDGE_CURVE('',#25189,#25190,#11215,.T.);
#31201=EDGE_CURVE('',#25190,#25188,#23453,.T.);
#31202=EDGE_CURVE('',#25191,#25189,#23454,.T.);
#31203=EDGE_CURVE('',#25191,#25192,#11216,.T.);
#31204=EDGE_CURVE('',#25192,#25190,#23455,.T.);
#31205=EDGE_CURVE('',#25193,#25191,#23456,.T.);
#31206=EDGE_CURVE('',#25193,#25194,#11217,.T.);
#31207=EDGE_CURVE('',#25194,#25192,#23457,.T.);
#31208=EDGE_CURVE('',#25195,#25193,#23458,.T.);
#31209=EDGE_CURVE('',#25195,#25196,#11218,.T.);
#31210=EDGE_CURVE('',#25196,#25194,#23459,.T.);
#31211=EDGE_CURVE('',#25197,#25195,#23460,.T.);
#31212=EDGE_CURVE('',#25197,#25198,#11219,.T.);
#31213=EDGE_CURVE('',#25198,#25196,#23461,.T.);
#31214=EDGE_CURVE('',#25199,#25197,#23462,.T.);
#31215=EDGE_CURVE('',#25199,#25200,#11220,.T.);
#31216=EDGE_CURVE('',#25200,#25198,#23463,.T.);
#31217=EDGE_CURVE('',#25201,#25199,#23464,.T.);
#31218=EDGE_CURVE('',#25201,#25202,#11221,.T.);
#31219=EDGE_CURVE('',#25202,#25200,#23465,.T.);
#31220=EDGE_CURVE('',#25203,#25201,#23466,.T.);
#31221=EDGE_CURVE('',#25203,#25204,#11222,.T.);
#31222=EDGE_CURVE('',#25204,#25202,#23467,.T.);
#31223=EDGE_CURVE('',#25205,#25203,#11223,.T.);
#31224=EDGE_CURVE('',#25205,#25206,#11224,.T.);
#31225=EDGE_CURVE('',#25206,#25204,#11225,.T.);
#31226=EDGE_CURVE('',#25207,#25205,#23468,.T.);
#31227=EDGE_CURVE('',#25207,#25208,#11226,.T.);
#31228=EDGE_CURVE('',#25208,#25206,#23469,.T.);
#31229=EDGE_CURVE('',#25209,#25207,#23470,.T.);
#31230=EDGE_CURVE('',#25209,#25210,#11227,.T.);
#31231=EDGE_CURVE('',#25210,#25208,#23471,.T.);
#31232=EDGE_CURVE('',#25211,#25209,#23472,.T.);
#31233=EDGE_CURVE('',#25211,#25212,#11228,.T.);
#31234=EDGE_CURVE('',#25212,#25210,#23473,.T.);
#31235=EDGE_CURVE('',#25213,#25211,#23474,.T.);
#31236=EDGE_CURVE('',#25213,#25214,#11229,.T.);
#31237=EDGE_CURVE('',#25214,#25212,#23475,.T.);
#31238=EDGE_CURVE('',#25215,#25213,#23476,.T.);
#31239=EDGE_CURVE('',#25215,#25216,#11230,.T.);
#31240=EDGE_CURVE('',#25216,#25214,#23477,.T.);
#31241=EDGE_CURVE('',#25217,#25215,#23478,.T.);
#31242=EDGE_CURVE('',#25217,#25218,#11231,.T.);
#31243=EDGE_CURVE('',#25218,#25216,#23479,.T.);
#31244=EDGE_CURVE('',#25219,#25217,#23480,.T.);
#31245=EDGE_CURVE('',#25219,#25220,#11232,.T.);
#31246=EDGE_CURVE('',#25220,#25218,#23481,.T.);
#31247=EDGE_CURVE('',#25221,#25219,#11233,.T.);
#31248=EDGE_CURVE('',#25221,#25222,#11234,.T.);
#31249=EDGE_CURVE('',#25222,#25220,#11235,.T.);
#31250=EDGE_CURVE('',#25223,#25221,#23482,.T.);
#31251=EDGE_CURVE('',#25223,#25224,#11236,.T.);
#31252=EDGE_CURVE('',#25224,#25222,#23483,.T.);
#31253=EDGE_CURVE('',#25225,#25223,#23484,.T.);
#31254=EDGE_CURVE('',#25225,#25226,#11237,.T.);
#31255=EDGE_CURVE('',#25226,#25224,#23485,.T.);
#31256=EDGE_CURVE('',#25227,#25225,#23486,.T.);
#31257=EDGE_CURVE('',#25227,#25228,#11238,.T.);
#31258=EDGE_CURVE('',#25228,#25226,#23487,.T.);
#31259=EDGE_CURVE('',#25229,#25227,#23488,.T.);
#31260=EDGE_CURVE('',#25229,#25230,#11239,.T.);
#31261=EDGE_CURVE('',#25230,#25228,#23489,.T.);
#31262=EDGE_CURVE('',#25231,#25229,#23490,.T.);
#31263=EDGE_CURVE('',#25231,#25232,#11240,.T.);
#31264=EDGE_CURVE('',#25232,#25230,#23491,.T.);
#31265=EDGE_CURVE('',#25233,#25231,#23492,.T.);
#31266=EDGE_CURVE('',#25233,#25234,#11241,.T.);
#31267=EDGE_CURVE('',#25234,#25232,#23493,.T.);
#31268=EDGE_CURVE('',#25235,#25233,#23494,.T.);
#31269=EDGE_CURVE('',#25235,#25236,#11242,.T.);
#31270=EDGE_CURVE('',#25236,#25234,#23495,.T.);
#31271=EDGE_CURVE('',#25237,#25235,#11243,.T.);
#31272=EDGE_CURVE('',#25237,#25238,#11244,.T.);
#31273=EDGE_CURVE('',#25238,#25236,#11245,.T.);
#31274=EDGE_CURVE('',#25180,#25237,#23496,.T.);
#31275=EDGE_CURVE('',#25182,#25238,#23497,.T.);
#31276=EDGE_CURVE('',#25239,#25240,#23498,.T.);
#31277=EDGE_CURVE('',#25239,#25241,#11246,.T.);
#31278=EDGE_CURVE('',#25241,#25242,#23499,.T.);
#31279=EDGE_CURVE('',#25240,#25242,#11247,.T.);
#31280=EDGE_CURVE('',#25243,#25239,#23500,.T.);
#31281=EDGE_CURVE('',#25243,#25244,#11248,.T.);
#31282=EDGE_CURVE('',#25244,#25241,#23501,.T.);
#31283=EDGE_CURVE('',#25245,#25243,#23502,.T.);
#31284=EDGE_CURVE('',#25245,#25246,#11249,.T.);
#31285=EDGE_CURVE('',#25246,#25244,#23503,.T.);
#31286=EDGE_CURVE('',#25247,#25245,#23504,.T.);
#31287=EDGE_CURVE('',#25247,#25248,#11250,.T.);
#31288=EDGE_CURVE('',#25248,#25246,#23505,.T.);
#31289=EDGE_CURVE('',#25249,#25247,#23506,.T.);
#31290=EDGE_CURVE('',#25249,#25250,#11251,.T.);
#31291=EDGE_CURVE('',#25250,#25248,#23507,.T.);
#31292=EDGE_CURVE('',#25251,#25249,#23508,.T.);
#31293=EDGE_CURVE('',#25251,#25252,#11252,.T.);
#31294=EDGE_CURVE('',#25252,#25250,#23509,.T.);
#31295=EDGE_CURVE('',#25253,#25251,#23510,.T.);
#31296=EDGE_CURVE('',#25253,#25254,#11253,.T.);
#31297=EDGE_CURVE('',#25254,#25252,#23511,.T.);
#31298=EDGE_CURVE('',#25240,#25253,#23512,.T.);
#31299=EDGE_CURVE('',#25242,#25254,#23513,.T.);
#31300=EDGE_CURVE('',#25255,#25256,#23514,.T.);
#31301=EDGE_CURVE('',#25255,#25257,#11254,.T.);
#31302=EDGE_CURVE('',#25257,#25258,#23515,.T.);
#31303=EDGE_CURVE('',#25256,#25258,#11255,.T.);
#31304=EDGE_CURVE('',#25259,#25255,#23516,.T.);
#31305=EDGE_CURVE('',#25259,#25260,#11256,.T.);
#31306=EDGE_CURVE('',#25260,#25257,#23517,.T.);
#31307=EDGE_CURVE('',#25261,#25259,#23518,.T.);
#31308=EDGE_CURVE('',#25261,#25262,#11257,.T.);
#31309=EDGE_CURVE('',#25262,#25260,#23519,.T.);
#31310=EDGE_CURVE('',#25263,#25261,#23520,.T.);
#31311=EDGE_CURVE('',#25263,#25264,#11258,.T.);
#31312=EDGE_CURVE('',#25264,#25262,#23521,.T.);
#31313=EDGE_CURVE('',#25265,#25263,#23522,.T.);
#31314=EDGE_CURVE('',#25265,#25266,#11259,.T.);
#31315=EDGE_CURVE('',#25266,#25264,#23523,.T.);
#31316=EDGE_CURVE('',#25267,#25265,#23524,.T.);
#31317=EDGE_CURVE('',#25267,#25268,#11260,.T.);
#31318=EDGE_CURVE('',#25268,#25266,#23525,.T.);
#31319=EDGE_CURVE('',#25269,#25267,#23526,.T.);
#31320=EDGE_CURVE('',#25269,#25270,#11261,.T.);
#31321=EDGE_CURVE('',#25270,#25268,#23527,.T.);
#31322=EDGE_CURVE('',#25271,#25269,#23528,.T.);
#31323=EDGE_CURVE('',#25271,#25272,#11262,.T.);
#31324=EDGE_CURVE('',#25272,#25270,#23529,.T.);
#31325=EDGE_CURVE('',#25273,#25271,#23530,.T.);
#31326=EDGE_CURVE('',#25273,#25274,#11263,.T.);
#31327=EDGE_CURVE('',#25274,#25272,#23531,.T.);
#31328=EDGE_CURVE('',#25275,#25273,#23532,.T.);
#31329=EDGE_CURVE('',#25275,#25276,#11264,.T.);
#31330=EDGE_CURVE('',#25276,#25274,#23533,.T.);
#31331=EDGE_CURVE('',#25277,#25275,#23534,.T.);
#31332=EDGE_CURVE('',#25277,#25278,#11265,.T.);
#31333=EDGE_CURVE('',#25278,#25276,#23535,.T.);
#31334=EDGE_CURVE('',#25256,#25277,#23536,.T.);
#31335=EDGE_CURVE('',#25258,#25278,#23537,.T.);
#31336=EDGE_CURVE('',#25279,#25280,#23538,.T.);
#31337=EDGE_CURVE('',#25279,#25281,#11266,.T.);
#31338=EDGE_CURVE('',#25281,#25282,#23539,.T.);
#31339=EDGE_CURVE('',#25280,#25282,#11267,.T.);
#31340=EDGE_CURVE('',#25283,#25279,#23540,.T.);
#31341=EDGE_CURVE('',#25283,#25284,#11268,.T.);
#31342=EDGE_CURVE('',#25284,#25281,#23541,.T.);
#31343=EDGE_CURVE('',#25285,#25283,#23542,.T.);
#31344=EDGE_CURVE('',#25285,#25286,#11269,.T.);
#31345=EDGE_CURVE('',#25286,#25284,#23543,.T.);
#31346=EDGE_CURVE('',#25287,#25285,#23544,.T.);
#31347=EDGE_CURVE('',#25287,#25288,#11270,.T.);
#31348=EDGE_CURVE('',#25288,#25286,#23545,.T.);
#31349=EDGE_CURVE('',#25289,#25287,#23546,.T.);
#31350=EDGE_CURVE('',#25289,#25290,#11271,.T.);
#31351=EDGE_CURVE('',#25290,#25288,#23547,.T.);
#31352=EDGE_CURVE('',#25291,#25289,#23548,.T.);
#31353=EDGE_CURVE('',#25291,#25292,#11272,.T.);
#31354=EDGE_CURVE('',#25292,#25290,#23549,.T.);
#31355=EDGE_CURVE('',#25293,#25291,#23550,.T.);
#31356=EDGE_CURVE('',#25293,#25294,#11273,.T.);
#31357=EDGE_CURVE('',#25294,#25292,#23551,.T.);
#31358=EDGE_CURVE('',#25295,#25293,#23552,.T.);
#31359=EDGE_CURVE('',#25295,#25296,#11274,.T.);
#31360=EDGE_CURVE('',#25296,#25294,#23553,.T.);
#31361=EDGE_CURVE('',#25297,#25295,#23554,.T.);
#31362=EDGE_CURVE('',#25297,#25298,#11275,.T.);
#31363=EDGE_CURVE('',#25298,#25296,#23555,.T.);
#31364=EDGE_CURVE('',#25299,#25297,#11276,.T.);
#31365=EDGE_CURVE('',#25299,#25300,#11277,.T.);
#31366=EDGE_CURVE('',#25300,#25298,#11278,.T.);
#31367=EDGE_CURVE('',#25301,#25299,#23556,.T.);
#31368=EDGE_CURVE('',#25301,#25302,#11279,.T.);
#31369=EDGE_CURVE('',#25302,#25300,#23557,.T.);
#31370=EDGE_CURVE('',#25303,#25301,#23558,.T.);
#31371=EDGE_CURVE('',#25303,#25304,#11280,.T.);
#31372=EDGE_CURVE('',#25304,#25302,#23559,.T.);
#31373=EDGE_CURVE('',#25305,#25303,#23560,.T.);
#31374=EDGE_CURVE('',#25305,#25306,#11281,.T.);
#31375=EDGE_CURVE('',#25306,#25304,#23561,.T.);
#31376=EDGE_CURVE('',#25307,#25305,#23562,.T.);
#31377=EDGE_CURVE('',#25307,#25308,#11282,.T.);
#31378=EDGE_CURVE('',#25308,#25306,#23563,.T.);
#31379=EDGE_CURVE('',#25309,#25307,#23564,.T.);
#31380=EDGE_CURVE('',#25309,#25310,#11283,.T.);
#31381=EDGE_CURVE('',#25310,#25308,#23565,.T.);
#31382=EDGE_CURVE('',#25311,#25309,#23566,.T.);
#31383=EDGE_CURVE('',#25311,#25312,#11284,.T.);
#31384=EDGE_CURVE('',#25312,#25310,#23567,.T.);
#31385=EDGE_CURVE('',#25313,#25311,#23568,.T.);
#31386=EDGE_CURVE('',#25313,#25314,#11285,.T.);
#31387=EDGE_CURVE('',#25314,#25312,#23569,.T.);
#31388=EDGE_CURVE('',#25315,#25313,#23570,.T.);
#31389=EDGE_CURVE('',#25315,#25316,#11286,.T.);
#31390=EDGE_CURVE('',#25316,#25314,#23571,.T.);
#31391=EDGE_CURVE('',#25317,#25315,#23572,.T.);
#31392=EDGE_CURVE('',#25317,#25318,#11287,.T.);
#31393=EDGE_CURVE('',#25318,#25316,#23573,.T.);
#31394=EDGE_CURVE('',#25319,#25317,#11288,.T.);
#31395=EDGE_CURVE('',#25319,#25320,#11289,.T.);
#31396=EDGE_CURVE('',#25320,#25318,#11290,.T.);
#31397=EDGE_CURVE('',#25321,#25319,#11291,.T.);
#31398=EDGE_CURVE('',#25321,#25322,#11292,.T.);
#31399=EDGE_CURVE('',#25322,#25320,#11293,.T.);
#31400=EDGE_CURVE('',#25280,#25321,#11294,.T.);
#31401=EDGE_CURVE('',#25282,#25322,#11295,.T.);
#31402=EDGE_CURVE('',#25323,#25324,#23574,.T.);
#31403=EDGE_CURVE('',#25323,#25325,#11296,.T.);
#31404=EDGE_CURVE('',#25325,#25326,#23575,.T.);
#31405=EDGE_CURVE('',#25324,#25326,#11297,.T.);
#31406=EDGE_CURVE('',#25327,#25323,#23576,.T.);
#31407=EDGE_CURVE('',#25327,#25328,#11298,.T.);
#31408=EDGE_CURVE('',#25328,#25325,#23577,.T.);
#31409=EDGE_CURVE('',#25329,#25327,#23578,.T.);
#31410=EDGE_CURVE('',#25329,#25330,#11299,.T.);
#31411=EDGE_CURVE('',#25330,#25328,#23579,.T.);
#31412=EDGE_CURVE('',#25331,#25329,#23580,.T.);
#31413=EDGE_CURVE('',#25331,#25332,#11300,.T.);
#31414=EDGE_CURVE('',#25332,#25330,#23581,.T.);
#31415=EDGE_CURVE('',#25333,#25331,#23582,.T.);
#31416=EDGE_CURVE('',#25333,#25334,#11301,.T.);
#31417=EDGE_CURVE('',#25334,#25332,#23583,.T.);
#31418=EDGE_CURVE('',#25335,#25333,#23584,.T.);
#31419=EDGE_CURVE('',#25335,#25336,#11302,.T.);
#31420=EDGE_CURVE('',#25336,#25334,#23585,.T.);
#31421=EDGE_CURVE('',#25337,#25335,#23586,.T.);
#31422=EDGE_CURVE('',#25337,#25338,#11303,.T.);
#31423=EDGE_CURVE('',#25338,#25336,#23587,.T.);
#31424=EDGE_CURVE('',#25324,#25337,#23588,.T.);
#31425=EDGE_CURVE('',#25326,#25338,#23589,.T.);
#31426=EDGE_CURVE('',#25339,#25340,#23590,.T.);
#31427=EDGE_CURVE('',#25339,#25341,#11304,.T.);
#31428=EDGE_CURVE('',#25341,#25342,#23591,.T.);
#31429=EDGE_CURVE('',#25340,#25342,#11305,.T.);
#31430=EDGE_CURVE('',#25343,#25339,#23592,.T.);
#31431=EDGE_CURVE('',#25343,#25344,#11306,.T.);
#31432=EDGE_CURVE('',#25344,#25341,#23593,.T.);
#31433=EDGE_CURVE('',#25345,#25343,#23594,.T.);
#31434=EDGE_CURVE('',#25345,#25346,#11307,.T.);
#31435=EDGE_CURVE('',#25346,#25344,#23595,.T.);
#31436=EDGE_CURVE('',#25347,#25345,#23596,.T.);
#31437=EDGE_CURVE('',#25347,#25348,#11308,.T.);
#31438=EDGE_CURVE('',#25348,#25346,#23597,.T.);
#31439=EDGE_CURVE('',#25349,#25347,#23598,.T.);
#31440=EDGE_CURVE('',#25349,#25350,#11309,.T.);
#31441=EDGE_CURVE('',#25350,#25348,#23599,.T.);
#31442=EDGE_CURVE('',#25351,#25349,#23600,.T.);
#31443=EDGE_CURVE('',#25351,#25352,#11310,.T.);
#31444=EDGE_CURVE('',#25352,#25350,#23601,.T.);
#31445=EDGE_CURVE('',#25353,#25351,#23602,.T.);
#31446=EDGE_CURVE('',#25353,#25354,#11311,.T.);
#31447=EDGE_CURVE('',#25354,#25352,#23603,.T.);
#31448=EDGE_CURVE('',#25355,#25353,#23604,.T.);
#31449=EDGE_CURVE('',#25355,#25356,#11312,.T.);
#31450=EDGE_CURVE('',#25356,#25354,#23605,.T.);
#31451=EDGE_CURVE('',#25357,#25355,#23606,.T.);
#31452=EDGE_CURVE('',#25357,#25358,#11313,.T.);
#31453=EDGE_CURVE('',#25358,#25356,#23607,.T.);
#31454=EDGE_CURVE('',#25359,#25357,#23608,.T.);
#31455=EDGE_CURVE('',#25359,#25360,#11314,.T.);
#31456=EDGE_CURVE('',#25360,#25358,#23609,.T.);
#31457=EDGE_CURVE('',#25361,#25359,#23610,.T.);
#31458=EDGE_CURVE('',#25361,#25362,#11315,.T.);
#31459=EDGE_CURVE('',#25362,#25360,#23611,.T.);
#31460=EDGE_CURVE('',#25340,#25361,#23612,.T.);
#31461=EDGE_CURVE('',#25342,#25362,#23613,.T.);
#31462=EDGE_CURVE('',#25363,#25364,#11316,.T.);
#31463=EDGE_CURVE('',#25363,#25365,#11317,.T.);
#31464=EDGE_CURVE('',#25365,#25366,#11318,.T.);
#31465=EDGE_CURVE('',#25364,#25366,#11319,.T.);
#31466=EDGE_CURVE('',#25367,#25363,#23614,.T.);
#31467=EDGE_CURVE('',#25367,#25368,#11320,.T.);
#31468=EDGE_CURVE('',#25368,#25365,#23615,.T.);
#31469=EDGE_CURVE('',#25369,#25367,#23616,.T.);
#31470=EDGE_CURVE('',#25369,#25370,#11321,.T.);
#31471=EDGE_CURVE('',#25370,#25368,#23617,.T.);
#31472=EDGE_CURVE('',#25371,#25369,#11322,.T.);
#31473=EDGE_CURVE('',#25371,#25372,#11323,.T.);
#31474=EDGE_CURVE('',#25372,#25370,#11324,.T.);
#31475=EDGE_CURVE('',#25373,#25371,#23618,.T.);
#31476=EDGE_CURVE('',#25373,#25374,#11325,.T.);
#31477=EDGE_CURVE('',#25374,#25372,#23619,.T.);
#31478=EDGE_CURVE('',#25375,#25373,#23620,.T.);
#31479=EDGE_CURVE('',#25375,#25376,#11326,.T.);
#31480=EDGE_CURVE('',#25376,#25374,#23621,.T.);
#31481=EDGE_CURVE('',#25377,#25375,#11327,.T.);
#31482=EDGE_CURVE('',#25377,#25378,#11328,.T.);
#31483=EDGE_CURVE('',#25378,#25376,#11329,.T.);
#31484=EDGE_CURVE('',#25379,#25377,#11330,.T.);
#31485=EDGE_CURVE('',#25379,#25380,#11331,.T.);
#31486=EDGE_CURVE('',#25380,#25378,#11332,.T.);
#31487=EDGE_CURVE('',#25364,#25379,#11333,.T.);
#31488=EDGE_CURVE('',#25366,#25380,#11334,.T.);
#31489=EDGE_CURVE('',#25381,#25382,#23622,.T.);
#31490=EDGE_CURVE('',#25381,#25383,#11335,.T.);
#31491=EDGE_CURVE('',#25383,#25384,#23623,.T.);
#31492=EDGE_CURVE('',#25382,#25384,#11336,.T.);
#31493=EDGE_CURVE('',#25385,#25381,#23624,.T.);
#31494=EDGE_CURVE('',#25385,#25386,#11337,.T.);
#31495=EDGE_CURVE('',#25386,#25383,#23625,.T.);
#31496=EDGE_CURVE('',#25387,#25385,#23626,.T.);
#31497=EDGE_CURVE('',#25387,#25388,#11338,.T.);
#31498=EDGE_CURVE('',#25388,#25386,#23627,.T.);
#31499=EDGE_CURVE('',#25389,#25387,#23628,.T.);
#31500=EDGE_CURVE('',#25389,#25390,#11339,.T.);
#31501=EDGE_CURVE('',#25390,#25388,#23629,.T.);
#31502=EDGE_CURVE('',#25391,#25389,#23630,.T.);
#31503=EDGE_CURVE('',#25391,#25392,#11340,.T.);
#31504=EDGE_CURVE('',#25392,#25390,#23631,.T.);
#31505=EDGE_CURVE('',#25393,#25391,#23632,.T.);
#31506=EDGE_CURVE('',#25393,#25394,#11341,.T.);
#31507=EDGE_CURVE('',#25394,#25392,#23633,.T.);
#31508=EDGE_CURVE('',#25395,#25393,#23634,.T.);
#31509=EDGE_CURVE('',#25395,#25396,#11342,.T.);
#31510=EDGE_CURVE('',#25396,#25394,#23635,.T.);
#31511=EDGE_CURVE('',#25382,#25395,#23636,.T.);
#31512=EDGE_CURVE('',#25384,#25396,#23637,.T.);
#31513=EDGE_CURVE('',#25397,#25398,#23638,.T.);
#31514=EDGE_CURVE('',#25397,#25399,#11343,.T.);
#31515=EDGE_CURVE('',#25399,#25400,#23639,.T.);
#31516=EDGE_CURVE('',#25398,#25400,#11344,.T.);
#31517=EDGE_CURVE('',#25401,#25397,#23640,.T.);
#31518=EDGE_CURVE('',#25401,#25402,#11345,.T.);
#31519=EDGE_CURVE('',#25402,#25399,#23641,.T.);
#31520=EDGE_CURVE('',#25403,#25401,#23642,.T.);
#31521=EDGE_CURVE('',#25403,#25404,#11346,.T.);
#31522=EDGE_CURVE('',#25404,#25402,#23643,.T.);
#31523=EDGE_CURVE('',#25405,#25403,#23644,.T.);
#31524=EDGE_CURVE('',#25405,#25406,#11347,.T.);
#31525=EDGE_CURVE('',#25406,#25404,#23645,.T.);
#31526=EDGE_CURVE('',#25407,#25405,#23646,.T.);
#31527=EDGE_CURVE('',#25407,#25408,#11348,.T.);
#31528=EDGE_CURVE('',#25408,#25406,#23647,.T.);
#31529=EDGE_CURVE('',#25409,#25407,#23648,.T.);
#31530=EDGE_CURVE('',#25409,#25410,#11349,.T.);
#31531=EDGE_CURVE('',#25410,#25408,#23649,.T.);
#31532=EDGE_CURVE('',#25411,#25409,#23650,.T.);
#31533=EDGE_CURVE('',#25411,#25412,#11350,.T.);
#31534=EDGE_CURVE('',#25412,#25410,#23651,.T.);
#31535=EDGE_CURVE('',#25413,#25411,#23652,.T.);
#31536=EDGE_CURVE('',#25413,#25414,#11351,.T.);
#31537=EDGE_CURVE('',#25414,#25412,#23653,.T.);
#31538=EDGE_CURVE('',#25415,#25413,#23654,.T.);
#31539=EDGE_CURVE('',#25415,#25416,#11352,.T.);
#31540=EDGE_CURVE('',#25416,#25414,#23655,.T.);
#31541=EDGE_CURVE('',#25417,#25415,#23656,.T.);
#31542=EDGE_CURVE('',#25417,#25418,#11353,.T.);
#31543=EDGE_CURVE('',#25418,#25416,#23657,.T.);
#31544=EDGE_CURVE('',#25419,#25417,#23658,.T.);
#31545=EDGE_CURVE('',#25419,#25420,#11354,.T.);
#31546=EDGE_CURVE('',#25420,#25418,#23659,.T.);
#31547=EDGE_CURVE('',#25398,#25419,#23660,.T.);
#31548=EDGE_CURVE('',#25400,#25420,#23661,.T.);
#31549=EDGE_CURVE('',#25421,#25422,#23662,.T.);
#31550=EDGE_CURVE('',#25421,#25423,#11355,.T.);
#31551=EDGE_CURVE('',#25423,#25424,#23663,.T.);
#31552=EDGE_CURVE('',#25422,#25424,#11356,.T.);
#31553=EDGE_CURVE('',#25425,#25421,#23664,.T.);
#31554=EDGE_CURVE('',#25425,#25426,#11357,.T.);
#31555=EDGE_CURVE('',#25426,#25423,#23665,.T.);
#31556=EDGE_CURVE('',#25427,#25425,#23666,.T.);
#31557=EDGE_CURVE('',#25427,#25428,#11358,.T.);
#31558=EDGE_CURVE('',#25428,#25426,#23667,.T.);
#31559=EDGE_CURVE('',#25429,#25427,#23668,.T.);
#31560=EDGE_CURVE('',#25429,#25430,#11359,.T.);
#31561=EDGE_CURVE('',#25430,#25428,#23669,.T.);
#31562=EDGE_CURVE('',#25431,#25429,#23670,.T.);
#31563=EDGE_CURVE('',#25431,#25432,#11360,.T.);
#31564=EDGE_CURVE('',#25432,#25430,#23671,.T.);
#31565=EDGE_CURVE('',#25433,#25431,#23672,.T.);
#31566=EDGE_CURVE('',#25433,#25434,#11361,.T.);
#31567=EDGE_CURVE('',#25434,#25432,#23673,.T.);
#31568=EDGE_CURVE('',#25435,#25433,#23674,.T.);
#31569=EDGE_CURVE('',#25435,#25436,#11362,.T.);
#31570=EDGE_CURVE('',#25436,#25434,#23675,.T.);
#31571=EDGE_CURVE('',#25422,#25435,#23676,.T.);
#31572=EDGE_CURVE('',#25424,#25436,#23677,.T.);
#31573=EDGE_CURVE('',#25437,#25438,#23678,.T.);
#31574=EDGE_CURVE('',#25437,#25439,#11363,.T.);
#31575=EDGE_CURVE('',#25439,#25440,#23679,.T.);
#31576=EDGE_CURVE('',#25438,#25440,#11364,.T.);
#31577=EDGE_CURVE('',#25441,#25437,#23680,.T.);
#31578=EDGE_CURVE('',#25441,#25442,#11365,.T.);
#31579=EDGE_CURVE('',#25442,#25439,#23681,.T.);
#31580=EDGE_CURVE('',#25443,#25441,#23682,.T.);
#31581=EDGE_CURVE('',#25443,#25444,#11366,.T.);
#31582=EDGE_CURVE('',#25444,#25442,#23683,.T.);
#31583=EDGE_CURVE('',#25445,#25443,#23684,.T.);
#31584=EDGE_CURVE('',#25445,#25446,#11367,.T.);
#31585=EDGE_CURVE('',#25446,#25444,#23685,.T.);
#31586=EDGE_CURVE('',#25447,#25445,#23686,.T.);
#31587=EDGE_CURVE('',#25447,#25448,#11368,.T.);
#31588=EDGE_CURVE('',#25448,#25446,#23687,.T.);
#31589=EDGE_CURVE('',#25449,#25447,#23688,.T.);
#31590=EDGE_CURVE('',#25449,#25450,#11369,.T.);
#31591=EDGE_CURVE('',#25450,#25448,#23689,.T.);
#31592=EDGE_CURVE('',#25451,#25449,#23690,.T.);
#31593=EDGE_CURVE('',#25451,#25452,#11370,.T.);
#31594=EDGE_CURVE('',#25452,#25450,#23691,.T.);
#31595=EDGE_CURVE('',#25453,#25451,#23692,.T.);
#31596=EDGE_CURVE('',#25453,#25454,#11371,.T.);
#31597=EDGE_CURVE('',#25454,#25452,#23693,.T.);
#31598=EDGE_CURVE('',#25455,#25453,#23694,.T.);
#31599=EDGE_CURVE('',#25455,#25456,#11372,.T.);
#31600=EDGE_CURVE('',#25456,#25454,#23695,.T.);
#31601=EDGE_CURVE('',#25457,#25455,#23696,.T.);
#31602=EDGE_CURVE('',#25457,#25458,#11373,.T.);
#31603=EDGE_CURVE('',#25458,#25456,#23697,.T.);
#31604=EDGE_CURVE('',#25459,#25457,#23698,.T.);
#31605=EDGE_CURVE('',#25459,#25460,#11374,.T.);
#31606=EDGE_CURVE('',#25460,#25458,#23699,.T.);
#31607=EDGE_CURVE('',#25438,#25459,#23700,.T.);
#31608=EDGE_CURVE('',#25440,#25460,#23701,.T.);
#31609=EDGE_CURVE('',#25461,#25462,#11375,.T.);
#31610=EDGE_CURVE('',#25461,#25463,#11376,.T.);
#31611=EDGE_CURVE('',#25463,#25464,#11377,.T.);
#31612=EDGE_CURVE('',#25462,#25464,#11378,.T.);
#31613=EDGE_CURVE('',#25465,#25461,#23702,.T.);
#31614=EDGE_CURVE('',#25465,#25466,#11379,.T.);
#31615=EDGE_CURVE('',#25466,#25463,#23703,.T.);
#31616=EDGE_CURVE('',#25467,#25465,#23704,.T.);
#31617=EDGE_CURVE('',#25467,#25468,#11380,.T.);
#31618=EDGE_CURVE('',#25468,#25466,#23705,.T.);
#31619=EDGE_CURVE('',#25469,#25467,#11381,.T.);
#31620=EDGE_CURVE('',#25469,#25470,#11382,.T.);
#31621=EDGE_CURVE('',#25470,#25468,#11383,.T.);
#31622=EDGE_CURVE('',#25471,#25469,#23706,.T.);
#31623=EDGE_CURVE('',#25471,#25472,#11384,.T.);
#31624=EDGE_CURVE('',#25472,#25470,#23707,.T.);
#31625=EDGE_CURVE('',#25473,#25471,#23708,.T.);
#31626=EDGE_CURVE('',#25473,#25474,#11385,.T.);
#31627=EDGE_CURVE('',#25474,#25472,#23709,.T.);
#31628=EDGE_CURVE('',#25475,#25473,#11386,.T.);
#31629=EDGE_CURVE('',#25475,#25476,#11387,.T.);
#31630=EDGE_CURVE('',#25476,#25474,#11388,.T.);
#31631=EDGE_CURVE('',#25477,#25475,#11389,.T.);
#31632=EDGE_CURVE('',#25477,#25478,#11390,.T.);
#31633=EDGE_CURVE('',#25478,#25476,#11391,.T.);
#31634=EDGE_CURVE('',#25462,#25477,#11392,.T.);
#31635=EDGE_CURVE('',#25464,#25478,#11393,.T.);
#31636=EDGE_CURVE('',#25479,#25480,#23710,.T.);
#31637=EDGE_CURVE('',#25479,#25481,#11394,.T.);
#31638=EDGE_CURVE('',#25481,#25482,#23711,.T.);
#31639=EDGE_CURVE('',#25480,#25482,#11395,.T.);
#31640=EDGE_CURVE('',#25483,#25479,#23712,.T.);
#31641=EDGE_CURVE('',#25483,#25484,#11396,.T.);
#31642=EDGE_CURVE('',#25484,#25481,#23713,.T.);
#31643=EDGE_CURVE('',#25485,#25483,#23714,.T.);
#31644=EDGE_CURVE('',#25485,#25486,#11397,.T.);
#31645=EDGE_CURVE('',#25486,#25484,#23715,.T.);
#31646=EDGE_CURVE('',#25487,#25485,#23716,.T.);
#31647=EDGE_CURVE('',#25487,#25488,#11398,.T.);
#31648=EDGE_CURVE('',#25488,#25486,#23717,.T.);
#31649=EDGE_CURVE('',#25489,#25487,#23718,.T.);
#31650=EDGE_CURVE('',#25489,#25490,#11399,.T.);
#31651=EDGE_CURVE('',#25490,#25488,#23719,.T.);
#31652=EDGE_CURVE('',#25491,#25489,#23720,.T.);
#31653=EDGE_CURVE('',#25491,#25492,#11400,.T.);
#31654=EDGE_CURVE('',#25492,#25490,#23721,.T.);
#31655=EDGE_CURVE('',#25493,#25491,#23722,.T.);
#31656=EDGE_CURVE('',#25493,#25494,#11401,.T.);
#31657=EDGE_CURVE('',#25494,#25492,#23723,.T.);
#31658=EDGE_CURVE('',#25480,#25493,#23724,.T.);
#31659=EDGE_CURVE('',#25482,#25494,#23725,.T.);
#31660=EDGE_CURVE('',#25495,#25496,#23726,.T.);
#31661=EDGE_CURVE('',#25495,#25497,#11402,.T.);
#31662=EDGE_CURVE('',#25497,#25498,#23727,.T.);
#31663=EDGE_CURVE('',#25496,#25498,#11403,.T.);
#31664=EDGE_CURVE('',#25499,#25495,#23728,.T.);
#31665=EDGE_CURVE('',#25499,#25500,#11404,.T.);
#31666=EDGE_CURVE('',#25500,#25497,#23729,.T.);
#31667=EDGE_CURVE('',#25501,#25499,#23730,.T.);
#31668=EDGE_CURVE('',#25501,#25502,#11405,.T.);
#31669=EDGE_CURVE('',#25502,#25500,#23731,.T.);
#31670=EDGE_CURVE('',#25503,#25501,#23732,.T.);
#31671=EDGE_CURVE('',#25503,#25504,#11406,.T.);
#31672=EDGE_CURVE('',#25504,#25502,#23733,.T.);
#31673=EDGE_CURVE('',#25505,#25503,#23734,.T.);
#31674=EDGE_CURVE('',#25505,#25506,#11407,.T.);
#31675=EDGE_CURVE('',#25506,#25504,#23735,.T.);
#31676=EDGE_CURVE('',#25507,#25505,#23736,.T.);
#31677=EDGE_CURVE('',#25507,#25508,#11408,.T.);
#31678=EDGE_CURVE('',#25508,#25506,#23737,.T.);
#31679=EDGE_CURVE('',#25509,#25507,#23738,.T.);
#31680=EDGE_CURVE('',#25509,#25510,#11409,.T.);
#31681=EDGE_CURVE('',#25510,#25508,#23739,.T.);
#31682=EDGE_CURVE('',#25511,#25509,#23740,.T.);
#31683=EDGE_CURVE('',#25511,#25512,#11410,.T.);
#31684=EDGE_CURVE('',#25512,#25510,#23741,.T.);
#31685=EDGE_CURVE('',#25513,#25511,#23742,.T.);
#31686=EDGE_CURVE('',#25513,#25514,#11411,.T.);
#31687=EDGE_CURVE('',#25514,#25512,#23743,.T.);
#31688=EDGE_CURVE('',#25515,#25513,#23744,.T.);
#31689=EDGE_CURVE('',#25515,#25516,#11412,.T.);
#31690=EDGE_CURVE('',#25516,#25514,#23745,.T.);
#31691=EDGE_CURVE('',#25517,#25515,#23746,.T.);
#31692=EDGE_CURVE('',#25517,#25518,#11413,.T.);
#31693=EDGE_CURVE('',#25518,#25516,#23747,.T.);
#31694=EDGE_CURVE('',#25496,#25517,#23748,.T.);
#31695=EDGE_CURVE('',#25498,#25518,#23749,.T.);
#31696=EDGE_CURVE('',#25519,#25520,#23750,.T.);
#31697=EDGE_CURVE('',#25519,#25521,#11414,.T.);
#31698=EDGE_CURVE('',#25521,#25522,#23751,.T.);
#31699=EDGE_CURVE('',#25520,#25522,#11415,.T.);
#31700=EDGE_CURVE('',#25523,#25519,#23752,.T.);
#31701=EDGE_CURVE('',#25523,#25524,#11416,.T.);
#31702=EDGE_CURVE('',#25524,#25521,#23753,.T.);
#31703=EDGE_CURVE('',#25525,#25523,#23754,.T.);
#31704=EDGE_CURVE('',#25525,#25526,#11417,.T.);
#31705=EDGE_CURVE('',#25526,#25524,#23755,.T.);
#31706=EDGE_CURVE('',#25527,#25525,#23756,.T.);
#31707=EDGE_CURVE('',#25527,#25528,#11418,.T.);
#31708=EDGE_CURVE('',#25528,#25526,#23757,.T.);
#31709=EDGE_CURVE('',#25529,#25527,#23758,.T.);
#31710=EDGE_CURVE('',#25529,#25530,#11419,.T.);
#31711=EDGE_CURVE('',#25530,#25528,#23759,.T.);
#31712=EDGE_CURVE('',#25531,#25529,#23760,.T.);
#31713=EDGE_CURVE('',#25531,#25532,#11420,.T.);
#31714=EDGE_CURVE('',#25532,#25530,#23761,.T.);
#31715=EDGE_CURVE('',#25533,#25531,#23762,.T.);
#31716=EDGE_CURVE('',#25533,#25534,#11421,.T.);
#31717=EDGE_CURVE('',#25534,#25532,#23763,.T.);
#31718=EDGE_CURVE('',#25535,#25533,#23764,.T.);
#31719=EDGE_CURVE('',#25535,#25536,#11422,.T.);
#31720=EDGE_CURVE('',#25536,#25534,#23765,.T.);
#31721=EDGE_CURVE('',#25537,#25535,#23766,.T.);
#31722=EDGE_CURVE('',#25537,#25538,#11423,.T.);
#31723=EDGE_CURVE('',#25538,#25536,#23767,.T.);
#31724=EDGE_CURVE('',#25539,#25537,#11424,.T.);
#31725=EDGE_CURVE('',#25539,#25540,#11425,.T.);
#31726=EDGE_CURVE('',#25540,#25538,#11426,.T.);
#31727=EDGE_CURVE('',#25541,#25539,#23768,.T.);
#31728=EDGE_CURVE('',#25541,#25542,#11427,.T.);
#31729=EDGE_CURVE('',#25542,#25540,#23769,.T.);
#31730=EDGE_CURVE('',#25543,#25541,#23770,.T.);
#31731=EDGE_CURVE('',#25543,#25544,#11428,.T.);
#31732=EDGE_CURVE('',#25544,#25542,#23771,.T.);
#31733=EDGE_CURVE('',#25545,#25543,#23772,.T.);
#31734=EDGE_CURVE('',#25545,#25546,#11429,.T.);
#31735=EDGE_CURVE('',#25546,#25544,#23773,.T.);
#31736=EDGE_CURVE('',#25547,#25545,#23774,.T.);
#31737=EDGE_CURVE('',#25547,#25548,#11430,.T.);
#31738=EDGE_CURVE('',#25548,#25546,#23775,.T.);
#31739=EDGE_CURVE('',#25549,#25547,#23776,.T.);
#31740=EDGE_CURVE('',#25549,#25550,#11431,.T.);
#31741=EDGE_CURVE('',#25550,#25548,#23777,.T.);
#31742=EDGE_CURVE('',#25551,#25549,#23778,.T.);
#31743=EDGE_CURVE('',#25551,#25552,#11432,.T.);
#31744=EDGE_CURVE('',#25552,#25550,#23779,.T.);
#31745=EDGE_CURVE('',#25553,#25551,#23780,.T.);
#31746=EDGE_CURVE('',#25553,#25554,#11433,.T.);
#31747=EDGE_CURVE('',#25554,#25552,#23781,.T.);
#31748=EDGE_CURVE('',#25555,#25553,#23782,.T.);
#31749=EDGE_CURVE('',#25555,#25556,#11434,.T.);
#31750=EDGE_CURVE('',#25556,#25554,#23783,.T.);
#31751=EDGE_CURVE('',#25557,#25555,#23784,.T.);
#31752=EDGE_CURVE('',#25557,#25558,#11435,.T.);
#31753=EDGE_CURVE('',#25558,#25556,#23785,.T.);
#31754=EDGE_CURVE('',#25559,#25557,#11436,.T.);
#31755=EDGE_CURVE('',#25559,#25560,#11437,.T.);
#31756=EDGE_CURVE('',#25560,#25558,#11438,.T.);
#31757=EDGE_CURVE('',#25561,#25559,#11439,.T.);
#31758=EDGE_CURVE('',#25561,#25562,#11440,.T.);
#31759=EDGE_CURVE('',#25562,#25560,#11441,.T.);
#31760=EDGE_CURVE('',#25520,#25561,#11442,.T.);
#31761=EDGE_CURVE('',#25522,#25562,#11443,.T.);
#31762=EDGE_CURVE('',#25563,#25564,#23786,.T.);
#31763=EDGE_CURVE('',#25563,#25565,#11444,.T.);
#31764=EDGE_CURVE('',#25565,#25566,#23787,.T.);
#31765=EDGE_CURVE('',#25564,#25566,#11445,.T.);
#31766=EDGE_CURVE('',#25567,#25563,#23788,.T.);
#31767=EDGE_CURVE('',#25567,#25568,#11446,.T.);
#31768=EDGE_CURVE('',#25568,#25565,#23789,.T.);
#31769=EDGE_CURVE('',#25569,#25567,#23790,.T.);
#31770=EDGE_CURVE('',#25569,#25570,#11447,.T.);
#31771=EDGE_CURVE('',#25570,#25568,#23791,.T.);
#31772=EDGE_CURVE('',#25571,#25569,#23792,.T.);
#31773=EDGE_CURVE('',#25571,#25572,#11448,.T.);
#31774=EDGE_CURVE('',#25572,#25570,#23793,.T.);
#31775=EDGE_CURVE('',#25573,#25571,#23794,.T.);
#31776=EDGE_CURVE('',#25573,#25574,#11449,.T.);
#31777=EDGE_CURVE('',#25574,#25572,#23795,.T.);
#31778=EDGE_CURVE('',#25575,#25573,#23796,.T.);
#31779=EDGE_CURVE('',#25575,#25576,#11450,.T.);
#31780=EDGE_CURVE('',#25576,#25574,#23797,.T.);
#31781=EDGE_CURVE('',#25577,#25575,#23798,.T.);
#31782=EDGE_CURVE('',#25577,#25578,#11451,.T.);
#31783=EDGE_CURVE('',#25578,#25576,#23799,.T.);
#31784=EDGE_CURVE('',#25564,#25577,#23800,.T.);
#31785=EDGE_CURVE('',#25566,#25578,#23801,.T.);
#31786=EDGE_CURVE('',#25579,#25580,#23802,.T.);
#31787=EDGE_CURVE('',#25579,#25581,#11452,.T.);
#31788=EDGE_CURVE('',#25581,#25582,#23803,.T.);
#31789=EDGE_CURVE('',#25580,#25582,#11453,.T.);
#31790=EDGE_CURVE('',#25583,#25579,#23804,.T.);
#31791=EDGE_CURVE('',#25583,#25584,#11454,.T.);
#31792=EDGE_CURVE('',#25584,#25581,#23805,.T.);
#31793=EDGE_CURVE('',#25585,#25583,#23806,.T.);
#31794=EDGE_CURVE('',#25585,#25586,#11455,.T.);
#31795=EDGE_CURVE('',#25586,#25584,#23807,.T.);
#31796=EDGE_CURVE('',#25587,#25585,#23808,.T.);
#31797=EDGE_CURVE('',#25587,#25588,#11456,.T.);
#31798=EDGE_CURVE('',#25588,#25586,#23809,.T.);
#31799=EDGE_CURVE('',#25589,#25587,#23810,.T.);
#31800=EDGE_CURVE('',#25589,#25590,#11457,.T.);
#31801=EDGE_CURVE('',#25590,#25588,#23811,.T.);
#31802=EDGE_CURVE('',#25591,#25589,#23812,.T.);
#31803=EDGE_CURVE('',#25591,#25592,#11458,.T.);
#31804=EDGE_CURVE('',#25592,#25590,#23813,.T.);
#31805=EDGE_CURVE('',#25593,#25591,#23814,.T.);
#31806=EDGE_CURVE('',#25593,#25594,#11459,.T.);
#31807=EDGE_CURVE('',#25594,#25592,#23815,.T.);
#31808=EDGE_CURVE('',#25595,#25593,#23816,.T.);
#31809=EDGE_CURVE('',#25595,#25596,#11460,.T.);
#31810=EDGE_CURVE('',#25596,#25594,#23817,.T.);
#31811=EDGE_CURVE('',#25597,#25595,#23818,.T.);
#31812=EDGE_CURVE('',#25597,#25598,#11461,.T.);
#31813=EDGE_CURVE('',#25598,#25596,#23819,.T.);
#31814=EDGE_CURVE('',#25599,#25597,#23820,.T.);
#31815=EDGE_CURVE('',#25599,#25600,#11462,.T.);
#31816=EDGE_CURVE('',#25600,#25598,#23821,.T.);
#31817=EDGE_CURVE('',#25601,#25599,#23822,.T.);
#31818=EDGE_CURVE('',#25601,#25602,#11463,.T.);
#31819=EDGE_CURVE('',#25602,#25600,#23823,.T.);
#31820=EDGE_CURVE('',#25580,#25601,#23824,.T.);
#31821=EDGE_CURVE('',#25582,#25602,#23825,.T.);
#31822=EDGE_CURVE('',#25603,#25604,#23826,.T.);
#31823=EDGE_CURVE('',#25603,#25605,#11464,.T.);
#31824=EDGE_CURVE('',#25605,#25606,#23827,.T.);
#31825=EDGE_CURVE('',#25604,#25606,#11465,.T.);
#31826=EDGE_CURVE('',#25607,#25603,#23828,.T.);
#31827=EDGE_CURVE('',#25607,#25608,#11466,.T.);
#31828=EDGE_CURVE('',#25608,#25605,#23829,.T.);
#31829=EDGE_CURVE('',#25609,#25607,#23830,.T.);
#31830=EDGE_CURVE('',#25609,#25610,#11467,.T.);
#31831=EDGE_CURVE('',#25610,#25608,#23831,.T.);
#31832=EDGE_CURVE('',#25611,#25609,#23832,.T.);
#31833=EDGE_CURVE('',#25611,#25612,#11468,.T.);
#31834=EDGE_CURVE('',#25612,#25610,#23833,.T.);
#31835=EDGE_CURVE('',#25613,#25611,#23834,.T.);
#31836=EDGE_CURVE('',#25613,#25614,#11469,.T.);
#31837=EDGE_CURVE('',#25614,#25612,#23835,.T.);
#31838=EDGE_CURVE('',#25615,#25613,#23836,.T.);
#31839=EDGE_CURVE('',#25615,#25616,#11470,.T.);
#31840=EDGE_CURVE('',#25616,#25614,#23837,.T.);
#31841=EDGE_CURVE('',#25617,#25615,#23838,.T.);
#31842=EDGE_CURVE('',#25617,#25618,#11471,.T.);
#31843=EDGE_CURVE('',#25618,#25616,#23839,.T.);
#31844=EDGE_CURVE('',#25619,#25617,#23840,.T.);
#31845=EDGE_CURVE('',#25619,#25620,#11472,.T.);
#31846=EDGE_CURVE('',#25620,#25618,#23841,.T.);
#31847=EDGE_CURVE('',#25621,#25619,#23842,.T.);
#31848=EDGE_CURVE('',#25621,#25622,#11473,.T.);
#31849=EDGE_CURVE('',#25622,#25620,#23843,.T.);
#31850=EDGE_CURVE('',#25623,#25621,#23844,.T.);
#31851=EDGE_CURVE('',#25623,#25624,#11474,.T.);
#31852=EDGE_CURVE('',#25624,#25622,#23845,.T.);
#31853=EDGE_CURVE('',#25625,#25623,#23846,.T.);
#31854=EDGE_CURVE('',#25625,#25626,#11475,.T.);
#31855=EDGE_CURVE('',#25626,#25624,#23847,.T.);
#31856=EDGE_CURVE('',#25627,#25625,#23848,.T.);
#31857=EDGE_CURVE('',#25627,#25628,#11476,.T.);
#31858=EDGE_CURVE('',#25628,#25626,#23849,.T.);
#31859=EDGE_CURVE('',#25629,#25627,#11477,.T.);
#31860=EDGE_CURVE('',#25629,#25630,#11478,.T.);
#31861=EDGE_CURVE('',#25630,#25628,#11479,.T.);
#31862=EDGE_CURVE('',#25631,#25629,#23850,.T.);
#31863=EDGE_CURVE('',#25631,#25632,#11480,.T.);
#31864=EDGE_CURVE('',#25632,#25630,#23851,.T.);
#31865=EDGE_CURVE('',#25633,#25631,#23852,.T.);
#31866=EDGE_CURVE('',#25633,#25634,#11481,.T.);
#31867=EDGE_CURVE('',#25634,#25632,#23853,.T.);
#31868=EDGE_CURVE('',#25635,#25633,#23854,.T.);
#31869=EDGE_CURVE('',#25635,#25636,#11482,.T.);
#31870=EDGE_CURVE('',#25636,#25634,#23855,.T.);
#31871=EDGE_CURVE('',#25637,#25635,#23856,.T.);
#31872=EDGE_CURVE('',#25637,#25638,#11483,.T.);
#31873=EDGE_CURVE('',#25638,#25636,#23857,.T.);
#31874=EDGE_CURVE('',#25639,#25637,#23858,.T.);
#31875=EDGE_CURVE('',#25639,#25640,#11484,.T.);
#31876=EDGE_CURVE('',#25640,#25638,#23859,.T.);
#31877=EDGE_CURVE('',#25641,#25639,#23860,.T.);
#31878=EDGE_CURVE('',#25641,#25642,#11485,.T.);
#31879=EDGE_CURVE('',#25642,#25640,#23861,.T.);
#31880=EDGE_CURVE('',#25643,#25641,#23862,.T.);
#31881=EDGE_CURVE('',#25643,#25644,#11486,.T.);
#31882=EDGE_CURVE('',#25644,#25642,#23863,.T.);
#31883=EDGE_CURVE('',#25645,#25643,#11487,.T.);
#31884=EDGE_CURVE('',#25645,#25646,#11488,.T.);
#31885=EDGE_CURVE('',#25646,#25644,#11489,.T.);
#31886=EDGE_CURVE('',#25647,#25645,#23864,.T.);
#31887=EDGE_CURVE('',#25647,#25648,#11490,.T.);
#31888=EDGE_CURVE('',#25648,#25646,#23865,.T.);
#31889=EDGE_CURVE('',#25649,#25647,#23866,.T.);
#31890=EDGE_CURVE('',#25649,#25650,#11491,.T.);
#31891=EDGE_CURVE('',#25650,#25648,#23867,.T.);
#31892=EDGE_CURVE('',#25651,#25649,#23868,.T.);
#31893=EDGE_CURVE('',#25651,#25652,#11492,.T.);
#31894=EDGE_CURVE('',#25652,#25650,#23869,.T.);
#31895=EDGE_CURVE('',#25653,#25651,#23870,.T.);
#31896=EDGE_CURVE('',#25653,#25654,#11493,.T.);
#31897=EDGE_CURVE('',#25654,#25652,#23871,.T.);
#31898=EDGE_CURVE('',#25655,#25653,#23872,.T.);
#31899=EDGE_CURVE('',#25655,#25656,#11494,.T.);
#31900=EDGE_CURVE('',#25656,#25654,#23873,.T.);
#31901=EDGE_CURVE('',#25657,#25655,#23874,.T.);
#31902=EDGE_CURVE('',#25657,#25658,#11495,.T.);
#31903=EDGE_CURVE('',#25658,#25656,#23875,.T.);
#31904=EDGE_CURVE('',#25659,#25657,#23876,.T.);
#31905=EDGE_CURVE('',#25659,#25660,#11496,.T.);
#31906=EDGE_CURVE('',#25660,#25658,#23877,.T.);
#31907=EDGE_CURVE('',#25661,#25659,#11497,.T.);
#31908=EDGE_CURVE('',#25661,#25662,#11498,.T.);
#31909=EDGE_CURVE('',#25662,#25660,#11499,.T.);
#31910=EDGE_CURVE('',#25604,#25661,#23878,.T.);
#31911=EDGE_CURVE('',#25606,#25662,#23879,.T.);
#31912=EDGE_CURVE('',#25663,#25664,#23880,.T.);
#31913=EDGE_CURVE('',#25663,#25665,#11500,.T.);
#31914=EDGE_CURVE('',#25665,#25666,#23881,.T.);
#31915=EDGE_CURVE('',#25664,#25666,#11501,.T.);
#31916=EDGE_CURVE('',#25667,#25663,#23882,.T.);
#31917=EDGE_CURVE('',#25667,#25668,#11502,.T.);
#31918=EDGE_CURVE('',#25668,#25665,#23883,.T.);
#31919=EDGE_CURVE('',#25669,#25667,#23884,.T.);
#31920=EDGE_CURVE('',#25669,#25670,#11503,.T.);
#31921=EDGE_CURVE('',#25670,#25668,#23885,.T.);
#31922=EDGE_CURVE('',#25671,#25669,#23886,.T.);
#31923=EDGE_CURVE('',#25671,#25672,#11504,.T.);
#31924=EDGE_CURVE('',#25672,#25670,#23887,.T.);
#31925=EDGE_CURVE('',#25673,#25671,#23888,.T.);
#31926=EDGE_CURVE('',#25673,#25674,#11505,.T.);
#31927=EDGE_CURVE('',#25674,#25672,#23889,.T.);
#31928=EDGE_CURVE('',#25675,#25673,#23890,.T.);
#31929=EDGE_CURVE('',#25675,#25676,#11506,.T.);
#31930=EDGE_CURVE('',#25676,#25674,#23891,.T.);
#31931=EDGE_CURVE('',#25677,#25675,#23892,.T.);
#31932=EDGE_CURVE('',#25677,#25678,#11507,.T.);
#31933=EDGE_CURVE('',#25678,#25676,#23893,.T.);
#31934=EDGE_CURVE('',#25664,#25677,#23894,.T.);
#31935=EDGE_CURVE('',#25666,#25678,#23895,.T.);
#31936=EDGE_CURVE('',#25679,#25680,#23896,.T.);
#31937=EDGE_CURVE('',#25679,#25681,#11508,.T.);
#31938=EDGE_CURVE('',#25681,#25682,#23897,.T.);
#31939=EDGE_CURVE('',#25680,#25682,#11509,.T.);
#31940=EDGE_CURVE('',#25683,#25679,#23898,.T.);
#31941=EDGE_CURVE('',#25683,#25684,#11510,.T.);
#31942=EDGE_CURVE('',#25684,#25681,#23899,.T.);
#31943=EDGE_CURVE('',#25685,#25683,#23900,.T.);
#31944=EDGE_CURVE('',#25685,#25686,#11511,.T.);
#31945=EDGE_CURVE('',#25686,#25684,#23901,.T.);
#31946=EDGE_CURVE('',#25687,#25685,#23902,.T.);
#31947=EDGE_CURVE('',#25687,#25688,#11512,.T.);
#31948=EDGE_CURVE('',#25688,#25686,#23903,.T.);
#31949=EDGE_CURVE('',#25689,#25687,#23904,.T.);
#31950=EDGE_CURVE('',#25689,#25690,#11513,.T.);
#31951=EDGE_CURVE('',#25690,#25688,#23905,.T.);
#31952=EDGE_CURVE('',#25691,#25689,#23906,.T.);
#31953=EDGE_CURVE('',#25691,#25692,#11514,.T.);
#31954=EDGE_CURVE('',#25692,#25690,#23907,.T.);
#31955=EDGE_CURVE('',#25693,#25691,#23908,.T.);
#31956=EDGE_CURVE('',#25693,#25694,#11515,.T.);
#31957=EDGE_CURVE('',#25694,#25692,#23909,.T.);
#31958=EDGE_CURVE('',#25695,#25693,#23910,.T.);
#31959=EDGE_CURVE('',#25695,#25696,#11516,.T.);
#31960=EDGE_CURVE('',#25696,#25694,#23911,.T.);
#31961=EDGE_CURVE('',#25697,#25695,#23912,.T.);
#31962=EDGE_CURVE('',#25697,#25698,#11517,.T.);
#31963=EDGE_CURVE('',#25698,#25696,#23913,.T.);
#31964=EDGE_CURVE('',#25699,#25697,#23914,.T.);
#31965=EDGE_CURVE('',#25699,#25700,#11518,.T.);
#31966=EDGE_CURVE('',#25700,#25698,#23915,.T.);
#31967=EDGE_CURVE('',#25701,#25699,#23916,.T.);
#31968=EDGE_CURVE('',#25701,#25702,#11519,.T.);
#31969=EDGE_CURVE('',#25702,#25700,#23917,.T.);
#31970=EDGE_CURVE('',#25680,#25701,#23918,.T.);
#31971=EDGE_CURVE('',#25682,#25702,#23919,.T.);
#31972=EDGE_CURVE('',#25703,#25704,#11520,.T.);
#31973=EDGE_CURVE('',#25703,#25705,#11521,.T.);
#31974=EDGE_CURVE('',#25705,#25706,#11522,.T.);
#31975=EDGE_CURVE('',#25704,#25706,#11523,.T.);
#31976=EDGE_CURVE('',#25707,#25703,#11524,.T.);
#31977=EDGE_CURVE('',#25707,#25708,#11525,.T.);
#31978=EDGE_CURVE('',#25708,#25705,#11526,.T.);
#31979=EDGE_CURVE('',#25704,#25707,#11527,.T.);
#31980=EDGE_CURVE('',#25706,#25708,#11528,.T.);
#31981=EDGE_CURVE('',#25709,#25710,#11529,.T.);
#31982=EDGE_CURVE('',#25709,#25711,#11530,.T.);
#31983=EDGE_CURVE('',#25711,#25712,#11531,.T.);
#31984=EDGE_CURVE('',#25710,#25712,#11532,.T.);
#31985=EDGE_CURVE('',#25713,#25709,#11533,.T.);
#31986=EDGE_CURVE('',#25713,#25714,#11534,.T.);
#31987=EDGE_CURVE('',#25714,#25711,#11535,.T.);
#31988=EDGE_CURVE('',#25715,#25713,#11536,.T.);
#31989=EDGE_CURVE('',#25715,#25716,#11537,.T.);
#31990=EDGE_CURVE('',#25716,#25714,#11538,.T.);
#31991=EDGE_CURVE('',#25717,#25715,#11539,.T.);
#31992=EDGE_CURVE('',#25717,#25718,#11540,.T.);
#31993=EDGE_CURVE('',#25718,#25716,#11541,.T.);
#31994=EDGE_CURVE('',#25719,#25717,#11542,.T.);
#31995=EDGE_CURVE('',#25719,#25720,#11543,.T.);
#31996=EDGE_CURVE('',#25720,#25718,#11544,.T.);
#31997=EDGE_CURVE('',#25721,#25719,#11545,.T.);
#31998=EDGE_CURVE('',#25721,#25722,#11546,.T.);
#31999=EDGE_CURVE('',#25722,#25720,#11547,.T.);
#32000=EDGE_CURVE('',#25723,#25721,#11548,.T.);
#32001=EDGE_CURVE('',#25723,#25724,#11549,.T.);
#32002=EDGE_CURVE('',#25724,#25722,#11550,.T.);
#32003=EDGE_CURVE('',#25725,#25723,#11551,.T.);
#32004=EDGE_CURVE('',#25725,#25726,#11552,.T.);
#32005=EDGE_CURVE('',#25726,#25724,#11553,.T.);
#32006=EDGE_CURVE('',#25727,#25725,#11554,.T.);
#32007=EDGE_CURVE('',#25727,#25728,#11555,.T.);
#32008=EDGE_CURVE('',#25728,#25726,#11556,.T.);
#32009=EDGE_CURVE('',#25729,#25727,#11557,.T.);
#32010=EDGE_CURVE('',#25729,#25730,#11558,.T.);
#32011=EDGE_CURVE('',#25730,#25728,#11559,.T.);
#32012=EDGE_CURVE('',#25710,#25729,#11560,.T.);
#32013=EDGE_CURVE('',#25712,#25730,#11561,.T.);
#32014=EDGE_CURVE('',#25731,#25732,#23920,.T.);
#32015=EDGE_CURVE('',#25731,#25733,#11562,.T.);
#32016=EDGE_CURVE('',#25733,#25734,#23921,.T.);
#32017=EDGE_CURVE('',#25732,#25734,#11563,.T.);
#32018=EDGE_CURVE('',#25735,#25731,#23922,.T.);
#32019=EDGE_CURVE('',#25735,#25736,#11564,.T.);
#32020=EDGE_CURVE('',#25736,#25733,#23923,.T.);
#32021=EDGE_CURVE('',#25737,#25735,#23924,.T.);
#32022=EDGE_CURVE('',#25737,#25738,#11565,.T.);
#32023=EDGE_CURVE('',#25738,#25736,#23925,.T.);
#32024=EDGE_CURVE('',#25739,#25737,#23926,.T.);
#32025=EDGE_CURVE('',#25739,#25740,#11566,.T.);
#32026=EDGE_CURVE('',#25740,#25738,#23927,.T.);
#32027=EDGE_CURVE('',#25741,#25739,#23928,.T.);
#32028=EDGE_CURVE('',#25741,#25742,#11567,.T.);
#32029=EDGE_CURVE('',#25742,#25740,#23929,.T.);
#32030=EDGE_CURVE('',#25743,#25741,#23930,.T.);
#32031=EDGE_CURVE('',#25743,#25744,#11568,.T.);
#32032=EDGE_CURVE('',#25744,#25742,#23931,.T.);
#32033=EDGE_CURVE('',#25745,#25743,#23932,.T.);
#32034=EDGE_CURVE('',#25745,#25746,#11569,.T.);
#32035=EDGE_CURVE('',#25746,#25744,#23933,.T.);
#32036=EDGE_CURVE('',#25732,#25745,#23934,.T.);
#32037=EDGE_CURVE('',#25734,#25746,#23935,.T.);
#32038=EDGE_CURVE('',#25747,#25748,#23936,.T.);
#32039=EDGE_CURVE('',#25747,#25749,#11570,.T.);
#32040=EDGE_CURVE('',#25749,#25750,#23937,.T.);
#32041=EDGE_CURVE('',#25748,#25750,#11571,.T.);
#32042=EDGE_CURVE('',#25751,#25747,#23938,.T.);
#32043=EDGE_CURVE('',#25751,#25752,#11572,.T.);
#32044=EDGE_CURVE('',#25752,#25749,#23939,.T.);
#32045=EDGE_CURVE('',#25753,#25751,#23940,.T.);
#32046=EDGE_CURVE('',#25753,#25754,#11573,.T.);
#32047=EDGE_CURVE('',#25754,#25752,#23941,.T.);
#32048=EDGE_CURVE('',#25755,#25753,#23942,.T.);
#32049=EDGE_CURVE('',#25755,#25756,#11574,.T.);
#32050=EDGE_CURVE('',#25756,#25754,#23943,.T.);
#32051=EDGE_CURVE('',#25757,#25755,#23944,.T.);
#32052=EDGE_CURVE('',#25757,#25758,#11575,.T.);
#32053=EDGE_CURVE('',#25758,#25756,#23945,.T.);
#32054=EDGE_CURVE('',#25759,#25757,#23946,.T.);
#32055=EDGE_CURVE('',#25759,#25760,#11576,.T.);
#32056=EDGE_CURVE('',#25760,#25758,#23947,.T.);
#32057=EDGE_CURVE('',#25761,#25759,#23948,.T.);
#32058=EDGE_CURVE('',#25761,#25762,#11577,.T.);
#32059=EDGE_CURVE('',#25762,#25760,#23949,.T.);
#32060=EDGE_CURVE('',#25763,#25761,#23950,.T.);
#32061=EDGE_CURVE('',#25763,#25764,#11578,.T.);
#32062=EDGE_CURVE('',#25764,#25762,#23951,.T.);
#32063=EDGE_CURVE('',#25765,#25763,#23952,.T.);
#32064=EDGE_CURVE('',#25765,#25766,#11579,.T.);
#32065=EDGE_CURVE('',#25766,#25764,#23953,.T.);
#32066=EDGE_CURVE('',#25767,#25765,#23954,.T.);
#32067=EDGE_CURVE('',#25767,#25768,#11580,.T.);
#32068=EDGE_CURVE('',#25768,#25766,#23955,.T.);
#32069=EDGE_CURVE('',#25769,#25767,#23956,.T.);
#32070=EDGE_CURVE('',#25769,#25770,#11581,.T.);
#32071=EDGE_CURVE('',#25770,#25768,#23957,.T.);
#32072=EDGE_CURVE('',#25748,#25769,#23958,.T.);
#32073=EDGE_CURVE('',#25750,#25770,#23959,.T.);
#32074=EDGE_CURVE('',#25771,#25772,#23960,.T.);
#32075=EDGE_CURVE('',#25771,#25773,#11582,.T.);
#32076=EDGE_CURVE('',#25773,#25774,#23961,.T.);
#32077=EDGE_CURVE('',#25772,#25774,#11583,.T.);
#32078=EDGE_CURVE('',#25775,#25771,#23962,.T.);
#32079=EDGE_CURVE('',#25775,#25776,#11584,.T.);
#32080=EDGE_CURVE('',#25776,#25773,#23963,.T.);
#32081=EDGE_CURVE('',#25777,#25775,#23964,.T.);
#32082=EDGE_CURVE('',#25777,#25778,#11585,.T.);
#32083=EDGE_CURVE('',#25778,#25776,#23965,.T.);
#32084=EDGE_CURVE('',#25779,#25777,#23966,.T.);
#32085=EDGE_CURVE('',#25779,#25780,#11586,.T.);
#32086=EDGE_CURVE('',#25780,#25778,#23967,.T.);
#32087=EDGE_CURVE('',#25781,#25779,#23968,.T.);
#32088=EDGE_CURVE('',#25781,#25782,#11587,.T.);
#32089=EDGE_CURVE('',#25782,#25780,#23969,.T.);
#32090=EDGE_CURVE('',#25783,#25781,#23970,.T.);
#32091=EDGE_CURVE('',#25783,#25784,#11588,.T.);
#32092=EDGE_CURVE('',#25784,#25782,#23971,.T.);
#32093=EDGE_CURVE('',#25785,#25783,#11589,.T.);
#32094=EDGE_CURVE('',#25785,#25786,#11590,.T.);
#32095=EDGE_CURVE('',#25786,#25784,#11591,.T.);
#32096=EDGE_CURVE('',#25787,#25785,#11592,.T.);
#32097=EDGE_CURVE('',#25787,#25788,#11593,.T.);
#32098=EDGE_CURVE('',#25788,#25786,#11594,.T.);
#32099=EDGE_CURVE('',#25789,#25787,#11595,.T.);
#32100=EDGE_CURVE('',#25789,#25790,#11596,.T.);
#32101=EDGE_CURVE('',#25790,#25788,#11597,.T.);
#32102=EDGE_CURVE('',#25791,#25789,#11598,.T.);
#32103=EDGE_CURVE('',#25791,#25792,#11599,.T.);
#32104=EDGE_CURVE('',#25792,#25790,#11600,.T.);
#32105=EDGE_CURVE('',#25793,#25791,#11601,.T.);
#32106=EDGE_CURVE('',#25793,#25794,#11602,.T.);
#32107=EDGE_CURVE('',#25794,#25792,#11603,.T.);
#32108=EDGE_CURVE('',#25795,#25793,#11604,.T.);
#32109=EDGE_CURVE('',#25795,#25796,#11605,.T.);
#32110=EDGE_CURVE('',#25796,#25794,#11606,.T.);
#32111=EDGE_CURVE('',#25797,#25795,#23972,.T.);
#32112=EDGE_CURVE('',#25797,#25798,#11607,.T.);
#32113=EDGE_CURVE('',#25798,#25796,#23973,.T.);
#32114=EDGE_CURVE('',#25799,#25797,#23974,.T.);
#32115=EDGE_CURVE('',#25799,#25800,#11608,.T.);
#32116=EDGE_CURVE('',#25800,#25798,#23975,.T.);
#32117=EDGE_CURVE('',#25801,#25799,#23976,.T.);
#32118=EDGE_CURVE('',#25801,#25802,#11609,.T.);
#32119=EDGE_CURVE('',#25802,#25800,#23977,.T.);
#32120=EDGE_CURVE('',#25803,#25801,#23978,.T.);
#32121=EDGE_CURVE('',#25803,#25804,#11610,.T.);
#32122=EDGE_CURVE('',#25804,#25802,#23979,.T.);
#32123=EDGE_CURVE('',#25805,#25803,#23980,.T.);
#32124=EDGE_CURVE('',#25805,#25806,#11611,.T.);
#32125=EDGE_CURVE('',#25806,#25804,#23981,.T.);
#32126=EDGE_CURVE('',#25807,#25805,#23982,.T.);
#32127=EDGE_CURVE('',#25807,#25808,#11612,.T.);
#32128=EDGE_CURVE('',#25808,#25806,#23983,.T.);
#32129=EDGE_CURVE('',#25809,#25807,#23984,.T.);
#32130=EDGE_CURVE('',#25809,#25810,#11613,.T.);
#32131=EDGE_CURVE('',#25810,#25808,#23985,.T.);
#32132=EDGE_CURVE('',#25811,#25809,#23986,.T.);
#32133=EDGE_CURVE('',#25811,#25812,#11614,.T.);
#32134=EDGE_CURVE('',#25812,#25810,#23987,.T.);
#32135=EDGE_CURVE('',#25813,#25811,#11615,.T.);
#32136=EDGE_CURVE('',#25813,#25814,#11616,.T.);
#32137=EDGE_CURVE('',#25814,#25812,#11617,.T.);
#32138=EDGE_CURVE('',#25772,#25813,#23988,.T.);
#32139=EDGE_CURVE('',#25774,#25814,#23989,.T.);
#32140=EDGE_CURVE('',#25815,#25816,#23990,.T.);
#32141=EDGE_CURVE('',#25815,#25817,#11618,.T.);
#32142=EDGE_CURVE('',#25817,#25818,#23991,.T.);
#32143=EDGE_CURVE('',#25816,#25818,#11619,.T.);
#32144=EDGE_CURVE('',#25819,#25815,#23992,.T.);
#32145=EDGE_CURVE('',#25819,#25820,#11620,.T.);
#32146=EDGE_CURVE('',#25820,#25817,#23993,.T.);
#32147=EDGE_CURVE('',#25821,#25819,#23994,.T.);
#32148=EDGE_CURVE('',#25821,#25822,#11621,.T.);
#32149=EDGE_CURVE('',#25822,#25820,#23995,.T.);
#32150=EDGE_CURVE('',#25823,#25821,#23996,.T.);
#32151=EDGE_CURVE('',#25823,#25824,#11622,.T.);
#32152=EDGE_CURVE('',#25824,#25822,#23997,.T.);
#32153=EDGE_CURVE('',#25825,#25823,#23998,.T.);
#32154=EDGE_CURVE('',#25825,#25826,#11623,.T.);
#32155=EDGE_CURVE('',#25826,#25824,#23999,.T.);
#32156=EDGE_CURVE('',#25827,#25825,#24000,.T.);
#32157=EDGE_CURVE('',#25827,#25828,#11624,.T.);
#32158=EDGE_CURVE('',#25828,#25826,#24001,.T.);
#32159=EDGE_CURVE('',#25829,#25827,#24002,.T.);
#32160=EDGE_CURVE('',#25829,#25830,#11625,.T.);
#32161=EDGE_CURVE('',#25830,#25828,#24003,.T.);
#32162=EDGE_CURVE('',#25816,#25829,#24004,.T.);
#32163=EDGE_CURVE('',#25818,#25830,#24005,.T.);
#32164=EDGE_CURVE('',#25831,#25832,#24006,.T.);
#32165=EDGE_CURVE('',#25831,#25833,#11626,.T.);
#32166=EDGE_CURVE('',#25833,#25834,#24007,.T.);
#32167=EDGE_CURVE('',#25832,#25834,#11627,.T.);
#32168=EDGE_CURVE('',#25835,#25831,#24008,.T.);
#32169=EDGE_CURVE('',#25835,#25836,#11628,.T.);
#32170=EDGE_CURVE('',#25836,#25833,#24009,.T.);
#32171=EDGE_CURVE('',#25837,#25835,#24010,.T.);
#32172=EDGE_CURVE('',#25837,#25838,#11629,.T.);
#32173=EDGE_CURVE('',#25838,#25836,#24011,.T.);
#32174=EDGE_CURVE('',#25839,#25837,#24012,.T.);
#32175=EDGE_CURVE('',#25839,#25840,#11630,.T.);
#32176=EDGE_CURVE('',#25840,#25838,#24013,.T.);
#32177=EDGE_CURVE('',#25841,#25839,#24014,.T.);
#32178=EDGE_CURVE('',#25841,#25842,#11631,.T.);
#32179=EDGE_CURVE('',#25842,#25840,#24015,.T.);
#32180=EDGE_CURVE('',#25843,#25841,#24016,.T.);
#32181=EDGE_CURVE('',#25843,#25844,#11632,.T.);
#32182=EDGE_CURVE('',#25844,#25842,#24017,.T.);
#32183=EDGE_CURVE('',#25845,#25843,#24018,.T.);
#32184=EDGE_CURVE('',#25845,#25846,#11633,.T.);
#32185=EDGE_CURVE('',#25846,#25844,#24019,.T.);
#32186=EDGE_CURVE('',#25847,#25845,#24020,.T.);
#32187=EDGE_CURVE('',#25847,#25848,#11634,.T.);
#32188=EDGE_CURVE('',#25848,#25846,#24021,.T.);
#32189=EDGE_CURVE('',#25849,#25847,#24022,.T.);
#32190=EDGE_CURVE('',#25849,#25850,#11635,.T.);
#32191=EDGE_CURVE('',#25850,#25848,#24023,.T.);
#32192=EDGE_CURVE('',#25851,#25849,#24024,.T.);
#32193=EDGE_CURVE('',#25851,#25852,#11636,.T.);
#32194=EDGE_CURVE('',#25852,#25850,#24025,.T.);
#32195=EDGE_CURVE('',#25853,#25851,#24026,.T.);
#32196=EDGE_CURVE('',#25853,#25854,#11637,.T.);
#32197=EDGE_CURVE('',#25854,#25852,#24027,.T.);
#32198=EDGE_CURVE('',#25832,#25853,#24028,.T.);
#32199=EDGE_CURVE('',#25834,#25854,#24029,.T.);
#32200=EDGE_CURVE('',#25855,#25856,#24030,.T.);
#32201=EDGE_CURVE('',#25855,#25857,#11638,.T.);
#32202=EDGE_CURVE('',#25857,#25858,#24031,.T.);
#32203=EDGE_CURVE('',#25856,#25858,#11639,.T.);
#32204=EDGE_CURVE('',#25859,#25855,#24032,.T.);
#32205=EDGE_CURVE('',#25859,#25860,#11640,.T.);
#32206=EDGE_CURVE('',#25860,#25857,#24033,.T.);
#32207=EDGE_CURVE('',#25861,#25859,#24034,.T.);
#32208=EDGE_CURVE('',#25861,#25862,#11641,.T.);
#32209=EDGE_CURVE('',#25862,#25860,#24035,.T.);
#32210=EDGE_CURVE('',#25863,#25861,#24036,.T.);
#32211=EDGE_CURVE('',#25863,#25864,#11642,.T.);
#32212=EDGE_CURVE('',#25864,#25862,#24037,.T.);
#32213=EDGE_CURVE('',#25865,#25863,#24038,.T.);
#32214=EDGE_CURVE('',#25865,#25866,#11643,.T.);
#32215=EDGE_CURVE('',#25866,#25864,#24039,.T.);
#32216=EDGE_CURVE('',#25867,#25865,#24040,.T.);
#32217=EDGE_CURVE('',#25867,#25868,#11644,.T.);
#32218=EDGE_CURVE('',#25868,#25866,#24041,.T.);
#32219=EDGE_CURVE('',#25869,#25867,#24042,.T.);
#32220=EDGE_CURVE('',#25869,#25870,#11645,.T.);
#32221=EDGE_CURVE('',#25870,#25868,#24043,.T.);
#32222=EDGE_CURVE('',#25871,#25869,#24044,.T.);
#32223=EDGE_CURVE('',#25871,#25872,#11646,.T.);
#32224=EDGE_CURVE('',#25872,#25870,#24045,.T.);
#32225=EDGE_CURVE('',#25856,#25871,#24046,.T.);
#32226=EDGE_CURVE('',#25858,#25872,#24047,.T.);
#32227=EDGE_CURVE('',#25873,#25874,#24048,.T.);
#32228=EDGE_CURVE('',#25873,#25875,#11647,.T.);
#32229=EDGE_CURVE('',#25875,#25876,#24049,.T.);
#32230=EDGE_CURVE('',#25874,#25876,#11648,.T.);
#32231=EDGE_CURVE('',#25877,#25873,#24050,.T.);
#32232=EDGE_CURVE('',#25877,#25878,#11649,.T.);
#32233=EDGE_CURVE('',#25878,#25875,#24051,.T.);
#32234=EDGE_CURVE('',#25879,#25877,#24052,.T.);
#32235=EDGE_CURVE('',#25879,#25880,#11650,.T.);
#32236=EDGE_CURVE('',#25880,#25878,#24053,.T.);
#32237=EDGE_CURVE('',#25881,#25879,#24054,.T.);
#32238=EDGE_CURVE('',#25881,#25882,#11651,.T.);
#32239=EDGE_CURVE('',#25882,#25880,#24055,.T.);
#32240=EDGE_CURVE('',#25883,#25881,#24056,.T.);
#32241=EDGE_CURVE('',#25883,#25884,#11652,.T.);
#32242=EDGE_CURVE('',#25884,#25882,#24057,.T.);
#32243=EDGE_CURVE('',#25885,#25883,#24058,.T.);
#32244=EDGE_CURVE('',#25885,#25886,#11653,.T.);
#32245=EDGE_CURVE('',#25886,#25884,#24059,.T.);
#32246=EDGE_CURVE('',#25887,#25885,#24060,.T.);
#32247=EDGE_CURVE('',#25887,#25888,#11654,.T.);
#32248=EDGE_CURVE('',#25888,#25886,#24061,.T.);
#32249=EDGE_CURVE('',#25889,#25887,#24062,.T.);
#32250=EDGE_CURVE('',#25889,#25890,#11655,.T.);
#32251=EDGE_CURVE('',#25890,#25888,#24063,.T.);
#32252=EDGE_CURVE('',#25891,#25889,#24064,.T.);
#32253=EDGE_CURVE('',#25891,#25892,#11656,.T.);
#32254=EDGE_CURVE('',#25892,#25890,#24065,.T.);
#32255=EDGE_CURVE('',#25893,#25891,#24066,.T.);
#32256=EDGE_CURVE('',#25893,#25894,#11657,.T.);
#32257=EDGE_CURVE('',#25894,#25892,#24067,.T.);
#32258=EDGE_CURVE('',#25895,#25893,#24068,.T.);
#32259=EDGE_CURVE('',#25895,#25896,#11658,.T.);
#32260=EDGE_CURVE('',#25896,#25894,#24069,.T.);
#32261=EDGE_CURVE('',#25897,#25895,#24070,.T.);
#32262=EDGE_CURVE('',#25897,#25898,#11659,.T.);
#32263=EDGE_CURVE('',#25898,#25896,#24071,.T.);
#32264=EDGE_CURVE('',#25899,#25897,#24072,.T.);
#32265=EDGE_CURVE('',#25899,#25900,#11660,.T.);
#32266=EDGE_CURVE('',#25900,#25898,#24073,.T.);
#32267=EDGE_CURVE('',#25901,#25899,#24074,.T.);
#32268=EDGE_CURVE('',#25901,#25902,#11661,.T.);
#32269=EDGE_CURVE('',#25902,#25900,#24075,.T.);
#32270=EDGE_CURVE('',#25903,#25901,#24076,.T.);
#32271=EDGE_CURVE('',#25903,#25904,#11662,.T.);
#32272=EDGE_CURVE('',#25904,#25902,#24077,.T.);
#32273=EDGE_CURVE('',#25905,#25903,#24078,.T.);
#32274=EDGE_CURVE('',#25905,#25906,#11663,.T.);
#32275=EDGE_CURVE('',#25906,#25904,#24079,.T.);
#32276=EDGE_CURVE('',#25907,#25905,#24080,.T.);
#32277=EDGE_CURVE('',#25907,#25908,#11664,.T.);
#32278=EDGE_CURVE('',#25908,#25906,#24081,.T.);
#32279=EDGE_CURVE('',#25909,#25907,#11665,.T.);
#32280=EDGE_CURVE('',#25909,#25910,#11666,.T.);
#32281=EDGE_CURVE('',#25910,#25908,#11667,.T.);
#32282=EDGE_CURVE('',#25874,#25909,#24082,.T.);
#32283=EDGE_CURVE('',#25876,#25910,#24083,.T.);
#32284=EDGE_CURVE('',#25911,#25912,#24084,.T.);
#32285=EDGE_CURVE('',#25911,#25913,#11668,.T.);
#32286=EDGE_CURVE('',#25913,#25914,#24085,.T.);
#32287=EDGE_CURVE('',#25912,#25914,#11669,.T.);
#32288=EDGE_CURVE('',#25915,#25911,#24086,.T.);
#32289=EDGE_CURVE('',#25915,#25916,#11670,.T.);
#32290=EDGE_CURVE('',#25916,#25913,#24087,.T.);
#32291=EDGE_CURVE('',#25917,#25915,#24088,.T.);
#32292=EDGE_CURVE('',#25917,#25918,#11671,.T.);
#32293=EDGE_CURVE('',#25918,#25916,#24089,.T.);
#32294=EDGE_CURVE('',#25919,#25917,#24090,.T.);
#32295=EDGE_CURVE('',#25919,#25920,#11672,.T.);
#32296=EDGE_CURVE('',#25920,#25918,#24091,.T.);
#32297=EDGE_CURVE('',#25921,#25919,#24092,.T.);
#32298=EDGE_CURVE('',#25921,#25922,#11673,.T.);
#32299=EDGE_CURVE('',#25922,#25920,#24093,.T.);
#32300=EDGE_CURVE('',#25923,#25921,#24094,.T.);
#32301=EDGE_CURVE('',#25923,#25924,#11674,.T.);
#32302=EDGE_CURVE('',#25924,#25922,#24095,.T.);
#32303=EDGE_CURVE('',#25925,#25923,#24096,.T.);
#32304=EDGE_CURVE('',#25925,#25926,#11675,.T.);
#32305=EDGE_CURVE('',#25926,#25924,#24097,.T.);
#32306=EDGE_CURVE('',#25912,#25925,#24098,.T.);
#32307=EDGE_CURVE('',#25914,#25926,#24099,.T.);
#32308=EDGE_CURVE('',#25927,#25928,#24100,.T.);
#32309=EDGE_CURVE('',#25927,#25929,#11676,.T.);
#32310=EDGE_CURVE('',#25929,#25930,#24101,.T.);
#32311=EDGE_CURVE('',#25928,#25930,#11677,.T.);
#32312=EDGE_CURVE('',#25931,#25927,#24102,.T.);
#32313=EDGE_CURVE('',#25931,#25932,#11678,.T.);
#32314=EDGE_CURVE('',#25932,#25929,#24103,.T.);
#32315=EDGE_CURVE('',#25933,#25931,#24104,.T.);
#32316=EDGE_CURVE('',#25933,#25934,#11679,.T.);
#32317=EDGE_CURVE('',#25934,#25932,#24105,.T.);
#32318=EDGE_CURVE('',#25935,#25933,#24106,.T.);
#32319=EDGE_CURVE('',#25935,#25936,#11680,.T.);
#32320=EDGE_CURVE('',#25936,#25934,#24107,.T.);
#32321=EDGE_CURVE('',#25937,#25935,#24108,.T.);
#32322=EDGE_CURVE('',#25937,#25938,#11681,.T.);
#32323=EDGE_CURVE('',#25938,#25936,#24109,.T.);
#32324=EDGE_CURVE('',#25939,#25937,#24110,.T.);
#32325=EDGE_CURVE('',#25939,#25940,#11682,.T.);
#32326=EDGE_CURVE('',#25940,#25938,#24111,.T.);
#32327=EDGE_CURVE('',#25941,#25939,#24112,.T.);
#32328=EDGE_CURVE('',#25941,#25942,#11683,.T.);
#32329=EDGE_CURVE('',#25942,#25940,#24113,.T.);
#32330=EDGE_CURVE('',#25943,#25941,#24114,.T.);
#32331=EDGE_CURVE('',#25943,#25944,#11684,.T.);
#32332=EDGE_CURVE('',#25944,#25942,#24115,.T.);
#32333=EDGE_CURVE('',#25945,#25943,#24116,.T.);
#32334=EDGE_CURVE('',#25945,#25946,#11685,.T.);
#32335=EDGE_CURVE('',#25946,#25944,#24117,.T.);
#32336=EDGE_CURVE('',#25947,#25945,#24118,.T.);
#32337=EDGE_CURVE('',#25947,#25948,#11686,.T.);
#32338=EDGE_CURVE('',#25948,#25946,#24119,.T.);
#32339=EDGE_CURVE('',#25949,#25947,#24120,.T.);
#32340=EDGE_CURVE('',#25949,#25950,#11687,.T.);
#32341=EDGE_CURVE('',#25950,#25948,#24121,.T.);
#32342=EDGE_CURVE('',#25928,#25949,#24122,.T.);
#32343=EDGE_CURVE('',#25930,#25950,#24123,.T.);
#32344=EDGE_CURVE('',#25951,#25952,#24124,.T.);
#32345=EDGE_CURVE('',#25951,#25953,#11688,.T.);
#32346=EDGE_CURVE('',#25953,#25954,#24125,.T.);
#32347=EDGE_CURVE('',#25952,#25954,#11689,.T.);
#32348=EDGE_CURVE('',#25955,#25951,#24126,.T.);
#32349=EDGE_CURVE('',#25955,#25956,#11690,.T.);
#32350=EDGE_CURVE('',#25956,#25953,#24127,.T.);
#32351=EDGE_CURVE('',#25957,#25955,#24128,.T.);
#32352=EDGE_CURVE('',#25957,#25958,#11691,.T.);
#32353=EDGE_CURVE('',#25958,#25956,#24129,.T.);
#32354=EDGE_CURVE('',#25959,#25957,#11692,.T.);
#32355=EDGE_CURVE('',#25959,#25960,#11693,.T.);
#32356=EDGE_CURVE('',#25960,#25958,#11694,.T.);
#32357=EDGE_CURVE('',#25961,#25959,#24130,.T.);
#32358=EDGE_CURVE('',#25961,#25962,#11695,.T.);
#32359=EDGE_CURVE('',#25962,#25960,#24131,.T.);
#32360=EDGE_CURVE('',#25963,#25961,#24132,.T.);
#32361=EDGE_CURVE('',#25963,#25964,#11696,.T.);
#32362=EDGE_CURVE('',#25964,#25962,#24133,.T.);
#32363=EDGE_CURVE('',#25965,#25963,#24134,.T.);
#32364=EDGE_CURVE('',#25965,#25966,#11697,.T.);
#32365=EDGE_CURVE('',#25966,#25964,#24135,.T.);
#32366=EDGE_CURVE('',#25967,#25965,#11698,.T.);
#32367=EDGE_CURVE('',#25967,#25968,#11699,.T.);
#32368=EDGE_CURVE('',#25968,#25966,#11700,.T.);
#32369=EDGE_CURVE('',#25969,#25967,#11701,.T.);
#32370=EDGE_CURVE('',#25969,#25970,#11702,.T.);
#32371=EDGE_CURVE('',#25970,#25968,#11703,.T.);
#32372=EDGE_CURVE('',#25971,#25969,#11704,.T.);
#32373=EDGE_CURVE('',#25971,#25972,#11705,.T.);
#32374=EDGE_CURVE('',#25972,#25970,#11706,.T.);
#32375=EDGE_CURVE('',#25952,#25971,#11707,.T.);
#32376=EDGE_CURVE('',#25954,#25972,#11708,.T.);
#32377=EDGE_CURVE('',#25973,#25974,#24136,.T.);
#32378=EDGE_CURVE('',#25973,#25975,#11709,.T.);
#32379=EDGE_CURVE('',#25975,#25976,#24137,.T.);
#32380=EDGE_CURVE('',#25974,#25976,#11710,.T.);
#32381=EDGE_CURVE('',#25977,#25973,#24138,.T.);
#32382=EDGE_CURVE('',#25977,#25978,#11711,.T.);
#32383=EDGE_CURVE('',#25978,#25975,#24139,.T.);
#32384=EDGE_CURVE('',#25979,#25977,#24140,.T.);
#32385=EDGE_CURVE('',#25979,#25980,#11712,.T.);
#32386=EDGE_CURVE('',#25980,#25978,#24141,.T.);
#32387=EDGE_CURVE('',#25981,#25979,#24142,.T.);
#32388=EDGE_CURVE('',#25981,#25982,#11713,.T.);
#32389=EDGE_CURVE('',#25982,#25980,#24143,.T.);
#32390=EDGE_CURVE('',#25983,#25981,#24144,.T.);
#32391=EDGE_CURVE('',#25983,#25984,#11714,.T.);
#32392=EDGE_CURVE('',#25984,#25982,#24145,.T.);
#32393=EDGE_CURVE('',#25985,#25983,#24146,.T.);
#32394=EDGE_CURVE('',#25985,#25986,#11715,.T.);
#32395=EDGE_CURVE('',#25986,#25984,#24147,.T.);
#32396=EDGE_CURVE('',#25987,#25985,#24148,.T.);
#32397=EDGE_CURVE('',#25987,#25988,#11716,.T.);
#32398=EDGE_CURVE('',#25988,#25986,#24149,.T.);
#32399=EDGE_CURVE('',#25974,#25987,#24150,.T.);
#32400=EDGE_CURVE('',#25976,#25988,#24151,.T.);
#32401=EDGE_CURVE('',#25989,#25990,#24152,.T.);
#32402=EDGE_CURVE('',#25989,#25991,#11717,.T.);
#32403=EDGE_CURVE('',#25991,#25992,#24153,.T.);
#32404=EDGE_CURVE('',#25990,#25992,#11718,.T.);
#32405=EDGE_CURVE('',#25993,#25989,#24154,.T.);
#32406=EDGE_CURVE('',#25993,#25994,#11719,.T.);
#32407=EDGE_CURVE('',#25994,#25991,#24155,.T.);
#32408=EDGE_CURVE('',#25995,#25993,#24156,.T.);
#32409=EDGE_CURVE('',#25995,#25996,#11720,.T.);
#32410=EDGE_CURVE('',#25996,#25994,#24157,.T.);
#32411=EDGE_CURVE('',#25997,#25995,#24158,.T.);
#32412=EDGE_CURVE('',#25997,#25998,#11721,.T.);
#32413=EDGE_CURVE('',#25998,#25996,#24159,.T.);
#32414=EDGE_CURVE('',#25999,#25997,#24160,.T.);
#32415=EDGE_CURVE('',#25999,#26000,#11722,.T.);
#32416=EDGE_CURVE('',#26000,#25998,#24161,.T.);
#32417=EDGE_CURVE('',#26001,#25999,#24162,.T.);
#32418=EDGE_CURVE('',#26001,#26002,#11723,.T.);
#32419=EDGE_CURVE('',#26002,#26000,#24163,.T.);
#32420=EDGE_CURVE('',#26003,#26001,#24164,.T.);
#32421=EDGE_CURVE('',#26003,#26004,#11724,.T.);
#32422=EDGE_CURVE('',#26004,#26002,#24165,.T.);
#32423=EDGE_CURVE('',#26005,#26003,#24166,.T.);
#32424=EDGE_CURVE('',#26005,#26006,#11725,.T.);
#32425=EDGE_CURVE('',#26006,#26004,#24167,.T.);
#32426=EDGE_CURVE('',#26007,#26005,#24168,.T.);
#32427=EDGE_CURVE('',#26007,#26008,#11726,.T.);
#32428=EDGE_CURVE('',#26008,#26006,#24169,.T.);
#32429=EDGE_CURVE('',#26009,#26007,#24170,.T.);
#32430=EDGE_CURVE('',#26009,#26010,#11727,.T.);
#32431=EDGE_CURVE('',#26010,#26008,#24171,.T.);
#32432=EDGE_CURVE('',#26011,#26009,#24172,.T.);
#32433=EDGE_CURVE('',#26011,#26012,#11728,.T.);
#32434=EDGE_CURVE('',#26012,#26010,#24173,.T.);
#32435=EDGE_CURVE('',#25990,#26011,#24174,.T.);
#32436=EDGE_CURVE('',#25992,#26012,#24175,.T.);
#32437=EDGE_CURVE('',#26013,#26014,#24176,.T.);
#32438=EDGE_CURVE('',#26013,#26015,#11729,.T.);
#32439=EDGE_CURVE('',#26015,#26016,#24177,.T.);
#32440=EDGE_CURVE('',#26014,#26016,#11730,.T.);
#32441=EDGE_CURVE('',#26017,#26013,#24178,.T.);
#32442=EDGE_CURVE('',#26017,#26018,#11731,.T.);
#32443=EDGE_CURVE('',#26018,#26015,#24179,.T.);
#32444=EDGE_CURVE('',#26019,#26017,#24180,.T.);
#32445=EDGE_CURVE('',#26019,#26020,#11732,.T.);
#32446=EDGE_CURVE('',#26020,#26018,#24181,.T.);
#32447=EDGE_CURVE('',#26021,#26019,#24182,.T.);
#32448=EDGE_CURVE('',#26021,#26022,#11733,.T.);
#32449=EDGE_CURVE('',#26022,#26020,#24183,.T.);
#32450=EDGE_CURVE('',#26023,#26021,#24184,.T.);
#32451=EDGE_CURVE('',#26023,#26024,#11734,.T.);
#32452=EDGE_CURVE('',#26024,#26022,#24185,.T.);
#32453=EDGE_CURVE('',#26025,#26023,#24186,.T.);
#32454=EDGE_CURVE('',#26025,#26026,#11735,.T.);
#32455=EDGE_CURVE('',#26026,#26024,#24187,.T.);
#32456=EDGE_CURVE('',#26027,#26025,#24188,.T.);
#32457=EDGE_CURVE('',#26027,#26028,#11736,.T.);
#32458=EDGE_CURVE('',#26028,#26026,#24189,.T.);
#32459=EDGE_CURVE('',#26014,#26027,#24190,.T.);
#32460=EDGE_CURVE('',#26016,#26028,#24191,.T.);
#32461=EDGE_CURVE('',#26029,#26030,#24192,.T.);
#32462=EDGE_CURVE('',#26029,#26031,#11737,.T.);
#32463=EDGE_CURVE('',#26031,#26032,#24193,.T.);
#32464=EDGE_CURVE('',#26030,#26032,#11738,.T.);
#32465=EDGE_CURVE('',#26033,#26029,#24194,.T.);
#32466=EDGE_CURVE('',#26033,#26034,#11739,.T.);
#32467=EDGE_CURVE('',#26034,#26031,#24195,.T.);
#32468=EDGE_CURVE('',#26035,#26033,#24196,.T.);
#32469=EDGE_CURVE('',#26035,#26036,#11740,.T.);
#32470=EDGE_CURVE('',#26036,#26034,#24197,.T.);
#32471=EDGE_CURVE('',#26037,#26035,#24198,.T.);
#32472=EDGE_CURVE('',#26037,#26038,#11741,.T.);
#32473=EDGE_CURVE('',#26038,#26036,#24199,.T.);
#32474=EDGE_CURVE('',#26039,#26037,#24200,.T.);
#32475=EDGE_CURVE('',#26039,#26040,#11742,.T.);
#32476=EDGE_CURVE('',#26040,#26038,#24201,.T.);
#32477=EDGE_CURVE('',#26041,#26039,#24202,.T.);
#32478=EDGE_CURVE('',#26041,#26042,#11743,.T.);
#32479=EDGE_CURVE('',#26042,#26040,#24203,.T.);
#32480=EDGE_CURVE('',#26043,#26041,#24204,.T.);
#32481=EDGE_CURVE('',#26043,#26044,#11744,.T.);
#32482=EDGE_CURVE('',#26044,#26042,#24205,.T.);
#32483=EDGE_CURVE('',#26045,#26043,#24206,.T.);
#32484=EDGE_CURVE('',#26045,#26046,#11745,.T.);
#32485=EDGE_CURVE('',#26046,#26044,#24207,.T.);
#32486=EDGE_CURVE('',#26030,#26045,#24208,.T.);
#32487=EDGE_CURVE('',#26032,#26046,#24209,.T.);
#32488=EDGE_CURVE('',#26047,#26048,#24210,.T.);
#32489=EDGE_CURVE('',#26047,#26049,#11746,.T.);
#32490=EDGE_CURVE('',#26049,#26050,#24211,.T.);
#32491=EDGE_CURVE('',#26048,#26050,#11747,.T.);
#32492=EDGE_CURVE('',#26051,#26047,#24212,.T.);
#32493=EDGE_CURVE('',#26051,#26052,#11748,.T.);
#32494=EDGE_CURVE('',#26052,#26049,#24213,.T.);
#32495=EDGE_CURVE('',#26053,#26051,#24214,.T.);
#32496=EDGE_CURVE('',#26053,#26054,#11749,.T.);
#32497=EDGE_CURVE('',#26054,#26052,#24215,.T.);
#32498=EDGE_CURVE('',#26055,#26053,#24216,.T.);
#32499=EDGE_CURVE('',#26055,#26056,#11750,.T.);
#32500=EDGE_CURVE('',#26056,#26054,#24217,.T.);
#32501=EDGE_CURVE('',#26057,#26055,#24218,.T.);
#32502=EDGE_CURVE('',#26057,#26058,#11751,.T.);
#32503=EDGE_CURVE('',#26058,#26056,#24219,.T.);
#32504=EDGE_CURVE('',#26059,#26057,#24220,.T.);
#32505=EDGE_CURVE('',#26059,#26060,#11752,.T.);
#32506=EDGE_CURVE('',#26060,#26058,#24221,.T.);
#32507=EDGE_CURVE('',#26061,#26059,#24222,.T.);
#32508=EDGE_CURVE('',#26061,#26062,#11753,.T.);
#32509=EDGE_CURVE('',#26062,#26060,#24223,.T.);
#32510=EDGE_CURVE('',#26063,#26061,#24224,.T.);
#32511=EDGE_CURVE('',#26063,#26064,#11754,.T.);
#32512=EDGE_CURVE('',#26064,#26062,#24225,.T.);
#32513=EDGE_CURVE('',#26065,#26063,#24226,.T.);
#32514=EDGE_CURVE('',#26065,#26066,#11755,.T.);
#32515=EDGE_CURVE('',#26066,#26064,#24227,.T.);
#32516=EDGE_CURVE('',#26067,#26065,#24228,.T.);
#32517=EDGE_CURVE('',#26067,#26068,#11756,.T.);
#32518=EDGE_CURVE('',#26068,#26066,#24229,.T.);
#32519=EDGE_CURVE('',#26069,#26067,#24230,.T.);
#32520=EDGE_CURVE('',#26069,#26070,#11757,.T.);
#32521=EDGE_CURVE('',#26070,#26068,#24231,.T.);
#32522=EDGE_CURVE('',#26071,#26069,#24232,.T.);
#32523=EDGE_CURVE('',#26071,#26072,#11758,.T.);
#32524=EDGE_CURVE('',#26072,#26070,#24233,.T.);
#32525=EDGE_CURVE('',#26073,#26071,#24234,.T.);
#32526=EDGE_CURVE('',#26073,#26074,#11759,.T.);
#32527=EDGE_CURVE('',#26074,#26072,#24235,.T.);
#32528=EDGE_CURVE('',#26075,#26073,#24236,.T.);
#32529=EDGE_CURVE('',#26075,#26076,#11760,.T.);
#32530=EDGE_CURVE('',#26076,#26074,#24237,.T.);
#32531=EDGE_CURVE('',#26077,#26075,#24238,.T.);
#32532=EDGE_CURVE('',#26077,#26078,#11761,.T.);
#32533=EDGE_CURVE('',#26078,#26076,#24239,.T.);
#32534=EDGE_CURVE('',#26048,#26077,#24240,.T.);
#32535=EDGE_CURVE('',#26050,#26078,#24241,.T.);
#32536=EDGE_CURVE('',#26079,#26080,#24242,.T.);
#32537=EDGE_CURVE('',#26079,#26081,#11762,.T.);
#32538=EDGE_CURVE('',#26081,#26082,#24243,.T.);
#32539=EDGE_CURVE('',#26080,#26082,#11763,.T.);
#32540=EDGE_CURVE('',#26083,#26079,#24244,.T.);
#32541=EDGE_CURVE('',#26083,#26084,#11764,.T.);
#32542=EDGE_CURVE('',#26084,#26081,#24245,.T.);
#32543=EDGE_CURVE('',#26085,#26083,#24246,.T.);
#32544=EDGE_CURVE('',#26085,#26086,#11765,.T.);
#32545=EDGE_CURVE('',#26086,#26084,#24247,.T.);
#32546=EDGE_CURVE('',#26087,#26085,#24248,.T.);
#32547=EDGE_CURVE('',#26087,#26088,#11766,.T.);
#32548=EDGE_CURVE('',#26088,#26086,#24249,.T.);
#32549=EDGE_CURVE('',#26089,#26087,#24250,.T.);
#32550=EDGE_CURVE('',#26089,#26090,#11767,.T.);
#32551=EDGE_CURVE('',#26090,#26088,#24251,.T.);
#32552=EDGE_CURVE('',#26091,#26089,#24252,.T.);
#32553=EDGE_CURVE('',#26091,#26092,#11768,.T.);
#32554=EDGE_CURVE('',#26092,#26090,#24253,.T.);
#32555=EDGE_CURVE('',#26093,#26091,#24254,.T.);
#32556=EDGE_CURVE('',#26093,#26094,#11769,.T.);
#32557=EDGE_CURVE('',#26094,#26092,#24255,.T.);
#32558=EDGE_CURVE('',#26080,#26093,#24256,.T.);
#32559=EDGE_CURVE('',#26082,#26094,#24257,.T.);
#32560=EDGE_CURVE('',#26095,#26096,#24258,.T.);
#32561=EDGE_CURVE('',#26095,#26097,#11770,.T.);
#32562=EDGE_CURVE('',#26097,#26098,#24259,.T.);
#32563=EDGE_CURVE('',#26096,#26098,#11771,.T.);
#32564=EDGE_CURVE('',#26099,#26095,#24260,.T.);
#32565=EDGE_CURVE('',#26099,#26100,#11772,.T.);
#32566=EDGE_CURVE('',#26100,#26097,#24261,.T.);
#32567=EDGE_CURVE('',#26101,#26099,#24262,.T.);
#32568=EDGE_CURVE('',#26101,#26102,#11773,.T.);
#32569=EDGE_CURVE('',#26102,#26100,#24263,.T.);
#32570=EDGE_CURVE('',#26103,#26101,#24264,.T.);
#32571=EDGE_CURVE('',#26103,#26104,#11774,.T.);
#32572=EDGE_CURVE('',#26104,#26102,#24265,.T.);
#32573=EDGE_CURVE('',#26105,#26103,#24266,.T.);
#32574=EDGE_CURVE('',#26105,#26106,#11775,.T.);
#32575=EDGE_CURVE('',#26106,#26104,#24267,.T.);
#32576=EDGE_CURVE('',#26107,#26105,#24268,.T.);
#32577=EDGE_CURVE('',#26107,#26108,#11776,.T.);
#32578=EDGE_CURVE('',#26108,#26106,#24269,.T.);
#32579=EDGE_CURVE('',#26109,#26107,#24270,.T.);
#32580=EDGE_CURVE('',#26109,#26110,#11777,.T.);
#32581=EDGE_CURVE('',#26110,#26108,#24271,.T.);
#32582=EDGE_CURVE('',#26111,#26109,#24272,.T.);
#32583=EDGE_CURVE('',#26111,#26112,#11778,.T.);
#32584=EDGE_CURVE('',#26112,#26110,#24273,.T.);
#32585=EDGE_CURVE('',#26113,#26111,#24274,.T.);
#32586=EDGE_CURVE('',#26113,#26114,#11779,.T.);
#32587=EDGE_CURVE('',#26114,#26112,#24275,.T.);
#32588=EDGE_CURVE('',#26115,#26113,#24276,.T.);
#32589=EDGE_CURVE('',#26115,#26116,#11780,.T.);
#32590=EDGE_CURVE('',#26116,#26114,#24277,.T.);
#32591=EDGE_CURVE('',#26117,#26115,#24278,.T.);
#32592=EDGE_CURVE('',#26117,#26118,#11781,.T.);
#32593=EDGE_CURVE('',#26118,#26116,#24279,.T.);
#32594=EDGE_CURVE('',#26096,#26117,#24280,.T.);
#32595=EDGE_CURVE('',#26098,#26118,#24281,.T.);
#32596=EDGE_CURVE('',#26119,#26120,#24282,.T.);
#32597=EDGE_CURVE('',#26119,#26121,#11782,.T.);
#32598=EDGE_CURVE('',#26121,#26122,#24283,.T.);
#32599=EDGE_CURVE('',#26120,#26122,#11783,.T.);
#32600=EDGE_CURVE('',#26123,#26119,#24284,.T.);
#32601=EDGE_CURVE('',#26123,#26124,#11784,.T.);
#32602=EDGE_CURVE('',#26124,#26121,#24285,.T.);
#32603=EDGE_CURVE('',#26125,#26123,#24286,.T.);
#32604=EDGE_CURVE('',#26125,#26126,#11785,.T.);
#32605=EDGE_CURVE('',#26126,#26124,#24287,.T.);
#32606=EDGE_CURVE('',#26127,#26125,#24288,.T.);
#32607=EDGE_CURVE('',#26127,#26128,#11786,.T.);
#32608=EDGE_CURVE('',#26128,#26126,#24289,.T.);
#32609=EDGE_CURVE('',#26129,#26127,#24290,.T.);
#32610=EDGE_CURVE('',#26129,#26130,#11787,.T.);
#32611=EDGE_CURVE('',#26130,#26128,#24291,.T.);
#32612=EDGE_CURVE('',#26131,#26129,#24292,.T.);
#32613=EDGE_CURVE('',#26131,#26132,#11788,.T.);
#32614=EDGE_CURVE('',#26132,#26130,#24293,.T.);
#32615=EDGE_CURVE('',#26133,#26131,#24294,.T.);
#32616=EDGE_CURVE('',#26133,#26134,#11789,.T.);
#32617=EDGE_CURVE('',#26134,#26132,#24295,.T.);
#32618=EDGE_CURVE('',#26120,#26133,#24296,.T.);
#32619=EDGE_CURVE('',#26122,#26134,#24297,.T.);
#32620=EDGE_CURVE('',#26135,#26136,#24298,.T.);
#32621=EDGE_CURVE('',#26135,#26137,#11790,.T.);
#32622=EDGE_CURVE('',#26137,#26138,#24299,.T.);
#32623=EDGE_CURVE('',#26136,#26138,#11791,.T.);
#32624=EDGE_CURVE('',#26139,#26135,#24300,.T.);
#32625=EDGE_CURVE('',#26139,#26140,#11792,.T.);
#32626=EDGE_CURVE('',#26140,#26137,#24301,.T.);
#32627=EDGE_CURVE('',#26141,#26139,#24302,.T.);
#32628=EDGE_CURVE('',#26141,#26142,#11793,.T.);
#32629=EDGE_CURVE('',#26142,#26140,#24303,.T.);
#32630=EDGE_CURVE('',#26143,#26141,#24304,.T.);
#32631=EDGE_CURVE('',#26143,#26144,#11794,.T.);
#32632=EDGE_CURVE('',#26144,#26142,#24305,.T.);
#32633=EDGE_CURVE('',#26145,#26143,#24306,.T.);
#32634=EDGE_CURVE('',#26145,#26146,#11795,.T.);
#32635=EDGE_CURVE('',#26146,#26144,#24307,.T.);
#32636=EDGE_CURVE('',#26147,#26145,#24308,.T.);
#32637=EDGE_CURVE('',#26147,#26148,#11796,.T.);
#32638=EDGE_CURVE('',#26148,#26146,#24309,.T.);
#32639=EDGE_CURVE('',#26149,#26147,#24310,.T.);
#32640=EDGE_CURVE('',#26149,#26150,#11797,.T.);
#32641=EDGE_CURVE('',#26150,#26148,#24311,.T.);
#32642=EDGE_CURVE('',#26151,#26149,#24312,.T.);
#32643=EDGE_CURVE('',#26151,#26152,#11798,.T.);
#32644=EDGE_CURVE('',#26152,#26150,#24313,.T.);
#32645=EDGE_CURVE('',#26153,#26151,#24314,.T.);
#32646=EDGE_CURVE('',#26153,#26154,#11799,.T.);
#32647=EDGE_CURVE('',#26154,#26152,#24315,.T.);
#32648=EDGE_CURVE('',#26155,#26153,#24316,.T.);
#32649=EDGE_CURVE('',#26155,#26156,#11800,.T.);
#32650=EDGE_CURVE('',#26156,#26154,#24317,.T.);
#32651=EDGE_CURVE('',#26157,#26155,#24318,.T.);
#32652=EDGE_CURVE('',#26157,#26158,#11801,.T.);
#32653=EDGE_CURVE('',#26158,#26156,#24319,.T.);
#32654=EDGE_CURVE('',#26159,#26157,#24320,.T.);
#32655=EDGE_CURVE('',#26159,#26160,#11802,.T.);
#32656=EDGE_CURVE('',#26160,#26158,#24321,.T.);
#32657=EDGE_CURVE('',#26161,#26159,#24322,.T.);
#32658=EDGE_CURVE('',#26161,#26162,#11803,.T.);
#32659=EDGE_CURVE('',#26162,#26160,#24323,.T.);
#32660=EDGE_CURVE('',#26163,#26161,#24324,.T.);
#32661=EDGE_CURVE('',#26163,#26164,#11804,.T.);
#32662=EDGE_CURVE('',#26164,#26162,#24325,.T.);
#32663=EDGE_CURVE('',#26165,#26163,#24326,.T.);
#32664=EDGE_CURVE('',#26165,#26166,#11805,.T.);
#32665=EDGE_CURVE('',#26166,#26164,#24327,.T.);
#32666=EDGE_CURVE('',#26167,#26165,#24328,.T.);
#32667=EDGE_CURVE('',#26167,#26168,#11806,.T.);
#32668=EDGE_CURVE('',#26168,#26166,#24329,.T.);
#32669=EDGE_CURVE('',#26169,#26167,#24330,.T.);
#32670=EDGE_CURVE('',#26169,#26170,#11807,.T.);
#32671=EDGE_CURVE('',#26170,#26168,#24331,.T.);
#32672=EDGE_CURVE('',#26171,#26169,#24332,.T.);
#32673=EDGE_CURVE('',#26171,#26172,#11808,.T.);
#32674=EDGE_CURVE('',#26172,#26170,#24333,.T.);
#32675=EDGE_CURVE('',#26173,#26171,#24334,.T.);
#32676=EDGE_CURVE('',#26173,#26174,#11809,.T.);
#32677=EDGE_CURVE('',#26174,#26172,#24335,.T.);
#32678=EDGE_CURVE('',#26175,#26173,#24336,.T.);
#32679=EDGE_CURVE('',#26175,#26176,#11810,.T.);
#32680=EDGE_CURVE('',#26176,#26174,#24337,.T.);
#32681=EDGE_CURVE('',#26177,#26175,#11811,.T.);
#32682=EDGE_CURVE('',#26177,#26178,#11812,.T.);
#32683=EDGE_CURVE('',#26178,#26176,#11813,.T.);
#32684=EDGE_CURVE('',#26136,#26177,#24338,.T.);
#32685=EDGE_CURVE('',#26138,#26178,#24339,.T.);
#32686=EDGE_CURVE('',#26179,#26180,#11814,.T.);
#32687=EDGE_CURVE('',#26179,#26181,#11815,.T.);
#32688=EDGE_CURVE('',#26181,#26182,#11816,.T.);
#32689=EDGE_CURVE('',#26180,#26182,#11817,.T.);
#32690=EDGE_CURVE('',#26183,#26179,#11818,.T.);
#32691=EDGE_CURVE('',#26183,#26184,#11819,.T.);
#32692=EDGE_CURVE('',#26184,#26181,#11820,.T.);
#32693=EDGE_CURVE('',#26185,#26183,#11821,.T.);
#32694=EDGE_CURVE('',#26185,#26186,#11822,.T.);
#32695=EDGE_CURVE('',#26186,#26184,#11823,.T.);
#32696=EDGE_CURVE('',#26180,#26185,#11824,.T.);
#32697=EDGE_CURVE('',#26182,#26186,#11825,.T.);
#32698=EDGE_CURVE('',#26187,#26188,#11826,.T.);
#32699=EDGE_CURVE('',#26187,#26189,#11827,.T.);
#32700=EDGE_CURVE('',#26189,#26190,#11828,.T.);
#32701=EDGE_CURVE('',#26188,#26190,#11829,.T.);
#32702=EDGE_CURVE('',#26191,#26187,#11830,.T.);
#32703=EDGE_CURVE('',#26191,#26192,#11831,.T.);
#32704=EDGE_CURVE('',#26192,#26189,#11832,.T.);
#32705=EDGE_CURVE('',#26193,#26191,#11833,.T.);
#32706=EDGE_CURVE('',#26193,#26194,#11834,.T.);
#32707=EDGE_CURVE('',#26194,#26192,#11835,.T.);
#32708=EDGE_CURVE('',#26188,#26193,#11836,.T.);
#32709=EDGE_CURVE('',#26190,#26194,#11837,.T.);
#32710=EDGE_CURVE('',#26195,#26196,#11838,.T.);
#32711=EDGE_CURVE('',#26195,#26197,#11839,.T.);
#32712=EDGE_CURVE('',#26197,#26198,#11840,.T.);
#32713=EDGE_CURVE('',#26196,#26198,#11841,.T.);
#32714=EDGE_CURVE('',#26199,#26195,#11842,.T.);
#32715=EDGE_CURVE('',#26199,#26200,#11843,.T.);
#32716=EDGE_CURVE('',#26200,#26197,#11844,.T.);
#32717=EDGE_CURVE('',#26201,#26199,#11845,.T.);
#32718=EDGE_CURVE('',#26201,#26202,#11846,.T.);
#32719=EDGE_CURVE('',#26202,#26200,#11847,.T.);
#32720=EDGE_CURVE('',#26196,#26201,#11848,.T.);
#32721=EDGE_CURVE('',#26198,#26202,#11849,.T.);
#32722=EDGE_CURVE('',#26203,#26204,#11850,.T.);
#32723=EDGE_CURVE('',#26203,#26205,#11851,.T.);
#32724=EDGE_CURVE('',#26205,#26206,#11852,.T.);
#32725=EDGE_CURVE('',#26204,#26206,#11853,.T.);
#32726=EDGE_CURVE('',#26207,#26203,#11854,.T.);
#32727=EDGE_CURVE('',#26207,#26208,#11855,.T.);
#32728=EDGE_CURVE('',#26208,#26205,#11856,.T.);
#32729=EDGE_CURVE('',#26209,#26207,#11857,.T.);
#32730=EDGE_CURVE('',#26209,#26210,#11858,.T.);
#32731=EDGE_CURVE('',#26210,#26208,#11859,.T.);
#32732=EDGE_CURVE('',#26204,#26209,#11860,.T.);
#32733=EDGE_CURVE('',#26206,#26210,#11861,.T.);
#32734=EDGE_CURVE('',#26211,#26212,#11862,.T.);
#32735=EDGE_CURVE('',#26211,#26213,#11863,.T.);
#32736=EDGE_CURVE('',#26213,#26214,#11864,.T.);
#32737=EDGE_CURVE('',#26212,#26214,#11865,.T.);
#32738=EDGE_CURVE('',#26215,#26211,#11866,.T.);
#32739=EDGE_CURVE('',#26215,#26216,#11867,.T.);
#32740=EDGE_CURVE('',#26216,#26213,#11868,.T.);
#32741=EDGE_CURVE('',#26217,#26215,#11869,.T.);
#32742=EDGE_CURVE('',#26217,#26218,#11870,.T.);
#32743=EDGE_CURVE('',#26218,#26216,#11871,.T.);
#32744=EDGE_CURVE('',#26212,#26217,#11872,.T.);
#32745=EDGE_CURVE('',#26214,#26218,#11873,.T.);
#32746=EDGE_CURVE('',#26219,#26220,#11874,.T.);
#32747=EDGE_CURVE('',#26219,#26221,#11875,.T.);
#32748=EDGE_CURVE('',#26221,#26222,#11876,.T.);
#32749=EDGE_CURVE('',#26220,#26222,#11877,.T.);
#32750=EDGE_CURVE('',#26223,#26219,#11878,.T.);
#32751=EDGE_CURVE('',#26223,#26224,#11879,.T.);
#32752=EDGE_CURVE('',#26224,#26221,#11880,.T.);
#32753=EDGE_CURVE('',#26225,#26223,#11881,.T.);
#32754=EDGE_CURVE('',#26225,#26226,#11882,.T.);
#32755=EDGE_CURVE('',#26226,#26224,#11883,.T.);
#32756=EDGE_CURVE('',#26220,#26225,#11884,.T.);
#32757=EDGE_CURVE('',#26222,#26226,#11885,.T.);
#32758=EDGE_CURVE('',#26227,#26228,#11886,.T.);
#32759=EDGE_CURVE('',#26227,#26229,#11887,.T.);
#32760=EDGE_CURVE('',#26229,#26230,#11888,.T.);
#32761=EDGE_CURVE('',#26228,#26230,#11889,.T.);
#32762=EDGE_CURVE('',#26231,#26227,#11890,.T.);
#32763=EDGE_CURVE('',#26231,#26232,#11891,.T.);
#32764=EDGE_CURVE('',#26232,#26229,#11892,.T.);
#32765=EDGE_CURVE('',#26233,#26231,#11893,.T.);
#32766=EDGE_CURVE('',#26233,#26234,#11894,.T.);
#32767=EDGE_CURVE('',#26234,#26232,#11895,.T.);
#32768=EDGE_CURVE('',#26228,#26233,#11896,.T.);
#32769=EDGE_CURVE('',#26230,#26234,#11897,.T.);
#32770=EDGE_CURVE('',#26235,#26236,#11898,.T.);
#32771=EDGE_CURVE('',#26235,#26237,#11899,.T.);
#32772=EDGE_CURVE('',#26237,#26238,#11900,.T.);
#32773=EDGE_CURVE('',#26236,#26238,#11901,.T.);
#32774=EDGE_CURVE('',#26239,#26235,#11902,.T.);
#32775=EDGE_CURVE('',#26239,#26240,#11903,.T.);
#32776=EDGE_CURVE('',#26240,#26237,#11904,.T.);
#32777=EDGE_CURVE('',#26241,#26239,#11905,.T.);
#32778=EDGE_CURVE('',#26241,#26242,#11906,.T.);
#32779=EDGE_CURVE('',#26242,#26240,#11907,.T.);
#32780=EDGE_CURVE('',#26236,#26241,#11908,.T.);
#32781=EDGE_CURVE('',#26238,#26242,#11909,.T.);
#32782=EDGE_CURVE('',#26243,#26244,#11910,.T.);
#32783=EDGE_CURVE('',#26243,#26245,#11911,.T.);
#32784=EDGE_CURVE('',#26245,#26246,#11912,.T.);
#32785=EDGE_CURVE('',#26244,#26246,#11913,.T.);
#32786=EDGE_CURVE('',#26247,#26243,#11914,.T.);
#32787=EDGE_CURVE('',#26247,#26248,#11915,.T.);
#32788=EDGE_CURVE('',#26248,#26245,#11916,.T.);
#32789=EDGE_CURVE('',#26249,#26247,#11917,.T.);
#32790=EDGE_CURVE('',#26249,#26250,#11918,.T.);
#32791=EDGE_CURVE('',#26250,#26248,#11919,.T.);
#32792=EDGE_CURVE('',#26244,#26249,#11920,.T.);
#32793=EDGE_CURVE('',#26246,#26250,#11921,.T.);
#32794=EDGE_CURVE('',#26251,#26252,#11922,.T.);
#32795=EDGE_CURVE('',#26251,#26253,#11923,.T.);
#32796=EDGE_CURVE('',#26253,#26254,#11924,.T.);
#32797=EDGE_CURVE('',#26252,#26254,#11925,.T.);
#32798=EDGE_CURVE('',#26255,#26251,#11926,.T.);
#32799=EDGE_CURVE('',#26255,#26256,#11927,.T.);
#32800=EDGE_CURVE('',#26256,#26253,#11928,.T.);
#32801=EDGE_CURVE('',#26257,#26255,#11929,.T.);
#32802=EDGE_CURVE('',#26257,#26258,#11930,.T.);
#32803=EDGE_CURVE('',#26258,#26256,#11931,.T.);
#32804=EDGE_CURVE('',#26252,#26257,#11932,.T.);
#32805=EDGE_CURVE('',#26254,#26258,#11933,.T.);
#32806=EDGE_CURVE('',#26259,#26260,#11934,.T.);
#32807=EDGE_CURVE('',#26259,#26261,#11935,.T.);
#32808=EDGE_CURVE('',#26261,#26262,#11936,.T.);
#32809=EDGE_CURVE('',#26260,#26262,#11937,.T.);
#32810=EDGE_CURVE('',#26263,#26259,#11938,.T.);
#32811=EDGE_CURVE('',#26263,#26264,#11939,.T.);
#32812=EDGE_CURVE('',#26264,#26261,#11940,.T.);
#32813=EDGE_CURVE('',#26265,#26263,#11941,.T.);
#32814=EDGE_CURVE('',#26265,#26266,#11942,.T.);
#32815=EDGE_CURVE('',#26266,#26264,#11943,.T.);
#32816=EDGE_CURVE('',#26260,#26265,#11944,.T.);
#32817=EDGE_CURVE('',#26262,#26266,#11945,.T.);
#32818=EDGE_CURVE('',#26267,#26268,#11946,.T.);
#32819=EDGE_CURVE('',#26267,#26269,#11947,.T.);
#32820=EDGE_CURVE('',#26269,#26270,#11948,.T.);
#32821=EDGE_CURVE('',#26268,#26270,#11949,.T.);
#32822=EDGE_CURVE('',#26271,#26267,#11950,.T.);
#32823=EDGE_CURVE('',#26271,#26272,#11951,.T.);
#32824=EDGE_CURVE('',#26272,#26269,#11952,.T.);
#32825=EDGE_CURVE('',#26273,#26271,#11953,.T.);
#32826=EDGE_CURVE('',#26273,#26274,#11954,.T.);
#32827=EDGE_CURVE('',#26274,#26272,#11955,.T.);
#32828=EDGE_CURVE('',#26268,#26273,#11956,.T.);
#32829=EDGE_CURVE('',#26270,#26274,#11957,.T.);
#32830=EDGE_CURVE('',#26275,#26276,#11958,.T.);
#32831=EDGE_CURVE('',#26275,#26277,#11959,.T.);
#32832=EDGE_CURVE('',#26277,#26278,#11960,.T.);
#32833=EDGE_CURVE('',#26276,#26278,#11961,.T.);
#32834=EDGE_CURVE('',#26279,#26275,#11962,.T.);
#32835=EDGE_CURVE('',#26279,#26280,#11963,.T.);
#32836=EDGE_CURVE('',#26280,#26277,#11964,.T.);
#32837=EDGE_CURVE('',#26281,#26279,#11965,.T.);
#32838=EDGE_CURVE('',#26281,#26282,#11966,.T.);
#32839=EDGE_CURVE('',#26282,#26280,#11967,.T.);
#32840=EDGE_CURVE('',#26276,#26281,#11968,.T.);
#32841=EDGE_CURVE('',#26278,#26282,#11969,.T.);
#32842=EDGE_CURVE('',#26283,#26284,#11970,.T.);
#32843=EDGE_CURVE('',#26283,#26285,#11971,.T.);
#32844=EDGE_CURVE('',#26285,#26286,#11972,.T.);
#32845=EDGE_CURVE('',#26284,#26286,#11973,.T.);
#32846=EDGE_CURVE('',#26287,#26283,#11974,.T.);
#32847=EDGE_CURVE('',#26287,#26288,#11975,.T.);
#32848=EDGE_CURVE('',#26288,#26285,#11976,.T.);
#32849=EDGE_CURVE('',#26289,#26287,#11977,.T.);
#32850=EDGE_CURVE('',#26289,#26290,#11978,.T.);
#32851=EDGE_CURVE('',#26290,#26288,#11979,.T.);
#32852=EDGE_CURVE('',#26284,#26289,#11980,.T.);
#32853=EDGE_CURVE('',#26286,#26290,#11981,.T.);
#32854=EDGE_CURVE('',#26291,#26292,#11982,.T.);
#32855=EDGE_CURVE('',#26291,#26293,#11983,.T.);
#32856=EDGE_CURVE('',#26293,#26294,#11984,.T.);
#32857=EDGE_CURVE('',#26292,#26294,#11985,.T.);
#32858=EDGE_CURVE('',#26295,#26291,#11986,.T.);
#32859=EDGE_CURVE('',#26295,#26296,#11987,.T.);
#32860=EDGE_CURVE('',#26296,#26293,#11988,.T.);
#32861=EDGE_CURVE('',#26297,#26295,#11989,.T.);
#32862=EDGE_CURVE('',#26297,#26298,#11990,.T.);
#32863=EDGE_CURVE('',#26298,#26296,#11991,.T.);
#32864=EDGE_CURVE('',#26292,#26297,#11992,.T.);
#32865=EDGE_CURVE('',#26294,#26298,#11993,.T.);
#32866=EDGE_CURVE('',#26299,#26300,#11994,.T.);
#32867=EDGE_CURVE('',#26299,#26301,#11995,.T.);
#32868=EDGE_CURVE('',#26301,#26302,#11996,.T.);
#32869=EDGE_CURVE('',#26300,#26302,#11997,.T.);
#32870=EDGE_CURVE('',#26303,#26299,#11998,.T.);
#32871=EDGE_CURVE('',#26303,#26304,#11999,.T.);
#32872=EDGE_CURVE('',#26304,#26301,#12000,.T.);
#32873=EDGE_CURVE('',#26305,#26303,#12001,.T.);
#32874=EDGE_CURVE('',#26305,#26306,#12002,.T.);
#32875=EDGE_CURVE('',#26306,#26304,#12003,.T.);
#32876=EDGE_CURVE('',#26300,#26305,#12004,.T.);
#32877=EDGE_CURVE('',#26302,#26306,#12005,.T.);
#32878=EDGE_CURVE('',#26307,#26308,#12006,.T.);
#32879=EDGE_CURVE('',#26307,#26309,#12007,.T.);
#32880=EDGE_CURVE('',#26309,#26310,#12008,.T.);
#32881=EDGE_CURVE('',#26308,#26310,#12009,.T.);
#32882=EDGE_CURVE('',#26311,#26307,#12010,.T.);
#32883=EDGE_CURVE('',#26311,#26312,#12011,.T.);
#32884=EDGE_CURVE('',#26312,#26309,#12012,.T.);
#32885=EDGE_CURVE('',#26313,#26311,#12013,.T.);
#32886=EDGE_CURVE('',#26313,#26314,#12014,.T.);
#32887=EDGE_CURVE('',#26314,#26312,#12015,.T.);
#32888=EDGE_CURVE('',#26308,#26313,#12016,.T.);
#32889=EDGE_CURVE('',#26310,#26314,#12017,.T.);
#32890=EDGE_CURVE('',#26315,#26316,#12018,.T.);
#32891=EDGE_CURVE('',#26315,#26317,#12019,.T.);
#32892=EDGE_CURVE('',#26317,#26318,#12020,.T.);
#32893=EDGE_CURVE('',#26316,#26318,#12021,.T.);
#32894=EDGE_CURVE('',#26319,#26315,#12022,.T.);
#32895=EDGE_CURVE('',#26319,#26320,#12023,.T.);
#32896=EDGE_CURVE('',#26320,#26317,#12024,.T.);
#32897=EDGE_CURVE('',#26321,#26319,#12025,.T.);
#32898=EDGE_CURVE('',#26321,#26322,#12026,.T.);
#32899=EDGE_CURVE('',#26322,#26320,#12027,.T.);
#32900=EDGE_CURVE('',#26316,#26321,#12028,.T.);
#32901=EDGE_CURVE('',#26318,#26322,#12029,.T.);
#32902=EDGE_CURVE('',#26323,#26324,#12030,.T.);
#32903=EDGE_CURVE('',#26323,#26325,#12031,.T.);
#32904=EDGE_CURVE('',#26325,#26326,#12032,.T.);
#32905=EDGE_CURVE('',#26324,#26326,#12033,.T.);
#32906=EDGE_CURVE('',#26327,#26323,#12034,.T.);
#32907=EDGE_CURVE('',#26327,#26328,#12035,.T.);
#32908=EDGE_CURVE('',#26328,#26325,#12036,.T.);
#32909=EDGE_CURVE('',#26329,#26327,#12037,.T.);
#32910=EDGE_CURVE('',#26329,#26330,#12038,.T.);
#32911=EDGE_CURVE('',#26330,#26328,#12039,.T.);
#32912=EDGE_CURVE('',#26324,#26329,#12040,.T.);
#32913=EDGE_CURVE('',#26326,#26330,#12041,.T.);
#32914=EDGE_CURVE('',#26331,#26332,#12042,.T.);
#32915=EDGE_CURVE('',#26331,#26333,#12043,.T.);
#32916=EDGE_CURVE('',#26333,#26334,#12044,.T.);
#32917=EDGE_CURVE('',#26332,#26334,#12045,.T.);
#32918=EDGE_CURVE('',#26335,#26331,#12046,.T.);
#32919=EDGE_CURVE('',#26335,#26336,#12047,.T.);
#32920=EDGE_CURVE('',#26336,#26333,#12048,.T.);
#32921=EDGE_CURVE('',#26337,#26335,#12049,.T.);
#32922=EDGE_CURVE('',#26337,#26338,#12050,.T.);
#32923=EDGE_CURVE('',#26338,#26336,#12051,.T.);
#32924=EDGE_CURVE('',#26332,#26337,#12052,.T.);
#32925=EDGE_CURVE('',#26334,#26338,#12053,.T.);
#32926=EDGE_CURVE('',#26339,#26340,#12054,.T.);
#32927=EDGE_CURVE('',#26339,#26341,#12055,.T.);
#32928=EDGE_CURVE('',#26341,#26342,#12056,.T.);
#32929=EDGE_CURVE('',#26340,#26342,#12057,.T.);
#32930=EDGE_CURVE('',#26343,#26339,#12058,.T.);
#32931=EDGE_CURVE('',#26343,#26344,#12059,.T.);
#32932=EDGE_CURVE('',#26344,#26341,#12060,.T.);
#32933=EDGE_CURVE('',#26345,#26343,#12061,.T.);
#32934=EDGE_CURVE('',#26345,#26346,#12062,.T.);
#32935=EDGE_CURVE('',#26346,#26344,#12063,.T.);
#32936=EDGE_CURVE('',#26340,#26345,#12064,.T.);
#32937=EDGE_CURVE('',#26342,#26346,#12065,.T.);
#32938=EDGE_CURVE('',#26347,#26348,#12066,.T.);
#32939=EDGE_CURVE('',#26347,#26349,#12067,.T.);
#32940=EDGE_CURVE('',#26349,#26350,#12068,.T.);
#32941=EDGE_CURVE('',#26348,#26350,#12069,.T.);
#32942=EDGE_CURVE('',#26351,#26347,#12070,.T.);
#32943=EDGE_CURVE('',#26351,#26352,#12071,.T.);
#32944=EDGE_CURVE('',#26352,#26349,#12072,.T.);
#32945=EDGE_CURVE('',#26353,#26351,#12073,.T.);
#32946=EDGE_CURVE('',#26353,#26354,#12074,.T.);
#32947=EDGE_CURVE('',#26354,#26352,#12075,.T.);
#32948=EDGE_CURVE('',#26348,#26353,#12076,.T.);
#32949=EDGE_CURVE('',#26350,#26354,#12077,.T.);
#32950=EDGE_CURVE('',#26355,#26356,#12078,.T.);
#32951=EDGE_CURVE('',#26355,#26357,#12079,.T.);
#32952=EDGE_CURVE('',#26357,#26358,#12080,.T.);
#32953=EDGE_CURVE('',#26356,#26358,#12081,.T.);
#32954=EDGE_CURVE('',#26359,#26355,#12082,.T.);
#32955=EDGE_CURVE('',#26359,#26360,#12083,.T.);
#32956=EDGE_CURVE('',#26360,#26357,#12084,.T.);
#32957=EDGE_CURVE('',#26361,#26359,#12085,.T.);
#32958=EDGE_CURVE('',#26361,#26362,#12086,.T.);
#32959=EDGE_CURVE('',#26362,#26360,#12087,.T.);
#32960=EDGE_CURVE('',#26356,#26361,#12088,.T.);
#32961=EDGE_CURVE('',#26358,#26362,#12089,.T.);
#32962=EDGE_CURVE('',#26363,#26364,#12090,.T.);
#32963=EDGE_CURVE('',#26363,#26365,#12091,.T.);
#32964=EDGE_CURVE('',#26365,#26366,#12092,.T.);
#32965=EDGE_CURVE('',#26364,#26366,#12093,.T.);
#32966=EDGE_CURVE('',#26367,#26363,#12094,.T.);
#32967=EDGE_CURVE('',#26367,#26368,#12095,.T.);
#32968=EDGE_CURVE('',#26368,#26365,#12096,.T.);
#32969=EDGE_CURVE('',#26369,#26367,#12097,.T.);
#32970=EDGE_CURVE('',#26369,#26370,#12098,.T.);
#32971=EDGE_CURVE('',#26370,#26368,#12099,.T.);
#32972=EDGE_CURVE('',#26364,#26369,#12100,.T.);
#32973=EDGE_CURVE('',#26366,#26370,#12101,.T.);
#32974=EDGE_CURVE('',#26371,#26372,#12102,.T.);
#32975=EDGE_CURVE('',#26371,#26373,#12103,.T.);
#32976=EDGE_CURVE('',#26373,#26374,#12104,.T.);
#32977=EDGE_CURVE('',#26372,#26374,#12105,.T.);
#32978=EDGE_CURVE('',#26375,#26371,#12106,.T.);
#32979=EDGE_CURVE('',#26375,#26376,#12107,.T.);
#32980=EDGE_CURVE('',#26376,#26373,#12108,.T.);
#32981=EDGE_CURVE('',#26377,#26375,#12109,.T.);
#32982=EDGE_CURVE('',#26377,#26378,#12110,.T.);
#32983=EDGE_CURVE('',#26378,#26376,#12111,.T.);
#32984=EDGE_CURVE('',#26372,#26377,#12112,.T.);
#32985=EDGE_CURVE('',#26374,#26378,#12113,.T.);
#32986=EDGE_CURVE('',#26379,#26380,#12114,.T.);
#32987=EDGE_CURVE('',#26379,#26381,#12115,.T.);
#32988=EDGE_CURVE('',#26381,#26382,#12116,.T.);
#32989=EDGE_CURVE('',#26380,#26382,#12117,.T.);
#32990=EDGE_CURVE('',#26383,#26379,#12118,.T.);
#32991=EDGE_CURVE('',#26383,#26384,#12119,.T.);
#32992=EDGE_CURVE('',#26384,#26381,#12120,.T.);
#32993=EDGE_CURVE('',#26385,#26383,#12121,.T.);
#32994=EDGE_CURVE('',#26385,#26386,#12122,.T.);
#32995=EDGE_CURVE('',#26386,#26384,#12123,.T.);
#32996=EDGE_CURVE('',#26380,#26385,#12124,.T.);
#32997=EDGE_CURVE('',#26382,#26386,#12125,.T.);
#32998=EDGE_CURVE('',#26387,#26388,#12126,.T.);
#32999=EDGE_CURVE('',#26387,#26389,#12127,.T.);
#33000=EDGE_CURVE('',#26389,#26390,#12128,.T.);
#33001=EDGE_CURVE('',#26388,#26390,#12129,.T.);
#33002=EDGE_CURVE('',#26391,#26387,#12130,.T.);
#33003=EDGE_CURVE('',#26391,#26392,#12131,.T.);
#33004=EDGE_CURVE('',#26392,#26389,#12132,.T.);
#33005=EDGE_CURVE('',#26393,#26391,#12133,.T.);
#33006=EDGE_CURVE('',#26393,#26394,#12134,.T.);
#33007=EDGE_CURVE('',#26394,#26392,#12135,.T.);
#33008=EDGE_CURVE('',#26388,#26393,#12136,.T.);
#33009=EDGE_CURVE('',#26390,#26394,#12137,.T.);
#33010=EDGE_CURVE('',#26395,#26396,#12138,.T.);
#33011=EDGE_CURVE('',#26395,#26397,#12139,.T.);
#33012=EDGE_CURVE('',#26397,#26398,#12140,.T.);
#33013=EDGE_CURVE('',#26396,#26398,#12141,.T.);
#33014=EDGE_CURVE('',#26399,#26395,#12142,.T.);
#33015=EDGE_CURVE('',#26399,#26400,#12143,.T.);
#33016=EDGE_CURVE('',#26400,#26397,#12144,.T.);
#33017=EDGE_CURVE('',#26401,#26399,#12145,.T.);
#33018=EDGE_CURVE('',#26401,#26402,#12146,.T.);
#33019=EDGE_CURVE('',#26402,#26400,#12147,.T.);
#33020=EDGE_CURVE('',#26396,#26401,#12148,.T.);
#33021=EDGE_CURVE('',#26398,#26402,#12149,.T.);
#33022=EDGE_CURVE('',#26403,#26404,#12150,.T.);
#33023=EDGE_CURVE('',#26403,#26405,#12151,.T.);
#33024=EDGE_CURVE('',#26405,#26406,#12152,.T.);
#33025=EDGE_CURVE('',#26404,#26406,#12153,.T.);
#33026=EDGE_CURVE('',#26407,#26403,#12154,.T.);
#33027=EDGE_CURVE('',#26407,#26408,#12155,.T.);
#33028=EDGE_CURVE('',#26408,#26405,#12156,.T.);
#33029=EDGE_CURVE('',#26409,#26407,#12157,.T.);
#33030=EDGE_CURVE('',#26409,#26410,#12158,.T.);
#33031=EDGE_CURVE('',#26410,#26408,#12159,.T.);
#33032=EDGE_CURVE('',#26404,#26409,#12160,.T.);
#33033=EDGE_CURVE('',#26406,#26410,#12161,.T.);
#33034=EDGE_CURVE('',#26411,#26412,#12162,.T.);
#33035=EDGE_CURVE('',#26411,#26413,#12163,.T.);
#33036=EDGE_CURVE('',#26413,#26414,#12164,.T.);
#33037=EDGE_CURVE('',#26412,#26414,#12165,.T.);
#33038=EDGE_CURVE('',#26415,#26411,#12166,.T.);
#33039=EDGE_CURVE('',#26415,#26416,#12167,.T.);
#33040=EDGE_CURVE('',#26416,#26413,#12168,.T.);
#33041=EDGE_CURVE('',#26417,#26415,#12169,.T.);
#33042=EDGE_CURVE('',#26417,#26418,#12170,.T.);
#33043=EDGE_CURVE('',#26418,#26416,#12171,.T.);
#33044=EDGE_CURVE('',#26412,#26417,#12172,.T.);
#33045=EDGE_CURVE('',#26414,#26418,#12173,.T.);
#33046=EDGE_CURVE('',#26419,#26420,#12174,.T.);
#33047=EDGE_CURVE('',#26419,#26421,#12175,.T.);
#33048=EDGE_CURVE('',#26421,#26422,#12176,.T.);
#33049=EDGE_CURVE('',#26420,#26422,#12177,.T.);
#33050=EDGE_CURVE('',#26423,#26419,#12178,.T.);
#33051=EDGE_CURVE('',#26423,#26424,#12179,.T.);
#33052=EDGE_CURVE('',#26424,#26421,#12180,.T.);
#33053=EDGE_CURVE('',#26425,#26423,#12181,.T.);
#33054=EDGE_CURVE('',#26425,#26426,#12182,.T.);
#33055=EDGE_CURVE('',#26426,#26424,#12183,.T.);
#33056=EDGE_CURVE('',#26420,#26425,#12184,.T.);
#33057=EDGE_CURVE('',#26422,#26426,#12185,.T.);
#33058=EDGE_CURVE('',#26427,#26428,#12186,.T.);
#33059=EDGE_CURVE('',#26427,#26429,#12187,.T.);
#33060=EDGE_CURVE('',#26429,#26430,#12188,.T.);
#33061=EDGE_CURVE('',#26428,#26430,#12189,.T.);
#33062=EDGE_CURVE('',#26431,#26427,#12190,.T.);
#33063=EDGE_CURVE('',#26431,#26432,#12191,.T.);
#33064=EDGE_CURVE('',#26432,#26429,#12192,.T.);
#33065=EDGE_CURVE('',#26433,#26431,#12193,.T.);
#33066=EDGE_CURVE('',#26433,#26434,#12194,.T.);
#33067=EDGE_CURVE('',#26434,#26432,#12195,.T.);
#33068=EDGE_CURVE('',#26428,#26433,#12196,.T.);
#33069=EDGE_CURVE('',#26430,#26434,#12197,.T.);
#33070=EDGE_CURVE('',#26435,#26436,#12198,.T.);
#33071=EDGE_CURVE('',#26435,#26437,#12199,.T.);
#33072=EDGE_CURVE('',#26437,#26438,#12200,.T.);
#33073=EDGE_CURVE('',#26436,#26438,#12201,.T.);
#33074=EDGE_CURVE('',#26439,#26435,#12202,.T.);
#33075=EDGE_CURVE('',#26439,#26440,#12203,.T.);
#33076=EDGE_CURVE('',#26440,#26437,#12204,.T.);
#33077=EDGE_CURVE('',#26441,#26439,#12205,.T.);
#33078=EDGE_CURVE('',#26441,#26442,#12206,.T.);
#33079=EDGE_CURVE('',#26442,#26440,#12207,.T.);
#33080=EDGE_CURVE('',#26436,#26441,#12208,.T.);
#33081=EDGE_CURVE('',#26438,#26442,#12209,.T.);
#33082=EDGE_CURVE('',#26443,#26444,#12210,.T.);
#33083=EDGE_CURVE('',#26443,#26445,#12211,.T.);
#33084=EDGE_CURVE('',#26445,#26446,#12212,.T.);
#33085=EDGE_CURVE('',#26444,#26446,#12213,.T.);
#33086=EDGE_CURVE('',#26447,#26443,#12214,.T.);
#33087=EDGE_CURVE('',#26447,#26448,#12215,.T.);
#33088=EDGE_CURVE('',#26448,#26445,#12216,.T.);
#33089=EDGE_CURVE('',#26449,#26447,#12217,.T.);
#33090=EDGE_CURVE('',#26449,#26450,#12218,.T.);
#33091=EDGE_CURVE('',#26450,#26448,#12219,.T.);
#33092=EDGE_CURVE('',#26444,#26449,#12220,.T.);
#33093=EDGE_CURVE('',#26446,#26450,#12221,.T.);
#33094=EDGE_CURVE('',#26451,#26452,#12222,.T.);
#33095=EDGE_CURVE('',#26451,#26453,#12223,.T.);
#33096=EDGE_CURVE('',#26453,#26454,#12224,.T.);
#33097=EDGE_CURVE('',#26452,#26454,#12225,.T.);
#33098=EDGE_CURVE('',#26455,#26451,#12226,.T.);
#33099=EDGE_CURVE('',#26455,#26456,#12227,.T.);
#33100=EDGE_CURVE('',#26456,#26453,#12228,.T.);
#33101=EDGE_CURVE('',#26457,#26455,#12229,.T.);
#33102=EDGE_CURVE('',#26457,#26458,#12230,.T.);
#33103=EDGE_CURVE('',#26458,#26456,#12231,.T.);
#33104=EDGE_CURVE('',#26452,#26457,#12232,.T.);
#33105=EDGE_CURVE('',#26454,#26458,#12233,.T.);
#33106=EDGE_CURVE('',#26459,#26460,#12234,.T.);
#33107=EDGE_CURVE('',#26459,#26461,#12235,.T.);
#33108=EDGE_CURVE('',#26461,#26462,#12236,.T.);
#33109=EDGE_CURVE('',#26460,#26462,#12237,.T.);
#33110=EDGE_CURVE('',#26463,#26459,#12238,.T.);
#33111=EDGE_CURVE('',#26463,#26464,#12239,.T.);
#33112=EDGE_CURVE('',#26464,#26461,#12240,.T.);
#33113=EDGE_CURVE('',#26465,#26463,#12241,.T.);
#33114=EDGE_CURVE('',#26465,#26466,#12242,.T.);
#33115=EDGE_CURVE('',#26466,#26464,#12243,.T.);
#33116=EDGE_CURVE('',#26460,#26465,#12244,.T.);
#33117=EDGE_CURVE('',#26462,#26466,#12245,.T.);
#33118=EDGE_CURVE('',#26467,#26468,#12246,.T.);
#33119=EDGE_CURVE('',#26467,#26469,#12247,.T.);
#33120=EDGE_CURVE('',#26469,#26470,#12248,.T.);
#33121=EDGE_CURVE('',#26468,#26470,#12249,.T.);
#33122=EDGE_CURVE('',#26471,#26467,#12250,.T.);
#33123=EDGE_CURVE('',#26471,#26472,#12251,.T.);
#33124=EDGE_CURVE('',#26472,#26469,#12252,.T.);
#33125=EDGE_CURVE('',#26473,#26471,#12253,.T.);
#33126=EDGE_CURVE('',#26473,#26474,#12254,.T.);
#33127=EDGE_CURVE('',#26474,#26472,#12255,.T.);
#33128=EDGE_CURVE('',#26468,#26473,#12256,.T.);
#33129=EDGE_CURVE('',#26470,#26474,#12257,.T.);
#33130=EDGE_CURVE('',#26475,#26476,#12258,.T.);
#33131=EDGE_CURVE('',#26475,#26477,#12259,.T.);
#33132=EDGE_CURVE('',#26477,#26478,#12260,.T.);
#33133=EDGE_CURVE('',#26476,#26478,#12261,.T.);
#33134=EDGE_CURVE('',#26479,#26475,#12262,.T.);
#33135=EDGE_CURVE('',#26479,#26480,#12263,.T.);
#33136=EDGE_CURVE('',#26480,#26477,#12264,.T.);
#33137=EDGE_CURVE('',#26481,#26479,#12265,.T.);
#33138=EDGE_CURVE('',#26481,#26482,#12266,.T.);
#33139=EDGE_CURVE('',#26482,#26480,#12267,.T.);
#33140=EDGE_CURVE('',#26476,#26481,#12268,.T.);
#33141=EDGE_CURVE('',#26478,#26482,#12269,.T.);
#33142=EDGE_CURVE('',#26483,#26484,#12270,.T.);
#33143=EDGE_CURVE('',#26483,#26485,#12271,.T.);
#33144=EDGE_CURVE('',#26485,#26486,#12272,.T.);
#33145=EDGE_CURVE('',#26484,#26486,#12273,.T.);
#33146=EDGE_CURVE('',#26487,#26483,#12274,.T.);
#33147=EDGE_CURVE('',#26487,#26488,#12275,.T.);
#33148=EDGE_CURVE('',#26488,#26485,#12276,.T.);
#33149=EDGE_CURVE('',#26489,#26487,#12277,.T.);
#33150=EDGE_CURVE('',#26489,#26490,#12278,.T.);
#33151=EDGE_CURVE('',#26490,#26488,#12279,.T.);
#33152=EDGE_CURVE('',#26484,#26489,#12280,.T.);
#33153=EDGE_CURVE('',#26486,#26490,#12281,.T.);
#33154=EDGE_CURVE('',#26491,#26492,#12282,.T.);
#33155=EDGE_CURVE('',#26491,#26493,#12283,.T.);
#33156=EDGE_CURVE('',#26493,#26494,#12284,.T.);
#33157=EDGE_CURVE('',#26492,#26494,#12285,.T.);
#33158=EDGE_CURVE('',#26495,#26491,#12286,.T.);
#33159=EDGE_CURVE('',#26495,#26496,#12287,.T.);
#33160=EDGE_CURVE('',#26496,#26493,#12288,.T.);
#33161=EDGE_CURVE('',#26497,#26495,#12289,.T.);
#33162=EDGE_CURVE('',#26497,#26498,#12290,.T.);
#33163=EDGE_CURVE('',#26498,#26496,#12291,.T.);
#33164=EDGE_CURVE('',#26492,#26497,#12292,.T.);
#33165=EDGE_CURVE('',#26494,#26498,#12293,.T.);
#33166=EDGE_CURVE('',#26499,#26500,#12294,.T.);
#33167=EDGE_CURVE('',#26499,#26501,#12295,.T.);
#33168=EDGE_CURVE('',#26501,#26502,#12296,.T.);
#33169=EDGE_CURVE('',#26500,#26502,#12297,.T.);
#33170=EDGE_CURVE('',#26503,#26499,#12298,.T.);
#33171=EDGE_CURVE('',#26503,#26504,#12299,.T.);
#33172=EDGE_CURVE('',#26504,#26501,#12300,.T.);
#33173=EDGE_CURVE('',#26505,#26503,#12301,.T.);
#33174=EDGE_CURVE('',#26505,#26506,#12302,.T.);
#33175=EDGE_CURVE('',#26506,#26504,#12303,.T.);
#33176=EDGE_CURVE('',#26500,#26505,#12304,.T.);
#33177=EDGE_CURVE('',#26502,#26506,#12305,.T.);
#33178=EDGE_CURVE('',#26507,#26508,#12306,.T.);
#33179=EDGE_CURVE('',#26507,#26509,#12307,.T.);
#33180=EDGE_CURVE('',#26509,#26510,#12308,.T.);
#33181=EDGE_CURVE('',#26508,#26510,#12309,.T.);
#33182=EDGE_CURVE('',#26511,#26507,#12310,.T.);
#33183=EDGE_CURVE('',#26511,#26512,#12311,.T.);
#33184=EDGE_CURVE('',#26512,#26509,#12312,.T.);
#33185=EDGE_CURVE('',#26513,#26511,#12313,.T.);
#33186=EDGE_CURVE('',#26513,#26514,#12314,.T.);
#33187=EDGE_CURVE('',#26514,#26512,#12315,.T.);
#33188=EDGE_CURVE('',#26508,#26513,#12316,.T.);
#33189=EDGE_CURVE('',#26510,#26514,#12317,.T.);
#33190=EDGE_CURVE('',#26515,#26516,#12318,.T.);
#33191=EDGE_CURVE('',#26515,#26517,#12319,.T.);
#33192=EDGE_CURVE('',#26517,#26518,#12320,.T.);
#33193=EDGE_CURVE('',#26516,#26518,#12321,.T.);
#33194=EDGE_CURVE('',#26519,#26515,#12322,.T.);
#33195=EDGE_CURVE('',#26519,#26520,#12323,.T.);
#33196=EDGE_CURVE('',#26520,#26517,#12324,.T.);
#33197=EDGE_CURVE('',#26521,#26519,#12325,.T.);
#33198=EDGE_CURVE('',#26521,#26522,#12326,.T.);
#33199=EDGE_CURVE('',#26522,#26520,#12327,.T.);
#33200=EDGE_CURVE('',#26516,#26521,#12328,.T.);
#33201=EDGE_CURVE('',#26518,#26522,#12329,.T.);
#33202=EDGE_CURVE('',#26523,#26524,#12330,.T.);
#33203=EDGE_CURVE('',#26523,#26525,#12331,.T.);
#33204=EDGE_CURVE('',#26525,#26526,#12332,.T.);
#33205=EDGE_CURVE('',#26524,#26526,#12333,.T.);
#33206=EDGE_CURVE('',#26527,#26523,#12334,.T.);
#33207=EDGE_CURVE('',#26527,#26528,#12335,.T.);
#33208=EDGE_CURVE('',#26528,#26525,#12336,.T.);
#33209=EDGE_CURVE('',#26529,#26527,#12337,.T.);
#33210=EDGE_CURVE('',#26529,#26530,#12338,.T.);
#33211=EDGE_CURVE('',#26530,#26528,#12339,.T.);
#33212=EDGE_CURVE('',#26524,#26529,#12340,.T.);
#33213=EDGE_CURVE('',#26526,#26530,#12341,.T.);
#33214=EDGE_CURVE('',#26531,#26532,#12342,.T.);
#33215=EDGE_CURVE('',#26531,#26533,#12343,.T.);
#33216=EDGE_CURVE('',#26533,#26534,#12344,.T.);
#33217=EDGE_CURVE('',#26532,#26534,#12345,.T.);
#33218=EDGE_CURVE('',#26535,#26531,#12346,.T.);
#33219=EDGE_CURVE('',#26535,#26536,#12347,.T.);
#33220=EDGE_CURVE('',#26536,#26533,#12348,.T.);
#33221=EDGE_CURVE('',#26537,#26535,#12349,.T.);
#33222=EDGE_CURVE('',#26537,#26538,#12350,.T.);
#33223=EDGE_CURVE('',#26538,#26536,#12351,.T.);
#33224=EDGE_CURVE('',#26532,#26537,#12352,.T.);
#33225=EDGE_CURVE('',#26534,#26538,#12353,.T.);
#33226=EDGE_CURVE('',#26539,#26540,#12354,.T.);
#33227=EDGE_CURVE('',#26539,#26541,#12355,.T.);
#33228=EDGE_CURVE('',#26541,#26542,#12356,.T.);
#33229=EDGE_CURVE('',#26540,#26542,#12357,.T.);
#33230=EDGE_CURVE('',#26543,#26539,#12358,.T.);
#33231=EDGE_CURVE('',#26543,#26544,#12359,.T.);
#33232=EDGE_CURVE('',#26544,#26541,#12360,.T.);
#33233=EDGE_CURVE('',#26545,#26543,#12361,.T.);
#33234=EDGE_CURVE('',#26545,#26546,#12362,.T.);
#33235=EDGE_CURVE('',#26546,#26544,#12363,.T.);
#33236=EDGE_CURVE('',#26540,#26545,#12364,.T.);
#33237=EDGE_CURVE('',#26542,#26546,#12365,.T.);
#33238=EDGE_CURVE('',#26547,#26548,#12366,.T.);
#33239=EDGE_CURVE('',#26547,#26549,#12367,.T.);
#33240=EDGE_CURVE('',#26549,#26550,#12368,.T.);
#33241=EDGE_CURVE('',#26548,#26550,#12369,.T.);
#33242=EDGE_CURVE('',#26551,#26547,#12370,.T.);
#33243=EDGE_CURVE('',#26551,#26552,#12371,.T.);
#33244=EDGE_CURVE('',#26552,#26549,#12372,.T.);
#33245=EDGE_CURVE('',#26553,#26551,#12373,.T.);
#33246=EDGE_CURVE('',#26553,#26554,#12374,.T.);
#33247=EDGE_CURVE('',#26554,#26552,#12375,.T.);
#33248=EDGE_CURVE('',#26548,#26553,#12376,.T.);
#33249=EDGE_CURVE('',#26550,#26554,#12377,.T.);
#33250=EDGE_CURVE('',#26555,#26556,#12378,.T.);
#33251=EDGE_CURVE('',#26555,#26557,#12379,.T.);
#33252=EDGE_CURVE('',#26557,#26558,#12380,.T.);
#33253=EDGE_CURVE('',#26556,#26558,#12381,.T.);
#33254=EDGE_CURVE('',#26559,#26555,#12382,.T.);
#33255=EDGE_CURVE('',#26559,#26560,#12383,.T.);
#33256=EDGE_CURVE('',#26560,#26557,#12384,.T.);
#33257=EDGE_CURVE('',#26561,#26559,#12385,.T.);
#33258=EDGE_CURVE('',#26561,#26562,#12386,.T.);
#33259=EDGE_CURVE('',#26562,#26560,#12387,.T.);
#33260=EDGE_CURVE('',#26556,#26561,#12388,.T.);
#33261=EDGE_CURVE('',#26558,#26562,#12389,.T.);
#33262=EDGE_CURVE('',#26563,#26564,#12390,.T.);
#33263=EDGE_CURVE('',#26563,#26565,#12391,.T.);
#33264=EDGE_CURVE('',#26565,#26566,#12392,.T.);
#33265=EDGE_CURVE('',#26564,#26566,#12393,.T.);
#33266=EDGE_CURVE('',#26567,#26563,#12394,.T.);
#33267=EDGE_CURVE('',#26567,#26568,#12395,.T.);
#33268=EDGE_CURVE('',#26568,#26565,#12396,.T.);
#33269=EDGE_CURVE('',#26569,#26567,#12397,.T.);
#33270=EDGE_CURVE('',#26569,#26570,#12398,.T.);
#33271=EDGE_CURVE('',#26570,#26568,#12399,.T.);
#33272=EDGE_CURVE('',#26564,#26569,#12400,.T.);
#33273=EDGE_CURVE('',#26566,#26570,#12401,.T.);
#33274=EDGE_CURVE('',#26571,#26572,#12402,.T.);
#33275=EDGE_CURVE('',#26571,#26573,#12403,.T.);
#33276=EDGE_CURVE('',#26573,#26574,#12404,.T.);
#33277=EDGE_CURVE('',#26572,#26574,#12405,.T.);
#33278=EDGE_CURVE('',#26575,#26571,#12406,.T.);
#33279=EDGE_CURVE('',#26575,#26576,#12407,.T.);
#33280=EDGE_CURVE('',#26576,#26573,#12408,.T.);
#33281=EDGE_CURVE('',#26577,#26575,#12409,.T.);
#33282=EDGE_CURVE('',#26577,#26578,#12410,.T.);
#33283=EDGE_CURVE('',#26578,#26576,#12411,.T.);
#33284=EDGE_CURVE('',#26572,#26577,#12412,.T.);
#33285=EDGE_CURVE('',#26574,#26578,#12413,.T.);
#33286=EDGE_CURVE('',#26579,#26580,#12414,.T.);
#33287=EDGE_CURVE('',#26579,#26581,#12415,.T.);
#33288=EDGE_CURVE('',#26581,#26582,#12416,.T.);
#33289=EDGE_CURVE('',#26580,#26582,#12417,.T.);
#33290=EDGE_CURVE('',#26583,#26579,#12418,.T.);
#33291=EDGE_CURVE('',#26583,#26584,#12419,.T.);
#33292=EDGE_CURVE('',#26584,#26581,#12420,.T.);
#33293=EDGE_CURVE('',#26585,#26583,#12421,.T.);
#33294=EDGE_CURVE('',#26585,#26586,#12422,.T.);
#33295=EDGE_CURVE('',#26586,#26584,#12423,.T.);
#33296=EDGE_CURVE('',#26580,#26585,#12424,.T.);
#33297=EDGE_CURVE('',#26582,#26586,#12425,.T.);
#33298=EDGE_CURVE('',#26587,#26588,#12426,.T.);
#33299=EDGE_CURVE('',#26587,#26589,#12427,.T.);
#33300=EDGE_CURVE('',#26589,#26590,#12428,.T.);
#33301=EDGE_CURVE('',#26588,#26590,#12429,.T.);
#33302=EDGE_CURVE('',#26591,#26587,#12430,.T.);
#33303=EDGE_CURVE('',#26591,#26592,#12431,.T.);
#33304=EDGE_CURVE('',#26592,#26589,#12432,.T.);
#33305=EDGE_CURVE('',#26593,#26591,#12433,.T.);
#33306=EDGE_CURVE('',#26593,#26594,#12434,.T.);
#33307=EDGE_CURVE('',#26594,#26592,#12435,.T.);
#33308=EDGE_CURVE('',#26588,#26593,#12436,.T.);
#33309=EDGE_CURVE('',#26590,#26594,#12437,.T.);
#33310=EDGE_CURVE('',#26595,#26596,#12438,.T.);
#33311=EDGE_CURVE('',#26595,#26597,#12439,.T.);
#33312=EDGE_CURVE('',#26597,#26598,#12440,.T.);
#33313=EDGE_CURVE('',#26596,#26598,#12441,.T.);
#33314=EDGE_CURVE('',#26599,#26595,#12442,.T.);
#33315=EDGE_CURVE('',#26599,#26600,#12443,.T.);
#33316=EDGE_CURVE('',#26600,#26597,#12444,.T.);
#33317=EDGE_CURVE('',#26601,#26599,#12445,.T.);
#33318=EDGE_CURVE('',#26601,#26602,#12446,.T.);
#33319=EDGE_CURVE('',#26602,#26600,#12447,.T.);
#33320=EDGE_CURVE('',#26596,#26601,#12448,.T.);
#33321=EDGE_CURVE('',#26598,#26602,#12449,.T.);
#33322=EDGE_CURVE('',#26603,#26604,#12450,.T.);
#33323=EDGE_CURVE('',#26603,#26605,#12451,.T.);
#33324=EDGE_CURVE('',#26605,#26606,#12452,.T.);
#33325=EDGE_CURVE('',#26604,#26606,#12453,.T.);
#33326=EDGE_CURVE('',#26607,#26603,#12454,.T.);
#33327=EDGE_CURVE('',#26607,#26608,#12455,.T.);
#33328=EDGE_CURVE('',#26608,#26605,#12456,.T.);
#33329=EDGE_CURVE('',#26609,#26607,#12457,.T.);
#33330=EDGE_CURVE('',#26609,#26610,#12458,.T.);
#33331=EDGE_CURVE('',#26610,#26608,#12459,.T.);
#33332=EDGE_CURVE('',#26604,#26609,#12460,.T.);
#33333=EDGE_CURVE('',#26606,#26610,#12461,.T.);
#33334=EDGE_CURVE('',#26611,#26612,#12462,.T.);
#33335=EDGE_CURVE('',#26611,#26613,#12463,.T.);
#33336=EDGE_CURVE('',#26613,#26614,#12464,.T.);
#33337=EDGE_CURVE('',#26612,#26614,#12465,.T.);
#33338=EDGE_CURVE('',#26615,#26611,#12466,.T.);
#33339=EDGE_CURVE('',#26615,#26616,#12467,.T.);
#33340=EDGE_CURVE('',#26616,#26613,#12468,.T.);
#33341=EDGE_CURVE('',#26617,#26615,#12469,.T.);
#33342=EDGE_CURVE('',#26617,#26618,#12470,.T.);
#33343=EDGE_CURVE('',#26618,#26616,#12471,.T.);
#33344=EDGE_CURVE('',#26612,#26617,#12472,.T.);
#33345=EDGE_CURVE('',#26614,#26618,#12473,.T.);
#33346=EDGE_CURVE('',#26619,#26620,#12474,.T.);
#33347=EDGE_CURVE('',#26619,#26621,#12475,.T.);
#33348=EDGE_CURVE('',#26621,#26622,#12476,.T.);
#33349=EDGE_CURVE('',#26620,#26622,#12477,.T.);
#33350=EDGE_CURVE('',#26623,#26619,#12478,.T.);
#33351=EDGE_CURVE('',#26623,#26624,#12479,.T.);
#33352=EDGE_CURVE('',#26624,#26621,#12480,.T.);
#33353=EDGE_CURVE('',#26625,#26623,#12481,.T.);
#33354=EDGE_CURVE('',#26625,#26626,#12482,.T.);
#33355=EDGE_CURVE('',#26626,#26624,#12483,.T.);
#33356=EDGE_CURVE('',#26620,#26625,#12484,.T.);
#33357=EDGE_CURVE('',#26622,#26626,#12485,.T.);
#33358=EDGE_CURVE('',#26627,#26628,#12486,.T.);
#33359=EDGE_CURVE('',#26627,#26629,#12487,.T.);
#33360=EDGE_CURVE('',#26629,#26630,#12488,.T.);
#33361=EDGE_CURVE('',#26628,#26630,#12489,.T.);
#33362=EDGE_CURVE('',#26631,#26627,#12490,.T.);
#33363=EDGE_CURVE('',#26631,#26632,#12491,.T.);
#33364=EDGE_CURVE('',#26632,#26629,#12492,.T.);
#33365=EDGE_CURVE('',#26633,#26631,#12493,.T.);
#33366=EDGE_CURVE('',#26633,#26634,#12494,.T.);
#33367=EDGE_CURVE('',#26634,#26632,#12495,.T.);
#33368=EDGE_CURVE('',#26628,#26633,#12496,.T.);
#33369=EDGE_CURVE('',#26630,#26634,#12497,.T.);
#33370=EDGE_CURVE('',#26635,#26636,#12498,.T.);
#33371=EDGE_CURVE('',#26635,#26637,#12499,.T.);
#33372=EDGE_CURVE('',#26637,#26638,#12500,.T.);
#33373=EDGE_CURVE('',#26636,#26638,#12501,.T.);
#33374=EDGE_CURVE('',#26639,#26635,#12502,.T.);
#33375=EDGE_CURVE('',#26639,#26640,#12503,.T.);
#33376=EDGE_CURVE('',#26640,#26637,#12504,.T.);
#33377=EDGE_CURVE('',#26641,#26639,#12505,.T.);
#33378=EDGE_CURVE('',#26641,#26642,#12506,.T.);
#33379=EDGE_CURVE('',#26642,#26640,#12507,.T.);
#33380=EDGE_CURVE('',#26636,#26641,#12508,.T.);
#33381=EDGE_CURVE('',#26638,#26642,#12509,.T.);
#33382=EDGE_CURVE('',#26643,#26644,#12510,.T.);
#33383=EDGE_CURVE('',#26643,#26645,#12511,.T.);
#33384=EDGE_CURVE('',#26645,#26646,#12512,.T.);
#33385=EDGE_CURVE('',#26644,#26646,#12513,.T.);
#33386=EDGE_CURVE('',#26647,#26643,#12514,.T.);
#33387=EDGE_CURVE('',#26647,#26648,#12515,.T.);
#33388=EDGE_CURVE('',#26648,#26645,#12516,.T.);
#33389=EDGE_CURVE('',#26649,#26647,#12517,.T.);
#33390=EDGE_CURVE('',#26649,#26650,#12518,.T.);
#33391=EDGE_CURVE('',#26650,#26648,#12519,.T.);
#33392=EDGE_CURVE('',#26644,#26649,#12520,.T.);
#33393=EDGE_CURVE('',#26646,#26650,#12521,.T.);
#33394=EDGE_CURVE('',#26651,#26652,#12522,.T.);
#33395=EDGE_CURVE('',#26651,#26653,#12523,.T.);
#33396=EDGE_CURVE('',#26653,#26654,#12524,.T.);
#33397=EDGE_CURVE('',#26652,#26654,#12525,.T.);
#33398=EDGE_CURVE('',#26655,#26651,#12526,.T.);
#33399=EDGE_CURVE('',#26655,#26656,#12527,.T.);
#33400=EDGE_CURVE('',#26656,#26653,#12528,.T.);
#33401=EDGE_CURVE('',#26657,#26655,#12529,.T.);
#33402=EDGE_CURVE('',#26657,#26658,#12530,.T.);
#33403=EDGE_CURVE('',#26658,#26656,#12531,.T.);
#33404=EDGE_CURVE('',#26652,#26657,#12532,.T.);
#33405=EDGE_CURVE('',#26654,#26658,#12533,.T.);
#33406=EDGE_CURVE('',#26659,#26660,#12534,.T.);
#33407=EDGE_CURVE('',#26659,#26661,#12535,.T.);
#33408=EDGE_CURVE('',#26661,#26662,#12536,.T.);
#33409=EDGE_CURVE('',#26660,#26662,#12537,.T.);
#33410=EDGE_CURVE('',#26663,#26659,#12538,.T.);
#33411=EDGE_CURVE('',#26663,#26664,#12539,.T.);
#33412=EDGE_CURVE('',#26664,#26661,#12540,.T.);
#33413=EDGE_CURVE('',#26665,#26663,#12541,.T.);
#33414=EDGE_CURVE('',#26665,#26666,#12542,.T.);
#33415=EDGE_CURVE('',#26666,#26664,#12543,.T.);
#33416=EDGE_CURVE('',#26660,#26665,#12544,.T.);
#33417=EDGE_CURVE('',#26662,#26666,#12545,.T.);
#33418=EDGE_CURVE('',#26667,#26668,#12546,.T.);
#33419=EDGE_CURVE('',#26667,#26669,#12547,.T.);
#33420=EDGE_CURVE('',#26669,#26670,#12548,.T.);
#33421=EDGE_CURVE('',#26668,#26670,#12549,.T.);
#33422=EDGE_CURVE('',#26671,#26667,#12550,.T.);
#33423=EDGE_CURVE('',#26671,#26672,#12551,.T.);
#33424=EDGE_CURVE('',#26672,#26669,#12552,.T.);
#33425=EDGE_CURVE('',#26673,#26671,#12553,.T.);
#33426=EDGE_CURVE('',#26673,#26674,#12554,.T.);
#33427=EDGE_CURVE('',#26674,#26672,#12555,.T.);
#33428=EDGE_CURVE('',#26668,#26673,#12556,.T.);
#33429=EDGE_CURVE('',#26670,#26674,#12557,.T.);
#33430=EDGE_CURVE('',#26675,#26676,#12558,.T.);
#33431=EDGE_CURVE('',#26675,#26677,#12559,.T.);
#33432=EDGE_CURVE('',#26677,#26678,#12560,.T.);
#33433=EDGE_CURVE('',#26676,#26678,#12561,.T.);
#33434=EDGE_CURVE('',#26679,#26675,#12562,.T.);
#33435=EDGE_CURVE('',#26679,#26680,#12563,.T.);
#33436=EDGE_CURVE('',#26680,#26677,#12564,.T.);
#33437=EDGE_CURVE('',#26681,#26679,#12565,.T.);
#33438=EDGE_CURVE('',#26681,#26682,#12566,.T.);
#33439=EDGE_CURVE('',#26682,#26680,#12567,.T.);
#33440=EDGE_CURVE('',#26676,#26681,#12568,.T.);
#33441=EDGE_CURVE('',#26678,#26682,#12569,.T.);
#33442=EDGE_CURVE('',#26683,#26684,#12570,.T.);
#33443=EDGE_CURVE('',#26683,#26685,#12571,.T.);
#33444=EDGE_CURVE('',#26685,#26686,#12572,.T.);
#33445=EDGE_CURVE('',#26684,#26686,#12573,.T.);
#33446=EDGE_CURVE('',#26687,#26683,#12574,.T.);
#33447=EDGE_CURVE('',#26687,#26688,#12575,.T.);
#33448=EDGE_CURVE('',#26688,#26685,#12576,.T.);
#33449=EDGE_CURVE('',#26689,#26687,#12577,.T.);
#33450=EDGE_CURVE('',#26689,#26690,#12578,.T.);
#33451=EDGE_CURVE('',#26690,#26688,#12579,.T.);
#33452=EDGE_CURVE('',#26684,#26689,#12580,.T.);
#33453=EDGE_CURVE('',#26686,#26690,#12581,.T.);
#33454=EDGE_CURVE('',#26691,#26692,#12582,.T.);
#33455=EDGE_CURVE('',#26691,#26693,#12583,.T.);
#33456=EDGE_CURVE('',#26693,#26694,#12584,.T.);
#33457=EDGE_CURVE('',#26692,#26694,#12585,.T.);
#33458=EDGE_CURVE('',#26695,#26691,#12586,.T.);
#33459=EDGE_CURVE('',#26695,#26696,#12587,.T.);
#33460=EDGE_CURVE('',#26696,#26693,#12588,.T.);
#33461=EDGE_CURVE('',#26697,#26695,#12589,.T.);
#33462=EDGE_CURVE('',#26697,#26698,#12590,.T.);
#33463=EDGE_CURVE('',#26698,#26696,#12591,.T.);
#33464=EDGE_CURVE('',#26692,#26697,#12592,.T.);
#33465=EDGE_CURVE('',#26694,#26698,#12593,.T.);
#33466=EDGE_CURVE('',#26699,#26700,#12594,.T.);
#33467=EDGE_CURVE('',#26699,#26701,#12595,.T.);
#33468=EDGE_CURVE('',#26701,#26702,#12596,.T.);
#33469=EDGE_CURVE('',#26700,#26702,#12597,.T.);
#33470=EDGE_CURVE('',#26703,#26699,#12598,.T.);
#33471=EDGE_CURVE('',#26703,#26704,#12599,.T.);
#33472=EDGE_CURVE('',#26704,#26701,#12600,.T.);
#33473=EDGE_CURVE('',#26705,#26703,#12601,.T.);
#33474=EDGE_CURVE('',#26705,#26706,#12602,.T.);
#33475=EDGE_CURVE('',#26706,#26704,#12603,.T.);
#33476=EDGE_CURVE('',#26700,#26705,#12604,.T.);
#33477=EDGE_CURVE('',#26702,#26706,#12605,.T.);
#33478=EDGE_CURVE('',#26707,#26708,#12606,.T.);
#33479=EDGE_CURVE('',#26707,#26709,#12607,.T.);
#33480=EDGE_CURVE('',#26709,#26710,#12608,.T.);
#33481=EDGE_CURVE('',#26708,#26710,#12609,.T.);
#33482=EDGE_CURVE('',#26711,#26707,#12610,.T.);
#33483=EDGE_CURVE('',#26711,#26712,#12611,.T.);
#33484=EDGE_CURVE('',#26712,#26709,#12612,.T.);
#33485=EDGE_CURVE('',#26713,#26711,#12613,.T.);
#33486=EDGE_CURVE('',#26713,#26714,#12614,.T.);
#33487=EDGE_CURVE('',#26714,#26712,#12615,.T.);
#33488=EDGE_CURVE('',#26708,#26713,#12616,.T.);
#33489=EDGE_CURVE('',#26710,#26714,#12617,.T.);
#33490=EDGE_CURVE('',#26715,#26716,#12618,.T.);
#33491=EDGE_CURVE('',#26715,#26717,#12619,.T.);
#33492=EDGE_CURVE('',#26717,#26718,#12620,.T.);
#33493=EDGE_CURVE('',#26716,#26718,#12621,.T.);
#33494=EDGE_CURVE('',#26719,#26715,#12622,.T.);
#33495=EDGE_CURVE('',#26719,#26720,#12623,.T.);
#33496=EDGE_CURVE('',#26720,#26717,#12624,.T.);
#33497=EDGE_CURVE('',#26721,#26719,#12625,.T.);
#33498=EDGE_CURVE('',#26721,#26722,#12626,.T.);
#33499=EDGE_CURVE('',#26722,#26720,#12627,.T.);
#33500=EDGE_CURVE('',#26716,#26721,#12628,.T.);
#33501=EDGE_CURVE('',#26718,#26722,#12629,.T.);
#33502=EDGE_CURVE('',#26723,#26724,#12630,.T.);
#33503=EDGE_CURVE('',#26723,#26725,#12631,.T.);
#33504=EDGE_CURVE('',#26725,#26726,#12632,.T.);
#33505=EDGE_CURVE('',#26724,#26726,#12633,.T.);
#33506=EDGE_CURVE('',#26727,#26723,#12634,.T.);
#33507=EDGE_CURVE('',#26727,#26728,#12635,.T.);
#33508=EDGE_CURVE('',#26728,#26725,#12636,.T.);
#33509=EDGE_CURVE('',#26729,#26727,#12637,.T.);
#33510=EDGE_CURVE('',#26729,#26730,#12638,.T.);
#33511=EDGE_CURVE('',#26730,#26728,#12639,.T.);
#33512=EDGE_CURVE('',#26724,#26729,#12640,.T.);
#33513=EDGE_CURVE('',#26726,#26730,#12641,.T.);
#33514=EDGE_CURVE('',#26731,#26732,#12642,.T.);
#33515=EDGE_CURVE('',#26731,#26733,#12643,.T.);
#33516=EDGE_CURVE('',#26733,#26734,#12644,.T.);
#33517=EDGE_CURVE('',#26732,#26734,#12645,.T.);
#33518=EDGE_CURVE('',#26735,#26731,#12646,.T.);
#33519=EDGE_CURVE('',#26735,#26736,#12647,.T.);
#33520=EDGE_CURVE('',#26736,#26733,#12648,.T.);
#33521=EDGE_CURVE('',#26737,#26735,#12649,.T.);
#33522=EDGE_CURVE('',#26737,#26738,#12650,.T.);
#33523=EDGE_CURVE('',#26738,#26736,#12651,.T.);
#33524=EDGE_CURVE('',#26732,#26737,#12652,.T.);
#33525=EDGE_CURVE('',#26734,#26738,#12653,.T.);
#33526=EDGE_CURVE('',#26739,#26740,#12654,.T.);
#33527=EDGE_CURVE('',#26739,#26741,#12655,.T.);
#33528=EDGE_CURVE('',#26741,#26742,#12656,.T.);
#33529=EDGE_CURVE('',#26740,#26742,#12657,.T.);
#33530=EDGE_CURVE('',#26743,#26739,#12658,.T.);
#33531=EDGE_CURVE('',#26743,#26744,#12659,.T.);
#33532=EDGE_CURVE('',#26744,#26741,#12660,.T.);
#33533=EDGE_CURVE('',#26745,#26743,#12661,.T.);
#33534=EDGE_CURVE('',#26745,#26746,#12662,.T.);
#33535=EDGE_CURVE('',#26746,#26744,#12663,.T.);
#33536=EDGE_CURVE('',#26740,#26745,#12664,.T.);
#33537=EDGE_CURVE('',#26742,#26746,#12665,.T.);
#33538=EDGE_CURVE('',#26747,#26748,#12666,.T.);
#33539=EDGE_CURVE('',#26747,#26749,#12667,.T.);
#33540=EDGE_CURVE('',#26749,#26750,#12668,.T.);
#33541=EDGE_CURVE('',#26748,#26750,#12669,.T.);
#33542=EDGE_CURVE('',#26751,#26747,#12670,.T.);
#33543=EDGE_CURVE('',#26751,#26752,#12671,.T.);
#33544=EDGE_CURVE('',#26752,#26749,#12672,.T.);
#33545=EDGE_CURVE('',#26753,#26751,#12673,.T.);
#33546=EDGE_CURVE('',#26753,#26754,#12674,.T.);
#33547=EDGE_CURVE('',#26754,#26752,#12675,.T.);
#33548=EDGE_CURVE('',#26748,#26753,#12676,.T.);
#33549=EDGE_CURVE('',#26750,#26754,#12677,.T.);
#33550=EDGE_CURVE('',#26755,#26756,#12678,.T.);
#33551=EDGE_CURVE('',#26755,#26757,#12679,.T.);
#33552=EDGE_CURVE('',#26757,#26758,#12680,.T.);
#33553=EDGE_CURVE('',#26756,#26758,#12681,.T.);
#33554=EDGE_CURVE('',#26759,#26755,#12682,.T.);
#33555=EDGE_CURVE('',#26759,#26760,#12683,.T.);
#33556=EDGE_CURVE('',#26760,#26757,#12684,.T.);
#33557=EDGE_CURVE('',#26761,#26759,#12685,.T.);
#33558=EDGE_CURVE('',#26761,#26762,#12686,.T.);
#33559=EDGE_CURVE('',#26762,#26760,#12687,.T.);
#33560=EDGE_CURVE('',#26756,#26761,#12688,.T.);
#33561=EDGE_CURVE('',#26758,#26762,#12689,.T.);
#33562=EDGE_CURVE('',#26763,#26764,#12690,.T.);
#33563=EDGE_CURVE('',#26763,#26765,#12691,.T.);
#33564=EDGE_CURVE('',#26765,#26766,#12692,.T.);
#33565=EDGE_CURVE('',#26764,#26766,#12693,.T.);
#33566=EDGE_CURVE('',#26767,#26763,#12694,.T.);
#33567=EDGE_CURVE('',#26767,#26768,#12695,.T.);
#33568=EDGE_CURVE('',#26768,#26765,#12696,.T.);
#33569=EDGE_CURVE('',#26769,#26767,#12697,.T.);
#33570=EDGE_CURVE('',#26769,#26770,#12698,.T.);
#33571=EDGE_CURVE('',#26770,#26768,#12699,.T.);
#33572=EDGE_CURVE('',#26764,#26769,#12700,.T.);
#33573=EDGE_CURVE('',#26766,#26770,#12701,.T.);
#33574=EDGE_CURVE('',#26771,#26772,#12702,.T.);
#33575=EDGE_CURVE('',#26771,#26773,#12703,.T.);
#33576=EDGE_CURVE('',#26773,#26774,#12704,.T.);
#33577=EDGE_CURVE('',#26772,#26774,#12705,.T.);
#33578=EDGE_CURVE('',#26775,#26771,#12706,.T.);
#33579=EDGE_CURVE('',#26775,#26776,#12707,.T.);
#33580=EDGE_CURVE('',#26776,#26773,#12708,.T.);
#33581=EDGE_CURVE('',#26777,#26775,#12709,.T.);
#33582=EDGE_CURVE('',#26777,#26778,#12710,.T.);
#33583=EDGE_CURVE('',#26778,#26776,#12711,.T.);
#33584=EDGE_CURVE('',#26772,#26777,#12712,.T.);
#33585=EDGE_CURVE('',#26774,#26778,#12713,.T.);
#33586=EDGE_CURVE('',#26779,#26780,#12714,.T.);
#33587=EDGE_CURVE('',#26779,#26781,#12715,.T.);
#33588=EDGE_CURVE('',#26781,#26782,#12716,.T.);
#33589=EDGE_CURVE('',#26780,#26782,#12717,.T.);
#33590=EDGE_CURVE('',#26783,#26779,#12718,.T.);
#33591=EDGE_CURVE('',#26783,#26784,#12719,.T.);
#33592=EDGE_CURVE('',#26784,#26781,#12720,.T.);
#33593=EDGE_CURVE('',#26785,#26783,#12721,.T.);
#33594=EDGE_CURVE('',#26785,#26786,#12722,.T.);
#33595=EDGE_CURVE('',#26786,#26784,#12723,.T.);
#33596=EDGE_CURVE('',#26780,#26785,#12724,.T.);
#33597=EDGE_CURVE('',#26782,#26786,#12725,.T.);
#33598=EDGE_CURVE('',#26787,#26788,#12726,.T.);
#33599=EDGE_CURVE('',#26787,#26789,#12727,.T.);
#33600=EDGE_CURVE('',#26789,#26790,#12728,.T.);
#33601=EDGE_CURVE('',#26788,#26790,#12729,.T.);
#33602=EDGE_CURVE('',#26791,#26787,#12730,.T.);
#33603=EDGE_CURVE('',#26791,#26792,#12731,.T.);
#33604=EDGE_CURVE('',#26792,#26789,#12732,.T.);
#33605=EDGE_CURVE('',#26793,#26791,#12733,.T.);
#33606=EDGE_CURVE('',#26793,#26794,#12734,.T.);
#33607=EDGE_CURVE('',#26794,#26792,#12735,.T.);
#33608=EDGE_CURVE('',#26788,#26793,#12736,.T.);
#33609=EDGE_CURVE('',#26790,#26794,#12737,.T.);
#33610=EDGE_CURVE('',#26795,#26796,#12738,.T.);
#33611=EDGE_CURVE('',#26795,#26797,#12739,.T.);
#33612=EDGE_CURVE('',#26797,#26798,#12740,.T.);
#33613=EDGE_CURVE('',#26796,#26798,#12741,.T.);
#33614=EDGE_CURVE('',#26799,#26795,#12742,.T.);
#33615=EDGE_CURVE('',#26799,#26800,#12743,.T.);
#33616=EDGE_CURVE('',#26800,#26797,#12744,.T.);
#33617=EDGE_CURVE('',#26801,#26799,#12745,.T.);
#33618=EDGE_CURVE('',#26801,#26802,#12746,.T.);
#33619=EDGE_CURVE('',#26802,#26800,#12747,.T.);
#33620=EDGE_CURVE('',#26796,#26801,#12748,.T.);
#33621=EDGE_CURVE('',#26798,#26802,#12749,.T.);
#33622=EDGE_CURVE('',#26803,#26804,#12750,.T.);
#33623=EDGE_CURVE('',#26803,#26805,#12751,.T.);
#33624=EDGE_CURVE('',#26805,#26806,#12752,.T.);
#33625=EDGE_CURVE('',#26804,#26806,#12753,.T.);
#33626=EDGE_CURVE('',#26807,#26803,#12754,.T.);
#33627=EDGE_CURVE('',#26807,#26808,#12755,.T.);
#33628=EDGE_CURVE('',#26808,#26805,#12756,.T.);
#33629=EDGE_CURVE('',#26809,#26807,#12757,.T.);
#33630=EDGE_CURVE('',#26809,#26810,#12758,.T.);
#33631=EDGE_CURVE('',#26810,#26808,#12759,.T.);
#33632=EDGE_CURVE('',#26804,#26809,#12760,.T.);
#33633=EDGE_CURVE('',#26806,#26810,#12761,.T.);
#33634=EDGE_CURVE('',#26811,#26812,#12762,.T.);
#33635=EDGE_CURVE('',#26811,#26813,#12763,.T.);
#33636=EDGE_CURVE('',#26813,#26814,#12764,.T.);
#33637=EDGE_CURVE('',#26812,#26814,#12765,.T.);
#33638=EDGE_CURVE('',#26815,#26811,#12766,.T.);
#33639=EDGE_CURVE('',#26815,#26816,#12767,.T.);
#33640=EDGE_CURVE('',#26816,#26813,#12768,.T.);
#33641=EDGE_CURVE('',#26817,#26815,#12769,.T.);
#33642=EDGE_CURVE('',#26817,#26818,#12770,.T.);
#33643=EDGE_CURVE('',#26818,#26816,#12771,.T.);
#33644=EDGE_CURVE('',#26812,#26817,#12772,.T.);
#33645=EDGE_CURVE('',#26814,#26818,#12773,.T.);
#33646=EDGE_CURVE('',#26819,#26820,#12774,.T.);
#33647=EDGE_CURVE('',#26819,#26821,#12775,.T.);
#33648=EDGE_CURVE('',#26821,#26822,#12776,.T.);
#33649=EDGE_CURVE('',#26820,#26822,#12777,.T.);
#33650=EDGE_CURVE('',#26823,#26819,#12778,.T.);
#33651=EDGE_CURVE('',#26823,#26824,#12779,.T.);
#33652=EDGE_CURVE('',#26824,#26821,#12780,.T.);
#33653=EDGE_CURVE('',#26825,#26823,#12781,.T.);
#33654=EDGE_CURVE('',#26825,#26826,#12782,.T.);
#33655=EDGE_CURVE('',#26826,#26824,#12783,.T.);
#33656=EDGE_CURVE('',#26820,#26825,#12784,.T.);
#33657=EDGE_CURVE('',#26822,#26826,#12785,.T.);
#33658=EDGE_CURVE('',#26827,#26828,#12786,.T.);
#33659=EDGE_CURVE('',#26827,#26829,#12787,.T.);
#33660=EDGE_CURVE('',#26829,#26830,#12788,.T.);
#33661=EDGE_CURVE('',#26828,#26830,#12789,.T.);
#33662=EDGE_CURVE('',#26831,#26827,#12790,.T.);
#33663=EDGE_CURVE('',#26831,#26832,#12791,.T.);
#33664=EDGE_CURVE('',#26832,#26829,#12792,.T.);
#33665=EDGE_CURVE('',#26833,#26831,#12793,.T.);
#33666=EDGE_CURVE('',#26833,#26834,#12794,.T.);
#33667=EDGE_CURVE('',#26834,#26832,#12795,.T.);
#33668=EDGE_CURVE('',#26828,#26833,#12796,.T.);
#33669=EDGE_CURVE('',#26830,#26834,#12797,.T.);
#33670=EDGE_CURVE('',#26835,#26836,#12798,.T.);
#33671=EDGE_CURVE('',#26835,#26837,#12799,.T.);
#33672=EDGE_CURVE('',#26837,#26838,#12800,.T.);
#33673=EDGE_CURVE('',#26836,#26838,#12801,.T.);
#33674=EDGE_CURVE('',#26839,#26835,#12802,.T.);
#33675=EDGE_CURVE('',#26839,#26840,#12803,.T.);
#33676=EDGE_CURVE('',#26840,#26837,#12804,.T.);
#33677=EDGE_CURVE('',#26841,#26839,#12805,.T.);
#33678=EDGE_CURVE('',#26841,#26842,#12806,.T.);
#33679=EDGE_CURVE('',#26842,#26840,#12807,.T.);
#33680=EDGE_CURVE('',#26836,#26841,#12808,.T.);
#33681=EDGE_CURVE('',#26838,#26842,#12809,.T.);
#33682=EDGE_CURVE('',#26843,#26844,#12810,.T.);
#33683=EDGE_CURVE('',#26843,#26845,#12811,.T.);
#33684=EDGE_CURVE('',#26845,#26846,#12812,.T.);
#33685=EDGE_CURVE('',#26844,#26846,#12813,.T.);
#33686=EDGE_CURVE('',#26847,#26843,#12814,.T.);
#33687=EDGE_CURVE('',#26847,#26848,#12815,.T.);
#33688=EDGE_CURVE('',#26848,#26845,#12816,.T.);
#33689=EDGE_CURVE('',#26849,#26847,#12817,.T.);
#33690=EDGE_CURVE('',#26849,#26850,#12818,.T.);
#33691=EDGE_CURVE('',#26850,#26848,#12819,.T.);
#33692=EDGE_CURVE('',#26844,#26849,#12820,.T.);
#33693=EDGE_CURVE('',#26846,#26850,#12821,.T.);
#33694=EDGE_CURVE('',#26851,#26852,#12822,.T.);
#33695=EDGE_CURVE('',#26851,#26853,#12823,.T.);
#33696=EDGE_CURVE('',#26853,#26854,#12824,.T.);
#33697=EDGE_CURVE('',#26852,#26854,#12825,.T.);
#33698=EDGE_CURVE('',#26855,#26851,#12826,.T.);
#33699=EDGE_CURVE('',#26855,#26856,#12827,.T.);
#33700=EDGE_CURVE('',#26856,#26853,#12828,.T.);
#33701=EDGE_CURVE('',#26857,#26855,#12829,.T.);
#33702=EDGE_CURVE('',#26857,#26858,#12830,.T.);
#33703=EDGE_CURVE('',#26858,#26856,#12831,.T.);
#33704=EDGE_CURVE('',#26852,#26857,#12832,.T.);
#33705=EDGE_CURVE('',#26854,#26858,#12833,.T.);
#33706=EDGE_CURVE('',#26859,#26860,#12834,.T.);
#33707=EDGE_CURVE('',#26859,#26861,#12835,.T.);
#33708=EDGE_CURVE('',#26861,#26862,#12836,.T.);
#33709=EDGE_CURVE('',#26860,#26862,#12837,.T.);
#33710=EDGE_CURVE('',#26863,#26859,#12838,.T.);
#33711=EDGE_CURVE('',#26863,#26864,#12839,.T.);
#33712=EDGE_CURVE('',#26864,#26861,#12840,.T.);
#33713=EDGE_CURVE('',#26865,#26863,#12841,.T.);
#33714=EDGE_CURVE('',#26865,#26866,#12842,.T.);
#33715=EDGE_CURVE('',#26866,#26864,#12843,.T.);
#33716=EDGE_CURVE('',#26860,#26865,#12844,.T.);
#33717=EDGE_CURVE('',#26862,#26866,#12845,.T.);
#33718=EDGE_CURVE('',#26867,#26868,#12846,.T.);
#33719=EDGE_CURVE('',#26867,#26869,#12847,.T.);
#33720=EDGE_CURVE('',#26869,#26870,#12848,.T.);
#33721=EDGE_CURVE('',#26868,#26870,#12849,.T.);
#33722=EDGE_CURVE('',#26871,#26867,#12850,.T.);
#33723=EDGE_CURVE('',#26871,#26872,#12851,.T.);
#33724=EDGE_CURVE('',#26872,#26869,#12852,.T.);
#33725=EDGE_CURVE('',#26873,#26871,#12853,.T.);
#33726=EDGE_CURVE('',#26873,#26874,#12854,.T.);
#33727=EDGE_CURVE('',#26874,#26872,#12855,.T.);
#33728=EDGE_CURVE('',#26868,#26873,#12856,.T.);
#33729=EDGE_CURVE('',#26870,#26874,#12857,.T.);
#33730=EDGE_CURVE('',#26875,#26876,#12858,.T.);
#33731=EDGE_CURVE('',#26875,#26877,#12859,.T.);
#33732=EDGE_CURVE('',#26877,#26878,#12860,.T.);
#33733=EDGE_CURVE('',#26876,#26878,#12861,.T.);
#33734=EDGE_CURVE('',#26879,#26875,#12862,.T.);
#33735=EDGE_CURVE('',#26879,#26880,#12863,.T.);
#33736=EDGE_CURVE('',#26880,#26877,#12864,.T.);
#33737=EDGE_CURVE('',#26881,#26879,#12865,.T.);
#33738=EDGE_CURVE('',#26881,#26882,#12866,.T.);
#33739=EDGE_CURVE('',#26882,#26880,#12867,.T.);
#33740=EDGE_CURVE('',#26876,#26881,#12868,.T.);
#33741=EDGE_CURVE('',#26878,#26882,#12869,.T.);
#33742=EDGE_CURVE('',#26883,#26884,#12870,.T.);
#33743=EDGE_CURVE('',#26883,#26885,#12871,.T.);
#33744=EDGE_CURVE('',#26885,#26886,#12872,.T.);
#33745=EDGE_CURVE('',#26884,#26886,#12873,.T.);
#33746=EDGE_CURVE('',#26887,#26883,#12874,.T.);
#33747=EDGE_CURVE('',#26887,#26888,#12875,.T.);
#33748=EDGE_CURVE('',#26888,#26885,#12876,.T.);
#33749=EDGE_CURVE('',#26889,#26887,#12877,.T.);
#33750=EDGE_CURVE('',#26889,#26890,#12878,.T.);
#33751=EDGE_CURVE('',#26890,#26888,#12879,.T.);
#33752=EDGE_CURVE('',#26884,#26889,#12880,.T.);
#33753=EDGE_CURVE('',#26886,#26890,#12881,.T.);
#33754=EDGE_CURVE('',#26891,#26892,#12882,.T.);
#33755=EDGE_CURVE('',#26891,#26893,#12883,.T.);
#33756=EDGE_CURVE('',#26893,#26894,#12884,.T.);
#33757=EDGE_CURVE('',#26892,#26894,#12885,.T.);
#33758=EDGE_CURVE('',#26895,#26891,#12886,.T.);
#33759=EDGE_CURVE('',#26895,#26896,#12887,.T.);
#33760=EDGE_CURVE('',#26896,#26893,#12888,.T.);
#33761=EDGE_CURVE('',#26897,#26895,#12889,.T.);
#33762=EDGE_CURVE('',#26897,#26898,#12890,.T.);
#33763=EDGE_CURVE('',#26898,#26896,#12891,.T.);
#33764=EDGE_CURVE('',#26892,#26897,#12892,.T.);
#33765=EDGE_CURVE('',#26894,#26898,#12893,.T.);
#33766=EDGE_CURVE('',#26899,#26900,#12894,.T.);
#33767=EDGE_CURVE('',#26899,#26901,#12895,.T.);
#33768=EDGE_CURVE('',#26901,#26902,#12896,.T.);
#33769=EDGE_CURVE('',#26900,#26902,#12897,.T.);
#33770=EDGE_CURVE('',#26903,#26899,#12898,.T.);
#33771=EDGE_CURVE('',#26903,#26904,#12899,.T.);
#33772=EDGE_CURVE('',#26904,#26901,#12900,.T.);
#33773=EDGE_CURVE('',#26905,#26903,#12901,.T.);
#33774=EDGE_CURVE('',#26905,#26906,#12902,.T.);
#33775=EDGE_CURVE('',#26906,#26904,#12903,.T.);
#33776=EDGE_CURVE('',#26900,#26905,#12904,.T.);
#33777=EDGE_CURVE('',#26902,#26906,#12905,.T.);
#33778=EDGE_CURVE('',#26907,#26908,#12906,.T.);
#33779=EDGE_CURVE('',#26907,#26909,#12907,.T.);
#33780=EDGE_CURVE('',#26909,#26910,#12908,.T.);
#33781=EDGE_CURVE('',#26908,#26910,#12909,.T.);
#33782=EDGE_CURVE('',#26911,#26907,#12910,.T.);
#33783=EDGE_CURVE('',#26911,#26912,#12911,.T.);
#33784=EDGE_CURVE('',#26912,#26909,#12912,.T.);
#33785=EDGE_CURVE('',#26913,#26911,#12913,.T.);
#33786=EDGE_CURVE('',#26913,#26914,#12914,.T.);
#33787=EDGE_CURVE('',#26914,#26912,#12915,.T.);
#33788=EDGE_CURVE('',#26908,#26913,#12916,.T.);
#33789=EDGE_CURVE('',#26910,#26914,#12917,.T.);
#33790=EDGE_CURVE('',#26915,#26916,#12918,.T.);
#33791=EDGE_CURVE('',#26915,#26917,#12919,.T.);
#33792=EDGE_CURVE('',#26917,#26918,#12920,.T.);
#33793=EDGE_CURVE('',#26916,#26918,#12921,.T.);
#33794=EDGE_CURVE('',#26919,#26915,#12922,.T.);
#33795=EDGE_CURVE('',#26919,#26920,#12923,.T.);
#33796=EDGE_CURVE('',#26920,#26917,#12924,.T.);
#33797=EDGE_CURVE('',#26921,#26919,#12925,.T.);
#33798=EDGE_CURVE('',#26921,#26922,#12926,.T.);
#33799=EDGE_CURVE('',#26922,#26920,#12927,.T.);
#33800=EDGE_CURVE('',#26916,#26921,#12928,.T.);
#33801=EDGE_CURVE('',#26918,#26922,#12929,.T.);
#33802=EDGE_CURVE('',#26923,#26924,#12930,.T.);
#33803=EDGE_CURVE('',#26923,#26925,#12931,.T.);
#33804=EDGE_CURVE('',#26925,#26926,#12932,.T.);
#33805=EDGE_CURVE('',#26924,#26926,#12933,.T.);
#33806=EDGE_CURVE('',#26927,#26923,#12934,.T.);
#33807=EDGE_CURVE('',#26927,#26928,#12935,.T.);
#33808=EDGE_CURVE('',#26928,#26925,#12936,.T.);
#33809=EDGE_CURVE('',#26929,#26927,#12937,.T.);
#33810=EDGE_CURVE('',#26929,#26930,#12938,.T.);
#33811=EDGE_CURVE('',#26930,#26928,#12939,.T.);
#33812=EDGE_CURVE('',#26924,#26929,#12940,.T.);
#33813=EDGE_CURVE('',#26926,#26930,#12941,.T.);
#33814=EDGE_CURVE('',#26931,#26932,#12942,.T.);
#33815=EDGE_CURVE('',#26931,#26933,#12943,.T.);
#33816=EDGE_CURVE('',#26933,#26934,#12944,.T.);
#33817=EDGE_CURVE('',#26932,#26934,#12945,.T.);
#33818=EDGE_CURVE('',#26935,#26931,#12946,.T.);
#33819=EDGE_CURVE('',#26935,#26936,#12947,.T.);
#33820=EDGE_CURVE('',#26936,#26933,#12948,.T.);
#33821=EDGE_CURVE('',#26937,#26935,#12949,.T.);
#33822=EDGE_CURVE('',#26937,#26938,#12950,.T.);
#33823=EDGE_CURVE('',#26938,#26936,#12951,.T.);
#33824=EDGE_CURVE('',#26932,#26937,#12952,.T.);
#33825=EDGE_CURVE('',#26934,#26938,#12953,.T.);
#33826=EDGE_CURVE('',#26939,#26940,#12954,.T.);
#33827=EDGE_CURVE('',#26939,#26941,#12955,.T.);
#33828=EDGE_CURVE('',#26941,#26942,#12956,.T.);
#33829=EDGE_CURVE('',#26940,#26942,#12957,.T.);
#33830=EDGE_CURVE('',#26943,#26939,#12958,.T.);
#33831=EDGE_CURVE('',#26943,#26944,#12959,.T.);
#33832=EDGE_CURVE('',#26944,#26941,#12960,.T.);
#33833=EDGE_CURVE('',#26945,#26943,#12961,.T.);
#33834=EDGE_CURVE('',#26945,#26946,#12962,.T.);
#33835=EDGE_CURVE('',#26946,#26944,#12963,.T.);
#33836=EDGE_CURVE('',#26940,#26945,#12964,.T.);
#33837=EDGE_CURVE('',#26942,#26946,#12965,.T.);
#33838=EDGE_CURVE('',#26947,#26948,#12966,.T.);
#33839=EDGE_CURVE('',#26947,#26949,#12967,.T.);
#33840=EDGE_CURVE('',#26949,#26950,#12968,.T.);
#33841=EDGE_CURVE('',#26948,#26950,#12969,.T.);
#33842=EDGE_CURVE('',#26951,#26947,#12970,.T.);
#33843=EDGE_CURVE('',#26951,#26952,#12971,.T.);
#33844=EDGE_CURVE('',#26952,#26949,#12972,.T.);
#33845=EDGE_CURVE('',#26953,#26951,#12973,.T.);
#33846=EDGE_CURVE('',#26953,#26954,#12974,.T.);
#33847=EDGE_CURVE('',#26954,#26952,#12975,.T.);
#33848=EDGE_CURVE('',#26948,#26953,#12976,.T.);
#33849=EDGE_CURVE('',#26950,#26954,#12977,.T.);
#33850=EDGE_CURVE('',#26955,#26956,#12978,.T.);
#33851=EDGE_CURVE('',#26955,#26957,#12979,.T.);
#33852=EDGE_CURVE('',#26957,#26958,#12980,.T.);
#33853=EDGE_CURVE('',#26956,#26958,#12981,.T.);
#33854=EDGE_CURVE('',#26959,#26955,#12982,.T.);
#33855=EDGE_CURVE('',#26959,#26960,#12983,.T.);
#33856=EDGE_CURVE('',#26960,#26957,#12984,.T.);
#33857=EDGE_CURVE('',#26961,#26959,#12985,.T.);
#33858=EDGE_CURVE('',#26961,#26962,#12986,.T.);
#33859=EDGE_CURVE('',#26962,#26960,#12987,.T.);
#33860=EDGE_CURVE('',#26956,#26961,#12988,.T.);
#33861=EDGE_CURVE('',#26958,#26962,#12989,.T.);
#33862=EDGE_CURVE('',#26963,#26964,#12990,.T.);
#33863=EDGE_CURVE('',#26963,#26965,#12991,.T.);
#33864=EDGE_CURVE('',#26965,#26966,#12992,.T.);
#33865=EDGE_CURVE('',#26964,#26966,#12993,.T.);
#33866=EDGE_CURVE('',#26967,#26963,#12994,.T.);
#33867=EDGE_CURVE('',#26967,#26968,#12995,.T.);
#33868=EDGE_CURVE('',#26968,#26965,#12996,.T.);
#33869=EDGE_CURVE('',#26969,#26967,#12997,.T.);
#33870=EDGE_CURVE('',#26969,#26970,#12998,.T.);
#33871=EDGE_CURVE('',#26970,#26968,#12999,.T.);
#33872=EDGE_CURVE('',#26964,#26969,#13000,.T.);
#33873=EDGE_CURVE('',#26966,#26970,#13001,.T.);
#33874=EDGE_CURVE('',#26971,#26972,#13002,.T.);
#33875=EDGE_CURVE('',#26971,#26973,#13003,.T.);
#33876=EDGE_CURVE('',#26973,#26974,#13004,.T.);
#33877=EDGE_CURVE('',#26972,#26974,#13005,.T.);
#33878=EDGE_CURVE('',#26975,#26971,#13006,.T.);
#33879=EDGE_CURVE('',#26975,#26976,#13007,.T.);
#33880=EDGE_CURVE('',#26976,#26973,#13008,.T.);
#33881=EDGE_CURVE('',#26977,#26975,#13009,.T.);
#33882=EDGE_CURVE('',#26977,#26978,#13010,.T.);
#33883=EDGE_CURVE('',#26978,#26976,#13011,.T.);
#33884=EDGE_CURVE('',#26972,#26977,#13012,.T.);
#33885=EDGE_CURVE('',#26974,#26978,#13013,.T.);
#33886=EDGE_CURVE('',#26979,#26980,#13014,.T.);
#33887=EDGE_CURVE('',#26979,#26981,#13015,.T.);
#33888=EDGE_CURVE('',#26981,#26982,#13016,.T.);
#33889=EDGE_CURVE('',#26980,#26982,#13017,.T.);
#33890=EDGE_CURVE('',#26983,#26979,#13018,.T.);
#33891=EDGE_CURVE('',#26983,#26984,#13019,.T.);
#33892=EDGE_CURVE('',#26984,#26981,#13020,.T.);
#33893=EDGE_CURVE('',#26985,#26983,#13021,.T.);
#33894=EDGE_CURVE('',#26985,#26986,#13022,.T.);
#33895=EDGE_CURVE('',#26986,#26984,#13023,.T.);
#33896=EDGE_CURVE('',#26980,#26985,#13024,.T.);
#33897=EDGE_CURVE('',#26982,#26986,#13025,.T.);
#33898=EDGE_CURVE('',#26987,#26988,#13026,.T.);
#33899=EDGE_CURVE('',#26987,#26989,#13027,.T.);
#33900=EDGE_CURVE('',#26989,#26990,#13028,.T.);
#33901=EDGE_CURVE('',#26988,#26990,#13029,.T.);
#33902=EDGE_CURVE('',#26991,#26987,#13030,.T.);
#33903=EDGE_CURVE('',#26991,#26992,#13031,.T.);
#33904=EDGE_CURVE('',#26992,#26989,#13032,.T.);
#33905=EDGE_CURVE('',#26993,#26991,#13033,.T.);
#33906=EDGE_CURVE('',#26993,#26994,#13034,.T.);
#33907=EDGE_CURVE('',#26994,#26992,#13035,.T.);
#33908=EDGE_CURVE('',#26988,#26993,#13036,.T.);
#33909=EDGE_CURVE('',#26990,#26994,#13037,.T.);
#33910=EDGE_CURVE('',#26995,#26996,#13038,.T.);
#33911=EDGE_CURVE('',#26995,#26997,#13039,.T.);
#33912=EDGE_CURVE('',#26997,#26998,#13040,.T.);
#33913=EDGE_CURVE('',#26996,#26998,#13041,.T.);
#33914=EDGE_CURVE('',#26999,#26995,#13042,.T.);
#33915=EDGE_CURVE('',#26999,#27000,#13043,.T.);
#33916=EDGE_CURVE('',#27000,#26997,#13044,.T.);
#33917=EDGE_CURVE('',#27001,#26999,#13045,.T.);
#33918=EDGE_CURVE('',#27001,#27002,#13046,.T.);
#33919=EDGE_CURVE('',#27002,#27000,#13047,.T.);
#33920=EDGE_CURVE('',#26996,#27001,#13048,.T.);
#33921=EDGE_CURVE('',#26998,#27002,#13049,.T.);
#33922=EDGE_CURVE('',#27003,#27004,#13050,.T.);
#33923=EDGE_CURVE('',#27003,#27005,#13051,.T.);
#33924=EDGE_CURVE('',#27005,#27006,#13052,.T.);
#33925=EDGE_CURVE('',#27004,#27006,#13053,.T.);
#33926=EDGE_CURVE('',#27007,#27003,#13054,.T.);
#33927=EDGE_CURVE('',#27007,#27008,#13055,.T.);
#33928=EDGE_CURVE('',#27008,#27005,#13056,.T.);
#33929=EDGE_CURVE('',#27009,#27007,#13057,.T.);
#33930=EDGE_CURVE('',#27009,#27010,#13058,.T.);
#33931=EDGE_CURVE('',#27010,#27008,#13059,.T.);
#33932=EDGE_CURVE('',#27004,#27009,#13060,.T.);
#33933=EDGE_CURVE('',#27006,#27010,#13061,.T.);
#33934=EDGE_CURVE('',#27011,#27012,#13062,.T.);
#33935=EDGE_CURVE('',#27011,#27013,#13063,.T.);
#33936=EDGE_CURVE('',#27013,#27014,#13064,.T.);
#33937=EDGE_CURVE('',#27012,#27014,#13065,.T.);
#33938=EDGE_CURVE('',#27015,#27011,#13066,.T.);
#33939=EDGE_CURVE('',#27015,#27016,#13067,.T.);
#33940=EDGE_CURVE('',#27016,#27013,#13068,.T.);
#33941=EDGE_CURVE('',#27017,#27015,#13069,.T.);
#33942=EDGE_CURVE('',#27017,#27018,#13070,.T.);
#33943=EDGE_CURVE('',#27018,#27016,#13071,.T.);
#33944=EDGE_CURVE('',#27012,#27017,#13072,.T.);
#33945=EDGE_CURVE('',#27014,#27018,#13073,.T.);
#33946=EDGE_CURVE('',#27019,#27020,#13074,.T.);
#33947=EDGE_CURVE('',#27019,#27021,#13075,.T.);
#33948=EDGE_CURVE('',#27021,#27022,#13076,.T.);
#33949=EDGE_CURVE('',#27020,#27022,#13077,.T.);
#33950=EDGE_CURVE('',#27023,#27019,#13078,.T.);
#33951=EDGE_CURVE('',#27023,#27024,#13079,.T.);
#33952=EDGE_CURVE('',#27024,#27021,#13080,.T.);
#33953=EDGE_CURVE('',#27025,#27023,#13081,.T.);
#33954=EDGE_CURVE('',#27025,#27026,#13082,.T.);
#33955=EDGE_CURVE('',#27026,#27024,#13083,.T.);
#33956=EDGE_CURVE('',#27020,#27025,#13084,.T.);
#33957=EDGE_CURVE('',#27022,#27026,#13085,.T.);
#33958=EDGE_CURVE('',#27027,#27028,#13086,.T.);
#33959=EDGE_CURVE('',#27027,#27029,#13087,.T.);
#33960=EDGE_CURVE('',#27029,#27030,#13088,.T.);
#33961=EDGE_CURVE('',#27028,#27030,#13089,.T.);
#33962=EDGE_CURVE('',#27031,#27027,#13090,.T.);
#33963=EDGE_CURVE('',#27031,#27032,#13091,.T.);
#33964=EDGE_CURVE('',#27032,#27029,#13092,.T.);
#33965=EDGE_CURVE('',#27033,#27031,#13093,.T.);
#33966=EDGE_CURVE('',#27033,#27034,#13094,.T.);
#33967=EDGE_CURVE('',#27034,#27032,#13095,.T.);
#33968=EDGE_CURVE('',#27028,#27033,#13096,.T.);
#33969=EDGE_CURVE('',#27030,#27034,#13097,.T.);
#33970=EDGE_CURVE('',#27035,#27036,#13098,.T.);
#33971=EDGE_CURVE('',#27035,#27037,#13099,.T.);
#33972=EDGE_CURVE('',#27037,#27038,#13100,.T.);
#33973=EDGE_CURVE('',#27036,#27038,#13101,.T.);
#33974=EDGE_CURVE('',#27039,#27035,#13102,.T.);
#33975=EDGE_CURVE('',#27039,#27040,#13103,.T.);
#33976=EDGE_CURVE('',#27040,#27037,#13104,.T.);
#33977=EDGE_CURVE('',#27041,#27039,#13105,.T.);
#33978=EDGE_CURVE('',#27041,#27042,#13106,.T.);
#33979=EDGE_CURVE('',#27042,#27040,#13107,.T.);
#33980=EDGE_CURVE('',#27036,#27041,#13108,.T.);
#33981=EDGE_CURVE('',#27038,#27042,#13109,.T.);
#33982=EDGE_CURVE('',#27043,#27044,#13110,.T.);
#33983=EDGE_CURVE('',#27043,#27045,#13111,.T.);
#33984=EDGE_CURVE('',#27045,#27046,#13112,.T.);
#33985=EDGE_CURVE('',#27044,#27046,#13113,.T.);
#33986=EDGE_CURVE('',#27047,#27043,#13114,.T.);
#33987=EDGE_CURVE('',#27047,#27048,#13115,.T.);
#33988=EDGE_CURVE('',#27048,#27045,#13116,.T.);
#33989=EDGE_CURVE('',#27049,#27047,#13117,.T.);
#33990=EDGE_CURVE('',#27049,#27050,#13118,.T.);
#33991=EDGE_CURVE('',#27050,#27048,#13119,.T.);
#33992=EDGE_CURVE('',#27044,#27049,#13120,.T.);
#33993=EDGE_CURVE('',#27046,#27050,#13121,.T.);
#33994=EDGE_CURVE('',#27051,#27052,#13122,.T.);
#33995=EDGE_CURVE('',#27051,#27053,#13123,.T.);
#33996=EDGE_CURVE('',#27053,#27054,#13124,.T.);
#33997=EDGE_CURVE('',#27052,#27054,#13125,.T.);
#33998=EDGE_CURVE('',#27055,#27051,#13126,.T.);
#33999=EDGE_CURVE('',#27055,#27056,#13127,.T.);
#34000=EDGE_CURVE('',#27056,#27053,#13128,.T.);
#34001=EDGE_CURVE('',#27057,#27055,#13129,.T.);
#34002=EDGE_CURVE('',#27057,#27058,#13130,.T.);
#34003=EDGE_CURVE('',#27058,#27056,#13131,.T.);
#34004=EDGE_CURVE('',#27052,#27057,#13132,.T.);
#34005=EDGE_CURVE('',#27054,#27058,#13133,.T.);
#34006=EDGE_CURVE('',#27059,#27060,#13134,.T.);
#34007=EDGE_CURVE('',#27059,#27061,#13135,.T.);
#34008=EDGE_CURVE('',#27061,#27062,#13136,.T.);
#34009=EDGE_CURVE('',#27060,#27062,#13137,.T.);
#34010=EDGE_CURVE('',#27063,#27059,#13138,.T.);
#34011=EDGE_CURVE('',#27063,#27064,#13139,.T.);
#34012=EDGE_CURVE('',#27064,#27061,#13140,.T.);
#34013=EDGE_CURVE('',#27065,#27063,#13141,.T.);
#34014=EDGE_CURVE('',#27065,#27066,#13142,.T.);
#34015=EDGE_CURVE('',#27066,#27064,#13143,.T.);
#34016=EDGE_CURVE('',#27060,#27065,#13144,.T.);
#34017=EDGE_CURVE('',#27062,#27066,#13145,.T.);
#34018=EDGE_CURVE('',#27067,#27068,#13146,.T.);
#34019=EDGE_CURVE('',#27067,#27069,#13147,.T.);
#34020=EDGE_CURVE('',#27069,#27070,#13148,.T.);
#34021=EDGE_CURVE('',#27068,#27070,#13149,.T.);
#34022=EDGE_CURVE('',#27071,#27067,#13150,.T.);
#34023=EDGE_CURVE('',#27071,#27072,#13151,.T.);
#34024=EDGE_CURVE('',#27072,#27069,#13152,.T.);
#34025=EDGE_CURVE('',#27073,#27071,#13153,.T.);
#34026=EDGE_CURVE('',#27073,#27074,#13154,.T.);
#34027=EDGE_CURVE('',#27074,#27072,#13155,.T.);
#34028=EDGE_CURVE('',#27068,#27073,#13156,.T.);
#34029=EDGE_CURVE('',#27070,#27074,#13157,.T.);
#34030=EDGE_CURVE('',#27075,#27076,#13158,.T.);
#34031=EDGE_CURVE('',#27075,#27077,#13159,.T.);
#34032=EDGE_CURVE('',#27077,#27078,#13160,.T.);
#34033=EDGE_CURVE('',#27076,#27078,#13161,.T.);
#34034=EDGE_CURVE('',#27079,#27075,#13162,.T.);
#34035=EDGE_CURVE('',#27079,#27080,#13163,.T.);
#34036=EDGE_CURVE('',#27080,#27077,#13164,.T.);
#34037=EDGE_CURVE('',#27081,#27079,#13165,.T.);
#34038=EDGE_CURVE('',#27081,#27082,#13166,.T.);
#34039=EDGE_CURVE('',#27082,#27080,#13167,.T.);
#34040=EDGE_CURVE('',#27076,#27081,#13168,.T.);
#34041=EDGE_CURVE('',#27078,#27082,#13169,.T.);
#34042=EDGE_CURVE('',#27083,#27084,#13170,.T.);
#34043=EDGE_CURVE('',#27083,#27085,#13171,.T.);
#34044=EDGE_CURVE('',#27085,#27086,#13172,.T.);
#34045=EDGE_CURVE('',#27084,#27086,#13173,.T.);
#34046=EDGE_CURVE('',#27087,#27083,#13174,.T.);
#34047=EDGE_CURVE('',#27087,#27088,#13175,.T.);
#34048=EDGE_CURVE('',#27088,#27085,#13176,.T.);
#34049=EDGE_CURVE('',#27089,#27087,#13177,.T.);
#34050=EDGE_CURVE('',#27089,#27090,#13178,.T.);
#34051=EDGE_CURVE('',#27090,#27088,#13179,.T.);
#34052=EDGE_CURVE('',#27084,#27089,#13180,.T.);
#34053=EDGE_CURVE('',#27086,#27090,#13181,.T.);
#34054=EDGE_CURVE('',#27091,#27092,#13182,.T.);
#34055=EDGE_CURVE('',#27091,#27093,#13183,.T.);
#34056=EDGE_CURVE('',#27093,#27094,#13184,.T.);
#34057=EDGE_CURVE('',#27092,#27094,#13185,.T.);
#34058=EDGE_CURVE('',#27095,#27091,#13186,.T.);
#34059=EDGE_CURVE('',#27095,#27096,#13187,.T.);
#34060=EDGE_CURVE('',#27096,#27093,#13188,.T.);
#34061=EDGE_CURVE('',#27097,#27095,#13189,.T.);
#34062=EDGE_CURVE('',#27097,#27098,#13190,.T.);
#34063=EDGE_CURVE('',#27098,#27096,#13191,.T.);
#34064=EDGE_CURVE('',#27092,#27097,#13192,.T.);
#34065=EDGE_CURVE('',#27094,#27098,#13193,.T.);
#34066=EDGE_CURVE('',#27099,#27100,#13194,.T.);
#34067=EDGE_CURVE('',#27099,#27101,#13195,.T.);
#34068=EDGE_CURVE('',#27101,#27102,#13196,.T.);
#34069=EDGE_CURVE('',#27100,#27102,#13197,.T.);
#34070=EDGE_CURVE('',#27103,#27099,#13198,.T.);
#34071=EDGE_CURVE('',#27103,#27104,#13199,.T.);
#34072=EDGE_CURVE('',#27104,#27101,#13200,.T.);
#34073=EDGE_CURVE('',#27105,#27103,#13201,.T.);
#34074=EDGE_CURVE('',#27105,#27106,#13202,.T.);
#34075=EDGE_CURVE('',#27106,#27104,#13203,.T.);
#34076=EDGE_CURVE('',#27100,#27105,#13204,.T.);
#34077=EDGE_CURVE('',#27102,#27106,#13205,.T.);
#34078=EDGE_CURVE('',#27107,#27108,#13206,.T.);
#34079=EDGE_CURVE('',#27107,#27109,#13207,.T.);
#34080=EDGE_CURVE('',#27109,#27110,#13208,.T.);
#34081=EDGE_CURVE('',#27108,#27110,#13209,.T.);
#34082=EDGE_CURVE('',#27111,#27107,#13210,.T.);
#34083=EDGE_CURVE('',#27111,#27112,#13211,.T.);
#34084=EDGE_CURVE('',#27112,#27109,#13212,.T.);
#34085=EDGE_CURVE('',#27113,#27111,#13213,.T.);
#34086=EDGE_CURVE('',#27113,#27114,#13214,.T.);
#34087=EDGE_CURVE('',#27114,#27112,#13215,.T.);
#34088=EDGE_CURVE('',#27108,#27113,#13216,.T.);
#34089=EDGE_CURVE('',#27110,#27114,#13217,.T.);
#34090=EDGE_CURVE('',#27115,#27116,#13218,.T.);
#34091=EDGE_CURVE('',#27115,#27117,#13219,.T.);
#34092=EDGE_CURVE('',#27117,#27118,#13220,.T.);
#34093=EDGE_CURVE('',#27116,#27118,#13221,.T.);
#34094=EDGE_CURVE('',#27119,#27115,#13222,.T.);
#34095=EDGE_CURVE('',#27119,#27120,#13223,.T.);
#34096=EDGE_CURVE('',#27120,#27117,#13224,.T.);
#34097=EDGE_CURVE('',#27121,#27119,#13225,.T.);
#34098=EDGE_CURVE('',#27121,#27122,#13226,.T.);
#34099=EDGE_CURVE('',#27122,#27120,#13227,.T.);
#34100=EDGE_CURVE('',#27116,#27121,#13228,.T.);
#34101=EDGE_CURVE('',#27118,#27122,#13229,.T.);
#34102=EDGE_CURVE('',#27123,#27124,#13230,.T.);
#34103=EDGE_CURVE('',#27123,#27125,#13231,.T.);
#34104=EDGE_CURVE('',#27125,#27126,#13232,.T.);
#34105=EDGE_CURVE('',#27124,#27126,#13233,.T.);
#34106=EDGE_CURVE('',#27127,#27123,#13234,.T.);
#34107=EDGE_CURVE('',#27127,#27128,#13235,.T.);
#34108=EDGE_CURVE('',#27128,#27125,#13236,.T.);
#34109=EDGE_CURVE('',#27129,#27127,#13237,.T.);
#34110=EDGE_CURVE('',#27129,#27130,#13238,.T.);
#34111=EDGE_CURVE('',#27130,#27128,#13239,.T.);
#34112=EDGE_CURVE('',#27124,#27129,#13240,.T.);
#34113=EDGE_CURVE('',#27126,#27130,#13241,.T.);
#34114=EDGE_CURVE('',#27131,#27132,#13242,.T.);
#34115=EDGE_CURVE('',#27131,#27133,#13243,.T.);
#34116=EDGE_CURVE('',#27133,#27134,#13244,.T.);
#34117=EDGE_CURVE('',#27132,#27134,#13245,.T.);
#34118=EDGE_CURVE('',#27135,#27131,#13246,.T.);
#34119=EDGE_CURVE('',#27135,#27136,#13247,.T.);
#34120=EDGE_CURVE('',#27136,#27133,#13248,.T.);
#34121=EDGE_CURVE('',#27137,#27135,#13249,.T.);
#34122=EDGE_CURVE('',#27137,#27138,#13250,.T.);
#34123=EDGE_CURVE('',#27138,#27136,#13251,.T.);
#34124=EDGE_CURVE('',#27132,#27137,#13252,.T.);
#34125=EDGE_CURVE('',#27134,#27138,#13253,.T.);
#34126=EDGE_CURVE('',#27139,#27140,#13254,.T.);
#34127=EDGE_CURVE('',#27139,#27141,#13255,.T.);
#34128=EDGE_CURVE('',#27141,#27142,#13256,.T.);
#34129=EDGE_CURVE('',#27140,#27142,#13257,.T.);
#34130=EDGE_CURVE('',#27143,#27139,#13258,.T.);
#34131=EDGE_CURVE('',#27143,#27144,#13259,.T.);
#34132=EDGE_CURVE('',#27144,#27141,#13260,.T.);
#34133=EDGE_CURVE('',#27145,#27143,#13261,.T.);
#34134=EDGE_CURVE('',#27145,#27146,#13262,.T.);
#34135=EDGE_CURVE('',#27146,#27144,#13263,.T.);
#34136=EDGE_CURVE('',#27140,#27145,#13264,.T.);
#34137=EDGE_CURVE('',#27142,#27146,#13265,.T.);
#34138=EDGE_CURVE('',#27147,#27148,#13266,.T.);
#34139=EDGE_CURVE('',#27147,#27149,#13267,.T.);
#34140=EDGE_CURVE('',#27149,#27150,#13268,.T.);
#34141=EDGE_CURVE('',#27148,#27150,#13269,.T.);
#34142=EDGE_CURVE('',#27151,#27147,#13270,.T.);
#34143=EDGE_CURVE('',#27151,#27152,#13271,.T.);
#34144=EDGE_CURVE('',#27152,#27149,#13272,.T.);
#34145=EDGE_CURVE('',#27153,#27151,#13273,.T.);
#34146=EDGE_CURVE('',#27153,#27154,#13274,.T.);
#34147=EDGE_CURVE('',#27154,#27152,#13275,.T.);
#34148=EDGE_CURVE('',#27148,#27153,#13276,.T.);
#34149=EDGE_CURVE('',#27150,#27154,#13277,.T.);
#34150=EDGE_CURVE('',#27155,#27156,#13278,.T.);
#34151=EDGE_CURVE('',#27155,#27157,#13279,.T.);
#34152=EDGE_CURVE('',#27157,#27158,#13280,.T.);
#34153=EDGE_CURVE('',#27156,#27158,#13281,.T.);
#34154=EDGE_CURVE('',#27159,#27155,#13282,.T.);
#34155=EDGE_CURVE('',#27159,#27160,#13283,.T.);
#34156=EDGE_CURVE('',#27160,#27157,#13284,.T.);
#34157=EDGE_CURVE('',#27161,#27159,#13285,.T.);
#34158=EDGE_CURVE('',#27161,#27162,#13286,.T.);
#34159=EDGE_CURVE('',#27162,#27160,#13287,.T.);
#34160=EDGE_CURVE('',#27156,#27161,#13288,.T.);
#34161=EDGE_CURVE('',#27158,#27162,#13289,.T.);
#34162=EDGE_CURVE('',#27163,#27164,#13290,.T.);
#34163=EDGE_CURVE('',#27163,#27165,#13291,.T.);
#34164=EDGE_CURVE('',#27165,#27166,#13292,.T.);
#34165=EDGE_CURVE('',#27164,#27166,#13293,.T.);
#34166=EDGE_CURVE('',#27167,#27163,#13294,.T.);
#34167=EDGE_CURVE('',#27167,#27168,#13295,.T.);
#34168=EDGE_CURVE('',#27168,#27165,#13296,.T.);
#34169=EDGE_CURVE('',#27169,#27167,#13297,.T.);
#34170=EDGE_CURVE('',#27169,#27170,#13298,.T.);
#34171=EDGE_CURVE('',#27170,#27168,#13299,.T.);
#34172=EDGE_CURVE('',#27164,#27169,#13300,.T.);
#34173=EDGE_CURVE('',#27166,#27170,#13301,.T.);
#34174=EDGE_CURVE('',#27171,#27172,#13302,.T.);
#34175=EDGE_CURVE('',#27171,#27173,#13303,.T.);
#34176=EDGE_CURVE('',#27173,#27174,#13304,.T.);
#34177=EDGE_CURVE('',#27172,#27174,#13305,.T.);
#34178=EDGE_CURVE('',#27175,#27171,#13306,.T.);
#34179=EDGE_CURVE('',#27175,#27176,#13307,.T.);
#34180=EDGE_CURVE('',#27176,#27173,#13308,.T.);
#34181=EDGE_CURVE('',#27177,#27175,#13309,.T.);
#34182=EDGE_CURVE('',#27177,#27178,#13310,.T.);
#34183=EDGE_CURVE('',#27178,#27176,#13311,.T.);
#34184=EDGE_CURVE('',#27172,#27177,#13312,.T.);
#34185=EDGE_CURVE('',#27174,#27178,#13313,.T.);
#34186=EDGE_CURVE('',#27179,#27180,#13314,.T.);
#34187=EDGE_CURVE('',#27179,#27181,#13315,.T.);
#34188=EDGE_CURVE('',#27181,#27182,#13316,.T.);
#34189=EDGE_CURVE('',#27180,#27182,#13317,.T.);
#34190=EDGE_CURVE('',#27183,#27179,#13318,.T.);
#34191=EDGE_CURVE('',#27183,#27184,#13319,.T.);
#34192=EDGE_CURVE('',#27184,#27181,#13320,.T.);
#34193=EDGE_CURVE('',#27185,#27183,#13321,.T.);
#34194=EDGE_CURVE('',#27185,#27186,#13322,.T.);
#34195=EDGE_CURVE('',#27186,#27184,#13323,.T.);
#34196=EDGE_CURVE('',#27180,#27185,#13324,.T.);
#34197=EDGE_CURVE('',#27182,#27186,#13325,.T.);
#34198=EDGE_CURVE('',#27187,#27188,#13326,.T.);
#34199=EDGE_CURVE('',#27187,#27189,#13327,.T.);
#34200=EDGE_CURVE('',#27189,#27190,#13328,.T.);
#34201=EDGE_CURVE('',#27188,#27190,#13329,.T.);
#34202=EDGE_CURVE('',#27191,#27187,#13330,.T.);
#34203=EDGE_CURVE('',#27191,#27192,#13331,.T.);
#34204=EDGE_CURVE('',#27192,#27189,#13332,.T.);
#34205=EDGE_CURVE('',#27193,#27191,#13333,.T.);
#34206=EDGE_CURVE('',#27193,#27194,#13334,.T.);
#34207=EDGE_CURVE('',#27194,#27192,#13335,.T.);
#34208=EDGE_CURVE('',#27188,#27193,#13336,.T.);
#34209=EDGE_CURVE('',#27190,#27194,#13337,.T.);
#34210=EDGE_CURVE('',#27195,#27196,#13338,.T.);
#34211=EDGE_CURVE('',#27195,#27197,#13339,.T.);
#34212=EDGE_CURVE('',#27197,#27198,#13340,.T.);
#34213=EDGE_CURVE('',#27196,#27198,#13341,.T.);
#34214=EDGE_CURVE('',#27199,#27195,#13342,.T.);
#34215=EDGE_CURVE('',#27199,#27200,#13343,.T.);
#34216=EDGE_CURVE('',#27200,#27197,#13344,.T.);
#34217=EDGE_CURVE('',#27201,#27199,#13345,.T.);
#34218=EDGE_CURVE('',#27201,#27202,#13346,.T.);
#34219=EDGE_CURVE('',#27202,#27200,#13347,.T.);
#34220=EDGE_CURVE('',#27196,#27201,#13348,.T.);
#34221=EDGE_CURVE('',#27198,#27202,#13349,.T.);
#34222=EDGE_CURVE('',#27203,#27204,#13350,.T.);
#34223=EDGE_CURVE('',#27203,#27205,#13351,.T.);
#34224=EDGE_CURVE('',#27205,#27206,#13352,.T.);
#34225=EDGE_CURVE('',#27204,#27206,#13353,.T.);
#34226=EDGE_CURVE('',#27207,#27203,#13354,.T.);
#34227=EDGE_CURVE('',#27207,#27208,#13355,.T.);
#34228=EDGE_CURVE('',#27208,#27205,#13356,.T.);
#34229=EDGE_CURVE('',#27209,#27207,#13357,.T.);
#34230=EDGE_CURVE('',#27209,#27210,#13358,.T.);
#34231=EDGE_CURVE('',#27210,#27208,#13359,.T.);
#34232=EDGE_CURVE('',#27204,#27209,#13360,.T.);
#34233=EDGE_CURVE('',#27206,#27210,#13361,.T.);
#34234=EDGE_CURVE('',#27211,#27212,#13362,.T.);
#34235=EDGE_CURVE('',#27211,#27213,#13363,.T.);
#34236=EDGE_CURVE('',#27213,#27214,#13364,.T.);
#34237=EDGE_CURVE('',#27212,#27214,#13365,.T.);
#34238=EDGE_CURVE('',#27215,#27211,#13366,.T.);
#34239=EDGE_CURVE('',#27215,#27216,#13367,.T.);
#34240=EDGE_CURVE('',#27216,#27213,#13368,.T.);
#34241=EDGE_CURVE('',#27217,#27215,#13369,.T.);
#34242=EDGE_CURVE('',#27217,#27218,#13370,.T.);
#34243=EDGE_CURVE('',#27218,#27216,#13371,.T.);
#34244=EDGE_CURVE('',#27212,#27217,#13372,.T.);
#34245=EDGE_CURVE('',#27214,#27218,#13373,.T.);
#34246=EDGE_CURVE('',#27219,#27220,#13374,.T.);
#34247=EDGE_CURVE('',#27219,#27221,#13375,.T.);
#34248=EDGE_CURVE('',#27221,#27222,#13376,.T.);
#34249=EDGE_CURVE('',#27220,#27222,#13377,.T.);
#34250=EDGE_CURVE('',#27223,#27219,#13378,.T.);
#34251=EDGE_CURVE('',#27223,#27224,#13379,.T.);
#34252=EDGE_CURVE('',#27224,#27221,#13380,.T.);
#34253=EDGE_CURVE('',#27225,#27223,#13381,.T.);
#34254=EDGE_CURVE('',#27225,#27226,#13382,.T.);
#34255=EDGE_CURVE('',#27226,#27224,#13383,.T.);
#34256=EDGE_CURVE('',#27220,#27225,#13384,.T.);
#34257=EDGE_CURVE('',#27222,#27226,#13385,.T.);
#34258=EDGE_CURVE('',#27227,#27228,#13386,.T.);
#34259=EDGE_CURVE('',#27227,#27229,#13387,.T.);
#34260=EDGE_CURVE('',#27229,#27230,#13388,.T.);
#34261=EDGE_CURVE('',#27228,#27230,#13389,.T.);
#34262=EDGE_CURVE('',#27231,#27227,#13390,.T.);
#34263=EDGE_CURVE('',#27231,#27232,#13391,.T.);
#34264=EDGE_CURVE('',#27232,#27229,#13392,.T.);
#34265=EDGE_CURVE('',#27233,#27231,#13393,.T.);
#34266=EDGE_CURVE('',#27233,#27234,#13394,.T.);
#34267=EDGE_CURVE('',#27234,#27232,#13395,.T.);
#34268=EDGE_CURVE('',#27228,#27233,#13396,.T.);
#34269=EDGE_CURVE('',#27230,#27234,#13397,.T.);
#34270=EDGE_CURVE('',#27235,#27236,#13398,.T.);
#34271=EDGE_CURVE('',#27235,#27237,#13399,.T.);
#34272=EDGE_CURVE('',#27237,#27238,#13400,.T.);
#34273=EDGE_CURVE('',#27236,#27238,#13401,.T.);
#34274=EDGE_CURVE('',#27239,#27235,#13402,.T.);
#34275=EDGE_CURVE('',#27239,#27240,#13403,.T.);
#34276=EDGE_CURVE('',#27240,#27237,#13404,.T.);
#34277=EDGE_CURVE('',#27241,#27239,#13405,.T.);
#34278=EDGE_CURVE('',#27241,#27242,#13406,.T.);
#34279=EDGE_CURVE('',#27242,#27240,#13407,.T.);
#34280=EDGE_CURVE('',#27236,#27241,#13408,.T.);
#34281=EDGE_CURVE('',#27238,#27242,#13409,.T.);
#34282=EDGE_CURVE('',#27243,#27244,#13410,.T.);
#34283=EDGE_CURVE('',#27243,#27245,#13411,.T.);
#34284=EDGE_CURVE('',#27245,#27246,#13412,.T.);
#34285=EDGE_CURVE('',#27244,#27246,#13413,.T.);
#34286=EDGE_CURVE('',#27247,#27243,#13414,.T.);
#34287=EDGE_CURVE('',#27247,#27248,#13415,.T.);
#34288=EDGE_CURVE('',#27248,#27245,#13416,.T.);
#34289=EDGE_CURVE('',#27249,#27247,#13417,.T.);
#34290=EDGE_CURVE('',#27249,#27250,#13418,.T.);
#34291=EDGE_CURVE('',#27250,#27248,#13419,.T.);
#34292=EDGE_CURVE('',#27244,#27249,#13420,.T.);
#34293=EDGE_CURVE('',#27246,#27250,#13421,.T.);
#34294=EDGE_CURVE('',#27251,#27252,#13422,.T.);
#34295=EDGE_CURVE('',#27251,#27253,#13423,.T.);
#34296=EDGE_CURVE('',#27253,#27254,#13424,.T.);
#34297=EDGE_CURVE('',#27252,#27254,#13425,.T.);
#34298=EDGE_CURVE('',#27255,#27251,#13426,.T.);
#34299=EDGE_CURVE('',#27255,#27256,#13427,.T.);
#34300=EDGE_CURVE('',#27256,#27253,#13428,.T.);
#34301=EDGE_CURVE('',#27257,#27255,#13429,.T.);
#34302=EDGE_CURVE('',#27257,#27258,#13430,.T.);
#34303=EDGE_CURVE('',#27258,#27256,#13431,.T.);
#34304=EDGE_CURVE('',#27252,#27257,#13432,.T.);
#34305=EDGE_CURVE('',#27254,#27258,#13433,.T.);
#34306=EDGE_CURVE('',#27259,#27260,#13434,.T.);
#34307=EDGE_CURVE('',#27259,#27261,#13435,.T.);
#34308=EDGE_CURVE('',#27261,#27262,#13436,.T.);
#34309=EDGE_CURVE('',#27260,#27262,#13437,.T.);
#34310=EDGE_CURVE('',#27263,#27259,#13438,.T.);
#34311=EDGE_CURVE('',#27263,#27264,#13439,.T.);
#34312=EDGE_CURVE('',#27264,#27261,#13440,.T.);
#34313=EDGE_CURVE('',#27265,#27263,#13441,.T.);
#34314=EDGE_CURVE('',#27265,#27266,#13442,.T.);
#34315=EDGE_CURVE('',#27266,#27264,#13443,.T.);
#34316=EDGE_CURVE('',#27260,#27265,#13444,.T.);
#34317=EDGE_CURVE('',#27262,#27266,#13445,.T.);
#34318=EDGE_CURVE('',#27267,#27268,#13446,.T.);
#34319=EDGE_CURVE('',#27267,#27269,#13447,.T.);
#34320=EDGE_CURVE('',#27269,#27270,#13448,.T.);
#34321=EDGE_CURVE('',#27268,#27270,#13449,.T.);
#34322=EDGE_CURVE('',#27271,#27267,#13450,.T.);
#34323=EDGE_CURVE('',#27271,#27272,#13451,.T.);
#34324=EDGE_CURVE('',#27272,#27269,#13452,.T.);
#34325=EDGE_CURVE('',#27273,#27271,#13453,.T.);
#34326=EDGE_CURVE('',#27273,#27274,#13454,.T.);
#34327=EDGE_CURVE('',#27274,#27272,#13455,.T.);
#34328=EDGE_CURVE('',#27268,#27273,#13456,.T.);
#34329=EDGE_CURVE('',#27270,#27274,#13457,.T.);
#34330=EDGE_CURVE('',#27275,#27276,#13458,.T.);
#34331=EDGE_CURVE('',#27275,#27277,#13459,.T.);
#34332=EDGE_CURVE('',#27277,#27278,#13460,.T.);
#34333=EDGE_CURVE('',#27276,#27278,#13461,.T.);
#34334=EDGE_CURVE('',#27279,#27275,#13462,.T.);
#34335=EDGE_CURVE('',#27279,#27280,#13463,.T.);
#34336=EDGE_CURVE('',#27280,#27277,#13464,.T.);
#34337=EDGE_CURVE('',#27281,#27279,#13465,.T.);
#34338=EDGE_CURVE('',#27281,#27282,#13466,.T.);
#34339=EDGE_CURVE('',#27282,#27280,#13467,.T.);
#34340=EDGE_CURVE('',#27276,#27281,#13468,.T.);
#34341=EDGE_CURVE('',#27278,#27282,#13469,.T.);
#34342=EDGE_CURVE('',#27283,#27284,#13470,.T.);
#34343=EDGE_CURVE('',#27283,#27285,#13471,.T.);
#34344=EDGE_CURVE('',#27285,#27286,#13472,.T.);
#34345=EDGE_CURVE('',#27284,#27286,#13473,.T.);
#34346=EDGE_CURVE('',#27287,#27283,#13474,.T.);
#34347=EDGE_CURVE('',#27287,#27288,#13475,.T.);
#34348=EDGE_CURVE('',#27288,#27285,#13476,.T.);
#34349=EDGE_CURVE('',#27289,#27287,#13477,.T.);
#34350=EDGE_CURVE('',#27289,#27290,#13478,.T.);
#34351=EDGE_CURVE('',#27290,#27288,#13479,.T.);
#34352=EDGE_CURVE('',#27284,#27289,#13480,.T.);
#34353=EDGE_CURVE('',#27286,#27290,#13481,.T.);
#34354=EDGE_CURVE('',#27291,#27292,#13482,.T.);
#34355=EDGE_CURVE('',#27291,#27293,#13483,.T.);
#34356=EDGE_CURVE('',#27293,#27294,#13484,.T.);
#34357=EDGE_CURVE('',#27292,#27294,#13485,.T.);
#34358=EDGE_CURVE('',#27295,#27291,#13486,.T.);
#34359=EDGE_CURVE('',#27295,#27296,#13487,.T.);
#34360=EDGE_CURVE('',#27296,#27293,#13488,.T.);
#34361=EDGE_CURVE('',#27297,#27295,#13489,.T.);
#34362=EDGE_CURVE('',#27297,#27298,#13490,.T.);
#34363=EDGE_CURVE('',#27298,#27296,#13491,.T.);
#34364=EDGE_CURVE('',#27292,#27297,#13492,.T.);
#34365=EDGE_CURVE('',#27294,#27298,#13493,.T.);
#34366=EDGE_CURVE('',#27299,#27300,#13494,.T.);
#34367=EDGE_CURVE('',#27299,#27301,#13495,.T.);
#34368=EDGE_CURVE('',#27301,#27302,#13496,.T.);
#34369=EDGE_CURVE('',#27300,#27302,#13497,.T.);
#34370=EDGE_CURVE('',#27303,#27299,#13498,.T.);
#34371=EDGE_CURVE('',#27303,#27304,#13499,.T.);
#34372=EDGE_CURVE('',#27304,#27301,#13500,.T.);
#34373=EDGE_CURVE('',#27305,#27303,#13501,.T.);
#34374=EDGE_CURVE('',#27305,#27306,#13502,.T.);
#34375=EDGE_CURVE('',#27306,#27304,#13503,.T.);
#34376=EDGE_CURVE('',#27300,#27305,#13504,.T.);
#34377=EDGE_CURVE('',#27302,#27306,#13505,.T.);
#34378=EDGE_CURVE('',#27307,#27308,#13506,.T.);
#34379=EDGE_CURVE('',#27307,#27309,#13507,.T.);
#34380=EDGE_CURVE('',#27309,#27310,#13508,.T.);
#34381=EDGE_CURVE('',#27308,#27310,#13509,.T.);
#34382=EDGE_CURVE('',#27311,#27307,#13510,.T.);
#34383=EDGE_CURVE('',#27311,#27312,#13511,.T.);
#34384=EDGE_CURVE('',#27312,#27309,#13512,.T.);
#34385=EDGE_CURVE('',#27313,#27311,#13513,.T.);
#34386=EDGE_CURVE('',#27313,#27314,#13514,.T.);
#34387=EDGE_CURVE('',#27314,#27312,#13515,.T.);
#34388=EDGE_CURVE('',#27308,#27313,#13516,.T.);
#34389=EDGE_CURVE('',#27310,#27314,#13517,.T.);
#34390=EDGE_CURVE('',#27315,#27316,#13518,.T.);
#34391=EDGE_CURVE('',#27315,#27317,#13519,.T.);
#34392=EDGE_CURVE('',#27317,#27318,#13520,.T.);
#34393=EDGE_CURVE('',#27316,#27318,#13521,.T.);
#34394=EDGE_CURVE('',#27319,#27315,#13522,.T.);
#34395=EDGE_CURVE('',#27319,#27320,#13523,.T.);
#34396=EDGE_CURVE('',#27320,#27317,#13524,.T.);
#34397=EDGE_CURVE('',#27321,#27319,#13525,.T.);
#34398=EDGE_CURVE('',#27321,#27322,#13526,.T.);
#34399=EDGE_CURVE('',#27322,#27320,#13527,.T.);
#34400=EDGE_CURVE('',#27316,#27321,#13528,.T.);
#34401=EDGE_CURVE('',#27318,#27322,#13529,.T.);
#34402=EDGE_CURVE('',#27323,#27324,#13530,.T.);
#34403=EDGE_CURVE('',#27323,#27325,#13531,.T.);
#34404=EDGE_CURVE('',#27325,#27326,#13532,.T.);
#34405=EDGE_CURVE('',#27324,#27326,#13533,.T.);
#34406=EDGE_CURVE('',#27327,#27323,#13534,.T.);
#34407=EDGE_CURVE('',#27327,#27328,#13535,.T.);
#34408=EDGE_CURVE('',#27328,#27325,#13536,.T.);
#34409=EDGE_CURVE('',#27329,#27327,#13537,.T.);
#34410=EDGE_CURVE('',#27329,#27330,#13538,.T.);
#34411=EDGE_CURVE('',#27330,#27328,#13539,.T.);
#34412=EDGE_CURVE('',#27324,#27329,#13540,.T.);
#34413=EDGE_CURVE('',#27326,#27330,#13541,.T.);
#34414=EDGE_CURVE('',#27331,#27332,#13542,.T.);
#34415=EDGE_CURVE('',#27331,#27333,#13543,.T.);
#34416=EDGE_CURVE('',#27333,#27334,#13544,.T.);
#34417=EDGE_CURVE('',#27332,#27334,#13545,.T.);
#34418=EDGE_CURVE('',#27335,#27331,#13546,.T.);
#34419=EDGE_CURVE('',#27335,#27336,#13547,.T.);
#34420=EDGE_CURVE('',#27336,#27333,#13548,.T.);
#34421=EDGE_CURVE('',#27337,#27335,#13549,.T.);
#34422=EDGE_CURVE('',#27337,#27338,#13550,.T.);
#34423=EDGE_CURVE('',#27338,#27336,#13551,.T.);
#34424=EDGE_CURVE('',#27332,#27337,#13552,.T.);
#34425=EDGE_CURVE('',#27334,#27338,#13553,.T.);
#34426=EDGE_CURVE('',#27339,#27340,#13554,.T.);
#34427=EDGE_CURVE('',#27339,#27341,#13555,.T.);
#34428=EDGE_CURVE('',#27341,#27342,#13556,.T.);
#34429=EDGE_CURVE('',#27340,#27342,#13557,.T.);
#34430=EDGE_CURVE('',#27343,#27339,#13558,.T.);
#34431=EDGE_CURVE('',#27343,#27344,#13559,.T.);
#34432=EDGE_CURVE('',#27344,#27341,#13560,.T.);
#34433=EDGE_CURVE('',#27345,#27343,#13561,.T.);
#34434=EDGE_CURVE('',#27345,#27346,#13562,.T.);
#34435=EDGE_CURVE('',#27346,#27344,#13563,.T.);
#34436=EDGE_CURVE('',#27340,#27345,#13564,.T.);
#34437=EDGE_CURVE('',#27342,#27346,#13565,.T.);
#34438=EDGE_CURVE('',#27347,#27348,#13566,.T.);
#34439=EDGE_CURVE('',#27347,#27349,#13567,.T.);
#34440=EDGE_CURVE('',#27349,#27350,#13568,.T.);
#34441=EDGE_CURVE('',#27348,#27350,#13569,.T.);
#34442=EDGE_CURVE('',#27351,#27347,#13570,.T.);
#34443=EDGE_CURVE('',#27351,#27352,#13571,.T.);
#34444=EDGE_CURVE('',#27352,#27349,#13572,.T.);
#34445=EDGE_CURVE('',#27353,#27351,#13573,.T.);
#34446=EDGE_CURVE('',#27353,#27354,#13574,.T.);
#34447=EDGE_CURVE('',#27354,#27352,#13575,.T.);
#34448=EDGE_CURVE('',#27348,#27353,#13576,.T.);
#34449=EDGE_CURVE('',#27350,#27354,#13577,.T.);
#34450=EDGE_CURVE('',#27355,#27356,#13578,.T.);
#34451=EDGE_CURVE('',#27355,#27357,#13579,.T.);
#34452=EDGE_CURVE('',#27357,#27358,#13580,.T.);
#34453=EDGE_CURVE('',#27356,#27358,#13581,.T.);
#34454=EDGE_CURVE('',#27359,#27355,#13582,.T.);
#34455=EDGE_CURVE('',#27359,#27360,#13583,.T.);
#34456=EDGE_CURVE('',#27360,#27357,#13584,.T.);
#34457=EDGE_CURVE('',#27361,#27359,#13585,.T.);
#34458=EDGE_CURVE('',#27361,#27362,#13586,.T.);
#34459=EDGE_CURVE('',#27362,#27360,#13587,.T.);
#34460=EDGE_CURVE('',#27356,#27361,#13588,.T.);
#34461=EDGE_CURVE('',#27358,#27362,#13589,.T.);
#34462=EDGE_CURVE('',#27363,#27364,#13590,.T.);
#34463=EDGE_CURVE('',#27363,#27365,#13591,.T.);
#34464=EDGE_CURVE('',#27365,#27366,#13592,.T.);
#34465=EDGE_CURVE('',#27364,#27366,#13593,.T.);
#34466=EDGE_CURVE('',#27367,#27363,#13594,.T.);
#34467=EDGE_CURVE('',#27367,#27368,#13595,.T.);
#34468=EDGE_CURVE('',#27368,#27365,#13596,.T.);
#34469=EDGE_CURVE('',#27369,#27367,#13597,.T.);
#34470=EDGE_CURVE('',#27369,#27370,#13598,.T.);
#34471=EDGE_CURVE('',#27370,#27368,#13599,.T.);
#34472=EDGE_CURVE('',#27364,#27369,#13600,.T.);
#34473=EDGE_CURVE('',#27366,#27370,#13601,.T.);
#34474=EDGE_CURVE('',#27371,#27372,#13602,.T.);
#34475=EDGE_CURVE('',#27371,#27373,#13603,.T.);
#34476=EDGE_CURVE('',#27373,#27374,#13604,.T.);
#34477=EDGE_CURVE('',#27372,#27374,#13605,.T.);
#34478=EDGE_CURVE('',#27375,#27371,#13606,.T.);
#34479=EDGE_CURVE('',#27375,#27376,#13607,.T.);
#34480=EDGE_CURVE('',#27376,#27373,#13608,.T.);
#34481=EDGE_CURVE('',#27377,#27375,#13609,.T.);
#34482=EDGE_CURVE('',#27377,#27378,#13610,.T.);
#34483=EDGE_CURVE('',#27378,#27376,#13611,.T.);
#34484=EDGE_CURVE('',#27372,#27377,#13612,.T.);
#34485=EDGE_CURVE('',#27374,#27378,#13613,.T.);
#34486=EDGE_CURVE('',#27379,#27380,#13614,.T.);
#34487=EDGE_CURVE('',#27379,#27381,#13615,.T.);
#34488=EDGE_CURVE('',#27381,#27382,#13616,.T.);
#34489=EDGE_CURVE('',#27380,#27382,#13617,.T.);
#34490=EDGE_CURVE('',#27383,#27379,#13618,.T.);
#34491=EDGE_CURVE('',#27383,#27384,#13619,.T.);
#34492=EDGE_CURVE('',#27384,#27381,#13620,.T.);
#34493=EDGE_CURVE('',#27385,#27383,#13621,.T.);
#34494=EDGE_CURVE('',#27385,#27386,#13622,.T.);
#34495=EDGE_CURVE('',#27386,#27384,#13623,.T.);
#34496=EDGE_CURVE('',#27380,#27385,#13624,.T.);
#34497=EDGE_CURVE('',#27382,#27386,#13625,.T.);
#34498=EDGE_CURVE('',#27387,#27388,#13626,.T.);
#34499=EDGE_CURVE('',#27387,#27389,#13627,.T.);
#34500=EDGE_CURVE('',#27389,#27390,#13628,.T.);
#34501=EDGE_CURVE('',#27388,#27390,#13629,.T.);
#34502=EDGE_CURVE('',#27391,#27387,#13630,.T.);
#34503=EDGE_CURVE('',#27391,#27392,#13631,.T.);
#34504=EDGE_CURVE('',#27392,#27389,#13632,.T.);
#34505=EDGE_CURVE('',#27393,#27391,#13633,.T.);
#34506=EDGE_CURVE('',#27393,#27394,#13634,.T.);
#34507=EDGE_CURVE('',#27394,#27392,#13635,.T.);
#34508=EDGE_CURVE('',#27388,#27393,#13636,.T.);
#34509=EDGE_CURVE('',#27390,#27394,#13637,.T.);
#34510=EDGE_CURVE('',#27395,#27396,#13638,.T.);
#34511=EDGE_CURVE('',#27395,#27397,#13639,.T.);
#34512=EDGE_CURVE('',#27397,#27398,#13640,.T.);
#34513=EDGE_CURVE('',#27396,#27398,#13641,.T.);
#34514=EDGE_CURVE('',#27399,#27395,#13642,.T.);
#34515=EDGE_CURVE('',#27399,#27400,#13643,.T.);
#34516=EDGE_CURVE('',#27400,#27397,#13644,.T.);
#34517=EDGE_CURVE('',#27401,#27399,#13645,.T.);
#34518=EDGE_CURVE('',#27401,#27402,#13646,.T.);
#34519=EDGE_CURVE('',#27402,#27400,#13647,.T.);
#34520=EDGE_CURVE('',#27396,#27401,#13648,.T.);
#34521=EDGE_CURVE('',#27398,#27402,#13649,.T.);
#34522=EDGE_CURVE('',#27403,#27404,#13650,.T.);
#34523=EDGE_CURVE('',#27403,#27405,#13651,.T.);
#34524=EDGE_CURVE('',#27405,#27406,#13652,.T.);
#34525=EDGE_CURVE('',#27404,#27406,#13653,.T.);
#34526=EDGE_CURVE('',#27407,#27403,#13654,.T.);
#34527=EDGE_CURVE('',#27407,#27408,#13655,.T.);
#34528=EDGE_CURVE('',#27408,#27405,#13656,.T.);
#34529=EDGE_CURVE('',#27409,#27407,#13657,.T.);
#34530=EDGE_CURVE('',#27409,#27410,#13658,.T.);
#34531=EDGE_CURVE('',#27410,#27408,#13659,.T.);
#34532=EDGE_CURVE('',#27404,#27409,#13660,.T.);
#34533=EDGE_CURVE('',#27406,#27410,#13661,.T.);
#34534=EDGE_CURVE('',#27411,#27412,#13662,.T.);
#34535=EDGE_CURVE('',#27411,#27413,#13663,.T.);
#34536=EDGE_CURVE('',#27413,#27414,#13664,.T.);
#34537=EDGE_CURVE('',#27412,#27414,#13665,.T.);
#34538=EDGE_CURVE('',#27415,#27411,#13666,.T.);
#34539=EDGE_CURVE('',#27415,#27416,#13667,.T.);
#34540=EDGE_CURVE('',#27416,#27413,#13668,.T.);
#34541=EDGE_CURVE('',#27417,#27415,#13669,.T.);
#34542=EDGE_CURVE('',#27417,#27418,#13670,.T.);
#34543=EDGE_CURVE('',#27418,#27416,#13671,.T.);
#34544=EDGE_CURVE('',#27412,#27417,#13672,.T.);
#34545=EDGE_CURVE('',#27414,#27418,#13673,.T.);
#34546=EDGE_CURVE('',#27419,#27420,#13674,.T.);
#34547=EDGE_CURVE('',#27419,#27421,#13675,.T.);
#34548=EDGE_CURVE('',#27421,#27422,#13676,.T.);
#34549=EDGE_CURVE('',#27420,#27422,#13677,.T.);
#34550=EDGE_CURVE('',#27423,#27419,#13678,.T.);
#34551=EDGE_CURVE('',#27423,#27424,#13679,.T.);
#34552=EDGE_CURVE('',#27424,#27421,#13680,.T.);
#34553=EDGE_CURVE('',#27425,#27423,#13681,.T.);
#34554=EDGE_CURVE('',#27425,#27426,#13682,.T.);
#34555=EDGE_CURVE('',#27426,#27424,#13683,.T.);
#34556=EDGE_CURVE('',#27420,#27425,#13684,.T.);
#34557=EDGE_CURVE('',#27422,#27426,#13685,.T.);
#34558=EDGE_CURVE('',#27427,#27428,#13686,.T.);
#34559=EDGE_CURVE('',#27427,#27429,#13687,.T.);
#34560=EDGE_CURVE('',#27429,#27430,#13688,.T.);
#34561=EDGE_CURVE('',#27428,#27430,#13689,.T.);
#34562=EDGE_CURVE('',#27431,#27427,#13690,.T.);
#34563=EDGE_CURVE('',#27431,#27432,#13691,.T.);
#34564=EDGE_CURVE('',#27432,#27429,#13692,.T.);
#34565=EDGE_CURVE('',#27433,#27431,#13693,.T.);
#34566=EDGE_CURVE('',#27433,#27434,#13694,.T.);
#34567=EDGE_CURVE('',#27434,#27432,#13695,.T.);
#34568=EDGE_CURVE('',#27428,#27433,#13696,.T.);
#34569=EDGE_CURVE('',#27430,#27434,#13697,.T.);
#34570=EDGE_CURVE('',#27435,#27436,#13698,.T.);
#34571=EDGE_CURVE('',#27435,#27437,#13699,.T.);
#34572=EDGE_CURVE('',#27437,#27438,#13700,.T.);
#34573=EDGE_CURVE('',#27436,#27438,#13701,.T.);
#34574=EDGE_CURVE('',#27439,#27435,#13702,.T.);
#34575=EDGE_CURVE('',#27439,#27440,#13703,.T.);
#34576=EDGE_CURVE('',#27440,#27437,#13704,.T.);
#34577=EDGE_CURVE('',#27441,#27439,#13705,.T.);
#34578=EDGE_CURVE('',#27441,#27442,#13706,.T.);
#34579=EDGE_CURVE('',#27442,#27440,#13707,.T.);
#34580=EDGE_CURVE('',#27436,#27441,#13708,.T.);
#34581=EDGE_CURVE('',#27438,#27442,#13709,.T.);
#34582=EDGE_CURVE('',#27443,#27444,#13710,.T.);
#34583=EDGE_CURVE('',#27443,#27445,#13711,.T.);
#34584=EDGE_CURVE('',#27445,#27446,#13712,.T.);
#34585=EDGE_CURVE('',#27444,#27446,#13713,.T.);
#34586=EDGE_CURVE('',#27447,#27443,#13714,.T.);
#34587=EDGE_CURVE('',#27447,#27448,#13715,.T.);
#34588=EDGE_CURVE('',#27448,#27445,#13716,.T.);
#34589=EDGE_CURVE('',#27449,#27447,#13717,.T.);
#34590=EDGE_CURVE('',#27449,#27450,#13718,.T.);
#34591=EDGE_CURVE('',#27450,#27448,#13719,.T.);
#34592=EDGE_CURVE('',#27444,#27449,#13720,.T.);
#34593=EDGE_CURVE('',#27446,#27450,#13721,.T.);
#34594=EDGE_CURVE('',#27451,#27452,#13722,.T.);
#34595=EDGE_CURVE('',#27451,#27453,#13723,.T.);
#34596=EDGE_CURVE('',#27453,#27454,#13724,.T.);
#34597=EDGE_CURVE('',#27452,#27454,#13725,.T.);
#34598=EDGE_CURVE('',#27455,#27451,#13726,.T.);
#34599=EDGE_CURVE('',#27455,#27456,#13727,.T.);
#34600=EDGE_CURVE('',#27456,#27453,#13728,.T.);
#34601=EDGE_CURVE('',#27457,#27455,#13729,.T.);
#34602=EDGE_CURVE('',#27457,#27458,#13730,.T.);
#34603=EDGE_CURVE('',#27458,#27456,#13731,.T.);
#34604=EDGE_CURVE('',#27452,#27457,#13732,.T.);
#34605=EDGE_CURVE('',#27454,#27458,#13733,.T.);
#34606=EDGE_CURVE('',#27459,#27460,#13734,.T.);
#34607=EDGE_CURVE('',#27459,#27461,#13735,.T.);
#34608=EDGE_CURVE('',#27461,#27462,#13736,.T.);
#34609=EDGE_CURVE('',#27460,#27462,#13737,.T.);
#34610=EDGE_CURVE('',#27463,#27459,#13738,.T.);
#34611=EDGE_CURVE('',#27463,#27464,#13739,.T.);
#34612=EDGE_CURVE('',#27464,#27461,#13740,.T.);
#34613=EDGE_CURVE('',#27465,#27463,#13741,.T.);
#34614=EDGE_CURVE('',#27465,#27466,#13742,.T.);
#34615=EDGE_CURVE('',#27466,#27464,#13743,.T.);
#34616=EDGE_CURVE('',#27460,#27465,#13744,.T.);
#34617=EDGE_CURVE('',#27462,#27466,#13745,.T.);
#34618=EDGE_CURVE('',#27467,#27468,#13746,.T.);
#34619=EDGE_CURVE('',#27467,#27469,#13747,.T.);
#34620=EDGE_CURVE('',#27469,#27470,#13748,.T.);
#34621=EDGE_CURVE('',#27468,#27470,#13749,.T.);
#34622=EDGE_CURVE('',#27471,#27467,#13750,.T.);
#34623=EDGE_CURVE('',#27471,#27472,#13751,.T.);
#34624=EDGE_CURVE('',#27472,#27469,#13752,.T.);
#34625=EDGE_CURVE('',#27473,#27471,#13753,.T.);
#34626=EDGE_CURVE('',#27473,#27474,#13754,.T.);
#34627=EDGE_CURVE('',#27474,#27472,#13755,.T.);
#34628=EDGE_CURVE('',#27468,#27473,#13756,.T.);
#34629=EDGE_CURVE('',#27470,#27474,#13757,.T.);
#34630=EDGE_CURVE('',#27475,#27476,#13758,.T.);
#34631=EDGE_CURVE('',#27475,#27477,#13759,.T.);
#34632=EDGE_CURVE('',#27477,#27478,#13760,.T.);
#34633=EDGE_CURVE('',#27476,#27478,#13761,.T.);
#34634=EDGE_CURVE('',#27479,#27475,#13762,.T.);
#34635=EDGE_CURVE('',#27479,#27480,#13763,.T.);
#34636=EDGE_CURVE('',#27480,#27477,#13764,.T.);
#34637=EDGE_CURVE('',#27481,#27479,#13765,.T.);
#34638=EDGE_CURVE('',#27481,#27482,#13766,.T.);
#34639=EDGE_CURVE('',#27482,#27480,#13767,.T.);
#34640=EDGE_CURVE('',#27476,#27481,#13768,.T.);
#34641=EDGE_CURVE('',#27478,#27482,#13769,.T.);
#34642=EDGE_CURVE('',#27483,#27484,#13770,.T.);
#34643=EDGE_CURVE('',#27483,#27485,#13771,.T.);
#34644=EDGE_CURVE('',#27485,#27486,#13772,.T.);
#34645=EDGE_CURVE('',#27484,#27486,#13773,.T.);
#34646=EDGE_CURVE('',#27487,#27483,#13774,.T.);
#34647=EDGE_CURVE('',#27487,#27488,#13775,.T.);
#34648=EDGE_CURVE('',#27488,#27485,#13776,.T.);
#34649=EDGE_CURVE('',#27489,#27487,#13777,.T.);
#34650=EDGE_CURVE('',#27489,#27490,#13778,.T.);
#34651=EDGE_CURVE('',#27490,#27488,#13779,.T.);
#34652=EDGE_CURVE('',#27484,#27489,#13780,.T.);
#34653=EDGE_CURVE('',#27486,#27490,#13781,.T.);
#34654=EDGE_CURVE('',#27491,#27492,#13782,.T.);
#34655=EDGE_CURVE('',#27491,#27493,#13783,.T.);
#34656=EDGE_CURVE('',#27493,#27494,#13784,.T.);
#34657=EDGE_CURVE('',#27492,#27494,#13785,.T.);
#34658=EDGE_CURVE('',#27495,#27491,#13786,.T.);
#34659=EDGE_CURVE('',#27495,#27496,#13787,.T.);
#34660=EDGE_CURVE('',#27496,#27493,#13788,.T.);
#34661=EDGE_CURVE('',#27497,#27495,#13789,.T.);
#34662=EDGE_CURVE('',#27497,#27498,#13790,.T.);
#34663=EDGE_CURVE('',#27498,#27496,#13791,.T.);
#34664=EDGE_CURVE('',#27492,#27497,#13792,.T.);
#34665=EDGE_CURVE('',#27494,#27498,#13793,.T.);
#34666=EDGE_CURVE('',#27499,#27500,#13794,.T.);
#34667=EDGE_CURVE('',#27499,#27501,#13795,.T.);
#34668=EDGE_CURVE('',#27501,#27502,#13796,.T.);
#34669=EDGE_CURVE('',#27500,#27502,#13797,.T.);
#34670=EDGE_CURVE('',#27503,#27499,#13798,.T.);
#34671=EDGE_CURVE('',#27503,#27504,#13799,.T.);
#34672=EDGE_CURVE('',#27504,#27501,#13800,.T.);
#34673=EDGE_CURVE('',#27505,#27503,#13801,.T.);
#34674=EDGE_CURVE('',#27505,#27506,#13802,.T.);
#34675=EDGE_CURVE('',#27506,#27504,#13803,.T.);
#34676=EDGE_CURVE('',#27500,#27505,#13804,.T.);
#34677=EDGE_CURVE('',#27502,#27506,#13805,.T.);
#34678=EDGE_CURVE('',#27507,#27508,#13806,.T.);
#34679=EDGE_CURVE('',#27507,#27509,#13807,.T.);
#34680=EDGE_CURVE('',#27509,#27510,#13808,.T.);
#34681=EDGE_CURVE('',#27508,#27510,#13809,.T.);
#34682=EDGE_CURVE('',#27511,#27507,#13810,.T.);
#34683=EDGE_CURVE('',#27511,#27512,#13811,.T.);
#34684=EDGE_CURVE('',#27512,#27509,#13812,.T.);
#34685=EDGE_CURVE('',#27513,#27511,#13813,.T.);
#34686=EDGE_CURVE('',#27513,#27514,#13814,.T.);
#34687=EDGE_CURVE('',#27514,#27512,#13815,.T.);
#34688=EDGE_CURVE('',#27508,#27513,#13816,.T.);
#34689=EDGE_CURVE('',#27510,#27514,#13817,.T.);
#34690=EDGE_CURVE('',#27515,#27516,#13818,.T.);
#34691=EDGE_CURVE('',#27515,#27517,#13819,.T.);
#34692=EDGE_CURVE('',#27517,#27518,#13820,.T.);
#34693=EDGE_CURVE('',#27516,#27518,#13821,.T.);
#34694=EDGE_CURVE('',#27519,#27515,#13822,.T.);
#34695=EDGE_CURVE('',#27519,#27520,#13823,.T.);
#34696=EDGE_CURVE('',#27520,#27517,#13824,.T.);
#34697=EDGE_CURVE('',#27521,#27519,#13825,.T.);
#34698=EDGE_CURVE('',#27521,#27522,#13826,.T.);
#34699=EDGE_CURVE('',#27522,#27520,#13827,.T.);
#34700=EDGE_CURVE('',#27516,#27521,#13828,.T.);
#34701=EDGE_CURVE('',#27518,#27522,#13829,.T.);
#34702=EDGE_CURVE('',#27523,#27524,#13830,.T.);
#34703=EDGE_CURVE('',#27523,#27525,#13831,.T.);
#34704=EDGE_CURVE('',#27525,#27526,#13832,.T.);
#34705=EDGE_CURVE('',#27524,#27526,#13833,.T.);
#34706=EDGE_CURVE('',#27527,#27523,#13834,.T.);
#34707=EDGE_CURVE('',#27527,#27528,#13835,.T.);
#34708=EDGE_CURVE('',#27528,#27525,#13836,.T.);
#34709=EDGE_CURVE('',#27529,#27527,#13837,.T.);
#34710=EDGE_CURVE('',#27529,#27530,#13838,.T.);
#34711=EDGE_CURVE('',#27530,#27528,#13839,.T.);
#34712=EDGE_CURVE('',#27524,#27529,#13840,.T.);
#34713=EDGE_CURVE('',#27526,#27530,#13841,.T.);
#34714=EDGE_CURVE('',#27531,#27532,#13842,.T.);
#34715=EDGE_CURVE('',#27531,#27533,#13843,.T.);
#34716=EDGE_CURVE('',#27533,#27534,#13844,.T.);
#34717=EDGE_CURVE('',#27532,#27534,#13845,.T.);
#34718=EDGE_CURVE('',#27535,#27531,#13846,.T.);
#34719=EDGE_CURVE('',#27535,#27536,#13847,.T.);
#34720=EDGE_CURVE('',#27536,#27533,#13848,.T.);
#34721=EDGE_CURVE('',#27537,#27535,#13849,.T.);
#34722=EDGE_CURVE('',#27537,#27538,#13850,.T.);
#34723=EDGE_CURVE('',#27538,#27536,#13851,.T.);
#34724=EDGE_CURVE('',#27532,#27537,#13852,.T.);
#34725=EDGE_CURVE('',#27534,#27538,#13853,.T.);
#34726=EDGE_CURVE('',#27539,#27540,#13854,.T.);
#34727=EDGE_CURVE('',#27539,#27541,#13855,.T.);
#34728=EDGE_CURVE('',#27541,#27542,#13856,.T.);
#34729=EDGE_CURVE('',#27540,#27542,#13857,.T.);
#34730=EDGE_CURVE('',#27543,#27539,#13858,.T.);
#34731=EDGE_CURVE('',#27543,#27544,#13859,.T.);
#34732=EDGE_CURVE('',#27544,#27541,#13860,.T.);
#34733=EDGE_CURVE('',#27545,#27543,#13861,.T.);
#34734=EDGE_CURVE('',#27545,#27546,#13862,.T.);
#34735=EDGE_CURVE('',#27546,#27544,#13863,.T.);
#34736=EDGE_CURVE('',#27540,#27545,#13864,.T.);
#34737=EDGE_CURVE('',#27542,#27546,#13865,.T.);
#34738=EDGE_CURVE('',#27547,#27548,#13866,.T.);
#34739=EDGE_CURVE('',#27547,#27549,#13867,.T.);
#34740=EDGE_CURVE('',#27549,#27550,#13868,.T.);
#34741=EDGE_CURVE('',#27548,#27550,#13869,.T.);
#34742=EDGE_CURVE('',#27551,#27547,#13870,.T.);
#34743=EDGE_CURVE('',#27551,#27552,#13871,.T.);
#34744=EDGE_CURVE('',#27552,#27549,#13872,.T.);
#34745=EDGE_CURVE('',#27553,#27551,#13873,.T.);
#34746=EDGE_CURVE('',#27553,#27554,#13874,.T.);
#34747=EDGE_CURVE('',#27554,#27552,#13875,.T.);
#34748=EDGE_CURVE('',#27548,#27553,#13876,.T.);
#34749=EDGE_CURVE('',#27550,#27554,#13877,.T.);
#34750=EDGE_CURVE('',#27555,#27556,#13878,.T.);
#34751=EDGE_CURVE('',#27555,#27557,#13879,.T.);
#34752=EDGE_CURVE('',#27557,#27558,#13880,.T.);
#34753=EDGE_CURVE('',#27556,#27558,#13881,.T.);
#34754=EDGE_CURVE('',#27559,#27555,#13882,.T.);
#34755=EDGE_CURVE('',#27559,#27560,#13883,.T.);
#34756=EDGE_CURVE('',#27560,#27557,#13884,.T.);
#34757=EDGE_CURVE('',#27561,#27559,#13885,.T.);
#34758=EDGE_CURVE('',#27561,#27562,#13886,.T.);
#34759=EDGE_CURVE('',#27562,#27560,#13887,.T.);
#34760=EDGE_CURVE('',#27556,#27561,#13888,.T.);
#34761=EDGE_CURVE('',#27558,#27562,#13889,.T.);
#34762=EDGE_CURVE('',#27563,#27564,#13890,.T.);
#34763=EDGE_CURVE('',#27563,#27565,#13891,.T.);
#34764=EDGE_CURVE('',#27565,#27566,#13892,.T.);
#34765=EDGE_CURVE('',#27564,#27566,#13893,.T.);
#34766=EDGE_CURVE('',#27567,#27563,#13894,.T.);
#34767=EDGE_CURVE('',#27567,#27568,#13895,.T.);
#34768=EDGE_CURVE('',#27568,#27565,#13896,.T.);
#34769=EDGE_CURVE('',#27569,#27567,#13897,.T.);
#34770=EDGE_CURVE('',#27569,#27570,#13898,.T.);
#34771=EDGE_CURVE('',#27570,#27568,#13899,.T.);
#34772=EDGE_CURVE('',#27564,#27569,#13900,.T.);
#34773=EDGE_CURVE('',#27566,#27570,#13901,.T.);
#34774=EDGE_CURVE('',#27571,#27572,#13902,.T.);
#34775=EDGE_CURVE('',#27571,#27573,#13903,.T.);
#34776=EDGE_CURVE('',#27573,#27574,#13904,.T.);
#34777=EDGE_CURVE('',#27572,#27574,#13905,.T.);
#34778=EDGE_CURVE('',#27575,#27571,#13906,.T.);
#34779=EDGE_CURVE('',#27575,#27576,#13907,.T.);
#34780=EDGE_CURVE('',#27576,#27573,#13908,.T.);
#34781=EDGE_CURVE('',#27577,#27575,#13909,.T.);
#34782=EDGE_CURVE('',#27577,#27578,#13910,.T.);
#34783=EDGE_CURVE('',#27578,#27576,#13911,.T.);
#34784=EDGE_CURVE('',#27572,#27577,#13912,.T.);
#34785=EDGE_CURVE('',#27574,#27578,#13913,.T.);
#34786=EDGE_CURVE('',#27579,#27580,#13914,.T.);
#34787=EDGE_CURVE('',#27579,#27581,#13915,.T.);
#34788=EDGE_CURVE('',#27581,#27582,#13916,.T.);
#34789=EDGE_CURVE('',#27580,#27582,#13917,.T.);
#34790=EDGE_CURVE('',#27583,#27579,#13918,.T.);
#34791=EDGE_CURVE('',#27583,#27584,#13919,.T.);
#34792=EDGE_CURVE('',#27584,#27581,#13920,.T.);
#34793=EDGE_CURVE('',#27585,#27583,#13921,.T.);
#34794=EDGE_CURVE('',#27585,#27586,#13922,.T.);
#34795=EDGE_CURVE('',#27586,#27584,#13923,.T.);
#34796=EDGE_CURVE('',#27580,#27585,#13924,.T.);
#34797=EDGE_CURVE('',#27582,#27586,#13925,.T.);
#34798=EDGE_CURVE('',#27587,#27588,#13926,.T.);
#34799=EDGE_CURVE('',#27587,#27589,#13927,.T.);
#34800=EDGE_CURVE('',#27589,#27590,#13928,.T.);
#34801=EDGE_CURVE('',#27588,#27590,#13929,.T.);
#34802=EDGE_CURVE('',#27591,#27587,#13930,.T.);
#34803=EDGE_CURVE('',#27591,#27592,#13931,.T.);
#34804=EDGE_CURVE('',#27592,#27589,#13932,.T.);
#34805=EDGE_CURVE('',#27593,#27591,#13933,.T.);
#34806=EDGE_CURVE('',#27593,#27594,#13934,.T.);
#34807=EDGE_CURVE('',#27594,#27592,#13935,.T.);
#34808=EDGE_CURVE('',#27588,#27593,#13936,.T.);
#34809=EDGE_CURVE('',#27590,#27594,#13937,.T.);
#34810=EDGE_CURVE('',#27595,#27596,#13938,.T.);
#34811=EDGE_CURVE('',#27595,#27597,#13939,.T.);
#34812=EDGE_CURVE('',#27597,#27598,#13940,.T.);
#34813=EDGE_CURVE('',#27596,#27598,#13941,.T.);
#34814=EDGE_CURVE('',#27599,#27595,#13942,.T.);
#34815=EDGE_CURVE('',#27599,#27600,#13943,.T.);
#34816=EDGE_CURVE('',#27600,#27597,#13944,.T.);
#34817=EDGE_CURVE('',#27601,#27599,#13945,.T.);
#34818=EDGE_CURVE('',#27601,#27602,#13946,.T.);
#34819=EDGE_CURVE('',#27602,#27600,#13947,.T.);
#34820=EDGE_CURVE('',#27596,#27601,#13948,.T.);
#34821=EDGE_CURVE('',#27598,#27602,#13949,.T.);
#34822=EDGE_CURVE('',#27603,#27604,#13950,.T.);
#34823=EDGE_CURVE('',#27603,#27605,#13951,.T.);
#34824=EDGE_CURVE('',#27605,#27606,#13952,.T.);
#34825=EDGE_CURVE('',#27604,#27606,#13953,.T.);
#34826=EDGE_CURVE('',#27607,#27603,#13954,.T.);
#34827=EDGE_CURVE('',#27607,#27608,#13955,.T.);
#34828=EDGE_CURVE('',#27608,#27605,#13956,.T.);
#34829=EDGE_CURVE('',#27609,#27607,#13957,.T.);
#34830=EDGE_CURVE('',#27609,#27610,#13958,.T.);
#34831=EDGE_CURVE('',#27610,#27608,#13959,.T.);
#34832=EDGE_CURVE('',#27604,#27609,#13960,.T.);
#34833=EDGE_CURVE('',#27606,#27610,#13961,.T.);
#34834=EDGE_CURVE('',#27611,#27612,#13962,.T.);
#34835=EDGE_CURVE('',#27611,#27613,#13963,.T.);
#34836=EDGE_CURVE('',#27613,#27614,#13964,.T.);
#34837=EDGE_CURVE('',#27612,#27614,#13965,.T.);
#34838=EDGE_CURVE('',#27615,#27611,#13966,.T.);
#34839=EDGE_CURVE('',#27615,#27616,#13967,.T.);
#34840=EDGE_CURVE('',#27616,#27613,#13968,.T.);
#34841=EDGE_CURVE('',#27617,#27615,#13969,.T.);
#34842=EDGE_CURVE('',#27617,#27618,#13970,.T.);
#34843=EDGE_CURVE('',#27618,#27616,#13971,.T.);
#34844=EDGE_CURVE('',#27612,#27617,#13972,.T.);
#34845=EDGE_CURVE('',#27614,#27618,#13973,.T.);
#34846=EDGE_CURVE('',#27619,#27620,#13974,.T.);
#34847=EDGE_CURVE('',#27619,#27621,#13975,.T.);
#34848=EDGE_CURVE('',#27621,#27622,#13976,.T.);
#34849=EDGE_CURVE('',#27620,#27622,#13977,.T.);
#34850=EDGE_CURVE('',#27623,#27619,#13978,.T.);
#34851=EDGE_CURVE('',#27623,#27624,#13979,.T.);
#34852=EDGE_CURVE('',#27624,#27621,#13980,.T.);
#34853=EDGE_CURVE('',#27625,#27623,#13981,.T.);
#34854=EDGE_CURVE('',#27625,#27626,#13982,.T.);
#34855=EDGE_CURVE('',#27626,#27624,#13983,.T.);
#34856=EDGE_CURVE('',#27620,#27625,#13984,.T.);
#34857=EDGE_CURVE('',#27622,#27626,#13985,.T.);
#34858=EDGE_CURVE('',#27627,#27628,#13986,.T.);
#34859=EDGE_CURVE('',#27629,#27627,#13987,.T.);
#34860=EDGE_CURVE('',#27629,#27630,#13988,.T.);
#34861=EDGE_CURVE('',#27631,#27630,#13989,.T.);
#34862=EDGE_CURVE('',#27632,#27631,#13990,.T.);
#34863=EDGE_CURVE('',#27628,#27632,#13991,.T.);
#34864=EDGE_CURVE('',#27633,#27634,#13992,.T.);
#34865=EDGE_CURVE('',#27635,#27633,#13993,.T.);
#34866=EDGE_CURVE('',#27636,#27635,#13994,.T.);
#34867=EDGE_CURVE('',#27637,#27636,#13995,.T.);
#34868=EDGE_CURVE('',#27637,#27638,#13996,.T.);
#34869=EDGE_CURVE('',#27634,#27638,#13997,.T.);
#34870=EDGE_CURVE('',#27630,#27637,#13998,.T.);
#34871=EDGE_CURVE('',#27638,#27629,#13999,.T.);
#34872=EDGE_CURVE('',#27639,#27636,#14000,.T.);
#34873=EDGE_CURVE('',#27640,#27639,#14001,.T.);
#34874=EDGE_CURVE('',#27641,#27640,#14002,.T.);
#34875=EDGE_CURVE('',#27642,#27641,#14003,.T.);
#34876=EDGE_CURVE('',#27643,#27642,#14004,.T.);
#34877=EDGE_CURVE('',#27643,#27644,#957,.T.);
#34878=EDGE_CURVE('',#27645,#27644,#14005,.T.);
#34879=EDGE_CURVE('',#27646,#27645,#14006,.T.);
#34880=EDGE_CURVE('',#27647,#27646,#14007,.T.);
#34881=EDGE_CURVE('',#27648,#27647,#14008,.T.);
#34882=EDGE_CURVE('',#27649,#27648,#14009,.T.);
#34883=EDGE_CURVE('',#27650,#27649,#14010,.T.);
#34884=EDGE_CURVE('',#27651,#27650,#14011,.T.);
#34885=EDGE_CURVE('',#27652,#27651,#14012,.T.);
#34886=EDGE_CURVE('',#27653,#27652,#14013,.T.);
#34887=EDGE_CURVE('',#27653,#27654,#958,.T.);
#34888=EDGE_CURVE('',#27655,#27654,#14014,.T.);
#34889=EDGE_CURVE('',#27656,#27655,#14015,.T.);
#34890=EDGE_CURVE('',#27657,#27656,#14016,.T.);
#34891=EDGE_CURVE('',#27658,#27657,#14017,.T.);
#34892=EDGE_CURVE('',#27631,#27658,#14018,.T.);
#34893=EDGE_CURVE('',#27634,#27659,#14019,.T.);
#34894=EDGE_CURVE('',#27659,#27660,#14020,.T.);
#34895=EDGE_CURVE('',#27660,#27633,#14021,.T.);
#34896=EDGE_CURVE('',#27628,#27661,#14022,.T.);
#34897=EDGE_CURVE('',#27662,#27661,#14023,.T.);
#34898=EDGE_CURVE('',#27662,#27627,#14024,.T.);
#34899=EDGE_CURVE('',#27635,#27663,#14025,.T.);
#34900=EDGE_CURVE('',#27639,#27663,#14026,.T.);
#34901=EDGE_CURVE('',#27663,#27660,#14027,.T.);
#34902=EDGE_CURVE('',#27664,#27664,#959,.T.);
#34903=EDGE_CURVE('',#27665,#27665,#960,.T.);
#34904=EDGE_CURVE('',#27666,#27666,#961,.T.);
#34905=EDGE_CURVE('',#27667,#27667,#962,.T.);
#34906=EDGE_CURVE('',#27667,#27668,#14028,.T.);
#34907=EDGE_CURVE('',#27669,#27669,#963,.T.);
#34908=EDGE_CURVE('',#27669,#27670,#14029,.T.);
#34909=EDGE_CURVE('',#27671,#27671,#964,.T.);
#34910=EDGE_CURVE('',#27671,#27669,#14030,.T.);
#34911=EDGE_CURVE('',#27672,#27672,#965,.T.);
#34912=EDGE_CURVE('',#27672,#27667,#14031,.T.);
#34913=EDGE_CURVE('',#27673,#27673,#966,.T.);
#34914=EDGE_CURVE('',#27673,#27674,#14032,.T.);
#34915=EDGE_CURVE('',#27674,#27674,#967,.T.);
#34916=EDGE_CURVE('',#27674,#27675,#14033,.T.);
#34917=EDGE_CURVE('',#27675,#27675,#968,.T.);
#34918=EDGE_CURVE('',#27676,#27677,#14034,.T.);
#34919=EDGE_CURVE('',#27678,#27676,#14035,.T.);
#34920=EDGE_CURVE('',#27679,#27678,#14036,.T.);
#34921=EDGE_CURVE('',#27679,#27677,#14037,.T.);
#34922=EDGE_CURVE('',#27680,#27680,#969,.T.);
#34923=EDGE_CURVE('',#27675,#27681,#14038,.T.);
#34924=EDGE_CURVE('',#27680,#27682,#14039,.T.);
#34925=EDGE_CURVE('',#27682,#27682,#970,.T.);
#34926=EDGE_CURVE('',#27682,#27683,#14040,.T.);
#34927=EDGE_CURVE('',#27683,#27683,#971,.T.);
#34928=EDGE_CURVE('',#27683,#27684,#14041,.T.);
#34929=EDGE_CURVE('',#27685,#27685,#972,.T.);
#34930=EDGE_CURVE('',#27685,#27686,#14042,.T.);
#34931=EDGE_CURVE('',#27686,#27686,#973,.T.);
#34932=EDGE_CURVE('',#27687,#27687,#974,.T.);
#34933=EDGE_CURVE('',#27688,#27688,#975,.T.);
#34934=EDGE_CURVE('',#27688,#27689,#14043,.T.);
#34935=EDGE_CURVE('',#27689,#27689,#976,.T.);
#34936=EDGE_CURVE('',#27690,#27690,#977,.T.);
#34937=EDGE_CURVE('',#27691,#27691,#978,.T.);
#34938=EDGE_CURVE('',#27691,#27692,#14044,.T.);
#34939=EDGE_CURVE('',#27692,#27692,#979,.T.);
#34940=EDGE_CURVE('',#27693,#27693,#980,.T.);
#34941=EDGE_CURVE('',#27694,#27694,#981,.T.);
#34942=EDGE_CURVE('',#27694,#27695,#14045,.T.);
#34943=EDGE_CURVE('',#27695,#27695,#982,.T.);
#34944=EDGE_CURVE('',#27696,#27696,#983,.T.);
#34945=EDGE_CURVE('',#27697,#27697,#984,.T.);
#34946=EDGE_CURVE('',#27697,#27698,#14046,.T.);
#34947=EDGE_CURVE('',#27698,#27698,#985,.T.);
#34948=EDGE_CURVE('',#27699,#27699,#986,.T.);
#34949=EDGE_CURVE('',#27700,#27700,#987,.T.);
#34950=EDGE_CURVE('',#27700,#27701,#14047,.T.);
#34951=EDGE_CURVE('',#27701,#27701,#988,.T.);
#34952=EDGE_CURVE('',#27702,#27702,#989,.T.);
#34953=EDGE_CURVE('',#27666,#27703,#14048,.T.);
#34954=EDGE_CURVE('',#27703,#27703,#990,.T.);
#34955=EDGE_CURVE('',#27704,#27632,#14049,.T.);
#34956=EDGE_CURVE('',#27661,#27704,#14050,.T.);
#34957=EDGE_CURVE('',#27705,#27705,#991,.T.);
#34958=EDGE_CURVE('',#27706,#27706,#992,.T.);
#34959=EDGE_CURVE('',#27707,#27707,#993,.T.);
#34960=EDGE_CURVE('',#27703,#27702,#14051,.T.);
#34961=EDGE_CURVE('',#27664,#27708,#14052,.T.);
#34962=EDGE_CURVE('',#27708,#27708,#994,.T.);
#34963=EDGE_CURVE('',#27708,#27699,#14053,.T.);
#34964=EDGE_CURVE('',#27707,#27709,#14054,.T.);
#34965=EDGE_CURVE('',#27709,#27709,#995,.T.);
#34966=EDGE_CURVE('',#27709,#27696,#14055,.T.);
#34967=EDGE_CURVE('',#27665,#27710,#14056,.T.);
#34968=EDGE_CURVE('',#27710,#27710,#996,.T.);
#34969=EDGE_CURVE('',#27710,#27693,#14057,.T.);
#34970=EDGE_CURVE('',#27706,#27711,#14058,.T.);
#34971=EDGE_CURVE('',#27711,#27711,#997,.T.);
#34972=EDGE_CURVE('',#27711,#27690,#14059,.T.);
#34973=EDGE_CURVE('',#27705,#27712,#14060,.T.);
#34974=EDGE_CURVE('',#27712,#27712,#998,.T.);
#34975=EDGE_CURVE('',#27712,#27687,#14061,.T.);
#34976=EDGE_CURVE('',#27713,#27714,#14062,.T.);
#34977=EDGE_CURVE('',#27714,#27715,#587,.T.);
#34978=EDGE_CURVE('',#27715,#27716,#14063,.T.);
#34979=EDGE_CURVE('',#27716,#27713,#14064,.T.);
#34980=EDGE_CURVE('',#27716,#27717,#14065,.T.);
#34981=EDGE_CURVE('',#27717,#27718,#14066,.T.);
#34982=EDGE_CURVE('',#27718,#27713,#14067,.T.);
#34983=EDGE_CURVE('',#27717,#27719,#14068,.T.);
#34984=EDGE_CURVE('',#27719,#27720,#14069,.T.);
#34985=EDGE_CURVE('',#27720,#27718,#14070,.T.);
#34986=EDGE_CURVE('',#27721,#27722,#14071,.T.);
#34987=EDGE_CURVE('',#27722,#27723,#14072,.T.);
#34988=EDGE_CURVE('',#27723,#27676,#14073,.T.);
#34989=EDGE_CURVE('',#27676,#27721,#14074,.T.);
#34990=EDGE_CURVE('',#27722,#27724,#14075,.T.);
#34991=EDGE_CURVE('',#27724,#27725,#14076,.T.);
#34992=EDGE_CURVE('',#27725,#27723,#14077,.T.);
#34993=EDGE_CURVE('',#27724,#27726,#14078,.T.);
#34994=EDGE_CURVE('',#27726,#27727,#14079,.T.);
#34995=EDGE_CURVE('',#27727,#27725,#14080,.T.);
#34996=EDGE_CURVE('',#27726,#27728,#14081,.T.);
#34997=EDGE_CURVE('',#27728,#27729,#588,.T.);
#34998=EDGE_CURVE('',#27729,#27727,#14082,.T.);
#34999=EDGE_CURVE('',#27730,#27721,#14083,.T.);
#35000=EDGE_CURVE('',#27677,#27730,#14084,.T.);
#35001=EDGE_CURVE('',#27719,#27730,#14085,.T.);
#35002=EDGE_CURVE('',#27677,#27720,#14086,.T.);
#35003=EDGE_CURVE('',#27731,#27714,#14087,.T.);
#35004=EDGE_CURVE('',#27644,#27731,#589,.T.);
#35005=EDGE_CURVE('',#27732,#27643,#590,.T.);
#35006=EDGE_CURVE('',#27733,#27732,#14088,.T.);
#35007=EDGE_CURVE('',#27734,#27733,#591,.T.);
#35008=EDGE_CURVE('',#27715,#27734,#999,.T.);
#35009=EDGE_CURVE('',#27735,#27713,#14089,.T.);
#35010=EDGE_CURVE('',#27731,#27735,#14090,.T.);
#35011=EDGE_CURVE('',#27718,#27736,#14091,.T.);
#35012=EDGE_CURVE('',#27735,#27736,#14092,.T.);
#35013=EDGE_CURVE('',#27720,#27737,#14093,.T.);
#35014=EDGE_CURVE('',#27736,#27737,#14094,.T.);
#35015=EDGE_CURVE('',#27737,#27679,#14095,.T.);
#35016=EDGE_CURVE('',#27738,#27723,#14096,.T.);
#35017=EDGE_CURVE('',#27678,#27738,#14097,.T.);
#35018=EDGE_CURVE('',#27739,#27740,#14098,.T.);
#35019=EDGE_CURVE('',#27740,#27741,#592,.T.);
#35020=EDGE_CURVE('',#27741,#27742,#14099,.T.);
#35021=EDGE_CURVE('',#27742,#27739,#14100,.T.);
#35022=EDGE_CURVE('',#27742,#27743,#14101,.T.);
#35023=EDGE_CURVE('',#27743,#27744,#14102,.T.);
#35024=EDGE_CURVE('',#27744,#27739,#14103,.T.);
#35025=EDGE_CURVE('',#27743,#27745,#14104,.T.);
#35026=EDGE_CURVE('',#27745,#27746,#14105,.T.);
#35027=EDGE_CURVE('',#27746,#27744,#14106,.T.);
#35028=EDGE_CURVE('',#27745,#27662,#14107,.T.);
#35029=EDGE_CURVE('',#27661,#27746,#14108,.T.);
#35030=EDGE_CURVE('',#27659,#27747,#14109,.T.);
#35031=EDGE_CURVE('',#27747,#27748,#14110,.T.);
#35032=EDGE_CURVE('',#27748,#27660,#14111,.T.);
#35033=EDGE_CURVE('',#27747,#27749,#14112,.T.);
#35034=EDGE_CURVE('',#27749,#27750,#14113,.T.);
#35035=EDGE_CURVE('',#27750,#27748,#14114,.T.);
#35036=EDGE_CURVE('',#27749,#27751,#14115,.T.);
#35037=EDGE_CURVE('',#27751,#27752,#14116,.T.);
#35038=EDGE_CURVE('',#27752,#27750,#14117,.T.);
#35039=EDGE_CURVE('',#27751,#27734,#14118,.T.);
#35040=EDGE_CURVE('',#27733,#27752,#14119,.T.);
#35041=EDGE_CURVE('',#27753,#27739,#14120,.T.);
#35042=EDGE_CURVE('',#27754,#27753,#14121,.T.);
#35043=EDGE_CURVE('',#27754,#27740,#14122,.T.);
#35044=EDGE_CURVE('',#27744,#27755,#14123,.T.);
#35045=EDGE_CURVE('',#27753,#27755,#14124,.T.);
#35046=EDGE_CURVE('',#27756,#27746,#14125,.T.);
#35047=EDGE_CURVE('',#27755,#27756,#14126,.T.);
#35048=EDGE_CURVE('',#27756,#27704,#14127,.T.);
#35049=EDGE_CURVE('',#27748,#27757,#14128,.T.);
#35050=EDGE_CURVE('',#27663,#27757,#14129,.T.);
#35051=EDGE_CURVE('',#27758,#27750,#14130,.T.);
#35052=EDGE_CURVE('',#27757,#27758,#14131,.T.);
#35053=EDGE_CURVE('',#27752,#27759,#14132,.T.);
#35054=EDGE_CURVE('',#27758,#27759,#14133,.T.);
#35055=EDGE_CURVE('',#27759,#27732,#14134,.T.);
#35056=EDGE_CURVE('',#27760,#27761,#14135,.T.);
#35057=EDGE_CURVE('',#27761,#27653,#593,.T.);
#35058=EDGE_CURVE('',#27652,#27760,#14136,.T.);
#35059=EDGE_CURVE('',#27651,#27762,#14137,.T.);
#35060=EDGE_CURVE('',#27762,#27760,#14138,.T.);
#35061=EDGE_CURVE('',#27650,#27738,#14139,.T.);
#35062=EDGE_CURVE('',#27738,#27762,#14140,.T.);
#35063=EDGE_CURVE('',#27649,#27678,#14141,.T.);
#35064=EDGE_CURVE('',#27648,#27679,#14142,.T.);
#35065=EDGE_CURVE('',#27647,#27737,#14143,.T.);
#35066=EDGE_CURVE('',#27646,#27736,#14144,.T.);
#35067=EDGE_CURVE('',#27645,#27735,#14145,.T.);
#35068=EDGE_CURVE('',#27642,#27759,#14146,.T.);
#35069=EDGE_CURVE('',#27641,#27758,#14147,.T.);
#35070=EDGE_CURVE('',#27640,#27757,#14148,.T.);
#35071=EDGE_CURVE('',#27658,#27704,#14149,.T.);
#35072=EDGE_CURVE('',#27657,#27756,#14150,.T.);
#35073=EDGE_CURVE('',#27656,#27755,#14151,.T.);
#35074=EDGE_CURVE('',#27655,#27753,#14152,.T.);
#35075=EDGE_CURVE('',#27654,#27754,#594,.T.);
#35076=EDGE_CURVE('',#27741,#27728,#1000,.T.);
#35077=EDGE_CURVE('',#27762,#27725,#14153,.T.);
#35078=EDGE_CURVE('',#27729,#27761,#14154,.T.);
#35079=EDGE_CURVE('',#27727,#27760,#14155,.T.);
#39039=ORIENTED_EDGE('',*,*,#30352,.F.);
#39040=ORIENTED_EDGE('',*,*,#30353,.T.);
#39041=ORIENTED_EDGE('',*,*,#30354,.T.);
#39042=ORIENTED_EDGE('',*,*,#30355,.F.);
#39043=ORIENTED_EDGE('',*,*,#30356,.F.);
#39044=ORIENTED_EDGE('',*,*,#30357,.T.);
#39045=ORIENTED_EDGE('',*,*,#30358,.T.);
#39046=ORIENTED_EDGE('',*,*,#30353,.F.);
#39047=ORIENTED_EDGE('',*,*,#30359,.F.);
#39048=ORIENTED_EDGE('',*,*,#30360,.T.);
#39049=ORIENTED_EDGE('',*,*,#30361,.T.);
#39050=ORIENTED_EDGE('',*,*,#30357,.F.);
#39051=ORIENTED_EDGE('',*,*,#30362,.F.);
#39052=ORIENTED_EDGE('',*,*,#30363,.T.);
#39053=ORIENTED_EDGE('',*,*,#30364,.T.);
#39054=ORIENTED_EDGE('',*,*,#30360,.F.);
#39055=ORIENTED_EDGE('',*,*,#30365,.F.);
#39056=ORIENTED_EDGE('',*,*,#30366,.T.);
#39057=ORIENTED_EDGE('',*,*,#30367,.T.);
#39058=ORIENTED_EDGE('',*,*,#30363,.F.);
#39059=ORIENTED_EDGE('',*,*,#30368,.F.);
#39060=ORIENTED_EDGE('',*,*,#30369,.T.);
#39061=ORIENTED_EDGE('',*,*,#30370,.T.);
#39062=ORIENTED_EDGE('',*,*,#30366,.F.);
#39063=ORIENTED_EDGE('',*,*,#30371,.F.);
#39064=ORIENTED_EDGE('',*,*,#30372,.T.);
#39065=ORIENTED_EDGE('',*,*,#30373,.T.);
#39066=ORIENTED_EDGE('',*,*,#30369,.F.);
#39067=ORIENTED_EDGE('',*,*,#30374,.F.);
#39068=ORIENTED_EDGE('',*,*,#30355,.T.);
#39069=ORIENTED_EDGE('',*,*,#30375,.T.);
#39070=ORIENTED_EDGE('',*,*,#30372,.F.);
#39071=ORIENTED_EDGE('',*,*,#30376,.F.);
#39072=ORIENTED_EDGE('',*,*,#30377,.T.);
#39073=ORIENTED_EDGE('',*,*,#30378,.T.);
#39074=ORIENTED_EDGE('',*,*,#30379,.F.);
#39075=ORIENTED_EDGE('',*,*,#30380,.F.);
#39076=ORIENTED_EDGE('',*,*,#30381,.T.);
#39077=ORIENTED_EDGE('',*,*,#30382,.T.);
#39078=ORIENTED_EDGE('',*,*,#30377,.F.);
#39079=ORIENTED_EDGE('',*,*,#30383,.F.);
#39080=ORIENTED_EDGE('',*,*,#30384,.T.);
#39081=ORIENTED_EDGE('',*,*,#30385,.T.);
#39082=ORIENTED_EDGE('',*,*,#30381,.F.);
#39083=ORIENTED_EDGE('',*,*,#30386,.F.);
#39084=ORIENTED_EDGE('',*,*,#30387,.T.);
#39085=ORIENTED_EDGE('',*,*,#30388,.T.);
#39086=ORIENTED_EDGE('',*,*,#30384,.F.);
#39087=ORIENTED_EDGE('',*,*,#30389,.F.);
#39088=ORIENTED_EDGE('',*,*,#30390,.T.);
#39089=ORIENTED_EDGE('',*,*,#30391,.T.);
#39090=ORIENTED_EDGE('',*,*,#30387,.F.);
#39091=ORIENTED_EDGE('',*,*,#30392,.F.);
#39092=ORIENTED_EDGE('',*,*,#30393,.T.);
#39093=ORIENTED_EDGE('',*,*,#30394,.T.);
#39094=ORIENTED_EDGE('',*,*,#30390,.F.);
#39095=ORIENTED_EDGE('',*,*,#30395,.F.);
#39096=ORIENTED_EDGE('',*,*,#30396,.T.);
#39097=ORIENTED_EDGE('',*,*,#30397,.T.);
#39098=ORIENTED_EDGE('',*,*,#30393,.F.);
#39099=ORIENTED_EDGE('',*,*,#30398,.F.);
#39100=ORIENTED_EDGE('',*,*,#30399,.T.);
#39101=ORIENTED_EDGE('',*,*,#30400,.T.);
#39102=ORIENTED_EDGE('',*,*,#30396,.F.);
#39103=ORIENTED_EDGE('',*,*,#30401,.F.);
#39104=ORIENTED_EDGE('',*,*,#30402,.T.);
#39105=ORIENTED_EDGE('',*,*,#30403,.T.);
#39106=ORIENTED_EDGE('',*,*,#30399,.F.);
#39107=ORIENTED_EDGE('',*,*,#30404,.F.);
#39108=ORIENTED_EDGE('',*,*,#30405,.T.);
#39109=ORIENTED_EDGE('',*,*,#30406,.T.);
#39110=ORIENTED_EDGE('',*,*,#30402,.F.);
#39111=ORIENTED_EDGE('',*,*,#30407,.F.);
#39112=ORIENTED_EDGE('',*,*,#30408,.T.);
#39113=ORIENTED_EDGE('',*,*,#30409,.T.);
#39114=ORIENTED_EDGE('',*,*,#30405,.F.);
#39115=ORIENTED_EDGE('',*,*,#30410,.F.);
#39116=ORIENTED_EDGE('',*,*,#30379,.T.);
#39117=ORIENTED_EDGE('',*,*,#30411,.T.);
#39118=ORIENTED_EDGE('',*,*,#30408,.F.);
#39119=ORIENTED_EDGE('',*,*,#30411,.F.);
#39120=ORIENTED_EDGE('',*,*,#30378,.F.);
#39121=ORIENTED_EDGE('',*,*,#30382,.F.);
#39122=ORIENTED_EDGE('',*,*,#30385,.F.);
#39123=ORIENTED_EDGE('',*,*,#30388,.F.);
#39124=ORIENTED_EDGE('',*,*,#30391,.F.);
#39125=ORIENTED_EDGE('',*,*,#30394,.F.);
#39126=ORIENTED_EDGE('',*,*,#30397,.F.);
#39127=ORIENTED_EDGE('',*,*,#30400,.F.);
#39128=ORIENTED_EDGE('',*,*,#30403,.F.);
#39129=ORIENTED_EDGE('',*,*,#30406,.F.);
#39130=ORIENTED_EDGE('',*,*,#30409,.F.);
#39131=ORIENTED_EDGE('',*,*,#30375,.F.);
#39132=ORIENTED_EDGE('',*,*,#30354,.F.);
#39133=ORIENTED_EDGE('',*,*,#30358,.F.);
#39134=ORIENTED_EDGE('',*,*,#30361,.F.);
#39135=ORIENTED_EDGE('',*,*,#30364,.F.);
#39136=ORIENTED_EDGE('',*,*,#30367,.F.);
#39137=ORIENTED_EDGE('',*,*,#30370,.F.);
#39138=ORIENTED_EDGE('',*,*,#30373,.F.);
#39139=ORIENTED_EDGE('',*,*,#30412,.F.);
#39140=ORIENTED_EDGE('',*,*,#30413,.T.);
#39141=ORIENTED_EDGE('',*,*,#30414,.T.);
#39142=ORIENTED_EDGE('',*,*,#30415,.F.);
#39143=ORIENTED_EDGE('',*,*,#30416,.F.);
#39144=ORIENTED_EDGE('',*,*,#30417,.T.);
#39145=ORIENTED_EDGE('',*,*,#30418,.T.);
#39146=ORIENTED_EDGE('',*,*,#30413,.F.);
#39147=ORIENTED_EDGE('',*,*,#30419,.F.);
#39148=ORIENTED_EDGE('',*,*,#30420,.T.);
#39149=ORIENTED_EDGE('',*,*,#30421,.T.);
#39150=ORIENTED_EDGE('',*,*,#30417,.F.);
#39151=ORIENTED_EDGE('',*,*,#30422,.F.);
#39152=ORIENTED_EDGE('',*,*,#30423,.T.);
#39153=ORIENTED_EDGE('',*,*,#30424,.T.);
#39154=ORIENTED_EDGE('',*,*,#30420,.F.);
#39155=ORIENTED_EDGE('',*,*,#30425,.F.);
#39156=ORIENTED_EDGE('',*,*,#30426,.T.);
#39157=ORIENTED_EDGE('',*,*,#30427,.T.);
#39158=ORIENTED_EDGE('',*,*,#30423,.F.);
#39159=ORIENTED_EDGE('',*,*,#30428,.F.);
#39160=ORIENTED_EDGE('',*,*,#30429,.T.);
#39161=ORIENTED_EDGE('',*,*,#30430,.T.);
#39162=ORIENTED_EDGE('',*,*,#30426,.F.);
#39163=ORIENTED_EDGE('',*,*,#30431,.F.);
#39164=ORIENTED_EDGE('',*,*,#30432,.T.);
#39165=ORIENTED_EDGE('',*,*,#30433,.T.);
#39166=ORIENTED_EDGE('',*,*,#30429,.F.);
#39167=ORIENTED_EDGE('',*,*,#30434,.F.);
#39168=ORIENTED_EDGE('',*,*,#30415,.T.);
#39169=ORIENTED_EDGE('',*,*,#30435,.T.);
#39170=ORIENTED_EDGE('',*,*,#30432,.F.);
#39171=ORIENTED_EDGE('',*,*,#30436,.F.);
#39172=ORIENTED_EDGE('',*,*,#30437,.T.);
#39173=ORIENTED_EDGE('',*,*,#30438,.T.);
#39174=ORIENTED_EDGE('',*,*,#30439,.F.);
#39175=ORIENTED_EDGE('',*,*,#30440,.F.);
#39176=ORIENTED_EDGE('',*,*,#30441,.T.);
#39177=ORIENTED_EDGE('',*,*,#30442,.T.);
#39178=ORIENTED_EDGE('',*,*,#30437,.F.);
#39179=ORIENTED_EDGE('',*,*,#30443,.F.);
#39180=ORIENTED_EDGE('',*,*,#30444,.T.);
#39181=ORIENTED_EDGE('',*,*,#30445,.T.);
#39182=ORIENTED_EDGE('',*,*,#30441,.F.);
#39183=ORIENTED_EDGE('',*,*,#30446,.F.);
#39184=ORIENTED_EDGE('',*,*,#30447,.T.);
#39185=ORIENTED_EDGE('',*,*,#30448,.T.);
#39186=ORIENTED_EDGE('',*,*,#30444,.F.);
#39187=ORIENTED_EDGE('',*,*,#30449,.F.);
#39188=ORIENTED_EDGE('',*,*,#30450,.T.);
#39189=ORIENTED_EDGE('',*,*,#30451,.T.);
#39190=ORIENTED_EDGE('',*,*,#30447,.F.);
#39191=ORIENTED_EDGE('',*,*,#30452,.F.);
#39192=ORIENTED_EDGE('',*,*,#30453,.T.);
#39193=ORIENTED_EDGE('',*,*,#30454,.T.);
#39194=ORIENTED_EDGE('',*,*,#30450,.F.);
#39195=ORIENTED_EDGE('',*,*,#30455,.F.);
#39196=ORIENTED_EDGE('',*,*,#30456,.T.);
#39197=ORIENTED_EDGE('',*,*,#30457,.T.);
#39198=ORIENTED_EDGE('',*,*,#30453,.F.);
#39199=ORIENTED_EDGE('',*,*,#30458,.F.);
#39200=ORIENTED_EDGE('',*,*,#30459,.T.);
#39201=ORIENTED_EDGE('',*,*,#30460,.T.);
#39202=ORIENTED_EDGE('',*,*,#30456,.F.);
#39203=ORIENTED_EDGE('',*,*,#30461,.F.);
#39204=ORIENTED_EDGE('',*,*,#30462,.T.);
#39205=ORIENTED_EDGE('',*,*,#30463,.T.);
#39206=ORIENTED_EDGE('',*,*,#30459,.F.);
#39207=ORIENTED_EDGE('',*,*,#30464,.F.);
#39208=ORIENTED_EDGE('',*,*,#30465,.T.);
#39209=ORIENTED_EDGE('',*,*,#30466,.T.);
#39210=ORIENTED_EDGE('',*,*,#30462,.F.);
#39211=ORIENTED_EDGE('',*,*,#30467,.F.);
#39212=ORIENTED_EDGE('',*,*,#30468,.T.);
#39213=ORIENTED_EDGE('',*,*,#30469,.T.);
#39214=ORIENTED_EDGE('',*,*,#30465,.F.);
#39215=ORIENTED_EDGE('',*,*,#30470,.F.);
#39216=ORIENTED_EDGE('',*,*,#30471,.T.);
#39217=ORIENTED_EDGE('',*,*,#30472,.T.);
#39218=ORIENTED_EDGE('',*,*,#30468,.F.);
#39219=ORIENTED_EDGE('',*,*,#30473,.F.);
#39220=ORIENTED_EDGE('',*,*,#30474,.T.);
#39221=ORIENTED_EDGE('',*,*,#30475,.T.);
#39222=ORIENTED_EDGE('',*,*,#30471,.F.);
#39223=ORIENTED_EDGE('',*,*,#30476,.F.);
#39224=ORIENTED_EDGE('',*,*,#30477,.T.);
#39225=ORIENTED_EDGE('',*,*,#30478,.T.);
#39226=ORIENTED_EDGE('',*,*,#30474,.F.);
#39227=ORIENTED_EDGE('',*,*,#30479,.F.);
#39228=ORIENTED_EDGE('',*,*,#30480,.T.);
#39229=ORIENTED_EDGE('',*,*,#30481,.T.);
#39230=ORIENTED_EDGE('',*,*,#30477,.F.);
#39231=ORIENTED_EDGE('',*,*,#30482,.F.);
#39232=ORIENTED_EDGE('',*,*,#30483,.T.);
#39233=ORIENTED_EDGE('',*,*,#30484,.T.);
#39234=ORIENTED_EDGE('',*,*,#30480,.F.);
#39235=ORIENTED_EDGE('',*,*,#30485,.F.);
#39236=ORIENTED_EDGE('',*,*,#30486,.T.);
#39237=ORIENTED_EDGE('',*,*,#30487,.T.);
#39238=ORIENTED_EDGE('',*,*,#30483,.F.);
#39239=ORIENTED_EDGE('',*,*,#30488,.F.);
#39240=ORIENTED_EDGE('',*,*,#30489,.T.);
#39241=ORIENTED_EDGE('',*,*,#30490,.T.);
#39242=ORIENTED_EDGE('',*,*,#30486,.F.);
#39243=ORIENTED_EDGE('',*,*,#30491,.F.);
#39244=ORIENTED_EDGE('',*,*,#30492,.T.);
#39245=ORIENTED_EDGE('',*,*,#30493,.T.);
#39246=ORIENTED_EDGE('',*,*,#30489,.F.);
#39247=ORIENTED_EDGE('',*,*,#30494,.F.);
#39248=ORIENTED_EDGE('',*,*,#30495,.T.);
#39249=ORIENTED_EDGE('',*,*,#30496,.T.);
#39250=ORIENTED_EDGE('',*,*,#30492,.F.);
#39251=ORIENTED_EDGE('',*,*,#30497,.F.);
#39252=ORIENTED_EDGE('',*,*,#30498,.T.);
#39253=ORIENTED_EDGE('',*,*,#30499,.T.);
#39254=ORIENTED_EDGE('',*,*,#30495,.F.);
#39255=ORIENTED_EDGE('',*,*,#30500,.F.);
#39256=ORIENTED_EDGE('',*,*,#30439,.T.);
#39257=ORIENTED_EDGE('',*,*,#30501,.T.);
#39258=ORIENTED_EDGE('',*,*,#30498,.F.);
#39259=ORIENTED_EDGE('',*,*,#30501,.F.);
#39260=ORIENTED_EDGE('',*,*,#30438,.F.);
#39261=ORIENTED_EDGE('',*,*,#30442,.F.);
#39262=ORIENTED_EDGE('',*,*,#30445,.F.);
#39263=ORIENTED_EDGE('',*,*,#30448,.F.);
#39264=ORIENTED_EDGE('',*,*,#30451,.F.);
#39265=ORIENTED_EDGE('',*,*,#30454,.F.);
#39266=ORIENTED_EDGE('',*,*,#30457,.F.);
#39267=ORIENTED_EDGE('',*,*,#30460,.F.);
#39268=ORIENTED_EDGE('',*,*,#30463,.F.);
#39269=ORIENTED_EDGE('',*,*,#30466,.F.);
#39270=ORIENTED_EDGE('',*,*,#30469,.F.);
#39271=ORIENTED_EDGE('',*,*,#30472,.F.);
#39272=ORIENTED_EDGE('',*,*,#30475,.F.);
#39273=ORIENTED_EDGE('',*,*,#30478,.F.);
#39274=ORIENTED_EDGE('',*,*,#30481,.F.);
#39275=ORIENTED_EDGE('',*,*,#30484,.F.);
#39276=ORIENTED_EDGE('',*,*,#30487,.F.);
#39277=ORIENTED_EDGE('',*,*,#30490,.F.);
#39278=ORIENTED_EDGE('',*,*,#30493,.F.);
#39279=ORIENTED_EDGE('',*,*,#30496,.F.);
#39280=ORIENTED_EDGE('',*,*,#30499,.F.);
#39281=ORIENTED_EDGE('',*,*,#30435,.F.);
#39282=ORIENTED_EDGE('',*,*,#30414,.F.);
#39283=ORIENTED_EDGE('',*,*,#30418,.F.);
#39284=ORIENTED_EDGE('',*,*,#30421,.F.);
#39285=ORIENTED_EDGE('',*,*,#30424,.F.);
#39286=ORIENTED_EDGE('',*,*,#30427,.F.);
#39287=ORIENTED_EDGE('',*,*,#30430,.F.);
#39288=ORIENTED_EDGE('',*,*,#30433,.F.);
#39289=ORIENTED_EDGE('',*,*,#30412,.T.);
#39290=ORIENTED_EDGE('',*,*,#30434,.T.);
#39291=ORIENTED_EDGE('',*,*,#30431,.T.);
#39292=ORIENTED_EDGE('',*,*,#30428,.T.);
#39293=ORIENTED_EDGE('',*,*,#30425,.T.);
#39294=ORIENTED_EDGE('',*,*,#30422,.T.);
#39295=ORIENTED_EDGE('',*,*,#30419,.T.);
#39296=ORIENTED_EDGE('',*,*,#30416,.T.);
#39297=ORIENTED_EDGE('',*,*,#30352,.T.);
#39298=ORIENTED_EDGE('',*,*,#30374,.T.);
#39299=ORIENTED_EDGE('',*,*,#30371,.T.);
#39300=ORIENTED_EDGE('',*,*,#30368,.T.);
#39301=ORIENTED_EDGE('',*,*,#30365,.T.);
#39302=ORIENTED_EDGE('',*,*,#30362,.T.);
#39303=ORIENTED_EDGE('',*,*,#30359,.T.);
#39304=ORIENTED_EDGE('',*,*,#30356,.T.);
#39305=ORIENTED_EDGE('',*,*,#30502,.F.);
#39306=ORIENTED_EDGE('',*,*,#30503,.T.);
#39307=ORIENTED_EDGE('',*,*,#30504,.T.);
#39308=ORIENTED_EDGE('',*,*,#30505,.F.);
#39309=ORIENTED_EDGE('',*,*,#30506,.F.);
#39310=ORIENTED_EDGE('',*,*,#30507,.T.);
#39311=ORIENTED_EDGE('',*,*,#30508,.T.);
#39312=ORIENTED_EDGE('',*,*,#30503,.F.);
#39313=ORIENTED_EDGE('',*,*,#30509,.F.);
#39314=ORIENTED_EDGE('',*,*,#30510,.T.);
#39315=ORIENTED_EDGE('',*,*,#30511,.T.);
#39316=ORIENTED_EDGE('',*,*,#30507,.F.);
#39317=ORIENTED_EDGE('',*,*,#30512,.F.);
#39318=ORIENTED_EDGE('',*,*,#30513,.T.);
#39319=ORIENTED_EDGE('',*,*,#30514,.T.);
#39320=ORIENTED_EDGE('',*,*,#30510,.F.);
#39321=ORIENTED_EDGE('',*,*,#30515,.F.);
#39322=ORIENTED_EDGE('',*,*,#30516,.T.);
#39323=ORIENTED_EDGE('',*,*,#30517,.T.);
#39324=ORIENTED_EDGE('',*,*,#30513,.F.);
#39325=ORIENTED_EDGE('',*,*,#30518,.F.);
#39326=ORIENTED_EDGE('',*,*,#30519,.T.);
#39327=ORIENTED_EDGE('',*,*,#30520,.T.);
#39328=ORIENTED_EDGE('',*,*,#30516,.F.);
#39329=ORIENTED_EDGE('',*,*,#30521,.F.);
#39330=ORIENTED_EDGE('',*,*,#30522,.T.);
#39331=ORIENTED_EDGE('',*,*,#30523,.T.);
#39332=ORIENTED_EDGE('',*,*,#30519,.F.);
#39333=ORIENTED_EDGE('',*,*,#30524,.F.);
#39334=ORIENTED_EDGE('',*,*,#30505,.T.);
#39335=ORIENTED_EDGE('',*,*,#30525,.T.);
#39336=ORIENTED_EDGE('',*,*,#30522,.F.);
#39337=ORIENTED_EDGE('',*,*,#30526,.F.);
#39338=ORIENTED_EDGE('',*,*,#30527,.T.);
#39339=ORIENTED_EDGE('',*,*,#30528,.T.);
#39340=ORIENTED_EDGE('',*,*,#30529,.F.);
#39341=ORIENTED_EDGE('',*,*,#30530,.F.);
#39342=ORIENTED_EDGE('',*,*,#30531,.T.);
#39343=ORIENTED_EDGE('',*,*,#30532,.T.);
#39344=ORIENTED_EDGE('',*,*,#30527,.F.);
#39345=ORIENTED_EDGE('',*,*,#30533,.F.);
#39346=ORIENTED_EDGE('',*,*,#30534,.T.);
#39347=ORIENTED_EDGE('',*,*,#30535,.T.);
#39348=ORIENTED_EDGE('',*,*,#30531,.F.);
#39349=ORIENTED_EDGE('',*,*,#30536,.F.);
#39350=ORIENTED_EDGE('',*,*,#30537,.T.);
#39351=ORIENTED_EDGE('',*,*,#30538,.T.);
#39352=ORIENTED_EDGE('',*,*,#30534,.F.);
#39353=ORIENTED_EDGE('',*,*,#30539,.F.);
#39354=ORIENTED_EDGE('',*,*,#30540,.T.);
#39355=ORIENTED_EDGE('',*,*,#30541,.T.);
#39356=ORIENTED_EDGE('',*,*,#30537,.F.);
#39357=ORIENTED_EDGE('',*,*,#30542,.F.);
#39358=ORIENTED_EDGE('',*,*,#30543,.T.);
#39359=ORIENTED_EDGE('',*,*,#30544,.T.);
#39360=ORIENTED_EDGE('',*,*,#30540,.F.);
#39361=ORIENTED_EDGE('',*,*,#30545,.F.);
#39362=ORIENTED_EDGE('',*,*,#30546,.T.);
#39363=ORIENTED_EDGE('',*,*,#30547,.T.);
#39364=ORIENTED_EDGE('',*,*,#30543,.F.);
#39365=ORIENTED_EDGE('',*,*,#30548,.F.);
#39366=ORIENTED_EDGE('',*,*,#30549,.T.);
#39367=ORIENTED_EDGE('',*,*,#30550,.T.);
#39368=ORIENTED_EDGE('',*,*,#30546,.F.);
#39369=ORIENTED_EDGE('',*,*,#30551,.F.);
#39370=ORIENTED_EDGE('',*,*,#30552,.T.);
#39371=ORIENTED_EDGE('',*,*,#30553,.T.);
#39372=ORIENTED_EDGE('',*,*,#30549,.F.);
#39373=ORIENTED_EDGE('',*,*,#30554,.F.);
#39374=ORIENTED_EDGE('',*,*,#30555,.T.);
#39375=ORIENTED_EDGE('',*,*,#30556,.T.);
#39376=ORIENTED_EDGE('',*,*,#30552,.F.);
#39377=ORIENTED_EDGE('',*,*,#30557,.F.);
#39378=ORIENTED_EDGE('',*,*,#30558,.T.);
#39379=ORIENTED_EDGE('',*,*,#30559,.T.);
#39380=ORIENTED_EDGE('',*,*,#30555,.F.);
#39381=ORIENTED_EDGE('',*,*,#30560,.F.);
#39382=ORIENTED_EDGE('',*,*,#30529,.T.);
#39383=ORIENTED_EDGE('',*,*,#30561,.T.);
#39384=ORIENTED_EDGE('',*,*,#30558,.F.);
#39385=ORIENTED_EDGE('',*,*,#30561,.F.);
#39386=ORIENTED_EDGE('',*,*,#30528,.F.);
#39387=ORIENTED_EDGE('',*,*,#30532,.F.);
#39388=ORIENTED_EDGE('',*,*,#30535,.F.);
#39389=ORIENTED_EDGE('',*,*,#30538,.F.);
#39390=ORIENTED_EDGE('',*,*,#30541,.F.);
#39391=ORIENTED_EDGE('',*,*,#30544,.F.);
#39392=ORIENTED_EDGE('',*,*,#30547,.F.);
#39393=ORIENTED_EDGE('',*,*,#30550,.F.);
#39394=ORIENTED_EDGE('',*,*,#30553,.F.);
#39395=ORIENTED_EDGE('',*,*,#30556,.F.);
#39396=ORIENTED_EDGE('',*,*,#30559,.F.);
#39397=ORIENTED_EDGE('',*,*,#30525,.F.);
#39398=ORIENTED_EDGE('',*,*,#30504,.F.);
#39399=ORIENTED_EDGE('',*,*,#30508,.F.);
#39400=ORIENTED_EDGE('',*,*,#30511,.F.);
#39401=ORIENTED_EDGE('',*,*,#30514,.F.);
#39402=ORIENTED_EDGE('',*,*,#30517,.F.);
#39403=ORIENTED_EDGE('',*,*,#30520,.F.);
#39404=ORIENTED_EDGE('',*,*,#30523,.F.);
#39405=ORIENTED_EDGE('',*,*,#30562,.F.);
#39406=ORIENTED_EDGE('',*,*,#30563,.T.);
#39407=ORIENTED_EDGE('',*,*,#30564,.T.);
#39408=ORIENTED_EDGE('',*,*,#30565,.F.);
#39409=ORIENTED_EDGE('',*,*,#30566,.F.);
#39410=ORIENTED_EDGE('',*,*,#30567,.T.);
#39411=ORIENTED_EDGE('',*,*,#30568,.T.);
#39412=ORIENTED_EDGE('',*,*,#30563,.F.);
#39413=ORIENTED_EDGE('',*,*,#30569,.F.);
#39414=ORIENTED_EDGE('',*,*,#30570,.T.);
#39415=ORIENTED_EDGE('',*,*,#30571,.T.);
#39416=ORIENTED_EDGE('',*,*,#30567,.F.);
#39417=ORIENTED_EDGE('',*,*,#30572,.F.);
#39418=ORIENTED_EDGE('',*,*,#30573,.T.);
#39419=ORIENTED_EDGE('',*,*,#30574,.T.);
#39420=ORIENTED_EDGE('',*,*,#30570,.F.);
#39421=ORIENTED_EDGE('',*,*,#30575,.F.);
#39422=ORIENTED_EDGE('',*,*,#30576,.T.);
#39423=ORIENTED_EDGE('',*,*,#30577,.T.);
#39424=ORIENTED_EDGE('',*,*,#30573,.F.);
#39425=ORIENTED_EDGE('',*,*,#30578,.F.);
#39426=ORIENTED_EDGE('',*,*,#30579,.T.);
#39427=ORIENTED_EDGE('',*,*,#30580,.T.);
#39428=ORIENTED_EDGE('',*,*,#30576,.F.);
#39429=ORIENTED_EDGE('',*,*,#30581,.F.);
#39430=ORIENTED_EDGE('',*,*,#30582,.T.);
#39431=ORIENTED_EDGE('',*,*,#30583,.T.);
#39432=ORIENTED_EDGE('',*,*,#30579,.F.);
#39433=ORIENTED_EDGE('',*,*,#30584,.F.);
#39434=ORIENTED_EDGE('',*,*,#30565,.T.);
#39435=ORIENTED_EDGE('',*,*,#30585,.T.);
#39436=ORIENTED_EDGE('',*,*,#30582,.F.);
#39437=ORIENTED_EDGE('',*,*,#30586,.F.);
#39438=ORIENTED_EDGE('',*,*,#30587,.T.);
#39439=ORIENTED_EDGE('',*,*,#30588,.T.);
#39440=ORIENTED_EDGE('',*,*,#30589,.F.);
#39441=ORIENTED_EDGE('',*,*,#30590,.F.);
#39442=ORIENTED_EDGE('',*,*,#30591,.T.);
#39443=ORIENTED_EDGE('',*,*,#30592,.T.);
#39444=ORIENTED_EDGE('',*,*,#30587,.F.);
#39445=ORIENTED_EDGE('',*,*,#30593,.F.);
#39446=ORIENTED_EDGE('',*,*,#30594,.T.);
#39447=ORIENTED_EDGE('',*,*,#30595,.T.);
#39448=ORIENTED_EDGE('',*,*,#30591,.F.);
#39449=ORIENTED_EDGE('',*,*,#30596,.F.);
#39450=ORIENTED_EDGE('',*,*,#30597,.T.);
#39451=ORIENTED_EDGE('',*,*,#30598,.T.);
#39452=ORIENTED_EDGE('',*,*,#30594,.F.);
#39453=ORIENTED_EDGE('',*,*,#30599,.F.);
#39454=ORIENTED_EDGE('',*,*,#30600,.T.);
#39455=ORIENTED_EDGE('',*,*,#30601,.T.);
#39456=ORIENTED_EDGE('',*,*,#30597,.F.);
#39457=ORIENTED_EDGE('',*,*,#30602,.F.);
#39458=ORIENTED_EDGE('',*,*,#30603,.T.);
#39459=ORIENTED_EDGE('',*,*,#30604,.T.);
#39460=ORIENTED_EDGE('',*,*,#30600,.F.);
#39461=ORIENTED_EDGE('',*,*,#30605,.F.);
#39462=ORIENTED_EDGE('',*,*,#30606,.T.);
#39463=ORIENTED_EDGE('',*,*,#30607,.T.);
#39464=ORIENTED_EDGE('',*,*,#30603,.F.);
#39465=ORIENTED_EDGE('',*,*,#30608,.F.);
#39466=ORIENTED_EDGE('',*,*,#30609,.T.);
#39467=ORIENTED_EDGE('',*,*,#30610,.T.);
#39468=ORIENTED_EDGE('',*,*,#30606,.F.);
#39469=ORIENTED_EDGE('',*,*,#30611,.F.);
#39470=ORIENTED_EDGE('',*,*,#30589,.T.);
#39471=ORIENTED_EDGE('',*,*,#30612,.T.);
#39472=ORIENTED_EDGE('',*,*,#30609,.F.);
#39473=ORIENTED_EDGE('',*,*,#30613,.F.);
#39474=ORIENTED_EDGE('',*,*,#30614,.T.);
#39475=ORIENTED_EDGE('',*,*,#30615,.T.);
#39476=ORIENTED_EDGE('',*,*,#30616,.F.);
#39477=ORIENTED_EDGE('',*,*,#30617,.F.);
#39478=ORIENTED_EDGE('',*,*,#30618,.T.);
#39479=ORIENTED_EDGE('',*,*,#30619,.T.);
#39480=ORIENTED_EDGE('',*,*,#30614,.F.);
#39481=ORIENTED_EDGE('',*,*,#30620,.F.);
#39482=ORIENTED_EDGE('',*,*,#30621,.T.);
#39483=ORIENTED_EDGE('',*,*,#30622,.T.);
#39484=ORIENTED_EDGE('',*,*,#30618,.F.);
#39485=ORIENTED_EDGE('',*,*,#30623,.F.);
#39486=ORIENTED_EDGE('',*,*,#30624,.T.);
#39487=ORIENTED_EDGE('',*,*,#30625,.T.);
#39488=ORIENTED_EDGE('',*,*,#30621,.F.);
#39489=ORIENTED_EDGE('',*,*,#30626,.F.);
#39490=ORIENTED_EDGE('',*,*,#30627,.T.);
#39491=ORIENTED_EDGE('',*,*,#30628,.T.);
#39492=ORIENTED_EDGE('',*,*,#30624,.F.);
#39493=ORIENTED_EDGE('',*,*,#30629,.F.);
#39494=ORIENTED_EDGE('',*,*,#30630,.T.);
#39495=ORIENTED_EDGE('',*,*,#30631,.T.);
#39496=ORIENTED_EDGE('',*,*,#30627,.F.);
#39497=ORIENTED_EDGE('',*,*,#30632,.F.);
#39498=ORIENTED_EDGE('',*,*,#30633,.T.);
#39499=ORIENTED_EDGE('',*,*,#30634,.T.);
#39500=ORIENTED_EDGE('',*,*,#30630,.F.);
#39501=ORIENTED_EDGE('',*,*,#30635,.F.);
#39502=ORIENTED_EDGE('',*,*,#30636,.T.);
#39503=ORIENTED_EDGE('',*,*,#30637,.T.);
#39504=ORIENTED_EDGE('',*,*,#30633,.F.);
#39505=ORIENTED_EDGE('',*,*,#30638,.F.);
#39506=ORIENTED_EDGE('',*,*,#30639,.T.);
#39507=ORIENTED_EDGE('',*,*,#30640,.T.);
#39508=ORIENTED_EDGE('',*,*,#30636,.F.);
#39509=ORIENTED_EDGE('',*,*,#30641,.F.);
#39510=ORIENTED_EDGE('',*,*,#30642,.T.);
#39511=ORIENTED_EDGE('',*,*,#30643,.T.);
#39512=ORIENTED_EDGE('',*,*,#30639,.F.);
#39513=ORIENTED_EDGE('',*,*,#30644,.F.);
#39514=ORIENTED_EDGE('',*,*,#30645,.T.);
#39515=ORIENTED_EDGE('',*,*,#30646,.T.);
#39516=ORIENTED_EDGE('',*,*,#30642,.F.);
#39517=ORIENTED_EDGE('',*,*,#30647,.F.);
#39518=ORIENTED_EDGE('',*,*,#30648,.T.);
#39519=ORIENTED_EDGE('',*,*,#30649,.T.);
#39520=ORIENTED_EDGE('',*,*,#30645,.F.);
#39521=ORIENTED_EDGE('',*,*,#30650,.F.);
#39522=ORIENTED_EDGE('',*,*,#30651,.T.);
#39523=ORIENTED_EDGE('',*,*,#30652,.T.);
#39524=ORIENTED_EDGE('',*,*,#30648,.F.);
#39525=ORIENTED_EDGE('',*,*,#30653,.F.);
#39526=ORIENTED_EDGE('',*,*,#30654,.T.);
#39527=ORIENTED_EDGE('',*,*,#30655,.T.);
#39528=ORIENTED_EDGE('',*,*,#30651,.F.);
#39529=ORIENTED_EDGE('',*,*,#30656,.F.);
#39530=ORIENTED_EDGE('',*,*,#30657,.T.);
#39531=ORIENTED_EDGE('',*,*,#30658,.T.);
#39532=ORIENTED_EDGE('',*,*,#30654,.F.);
#39533=ORIENTED_EDGE('',*,*,#30659,.F.);
#39534=ORIENTED_EDGE('',*,*,#30616,.T.);
#39535=ORIENTED_EDGE('',*,*,#30660,.T.);
#39536=ORIENTED_EDGE('',*,*,#30657,.F.);
#39537=ORIENTED_EDGE('',*,*,#30660,.F.);
#39538=ORIENTED_EDGE('',*,*,#30615,.F.);
#39539=ORIENTED_EDGE('',*,*,#30619,.F.);
#39540=ORIENTED_EDGE('',*,*,#30622,.F.);
#39541=ORIENTED_EDGE('',*,*,#30625,.F.);
#39542=ORIENTED_EDGE('',*,*,#30628,.F.);
#39543=ORIENTED_EDGE('',*,*,#30631,.F.);
#39544=ORIENTED_EDGE('',*,*,#30634,.F.);
#39545=ORIENTED_EDGE('',*,*,#30637,.F.);
#39546=ORIENTED_EDGE('',*,*,#30640,.F.);
#39547=ORIENTED_EDGE('',*,*,#30643,.F.);
#39548=ORIENTED_EDGE('',*,*,#30646,.F.);
#39549=ORIENTED_EDGE('',*,*,#30649,.F.);
#39550=ORIENTED_EDGE('',*,*,#30652,.F.);
#39551=ORIENTED_EDGE('',*,*,#30655,.F.);
#39552=ORIENTED_EDGE('',*,*,#30658,.F.);
#39553=ORIENTED_EDGE('',*,*,#30612,.F.);
#39554=ORIENTED_EDGE('',*,*,#30588,.F.);
#39555=ORIENTED_EDGE('',*,*,#30592,.F.);
#39556=ORIENTED_EDGE('',*,*,#30595,.F.);
#39557=ORIENTED_EDGE('',*,*,#30598,.F.);
#39558=ORIENTED_EDGE('',*,*,#30601,.F.);
#39559=ORIENTED_EDGE('',*,*,#30604,.F.);
#39560=ORIENTED_EDGE('',*,*,#30607,.F.);
#39561=ORIENTED_EDGE('',*,*,#30610,.F.);
#39562=ORIENTED_EDGE('',*,*,#30585,.F.);
#39563=ORIENTED_EDGE('',*,*,#30564,.F.);
#39564=ORIENTED_EDGE('',*,*,#30568,.F.);
#39565=ORIENTED_EDGE('',*,*,#30571,.F.);
#39566=ORIENTED_EDGE('',*,*,#30574,.F.);
#39567=ORIENTED_EDGE('',*,*,#30577,.F.);
#39568=ORIENTED_EDGE('',*,*,#30580,.F.);
#39569=ORIENTED_EDGE('',*,*,#30583,.F.);
#39570=ORIENTED_EDGE('',*,*,#30586,.T.);
#39571=ORIENTED_EDGE('',*,*,#30611,.T.);
#39572=ORIENTED_EDGE('',*,*,#30608,.T.);
#39573=ORIENTED_EDGE('',*,*,#30605,.T.);
#39574=ORIENTED_EDGE('',*,*,#30602,.T.);
#39575=ORIENTED_EDGE('',*,*,#30599,.T.);
#39576=ORIENTED_EDGE('',*,*,#30596,.T.);
#39577=ORIENTED_EDGE('',*,*,#30593,.T.);
#39578=ORIENTED_EDGE('',*,*,#30590,.T.);
#39579=ORIENTED_EDGE('',*,*,#30562,.T.);
#39580=ORIENTED_EDGE('',*,*,#30584,.T.);
#39581=ORIENTED_EDGE('',*,*,#30581,.T.);
#39582=ORIENTED_EDGE('',*,*,#30578,.T.);
#39583=ORIENTED_EDGE('',*,*,#30575,.T.);
#39584=ORIENTED_EDGE('',*,*,#30572,.T.);
#39585=ORIENTED_EDGE('',*,*,#30569,.T.);
#39586=ORIENTED_EDGE('',*,*,#30566,.T.);
#39587=ORIENTED_EDGE('',*,*,#30502,.T.);
#39588=ORIENTED_EDGE('',*,*,#30524,.T.);
#39589=ORIENTED_EDGE('',*,*,#30521,.T.);
#39590=ORIENTED_EDGE('',*,*,#30518,.T.);
#39591=ORIENTED_EDGE('',*,*,#30515,.T.);
#39592=ORIENTED_EDGE('',*,*,#30512,.T.);
#39593=ORIENTED_EDGE('',*,*,#30509,.T.);
#39594=ORIENTED_EDGE('',*,*,#30506,.T.);
#39595=ORIENTED_EDGE('',*,*,#30661,.F.);
#39596=ORIENTED_EDGE('',*,*,#30662,.T.);
#39597=ORIENTED_EDGE('',*,*,#30663,.T.);
#39598=ORIENTED_EDGE('',*,*,#30664,.F.);
#39599=ORIENTED_EDGE('',*,*,#30665,.F.);
#39600=ORIENTED_EDGE('',*,*,#30666,.T.);
#39601=ORIENTED_EDGE('',*,*,#30667,.T.);
#39602=ORIENTED_EDGE('',*,*,#30662,.F.);
#39603=ORIENTED_EDGE('',*,*,#30668,.F.);
#39604=ORIENTED_EDGE('',*,*,#30669,.T.);
#39605=ORIENTED_EDGE('',*,*,#30670,.T.);
#39606=ORIENTED_EDGE('',*,*,#30666,.F.);
#39607=ORIENTED_EDGE('',*,*,#30671,.F.);
#39608=ORIENTED_EDGE('',*,*,#30672,.T.);
#39609=ORIENTED_EDGE('',*,*,#30673,.T.);
#39610=ORIENTED_EDGE('',*,*,#30669,.F.);
#39611=ORIENTED_EDGE('',*,*,#30674,.F.);
#39612=ORIENTED_EDGE('',*,*,#30675,.T.);
#39613=ORIENTED_EDGE('',*,*,#30676,.T.);
#39614=ORIENTED_EDGE('',*,*,#30672,.F.);
#39615=ORIENTED_EDGE('',*,*,#30677,.F.);
#39616=ORIENTED_EDGE('',*,*,#30678,.T.);
#39617=ORIENTED_EDGE('',*,*,#30679,.T.);
#39618=ORIENTED_EDGE('',*,*,#30675,.F.);
#39619=ORIENTED_EDGE('',*,*,#30680,.F.);
#39620=ORIENTED_EDGE('',*,*,#30681,.T.);
#39621=ORIENTED_EDGE('',*,*,#30682,.T.);
#39622=ORIENTED_EDGE('',*,*,#30678,.F.);
#39623=ORIENTED_EDGE('',*,*,#30683,.F.);
#39624=ORIENTED_EDGE('',*,*,#30664,.T.);
#39625=ORIENTED_EDGE('',*,*,#30684,.T.);
#39626=ORIENTED_EDGE('',*,*,#30681,.F.);
#39627=ORIENTED_EDGE('',*,*,#30685,.F.);
#39628=ORIENTED_EDGE('',*,*,#30686,.T.);
#39629=ORIENTED_EDGE('',*,*,#30687,.T.);
#39630=ORIENTED_EDGE('',*,*,#30688,.F.);
#39631=ORIENTED_EDGE('',*,*,#30689,.F.);
#39632=ORIENTED_EDGE('',*,*,#30690,.T.);
#39633=ORIENTED_EDGE('',*,*,#30691,.T.);
#39634=ORIENTED_EDGE('',*,*,#30686,.F.);
#39635=ORIENTED_EDGE('',*,*,#30692,.F.);
#39636=ORIENTED_EDGE('',*,*,#30693,.T.);
#39637=ORIENTED_EDGE('',*,*,#30694,.T.);
#39638=ORIENTED_EDGE('',*,*,#30690,.F.);
#39639=ORIENTED_EDGE('',*,*,#30695,.F.);
#39640=ORIENTED_EDGE('',*,*,#30696,.T.);
#39641=ORIENTED_EDGE('',*,*,#30697,.T.);
#39642=ORIENTED_EDGE('',*,*,#30693,.F.);
#39643=ORIENTED_EDGE('',*,*,#30698,.F.);
#39644=ORIENTED_EDGE('',*,*,#30699,.T.);
#39645=ORIENTED_EDGE('',*,*,#30700,.T.);
#39646=ORIENTED_EDGE('',*,*,#30696,.F.);
#39647=ORIENTED_EDGE('',*,*,#30701,.F.);
#39648=ORIENTED_EDGE('',*,*,#30702,.T.);
#39649=ORIENTED_EDGE('',*,*,#30703,.T.);
#39650=ORIENTED_EDGE('',*,*,#30699,.F.);
#39651=ORIENTED_EDGE('',*,*,#30704,.F.);
#39652=ORIENTED_EDGE('',*,*,#30705,.T.);
#39653=ORIENTED_EDGE('',*,*,#30706,.T.);
#39654=ORIENTED_EDGE('',*,*,#30702,.F.);
#39655=ORIENTED_EDGE('',*,*,#30707,.F.);
#39656=ORIENTED_EDGE('',*,*,#30708,.T.);
#39657=ORIENTED_EDGE('',*,*,#30709,.T.);
#39658=ORIENTED_EDGE('',*,*,#30705,.F.);
#39659=ORIENTED_EDGE('',*,*,#30710,.F.);
#39660=ORIENTED_EDGE('',*,*,#30711,.T.);
#39661=ORIENTED_EDGE('',*,*,#30712,.T.);
#39662=ORIENTED_EDGE('',*,*,#30708,.F.);
#39663=ORIENTED_EDGE('',*,*,#30713,.F.);
#39664=ORIENTED_EDGE('',*,*,#30714,.T.);
#39665=ORIENTED_EDGE('',*,*,#30715,.T.);
#39666=ORIENTED_EDGE('',*,*,#30711,.F.);
#39667=ORIENTED_EDGE('',*,*,#30716,.F.);
#39668=ORIENTED_EDGE('',*,*,#30717,.T.);
#39669=ORIENTED_EDGE('',*,*,#30718,.T.);
#39670=ORIENTED_EDGE('',*,*,#30714,.F.);
#39671=ORIENTED_EDGE('',*,*,#30719,.F.);
#39672=ORIENTED_EDGE('',*,*,#30688,.T.);
#39673=ORIENTED_EDGE('',*,*,#30720,.T.);
#39674=ORIENTED_EDGE('',*,*,#30717,.F.);
#39675=ORIENTED_EDGE('',*,*,#30720,.F.);
#39676=ORIENTED_EDGE('',*,*,#30687,.F.);
#39677=ORIENTED_EDGE('',*,*,#30691,.F.);
#39678=ORIENTED_EDGE('',*,*,#30694,.F.);
#39679=ORIENTED_EDGE('',*,*,#30697,.F.);
#39680=ORIENTED_EDGE('',*,*,#30700,.F.);
#39681=ORIENTED_EDGE('',*,*,#30703,.F.);
#39682=ORIENTED_EDGE('',*,*,#30706,.F.);
#39683=ORIENTED_EDGE('',*,*,#30709,.F.);
#39684=ORIENTED_EDGE('',*,*,#30712,.F.);
#39685=ORIENTED_EDGE('',*,*,#30715,.F.);
#39686=ORIENTED_EDGE('',*,*,#30718,.F.);
#39687=ORIENTED_EDGE('',*,*,#30684,.F.);
#39688=ORIENTED_EDGE('',*,*,#30663,.F.);
#39689=ORIENTED_EDGE('',*,*,#30667,.F.);
#39690=ORIENTED_EDGE('',*,*,#30670,.F.);
#39691=ORIENTED_EDGE('',*,*,#30673,.F.);
#39692=ORIENTED_EDGE('',*,*,#30676,.F.);
#39693=ORIENTED_EDGE('',*,*,#30679,.F.);
#39694=ORIENTED_EDGE('',*,*,#30682,.F.);
#39695=ORIENTED_EDGE('',*,*,#30721,.F.);
#39696=ORIENTED_EDGE('',*,*,#30722,.T.);
#39697=ORIENTED_EDGE('',*,*,#30723,.T.);
#39698=ORIENTED_EDGE('',*,*,#30724,.F.);
#39699=ORIENTED_EDGE('',*,*,#30725,.F.);
#39700=ORIENTED_EDGE('',*,*,#30726,.T.);
#39701=ORIENTED_EDGE('',*,*,#30727,.T.);
#39702=ORIENTED_EDGE('',*,*,#30722,.F.);
#39703=ORIENTED_EDGE('',*,*,#30728,.F.);
#39704=ORIENTED_EDGE('',*,*,#30729,.T.);
#39705=ORIENTED_EDGE('',*,*,#30730,.T.);
#39706=ORIENTED_EDGE('',*,*,#30726,.F.);
#39707=ORIENTED_EDGE('',*,*,#30731,.F.);
#39708=ORIENTED_EDGE('',*,*,#30732,.T.);
#39709=ORIENTED_EDGE('',*,*,#30733,.T.);
#39710=ORIENTED_EDGE('',*,*,#30729,.F.);
#39711=ORIENTED_EDGE('',*,*,#30734,.F.);
#39712=ORIENTED_EDGE('',*,*,#30735,.T.);
#39713=ORIENTED_EDGE('',*,*,#30736,.T.);
#39714=ORIENTED_EDGE('',*,*,#30732,.F.);
#39715=ORIENTED_EDGE('',*,*,#30737,.F.);
#39716=ORIENTED_EDGE('',*,*,#30738,.T.);
#39717=ORIENTED_EDGE('',*,*,#30739,.T.);
#39718=ORIENTED_EDGE('',*,*,#30735,.F.);
#39719=ORIENTED_EDGE('',*,*,#30740,.F.);
#39720=ORIENTED_EDGE('',*,*,#30741,.T.);
#39721=ORIENTED_EDGE('',*,*,#30742,.T.);
#39722=ORIENTED_EDGE('',*,*,#30738,.F.);
#39723=ORIENTED_EDGE('',*,*,#30743,.F.);
#39724=ORIENTED_EDGE('',*,*,#30744,.T.);
#39725=ORIENTED_EDGE('',*,*,#30745,.T.);
#39726=ORIENTED_EDGE('',*,*,#30741,.F.);
#39727=ORIENTED_EDGE('',*,*,#30746,.F.);
#39728=ORIENTED_EDGE('',*,*,#30747,.T.);
#39729=ORIENTED_EDGE('',*,*,#30748,.T.);
#39730=ORIENTED_EDGE('',*,*,#30744,.F.);
#39731=ORIENTED_EDGE('',*,*,#30749,.F.);
#39732=ORIENTED_EDGE('',*,*,#30750,.T.);
#39733=ORIENTED_EDGE('',*,*,#30751,.T.);
#39734=ORIENTED_EDGE('',*,*,#30747,.F.);
#39735=ORIENTED_EDGE('',*,*,#30752,.F.);
#39736=ORIENTED_EDGE('',*,*,#30724,.T.);
#39737=ORIENTED_EDGE('',*,*,#30753,.T.);
#39738=ORIENTED_EDGE('',*,*,#30750,.F.);
#39739=ORIENTED_EDGE('',*,*,#30753,.F.);
#39740=ORIENTED_EDGE('',*,*,#30723,.F.);
#39741=ORIENTED_EDGE('',*,*,#30727,.F.);
#39742=ORIENTED_EDGE('',*,*,#30730,.F.);
#39743=ORIENTED_EDGE('',*,*,#30733,.F.);
#39744=ORIENTED_EDGE('',*,*,#30736,.F.);
#39745=ORIENTED_EDGE('',*,*,#30739,.F.);
#39746=ORIENTED_EDGE('',*,*,#30742,.F.);
#39747=ORIENTED_EDGE('',*,*,#30745,.F.);
#39748=ORIENTED_EDGE('',*,*,#30748,.F.);
#39749=ORIENTED_EDGE('',*,*,#30751,.F.);
#39750=ORIENTED_EDGE('',*,*,#30661,.T.);
#39751=ORIENTED_EDGE('',*,*,#30683,.T.);
#39752=ORIENTED_EDGE('',*,*,#30680,.T.);
#39753=ORIENTED_EDGE('',*,*,#30677,.T.);
#39754=ORIENTED_EDGE('',*,*,#30674,.T.);
#39755=ORIENTED_EDGE('',*,*,#30671,.T.);
#39756=ORIENTED_EDGE('',*,*,#30668,.T.);
#39757=ORIENTED_EDGE('',*,*,#30665,.T.);
#39758=ORIENTED_EDGE('',*,*,#30754,.F.);
#39759=ORIENTED_EDGE('',*,*,#30755,.T.);
#39760=ORIENTED_EDGE('',*,*,#30756,.T.);
#39761=ORIENTED_EDGE('',*,*,#30757,.F.);
#39762=ORIENTED_EDGE('',*,*,#30758,.F.);
#39763=ORIENTED_EDGE('',*,*,#30759,.T.);
#39764=ORIENTED_EDGE('',*,*,#30760,.T.);
#39765=ORIENTED_EDGE('',*,*,#30755,.F.);
#39766=ORIENTED_EDGE('',*,*,#30761,.F.);
#39767=ORIENTED_EDGE('',*,*,#30762,.T.);
#39768=ORIENTED_EDGE('',*,*,#30763,.T.);
#39769=ORIENTED_EDGE('',*,*,#30759,.F.);
#39770=ORIENTED_EDGE('',*,*,#30764,.F.);
#39771=ORIENTED_EDGE('',*,*,#30765,.T.);
#39772=ORIENTED_EDGE('',*,*,#30766,.T.);
#39773=ORIENTED_EDGE('',*,*,#30762,.F.);
#39774=ORIENTED_EDGE('',*,*,#30767,.F.);
#39775=ORIENTED_EDGE('',*,*,#30768,.T.);
#39776=ORIENTED_EDGE('',*,*,#30769,.T.);
#39777=ORIENTED_EDGE('',*,*,#30765,.F.);
#39778=ORIENTED_EDGE('',*,*,#30770,.F.);
#39779=ORIENTED_EDGE('',*,*,#30771,.T.);
#39780=ORIENTED_EDGE('',*,*,#30772,.T.);
#39781=ORIENTED_EDGE('',*,*,#30768,.F.);
#39782=ORIENTED_EDGE('',*,*,#30773,.F.);
#39783=ORIENTED_EDGE('',*,*,#30774,.T.);
#39784=ORIENTED_EDGE('',*,*,#30775,.T.);
#39785=ORIENTED_EDGE('',*,*,#30771,.F.);
#39786=ORIENTED_EDGE('',*,*,#30776,.F.);
#39787=ORIENTED_EDGE('',*,*,#30757,.T.);
#39788=ORIENTED_EDGE('',*,*,#30777,.T.);
#39789=ORIENTED_EDGE('',*,*,#30774,.F.);
#39790=ORIENTED_EDGE('',*,*,#30778,.F.);
#39791=ORIENTED_EDGE('',*,*,#30779,.T.);
#39792=ORIENTED_EDGE('',*,*,#30780,.T.);
#39793=ORIENTED_EDGE('',*,*,#30781,.F.);
#39794=ORIENTED_EDGE('',*,*,#30782,.F.);
#39795=ORIENTED_EDGE('',*,*,#30783,.T.);
#39796=ORIENTED_EDGE('',*,*,#30784,.T.);
#39797=ORIENTED_EDGE('',*,*,#30779,.F.);
#39798=ORIENTED_EDGE('',*,*,#30785,.F.);
#39799=ORIENTED_EDGE('',*,*,#30786,.T.);
#39800=ORIENTED_EDGE('',*,*,#30787,.T.);
#39801=ORIENTED_EDGE('',*,*,#30783,.F.);
#39802=ORIENTED_EDGE('',*,*,#30788,.F.);
#39803=ORIENTED_EDGE('',*,*,#30789,.T.);
#39804=ORIENTED_EDGE('',*,*,#30790,.T.);
#39805=ORIENTED_EDGE('',*,*,#30786,.F.);
#39806=ORIENTED_EDGE('',*,*,#30791,.F.);
#39807=ORIENTED_EDGE('',*,*,#30792,.T.);
#39808=ORIENTED_EDGE('',*,*,#30793,.T.);
#39809=ORIENTED_EDGE('',*,*,#30789,.F.);
#39810=ORIENTED_EDGE('',*,*,#30794,.F.);
#39811=ORIENTED_EDGE('',*,*,#30795,.T.);
#39812=ORIENTED_EDGE('',*,*,#30796,.T.);
#39813=ORIENTED_EDGE('',*,*,#30792,.F.);
#39814=ORIENTED_EDGE('',*,*,#30797,.F.);
#39815=ORIENTED_EDGE('',*,*,#30798,.T.);
#39816=ORIENTED_EDGE('',*,*,#30799,.T.);
#39817=ORIENTED_EDGE('',*,*,#30795,.F.);
#39818=ORIENTED_EDGE('',*,*,#30800,.F.);
#39819=ORIENTED_EDGE('',*,*,#30801,.T.);
#39820=ORIENTED_EDGE('',*,*,#30802,.T.);
#39821=ORIENTED_EDGE('',*,*,#30798,.F.);
#39822=ORIENTED_EDGE('',*,*,#30803,.F.);
#39823=ORIENTED_EDGE('',*,*,#30804,.T.);
#39824=ORIENTED_EDGE('',*,*,#30805,.T.);
#39825=ORIENTED_EDGE('',*,*,#30801,.F.);
#39826=ORIENTED_EDGE('',*,*,#30806,.F.);
#39827=ORIENTED_EDGE('',*,*,#30807,.T.);
#39828=ORIENTED_EDGE('',*,*,#30808,.T.);
#39829=ORIENTED_EDGE('',*,*,#30804,.F.);
#39830=ORIENTED_EDGE('',*,*,#30809,.F.);
#39831=ORIENTED_EDGE('',*,*,#30810,.T.);
#39832=ORIENTED_EDGE('',*,*,#30811,.T.);
#39833=ORIENTED_EDGE('',*,*,#30807,.F.);
#39834=ORIENTED_EDGE('',*,*,#30812,.F.);
#39835=ORIENTED_EDGE('',*,*,#30781,.T.);
#39836=ORIENTED_EDGE('',*,*,#30813,.T.);
#39837=ORIENTED_EDGE('',*,*,#30810,.F.);
#39838=ORIENTED_EDGE('',*,*,#30813,.F.);
#39839=ORIENTED_EDGE('',*,*,#30780,.F.);
#39840=ORIENTED_EDGE('',*,*,#30784,.F.);
#39841=ORIENTED_EDGE('',*,*,#30787,.F.);
#39842=ORIENTED_EDGE('',*,*,#30790,.F.);
#39843=ORIENTED_EDGE('',*,*,#30793,.F.);
#39844=ORIENTED_EDGE('',*,*,#30796,.F.);
#39845=ORIENTED_EDGE('',*,*,#30799,.F.);
#39846=ORIENTED_EDGE('',*,*,#30802,.F.);
#39847=ORIENTED_EDGE('',*,*,#30805,.F.);
#39848=ORIENTED_EDGE('',*,*,#30808,.F.);
#39849=ORIENTED_EDGE('',*,*,#30811,.F.);
#39850=ORIENTED_EDGE('',*,*,#30777,.F.);
#39851=ORIENTED_EDGE('',*,*,#30756,.F.);
#39852=ORIENTED_EDGE('',*,*,#30760,.F.);
#39853=ORIENTED_EDGE('',*,*,#30763,.F.);
#39854=ORIENTED_EDGE('',*,*,#30766,.F.);
#39855=ORIENTED_EDGE('',*,*,#30769,.F.);
#39856=ORIENTED_EDGE('',*,*,#30772,.F.);
#39857=ORIENTED_EDGE('',*,*,#30775,.F.);
#39858=ORIENTED_EDGE('',*,*,#30814,.F.);
#39859=ORIENTED_EDGE('',*,*,#30815,.T.);
#39860=ORIENTED_EDGE('',*,*,#30816,.T.);
#39861=ORIENTED_EDGE('',*,*,#30817,.F.);
#39862=ORIENTED_EDGE('',*,*,#30818,.F.);
#39863=ORIENTED_EDGE('',*,*,#30819,.T.);
#39864=ORIENTED_EDGE('',*,*,#30820,.T.);
#39865=ORIENTED_EDGE('',*,*,#30815,.F.);
#39866=ORIENTED_EDGE('',*,*,#30821,.F.);
#39867=ORIENTED_EDGE('',*,*,#30822,.T.);
#39868=ORIENTED_EDGE('',*,*,#30823,.T.);
#39869=ORIENTED_EDGE('',*,*,#30819,.F.);
#39870=ORIENTED_EDGE('',*,*,#30824,.F.);
#39871=ORIENTED_EDGE('',*,*,#30825,.T.);
#39872=ORIENTED_EDGE('',*,*,#30826,.T.);
#39873=ORIENTED_EDGE('',*,*,#30822,.F.);
#39874=ORIENTED_EDGE('',*,*,#30827,.F.);
#39875=ORIENTED_EDGE('',*,*,#30828,.T.);
#39876=ORIENTED_EDGE('',*,*,#30829,.T.);
#39877=ORIENTED_EDGE('',*,*,#30825,.F.);
#39878=ORIENTED_EDGE('',*,*,#30830,.F.);
#39879=ORIENTED_EDGE('',*,*,#30831,.T.);
#39880=ORIENTED_EDGE('',*,*,#30832,.T.);
#39881=ORIENTED_EDGE('',*,*,#30828,.F.);
#39882=ORIENTED_EDGE('',*,*,#30833,.F.);
#39883=ORIENTED_EDGE('',*,*,#30834,.T.);
#39884=ORIENTED_EDGE('',*,*,#30835,.T.);
#39885=ORIENTED_EDGE('',*,*,#30831,.F.);
#39886=ORIENTED_EDGE('',*,*,#30836,.F.);
#39887=ORIENTED_EDGE('',*,*,#30837,.T.);
#39888=ORIENTED_EDGE('',*,*,#30838,.T.);
#39889=ORIENTED_EDGE('',*,*,#30834,.F.);
#39890=ORIENTED_EDGE('',*,*,#30839,.F.);
#39891=ORIENTED_EDGE('',*,*,#30817,.T.);
#39892=ORIENTED_EDGE('',*,*,#30840,.T.);
#39893=ORIENTED_EDGE('',*,*,#30837,.F.);
#39894=ORIENTED_EDGE('',*,*,#30841,.F.);
#39895=ORIENTED_EDGE('',*,*,#30842,.T.);
#39896=ORIENTED_EDGE('',*,*,#30843,.T.);
#39897=ORIENTED_EDGE('',*,*,#30844,.F.);
#39898=ORIENTED_EDGE('',*,*,#30845,.F.);
#39899=ORIENTED_EDGE('',*,*,#30846,.T.);
#39900=ORIENTED_EDGE('',*,*,#30847,.T.);
#39901=ORIENTED_EDGE('',*,*,#30842,.F.);
#39902=ORIENTED_EDGE('',*,*,#30848,.F.);
#39903=ORIENTED_EDGE('',*,*,#30849,.T.);
#39904=ORIENTED_EDGE('',*,*,#30850,.T.);
#39905=ORIENTED_EDGE('',*,*,#30846,.F.);
#39906=ORIENTED_EDGE('',*,*,#30851,.F.);
#39907=ORIENTED_EDGE('',*,*,#30852,.T.);
#39908=ORIENTED_EDGE('',*,*,#30853,.T.);
#39909=ORIENTED_EDGE('',*,*,#30849,.F.);
#39910=ORIENTED_EDGE('',*,*,#30854,.F.);
#39911=ORIENTED_EDGE('',*,*,#30855,.T.);
#39912=ORIENTED_EDGE('',*,*,#30856,.T.);
#39913=ORIENTED_EDGE('',*,*,#30852,.F.);
#39914=ORIENTED_EDGE('',*,*,#30857,.F.);
#39915=ORIENTED_EDGE('',*,*,#30858,.T.);
#39916=ORIENTED_EDGE('',*,*,#30859,.T.);
#39917=ORIENTED_EDGE('',*,*,#30855,.F.);
#39918=ORIENTED_EDGE('',*,*,#30860,.F.);
#39919=ORIENTED_EDGE('',*,*,#30861,.T.);
#39920=ORIENTED_EDGE('',*,*,#30862,.T.);
#39921=ORIENTED_EDGE('',*,*,#30858,.F.);
#39922=ORIENTED_EDGE('',*,*,#30863,.F.);
#39923=ORIENTED_EDGE('',*,*,#30864,.T.);
#39924=ORIENTED_EDGE('',*,*,#30865,.T.);
#39925=ORIENTED_EDGE('',*,*,#30861,.F.);
#39926=ORIENTED_EDGE('',*,*,#30866,.F.);
#39927=ORIENTED_EDGE('',*,*,#30867,.T.);
#39928=ORIENTED_EDGE('',*,*,#30868,.T.);
#39929=ORIENTED_EDGE('',*,*,#30864,.F.);
#39930=ORIENTED_EDGE('',*,*,#30869,.F.);
#39931=ORIENTED_EDGE('',*,*,#30870,.T.);
#39932=ORIENTED_EDGE('',*,*,#30871,.T.);
#39933=ORIENTED_EDGE('',*,*,#30867,.F.);
#39934=ORIENTED_EDGE('',*,*,#30872,.F.);
#39935=ORIENTED_EDGE('',*,*,#30873,.T.);
#39936=ORIENTED_EDGE('',*,*,#30874,.T.);
#39937=ORIENTED_EDGE('',*,*,#30870,.F.);
#39938=ORIENTED_EDGE('',*,*,#30875,.F.);
#39939=ORIENTED_EDGE('',*,*,#30876,.T.);
#39940=ORIENTED_EDGE('',*,*,#30877,.T.);
#39941=ORIENTED_EDGE('',*,*,#30873,.F.);
#39942=ORIENTED_EDGE('',*,*,#30878,.F.);
#39943=ORIENTED_EDGE('',*,*,#30879,.T.);
#39944=ORIENTED_EDGE('',*,*,#30880,.T.);
#39945=ORIENTED_EDGE('',*,*,#30876,.F.);
#39946=ORIENTED_EDGE('',*,*,#30881,.F.);
#39947=ORIENTED_EDGE('',*,*,#30882,.T.);
#39948=ORIENTED_EDGE('',*,*,#30883,.T.);
#39949=ORIENTED_EDGE('',*,*,#30879,.F.);
#39950=ORIENTED_EDGE('',*,*,#30884,.F.);
#39951=ORIENTED_EDGE('',*,*,#30885,.T.);
#39952=ORIENTED_EDGE('',*,*,#30886,.T.);
#39953=ORIENTED_EDGE('',*,*,#30882,.F.);
#39954=ORIENTED_EDGE('',*,*,#30887,.F.);
#39955=ORIENTED_EDGE('',*,*,#30888,.T.);
#39956=ORIENTED_EDGE('',*,*,#30889,.T.);
#39957=ORIENTED_EDGE('',*,*,#30885,.F.);
#39958=ORIENTED_EDGE('',*,*,#30890,.F.);
#39959=ORIENTED_EDGE('',*,*,#30891,.T.);
#39960=ORIENTED_EDGE('',*,*,#30892,.T.);
#39961=ORIENTED_EDGE('',*,*,#30888,.F.);
#39962=ORIENTED_EDGE('',*,*,#30893,.F.);
#39963=ORIENTED_EDGE('',*,*,#30894,.T.);
#39964=ORIENTED_EDGE('',*,*,#30895,.T.);
#39965=ORIENTED_EDGE('',*,*,#30891,.F.);
#39966=ORIENTED_EDGE('',*,*,#30896,.F.);
#39967=ORIENTED_EDGE('',*,*,#30844,.T.);
#39968=ORIENTED_EDGE('',*,*,#30897,.T.);
#39969=ORIENTED_EDGE('',*,*,#30894,.F.);
#39970=ORIENTED_EDGE('',*,*,#30897,.F.);
#39971=ORIENTED_EDGE('',*,*,#30843,.F.);
#39972=ORIENTED_EDGE('',*,*,#30847,.F.);
#39973=ORIENTED_EDGE('',*,*,#30850,.F.);
#39974=ORIENTED_EDGE('',*,*,#30853,.F.);
#39975=ORIENTED_EDGE('',*,*,#30856,.F.);
#39976=ORIENTED_EDGE('',*,*,#30859,.F.);
#39977=ORIENTED_EDGE('',*,*,#30862,.F.);
#39978=ORIENTED_EDGE('',*,*,#30865,.F.);
#39979=ORIENTED_EDGE('',*,*,#30868,.F.);
#39980=ORIENTED_EDGE('',*,*,#30871,.F.);
#39981=ORIENTED_EDGE('',*,*,#30874,.F.);
#39982=ORIENTED_EDGE('',*,*,#30877,.F.);
#39983=ORIENTED_EDGE('',*,*,#30880,.F.);
#39984=ORIENTED_EDGE('',*,*,#30883,.F.);
#39985=ORIENTED_EDGE('',*,*,#30886,.F.);
#39986=ORIENTED_EDGE('',*,*,#30889,.F.);
#39987=ORIENTED_EDGE('',*,*,#30892,.F.);
#39988=ORIENTED_EDGE('',*,*,#30895,.F.);
#39989=ORIENTED_EDGE('',*,*,#30840,.F.);
#39990=ORIENTED_EDGE('',*,*,#30816,.F.);
#39991=ORIENTED_EDGE('',*,*,#30820,.F.);
#39992=ORIENTED_EDGE('',*,*,#30823,.F.);
#39993=ORIENTED_EDGE('',*,*,#30826,.F.);
#39994=ORIENTED_EDGE('',*,*,#30829,.F.);
#39995=ORIENTED_EDGE('',*,*,#30832,.F.);
#39996=ORIENTED_EDGE('',*,*,#30835,.F.);
#39997=ORIENTED_EDGE('',*,*,#30838,.F.);
#39998=ORIENTED_EDGE('',*,*,#30814,.T.);
#39999=ORIENTED_EDGE('',*,*,#30839,.T.);
#40000=ORIENTED_EDGE('',*,*,#30836,.T.);
#40001=ORIENTED_EDGE('',*,*,#30833,.T.);
#40002=ORIENTED_EDGE('',*,*,#30830,.T.);
#40003=ORIENTED_EDGE('',*,*,#30827,.T.);
#40004=ORIENTED_EDGE('',*,*,#30824,.T.);
#40005=ORIENTED_EDGE('',*,*,#30821,.T.);
#40006=ORIENTED_EDGE('',*,*,#30818,.T.);
#40007=ORIENTED_EDGE('',*,*,#30754,.T.);
#40008=ORIENTED_EDGE('',*,*,#30776,.T.);
#40009=ORIENTED_EDGE('',*,*,#30773,.T.);
#40010=ORIENTED_EDGE('',*,*,#30770,.T.);
#40011=ORIENTED_EDGE('',*,*,#30767,.T.);
#40012=ORIENTED_EDGE('',*,*,#30764,.T.);
#40013=ORIENTED_EDGE('',*,*,#30761,.T.);
#40014=ORIENTED_EDGE('',*,*,#30758,.T.);
#40015=ORIENTED_EDGE('',*,*,#30898,.F.);
#40016=ORIENTED_EDGE('',*,*,#30899,.T.);
#40017=ORIENTED_EDGE('',*,*,#30900,.T.);
#40018=ORIENTED_EDGE('',*,*,#30901,.F.);
#40019=ORIENTED_EDGE('',*,*,#30902,.F.);
#40020=ORIENTED_EDGE('',*,*,#30903,.T.);
#40021=ORIENTED_EDGE('',*,*,#30904,.T.);
#40022=ORIENTED_EDGE('',*,*,#30899,.F.);
#40023=ORIENTED_EDGE('',*,*,#30905,.F.);
#40024=ORIENTED_EDGE('',*,*,#30906,.T.);
#40025=ORIENTED_EDGE('',*,*,#30907,.T.);
#40026=ORIENTED_EDGE('',*,*,#30903,.F.);
#40027=ORIENTED_EDGE('',*,*,#30908,.F.);
#40028=ORIENTED_EDGE('',*,*,#30909,.T.);
#40029=ORIENTED_EDGE('',*,*,#30910,.T.);
#40030=ORIENTED_EDGE('',*,*,#30906,.F.);
#40031=ORIENTED_EDGE('',*,*,#30911,.F.);
#40032=ORIENTED_EDGE('',*,*,#30912,.T.);
#40033=ORIENTED_EDGE('',*,*,#30913,.T.);
#40034=ORIENTED_EDGE('',*,*,#30909,.F.);
#40035=ORIENTED_EDGE('',*,*,#30914,.F.);
#40036=ORIENTED_EDGE('',*,*,#30915,.T.);
#40037=ORIENTED_EDGE('',*,*,#30916,.T.);
#40038=ORIENTED_EDGE('',*,*,#30912,.F.);
#40039=ORIENTED_EDGE('',*,*,#30917,.F.);
#40040=ORIENTED_EDGE('',*,*,#30918,.T.);
#40041=ORIENTED_EDGE('',*,*,#30919,.T.);
#40042=ORIENTED_EDGE('',*,*,#30915,.F.);
#40043=ORIENTED_EDGE('',*,*,#30920,.F.);
#40044=ORIENTED_EDGE('',*,*,#30901,.T.);
#40045=ORIENTED_EDGE('',*,*,#30921,.T.);
#40046=ORIENTED_EDGE('',*,*,#30918,.F.);
#40047=ORIENTED_EDGE('',*,*,#30922,.F.);
#40048=ORIENTED_EDGE('',*,*,#30923,.T.);
#40049=ORIENTED_EDGE('',*,*,#30924,.T.);
#40050=ORIENTED_EDGE('',*,*,#30925,.F.);
#40051=ORIENTED_EDGE('',*,*,#30926,.F.);
#40052=ORIENTED_EDGE('',*,*,#30927,.T.);
#40053=ORIENTED_EDGE('',*,*,#30928,.T.);
#40054=ORIENTED_EDGE('',*,*,#30923,.F.);
#40055=ORIENTED_EDGE('',*,*,#30929,.F.);
#40056=ORIENTED_EDGE('',*,*,#30930,.T.);
#40057=ORIENTED_EDGE('',*,*,#30931,.T.);
#40058=ORIENTED_EDGE('',*,*,#30927,.F.);
#40059=ORIENTED_EDGE('',*,*,#30932,.F.);
#40060=ORIENTED_EDGE('',*,*,#30933,.T.);
#40061=ORIENTED_EDGE('',*,*,#30934,.T.);
#40062=ORIENTED_EDGE('',*,*,#30930,.F.);
#40063=ORIENTED_EDGE('',*,*,#30935,.F.);
#40064=ORIENTED_EDGE('',*,*,#30936,.T.);
#40065=ORIENTED_EDGE('',*,*,#30937,.T.);
#40066=ORIENTED_EDGE('',*,*,#30933,.F.);
#40067=ORIENTED_EDGE('',*,*,#30938,.F.);
#40068=ORIENTED_EDGE('',*,*,#30939,.T.);
#40069=ORIENTED_EDGE('',*,*,#30940,.T.);
#40070=ORIENTED_EDGE('',*,*,#30936,.F.);
#40071=ORIENTED_EDGE('',*,*,#30941,.F.);
#40072=ORIENTED_EDGE('',*,*,#30942,.T.);
#40073=ORIENTED_EDGE('',*,*,#30943,.T.);
#40074=ORIENTED_EDGE('',*,*,#30939,.F.);
#40075=ORIENTED_EDGE('',*,*,#30944,.F.);
#40076=ORIENTED_EDGE('',*,*,#30945,.T.);
#40077=ORIENTED_EDGE('',*,*,#30946,.T.);
#40078=ORIENTED_EDGE('',*,*,#30942,.F.);
#40079=ORIENTED_EDGE('',*,*,#30947,.F.);
#40080=ORIENTED_EDGE('',*,*,#30948,.T.);
#40081=ORIENTED_EDGE('',*,*,#30949,.T.);
#40082=ORIENTED_EDGE('',*,*,#30945,.F.);
#40083=ORIENTED_EDGE('',*,*,#30950,.F.);
#40084=ORIENTED_EDGE('',*,*,#30951,.T.);
#40085=ORIENTED_EDGE('',*,*,#30952,.T.);
#40086=ORIENTED_EDGE('',*,*,#30948,.F.);
#40087=ORIENTED_EDGE('',*,*,#30953,.F.);
#40088=ORIENTED_EDGE('',*,*,#30954,.T.);
#40089=ORIENTED_EDGE('',*,*,#30955,.T.);
#40090=ORIENTED_EDGE('',*,*,#30951,.F.);
#40091=ORIENTED_EDGE('',*,*,#30956,.F.);
#40092=ORIENTED_EDGE('',*,*,#30925,.T.);
#40093=ORIENTED_EDGE('',*,*,#30957,.T.);
#40094=ORIENTED_EDGE('',*,*,#30954,.F.);
#40095=ORIENTED_EDGE('',*,*,#30957,.F.);
#40096=ORIENTED_EDGE('',*,*,#30924,.F.);
#40097=ORIENTED_EDGE('',*,*,#30928,.F.);
#40098=ORIENTED_EDGE('',*,*,#30931,.F.);
#40099=ORIENTED_EDGE('',*,*,#30934,.F.);
#40100=ORIENTED_EDGE('',*,*,#30937,.F.);
#40101=ORIENTED_EDGE('',*,*,#30940,.F.);
#40102=ORIENTED_EDGE('',*,*,#30943,.F.);
#40103=ORIENTED_EDGE('',*,*,#30946,.F.);
#40104=ORIENTED_EDGE('',*,*,#30949,.F.);
#40105=ORIENTED_EDGE('',*,*,#30952,.F.);
#40106=ORIENTED_EDGE('',*,*,#30955,.F.);
#40107=ORIENTED_EDGE('',*,*,#30921,.F.);
#40108=ORIENTED_EDGE('',*,*,#30900,.F.);
#40109=ORIENTED_EDGE('',*,*,#30904,.F.);
#40110=ORIENTED_EDGE('',*,*,#30907,.F.);
#40111=ORIENTED_EDGE('',*,*,#30910,.F.);
#40112=ORIENTED_EDGE('',*,*,#30913,.F.);
#40113=ORIENTED_EDGE('',*,*,#30916,.F.);
#40114=ORIENTED_EDGE('',*,*,#30919,.F.);
#40115=ORIENTED_EDGE('',*,*,#30958,.F.);
#40116=ORIENTED_EDGE('',*,*,#30959,.T.);
#40117=ORIENTED_EDGE('',*,*,#30960,.T.);
#40118=ORIENTED_EDGE('',*,*,#30961,.F.);
#40119=ORIENTED_EDGE('',*,*,#30962,.F.);
#40120=ORIENTED_EDGE('',*,*,#30963,.T.);
#40121=ORIENTED_EDGE('',*,*,#30964,.T.);
#40122=ORIENTED_EDGE('',*,*,#30959,.F.);
#40123=ORIENTED_EDGE('',*,*,#30965,.F.);
#40124=ORIENTED_EDGE('',*,*,#30966,.T.);
#40125=ORIENTED_EDGE('',*,*,#30967,.T.);
#40126=ORIENTED_EDGE('',*,*,#30963,.F.);
#40127=ORIENTED_EDGE('',*,*,#30968,.F.);
#40128=ORIENTED_EDGE('',*,*,#30969,.T.);
#40129=ORIENTED_EDGE('',*,*,#30970,.T.);
#40130=ORIENTED_EDGE('',*,*,#30966,.F.);
#40131=ORIENTED_EDGE('',*,*,#30971,.F.);
#40132=ORIENTED_EDGE('',*,*,#30972,.T.);
#40133=ORIENTED_EDGE('',*,*,#30973,.T.);
#40134=ORIENTED_EDGE('',*,*,#30969,.F.);
#40135=ORIENTED_EDGE('',*,*,#30974,.F.);
#40136=ORIENTED_EDGE('',*,*,#30975,.T.);
#40137=ORIENTED_EDGE('',*,*,#30976,.T.);
#40138=ORIENTED_EDGE('',*,*,#30972,.F.);
#40139=ORIENTED_EDGE('',*,*,#30977,.F.);
#40140=ORIENTED_EDGE('',*,*,#30978,.T.);
#40141=ORIENTED_EDGE('',*,*,#30979,.T.);
#40142=ORIENTED_EDGE('',*,*,#30975,.F.);
#40143=ORIENTED_EDGE('',*,*,#30980,.F.);
#40144=ORIENTED_EDGE('',*,*,#30981,.T.);
#40145=ORIENTED_EDGE('',*,*,#30982,.T.);
#40146=ORIENTED_EDGE('',*,*,#30978,.F.);
#40147=ORIENTED_EDGE('',*,*,#30983,.F.);
#40148=ORIENTED_EDGE('',*,*,#30984,.T.);
#40149=ORIENTED_EDGE('',*,*,#30985,.T.);
#40150=ORIENTED_EDGE('',*,*,#30981,.F.);
#40151=ORIENTED_EDGE('',*,*,#30986,.F.);
#40152=ORIENTED_EDGE('',*,*,#30987,.T.);
#40153=ORIENTED_EDGE('',*,*,#30988,.T.);
#40154=ORIENTED_EDGE('',*,*,#30984,.F.);
#40155=ORIENTED_EDGE('',*,*,#30989,.F.);
#40156=ORIENTED_EDGE('',*,*,#30990,.T.);
#40157=ORIENTED_EDGE('',*,*,#30991,.T.);
#40158=ORIENTED_EDGE('',*,*,#30987,.F.);
#40159=ORIENTED_EDGE('',*,*,#30992,.F.);
#40160=ORIENTED_EDGE('',*,*,#30993,.T.);
#40161=ORIENTED_EDGE('',*,*,#30994,.T.);
#40162=ORIENTED_EDGE('',*,*,#30990,.F.);
#40163=ORIENTED_EDGE('',*,*,#30995,.F.);
#40164=ORIENTED_EDGE('',*,*,#30996,.T.);
#40165=ORIENTED_EDGE('',*,*,#30997,.T.);
#40166=ORIENTED_EDGE('',*,*,#30993,.F.);
#40167=ORIENTED_EDGE('',*,*,#30998,.F.);
#40168=ORIENTED_EDGE('',*,*,#30999,.T.);
#40169=ORIENTED_EDGE('',*,*,#31000,.T.);
#40170=ORIENTED_EDGE('',*,*,#30996,.F.);
#40171=ORIENTED_EDGE('',*,*,#31001,.F.);
#40172=ORIENTED_EDGE('',*,*,#31002,.T.);
#40173=ORIENTED_EDGE('',*,*,#31003,.T.);
#40174=ORIENTED_EDGE('',*,*,#30999,.F.);
#40175=ORIENTED_EDGE('',*,*,#31004,.F.);
#40176=ORIENTED_EDGE('',*,*,#31005,.T.);
#40177=ORIENTED_EDGE('',*,*,#31006,.T.);
#40178=ORIENTED_EDGE('',*,*,#31002,.F.);
#40179=ORIENTED_EDGE('',*,*,#31007,.F.);
#40180=ORIENTED_EDGE('',*,*,#31008,.T.);
#40181=ORIENTED_EDGE('',*,*,#31009,.T.);
#40182=ORIENTED_EDGE('',*,*,#31005,.F.);
#40183=ORIENTED_EDGE('',*,*,#31010,.F.);
#40184=ORIENTED_EDGE('',*,*,#31011,.T.);
#40185=ORIENTED_EDGE('',*,*,#31012,.T.);
#40186=ORIENTED_EDGE('',*,*,#31008,.F.);
#40187=ORIENTED_EDGE('',*,*,#31013,.F.);
#40188=ORIENTED_EDGE('',*,*,#31014,.T.);
#40189=ORIENTED_EDGE('',*,*,#31015,.T.);
#40190=ORIENTED_EDGE('',*,*,#31011,.F.);
#40191=ORIENTED_EDGE('',*,*,#31016,.F.);
#40192=ORIENTED_EDGE('',*,*,#31017,.T.);
#40193=ORIENTED_EDGE('',*,*,#31018,.T.);
#40194=ORIENTED_EDGE('',*,*,#31014,.F.);
#40195=ORIENTED_EDGE('',*,*,#31019,.F.);
#40196=ORIENTED_EDGE('',*,*,#31020,.T.);
#40197=ORIENTED_EDGE('',*,*,#31021,.T.);
#40198=ORIENTED_EDGE('',*,*,#31017,.F.);
#40199=ORIENTED_EDGE('',*,*,#31022,.F.);
#40200=ORIENTED_EDGE('',*,*,#30961,.T.);
#40201=ORIENTED_EDGE('',*,*,#31023,.T.);
#40202=ORIENTED_EDGE('',*,*,#31020,.F.);
#40203=ORIENTED_EDGE('',*,*,#31023,.F.);
#40204=ORIENTED_EDGE('',*,*,#30960,.F.);
#40205=ORIENTED_EDGE('',*,*,#30964,.F.);
#40206=ORIENTED_EDGE('',*,*,#30967,.F.);
#40207=ORIENTED_EDGE('',*,*,#30970,.F.);
#40208=ORIENTED_EDGE('',*,*,#30973,.F.);
#40209=ORIENTED_EDGE('',*,*,#30976,.F.);
#40210=ORIENTED_EDGE('',*,*,#30979,.F.);
#40211=ORIENTED_EDGE('',*,*,#30982,.F.);
#40212=ORIENTED_EDGE('',*,*,#30985,.F.);
#40213=ORIENTED_EDGE('',*,*,#30988,.F.);
#40214=ORIENTED_EDGE('',*,*,#30991,.F.);
#40215=ORIENTED_EDGE('',*,*,#30994,.F.);
#40216=ORIENTED_EDGE('',*,*,#30997,.F.);
#40217=ORIENTED_EDGE('',*,*,#31000,.F.);
#40218=ORIENTED_EDGE('',*,*,#31003,.F.);
#40219=ORIENTED_EDGE('',*,*,#31006,.F.);
#40220=ORIENTED_EDGE('',*,*,#31009,.F.);
#40221=ORIENTED_EDGE('',*,*,#31012,.F.);
#40222=ORIENTED_EDGE('',*,*,#31015,.F.);
#40223=ORIENTED_EDGE('',*,*,#31018,.F.);
#40224=ORIENTED_EDGE('',*,*,#31021,.F.);
#40225=ORIENTED_EDGE('',*,*,#30898,.T.);
#40226=ORIENTED_EDGE('',*,*,#30920,.T.);
#40227=ORIENTED_EDGE('',*,*,#30917,.T.);
#40228=ORIENTED_EDGE('',*,*,#30914,.T.);
#40229=ORIENTED_EDGE('',*,*,#30911,.T.);
#40230=ORIENTED_EDGE('',*,*,#30908,.T.);
#40231=ORIENTED_EDGE('',*,*,#30905,.T.);
#40232=ORIENTED_EDGE('',*,*,#30902,.T.);
#40233=ORIENTED_EDGE('',*,*,#31024,.F.);
#40234=ORIENTED_EDGE('',*,*,#31025,.T.);
#40235=ORIENTED_EDGE('',*,*,#31026,.T.);
#40236=ORIENTED_EDGE('',*,*,#31027,.F.);
#40237=ORIENTED_EDGE('',*,*,#31028,.F.);
#40238=ORIENTED_EDGE('',*,*,#31029,.T.);
#40239=ORIENTED_EDGE('',*,*,#31030,.T.);
#40240=ORIENTED_EDGE('',*,*,#31025,.F.);
#40241=ORIENTED_EDGE('',*,*,#31031,.F.);
#40242=ORIENTED_EDGE('',*,*,#31032,.T.);
#40243=ORIENTED_EDGE('',*,*,#31033,.T.);
#40244=ORIENTED_EDGE('',*,*,#31029,.F.);
#40245=ORIENTED_EDGE('',*,*,#31034,.F.);
#40246=ORIENTED_EDGE('',*,*,#31035,.T.);
#40247=ORIENTED_EDGE('',*,*,#31036,.T.);
#40248=ORIENTED_EDGE('',*,*,#31032,.F.);
#40249=ORIENTED_EDGE('',*,*,#31037,.F.);
#40250=ORIENTED_EDGE('',*,*,#31038,.T.);
#40251=ORIENTED_EDGE('',*,*,#31039,.T.);
#40252=ORIENTED_EDGE('',*,*,#31035,.F.);
#40253=ORIENTED_EDGE('',*,*,#31040,.F.);
#40254=ORIENTED_EDGE('',*,*,#31041,.T.);
#40255=ORIENTED_EDGE('',*,*,#31042,.T.);
#40256=ORIENTED_EDGE('',*,*,#31038,.F.);
#40257=ORIENTED_EDGE('',*,*,#31043,.F.);
#40258=ORIENTED_EDGE('',*,*,#31044,.T.);
#40259=ORIENTED_EDGE('',*,*,#31045,.T.);
#40260=ORIENTED_EDGE('',*,*,#31041,.F.);
#40261=ORIENTED_EDGE('',*,*,#31046,.F.);
#40262=ORIENTED_EDGE('',*,*,#31027,.T.);
#40263=ORIENTED_EDGE('',*,*,#31047,.T.);
#40264=ORIENTED_EDGE('',*,*,#31044,.F.);
#40265=ORIENTED_EDGE('',*,*,#31048,.F.);
#40266=ORIENTED_EDGE('',*,*,#31049,.T.);
#40267=ORIENTED_EDGE('',*,*,#31050,.T.);
#40268=ORIENTED_EDGE('',*,*,#31051,.F.);
#40269=ORIENTED_EDGE('',*,*,#31052,.F.);
#40270=ORIENTED_EDGE('',*,*,#31053,.T.);
#40271=ORIENTED_EDGE('',*,*,#31054,.T.);
#40272=ORIENTED_EDGE('',*,*,#31049,.F.);
#40273=ORIENTED_EDGE('',*,*,#31055,.F.);
#40274=ORIENTED_EDGE('',*,*,#31056,.T.);
#40275=ORIENTED_EDGE('',*,*,#31057,.T.);
#40276=ORIENTED_EDGE('',*,*,#31053,.F.);
#40277=ORIENTED_EDGE('',*,*,#31058,.F.);
#40278=ORIENTED_EDGE('',*,*,#31059,.T.);
#40279=ORIENTED_EDGE('',*,*,#31060,.T.);
#40280=ORIENTED_EDGE('',*,*,#31056,.F.);
#40281=ORIENTED_EDGE('',*,*,#31061,.F.);
#40282=ORIENTED_EDGE('',*,*,#31062,.T.);
#40283=ORIENTED_EDGE('',*,*,#31063,.T.);
#40284=ORIENTED_EDGE('',*,*,#31059,.F.);
#40285=ORIENTED_EDGE('',*,*,#31064,.F.);
#40286=ORIENTED_EDGE('',*,*,#31065,.T.);
#40287=ORIENTED_EDGE('',*,*,#31066,.T.);
#40288=ORIENTED_EDGE('',*,*,#31062,.F.);
#40289=ORIENTED_EDGE('',*,*,#31067,.F.);
#40290=ORIENTED_EDGE('',*,*,#31068,.T.);
#40291=ORIENTED_EDGE('',*,*,#31069,.T.);
#40292=ORIENTED_EDGE('',*,*,#31065,.F.);
#40293=ORIENTED_EDGE('',*,*,#31070,.F.);
#40294=ORIENTED_EDGE('',*,*,#31071,.T.);
#40295=ORIENTED_EDGE('',*,*,#31072,.T.);
#40296=ORIENTED_EDGE('',*,*,#31068,.F.);
#40297=ORIENTED_EDGE('',*,*,#31073,.F.);
#40298=ORIENTED_EDGE('',*,*,#31074,.T.);
#40299=ORIENTED_EDGE('',*,*,#31075,.T.);
#40300=ORIENTED_EDGE('',*,*,#31071,.F.);
#40301=ORIENTED_EDGE('',*,*,#31076,.F.);
#40302=ORIENTED_EDGE('',*,*,#31077,.T.);
#40303=ORIENTED_EDGE('',*,*,#31078,.T.);
#40304=ORIENTED_EDGE('',*,*,#31074,.F.);
#40305=ORIENTED_EDGE('',*,*,#31079,.F.);
#40306=ORIENTED_EDGE('',*,*,#31080,.T.);
#40307=ORIENTED_EDGE('',*,*,#31081,.T.);
#40308=ORIENTED_EDGE('',*,*,#31077,.F.);
#40309=ORIENTED_EDGE('',*,*,#31082,.F.);
#40310=ORIENTED_EDGE('',*,*,#31051,.T.);
#40311=ORIENTED_EDGE('',*,*,#31083,.T.);
#40312=ORIENTED_EDGE('',*,*,#31080,.F.);
#40313=ORIENTED_EDGE('',*,*,#31083,.F.);
#40314=ORIENTED_EDGE('',*,*,#31050,.F.);
#40315=ORIENTED_EDGE('',*,*,#31054,.F.);
#40316=ORIENTED_EDGE('',*,*,#31057,.F.);
#40317=ORIENTED_EDGE('',*,*,#31060,.F.);
#40318=ORIENTED_EDGE('',*,*,#31063,.F.);
#40319=ORIENTED_EDGE('',*,*,#31066,.F.);
#40320=ORIENTED_EDGE('',*,*,#31069,.F.);
#40321=ORIENTED_EDGE('',*,*,#31072,.F.);
#40322=ORIENTED_EDGE('',*,*,#31075,.F.);
#40323=ORIENTED_EDGE('',*,*,#31078,.F.);
#40324=ORIENTED_EDGE('',*,*,#31081,.F.);
#40325=ORIENTED_EDGE('',*,*,#31047,.F.);
#40326=ORIENTED_EDGE('',*,*,#31026,.F.);
#40327=ORIENTED_EDGE('',*,*,#31030,.F.);
#40328=ORIENTED_EDGE('',*,*,#31033,.F.);
#40329=ORIENTED_EDGE('',*,*,#31036,.F.);
#40330=ORIENTED_EDGE('',*,*,#31039,.F.);
#40331=ORIENTED_EDGE('',*,*,#31042,.F.);
#40332=ORIENTED_EDGE('',*,*,#31045,.F.);
#40333=ORIENTED_EDGE('',*,*,#31084,.F.);
#40334=ORIENTED_EDGE('',*,*,#31085,.T.);
#40335=ORIENTED_EDGE('',*,*,#31086,.T.);
#40336=ORIENTED_EDGE('',*,*,#31087,.F.);
#40337=ORIENTED_EDGE('',*,*,#31088,.F.);
#40338=ORIENTED_EDGE('',*,*,#31089,.T.);
#40339=ORIENTED_EDGE('',*,*,#31090,.T.);
#40340=ORIENTED_EDGE('',*,*,#31085,.F.);
#40341=ORIENTED_EDGE('',*,*,#31091,.F.);
#40342=ORIENTED_EDGE('',*,*,#31087,.T.);
#40343=ORIENTED_EDGE('',*,*,#31092,.T.);
#40344=ORIENTED_EDGE('',*,*,#31089,.F.);
#40345=ORIENTED_EDGE('',*,*,#31093,.F.);
#40346=ORIENTED_EDGE('',*,*,#31094,.T.);
#40347=ORIENTED_EDGE('',*,*,#31095,.T.);
#40348=ORIENTED_EDGE('',*,*,#31096,.F.);
#40349=ORIENTED_EDGE('',*,*,#31097,.F.);
#40350=ORIENTED_EDGE('',*,*,#31098,.T.);
#40351=ORIENTED_EDGE('',*,*,#31099,.T.);
#40352=ORIENTED_EDGE('',*,*,#31094,.F.);
#40353=ORIENTED_EDGE('',*,*,#31100,.F.);
#40354=ORIENTED_EDGE('',*,*,#31101,.T.);
#40355=ORIENTED_EDGE('',*,*,#31102,.T.);
#40356=ORIENTED_EDGE('',*,*,#31098,.F.);
#40357=ORIENTED_EDGE('',*,*,#31103,.F.);
#40358=ORIENTED_EDGE('',*,*,#31104,.T.);
#40359=ORIENTED_EDGE('',*,*,#31105,.T.);
#40360=ORIENTED_EDGE('',*,*,#31101,.F.);
#40361=ORIENTED_EDGE('',*,*,#31106,.F.);
#40362=ORIENTED_EDGE('',*,*,#31107,.T.);
#40363=ORIENTED_EDGE('',*,*,#31108,.T.);
#40364=ORIENTED_EDGE('',*,*,#31104,.F.);
#40365=ORIENTED_EDGE('',*,*,#31109,.F.);
#40366=ORIENTED_EDGE('',*,*,#31110,.T.);
#40367=ORIENTED_EDGE('',*,*,#31111,.T.);
#40368=ORIENTED_EDGE('',*,*,#31107,.F.);
#40369=ORIENTED_EDGE('',*,*,#31112,.F.);
#40370=ORIENTED_EDGE('',*,*,#31113,.T.);
#40371=ORIENTED_EDGE('',*,*,#31114,.T.);
#40372=ORIENTED_EDGE('',*,*,#31110,.F.);
#40373=ORIENTED_EDGE('',*,*,#31115,.F.);
#40374=ORIENTED_EDGE('',*,*,#31116,.T.);
#40375=ORIENTED_EDGE('',*,*,#31117,.T.);
#40376=ORIENTED_EDGE('',*,*,#31113,.F.);
#40377=ORIENTED_EDGE('',*,*,#31118,.F.);
#40378=ORIENTED_EDGE('',*,*,#31119,.T.);
#40379=ORIENTED_EDGE('',*,*,#31120,.T.);
#40380=ORIENTED_EDGE('',*,*,#31116,.F.);
#40381=ORIENTED_EDGE('',*,*,#31121,.F.);
#40382=ORIENTED_EDGE('',*,*,#31122,.T.);
#40383=ORIENTED_EDGE('',*,*,#31123,.T.);
#40384=ORIENTED_EDGE('',*,*,#31119,.F.);
#40385=ORIENTED_EDGE('',*,*,#31124,.F.);
#40386=ORIENTED_EDGE('',*,*,#31096,.T.);
#40387=ORIENTED_EDGE('',*,*,#31125,.T.);
#40388=ORIENTED_EDGE('',*,*,#31122,.F.);
#40389=ORIENTED_EDGE('',*,*,#31125,.F.);
#40390=ORIENTED_EDGE('',*,*,#31095,.F.);
#40391=ORIENTED_EDGE('',*,*,#31099,.F.);
#40392=ORIENTED_EDGE('',*,*,#31102,.F.);
#40393=ORIENTED_EDGE('',*,*,#31105,.F.);
#40394=ORIENTED_EDGE('',*,*,#31108,.F.);
#40395=ORIENTED_EDGE('',*,*,#31111,.F.);
#40396=ORIENTED_EDGE('',*,*,#31114,.F.);
#40397=ORIENTED_EDGE('',*,*,#31117,.F.);
#40398=ORIENTED_EDGE('',*,*,#31120,.F.);
#40399=ORIENTED_EDGE('',*,*,#31123,.F.);
#40400=ORIENTED_EDGE('',*,*,#31092,.F.);
#40401=ORIENTED_EDGE('',*,*,#31086,.F.);
#40402=ORIENTED_EDGE('',*,*,#31090,.F.);
#40403=ORIENTED_EDGE('',*,*,#31084,.T.);
#40404=ORIENTED_EDGE('',*,*,#31091,.T.);
#40405=ORIENTED_EDGE('',*,*,#31088,.T.);
#40406=ORIENTED_EDGE('',*,*,#31024,.T.);
#40407=ORIENTED_EDGE('',*,*,#31046,.T.);
#40408=ORIENTED_EDGE('',*,*,#31043,.T.);
#40409=ORIENTED_EDGE('',*,*,#31040,.T.);
#40410=ORIENTED_EDGE('',*,*,#31037,.T.);
#40411=ORIENTED_EDGE('',*,*,#31034,.T.);
#40412=ORIENTED_EDGE('',*,*,#31031,.T.);
#40413=ORIENTED_EDGE('',*,*,#31028,.T.);
#40414=ORIENTED_EDGE('',*,*,#31126,.F.);
#40415=ORIENTED_EDGE('',*,*,#31127,.T.);
#40416=ORIENTED_EDGE('',*,*,#31128,.T.);
#40417=ORIENTED_EDGE('',*,*,#31129,.F.);
#40418=ORIENTED_EDGE('',*,*,#31130,.F.);
#40419=ORIENTED_EDGE('',*,*,#31131,.T.);
#40420=ORIENTED_EDGE('',*,*,#31132,.T.);
#40421=ORIENTED_EDGE('',*,*,#31127,.F.);
#40422=ORIENTED_EDGE('',*,*,#31133,.F.);
#40423=ORIENTED_EDGE('',*,*,#31134,.T.);
#40424=ORIENTED_EDGE('',*,*,#31135,.T.);
#40425=ORIENTED_EDGE('',*,*,#31131,.F.);
#40426=ORIENTED_EDGE('',*,*,#31136,.F.);
#40427=ORIENTED_EDGE('',*,*,#31137,.T.);
#40428=ORIENTED_EDGE('',*,*,#31138,.T.);
#40429=ORIENTED_EDGE('',*,*,#31134,.F.);
#40430=ORIENTED_EDGE('',*,*,#31139,.F.);
#40431=ORIENTED_EDGE('',*,*,#31140,.T.);
#40432=ORIENTED_EDGE('',*,*,#31141,.T.);
#40433=ORIENTED_EDGE('',*,*,#31137,.F.);
#40434=ORIENTED_EDGE('',*,*,#31142,.F.);
#40435=ORIENTED_EDGE('',*,*,#31143,.T.);
#40436=ORIENTED_EDGE('',*,*,#31144,.T.);
#40437=ORIENTED_EDGE('',*,*,#31140,.F.);
#40438=ORIENTED_EDGE('',*,*,#31145,.F.);
#40439=ORIENTED_EDGE('',*,*,#31146,.T.);
#40440=ORIENTED_EDGE('',*,*,#31147,.T.);
#40441=ORIENTED_EDGE('',*,*,#31143,.F.);
#40442=ORIENTED_EDGE('',*,*,#31148,.F.);
#40443=ORIENTED_EDGE('',*,*,#31129,.T.);
#40444=ORIENTED_EDGE('',*,*,#31149,.T.);
#40445=ORIENTED_EDGE('',*,*,#31146,.F.);
#40446=ORIENTED_EDGE('',*,*,#31150,.F.);
#40447=ORIENTED_EDGE('',*,*,#31151,.T.);
#40448=ORIENTED_EDGE('',*,*,#31152,.T.);
#40449=ORIENTED_EDGE('',*,*,#31153,.F.);
#40450=ORIENTED_EDGE('',*,*,#31154,.F.);
#40451=ORIENTED_EDGE('',*,*,#31155,.T.);
#40452=ORIENTED_EDGE('',*,*,#31156,.T.);
#40453=ORIENTED_EDGE('',*,*,#31151,.F.);
#40454=ORIENTED_EDGE('',*,*,#31157,.F.);
#40455=ORIENTED_EDGE('',*,*,#31158,.T.);
#40456=ORIENTED_EDGE('',*,*,#31159,.T.);
#40457=ORIENTED_EDGE('',*,*,#31155,.F.);
#40458=ORIENTED_EDGE('',*,*,#31160,.F.);
#40459=ORIENTED_EDGE('',*,*,#31161,.T.);
#40460=ORIENTED_EDGE('',*,*,#31162,.T.);
#40461=ORIENTED_EDGE('',*,*,#31158,.F.);
#40462=ORIENTED_EDGE('',*,*,#31163,.F.);
#40463=ORIENTED_EDGE('',*,*,#31164,.T.);
#40464=ORIENTED_EDGE('',*,*,#31165,.T.);
#40465=ORIENTED_EDGE('',*,*,#31161,.F.);
#40466=ORIENTED_EDGE('',*,*,#31166,.F.);
#40467=ORIENTED_EDGE('',*,*,#31167,.T.);
#40468=ORIENTED_EDGE('',*,*,#31168,.T.);
#40469=ORIENTED_EDGE('',*,*,#31164,.F.);
#40470=ORIENTED_EDGE('',*,*,#31169,.F.);
#40471=ORIENTED_EDGE('',*,*,#31170,.T.);
#40472=ORIENTED_EDGE('',*,*,#31171,.T.);
#40473=ORIENTED_EDGE('',*,*,#31167,.F.);
#40474=ORIENTED_EDGE('',*,*,#31172,.F.);
#40475=ORIENTED_EDGE('',*,*,#31173,.T.);
#40476=ORIENTED_EDGE('',*,*,#31174,.T.);
#40477=ORIENTED_EDGE('',*,*,#31170,.F.);
#40478=ORIENTED_EDGE('',*,*,#31175,.F.);
#40479=ORIENTED_EDGE('',*,*,#31176,.T.);
#40480=ORIENTED_EDGE('',*,*,#31177,.T.);
#40481=ORIENTED_EDGE('',*,*,#31173,.F.);
#40482=ORIENTED_EDGE('',*,*,#31178,.F.);
#40483=ORIENTED_EDGE('',*,*,#31179,.T.);
#40484=ORIENTED_EDGE('',*,*,#31180,.T.);
#40485=ORIENTED_EDGE('',*,*,#31176,.F.);
#40486=ORIENTED_EDGE('',*,*,#31181,.F.);
#40487=ORIENTED_EDGE('',*,*,#31182,.T.);
#40488=ORIENTED_EDGE('',*,*,#31183,.T.);
#40489=ORIENTED_EDGE('',*,*,#31179,.F.);
#40490=ORIENTED_EDGE('',*,*,#31184,.F.);
#40491=ORIENTED_EDGE('',*,*,#31153,.T.);
#40492=ORIENTED_EDGE('',*,*,#31185,.T.);
#40493=ORIENTED_EDGE('',*,*,#31182,.F.);
#40494=ORIENTED_EDGE('',*,*,#31185,.F.);
#40495=ORIENTED_EDGE('',*,*,#31152,.F.);
#40496=ORIENTED_EDGE('',*,*,#31156,.F.);
#40497=ORIENTED_EDGE('',*,*,#31159,.F.);
#40498=ORIENTED_EDGE('',*,*,#31162,.F.);
#40499=ORIENTED_EDGE('',*,*,#31165,.F.);
#40500=ORIENTED_EDGE('',*,*,#31168,.F.);
#40501=ORIENTED_EDGE('',*,*,#31171,.F.);
#40502=ORIENTED_EDGE('',*,*,#31174,.F.);
#40503=ORIENTED_EDGE('',*,*,#31177,.F.);
#40504=ORIENTED_EDGE('',*,*,#31180,.F.);
#40505=ORIENTED_EDGE('',*,*,#31183,.F.);
#40506=ORIENTED_EDGE('',*,*,#31149,.F.);
#40507=ORIENTED_EDGE('',*,*,#31128,.F.);
#40508=ORIENTED_EDGE('',*,*,#31132,.F.);
#40509=ORIENTED_EDGE('',*,*,#31135,.F.);
#40510=ORIENTED_EDGE('',*,*,#31138,.F.);
#40511=ORIENTED_EDGE('',*,*,#31141,.F.);
#40512=ORIENTED_EDGE('',*,*,#31144,.F.);
#40513=ORIENTED_EDGE('',*,*,#31147,.F.);
#40514=ORIENTED_EDGE('',*,*,#31186,.F.);
#40515=ORIENTED_EDGE('',*,*,#31187,.T.);
#40516=ORIENTED_EDGE('',*,*,#31188,.T.);
#40517=ORIENTED_EDGE('',*,*,#31189,.F.);
#40518=ORIENTED_EDGE('',*,*,#31190,.F.);
#40519=ORIENTED_EDGE('',*,*,#31191,.T.);
#40520=ORIENTED_EDGE('',*,*,#31192,.T.);
#40521=ORIENTED_EDGE('',*,*,#31187,.F.);
#40522=ORIENTED_EDGE('',*,*,#31193,.F.);
#40523=ORIENTED_EDGE('',*,*,#31194,.T.);
#40524=ORIENTED_EDGE('',*,*,#31195,.T.);
#40525=ORIENTED_EDGE('',*,*,#31191,.F.);
#40526=ORIENTED_EDGE('',*,*,#31196,.F.);
#40527=ORIENTED_EDGE('',*,*,#31197,.T.);
#40528=ORIENTED_EDGE('',*,*,#31198,.T.);
#40529=ORIENTED_EDGE('',*,*,#31194,.F.);
#40530=ORIENTED_EDGE('',*,*,#31199,.F.);
#40531=ORIENTED_EDGE('',*,*,#31200,.T.);
#40532=ORIENTED_EDGE('',*,*,#31201,.T.);
#40533=ORIENTED_EDGE('',*,*,#31197,.F.);
#40534=ORIENTED_EDGE('',*,*,#31202,.F.);
#40535=ORIENTED_EDGE('',*,*,#31203,.T.);
#40536=ORIENTED_EDGE('',*,*,#31204,.T.);
#40537=ORIENTED_EDGE('',*,*,#31200,.F.);
#40538=ORIENTED_EDGE('',*,*,#31205,.F.);
#40539=ORIENTED_EDGE('',*,*,#31206,.T.);
#40540=ORIENTED_EDGE('',*,*,#31207,.T.);
#40541=ORIENTED_EDGE('',*,*,#31203,.F.);
#40542=ORIENTED_EDGE('',*,*,#31208,.F.);
#40543=ORIENTED_EDGE('',*,*,#31209,.T.);
#40544=ORIENTED_EDGE('',*,*,#31210,.T.);
#40545=ORIENTED_EDGE('',*,*,#31206,.F.);
#40546=ORIENTED_EDGE('',*,*,#31211,.F.);
#40547=ORIENTED_EDGE('',*,*,#31212,.T.);
#40548=ORIENTED_EDGE('',*,*,#31213,.T.);
#40549=ORIENTED_EDGE('',*,*,#31209,.F.);
#40550=ORIENTED_EDGE('',*,*,#31214,.F.);
#40551=ORIENTED_EDGE('',*,*,#31215,.T.);
#40552=ORIENTED_EDGE('',*,*,#31216,.T.);
#40553=ORIENTED_EDGE('',*,*,#31212,.F.);
#40554=ORIENTED_EDGE('',*,*,#31217,.F.);
#40555=ORIENTED_EDGE('',*,*,#31218,.T.);
#40556=ORIENTED_EDGE('',*,*,#31219,.T.);
#40557=ORIENTED_EDGE('',*,*,#31215,.F.);
#40558=ORIENTED_EDGE('',*,*,#31220,.F.);
#40559=ORIENTED_EDGE('',*,*,#31221,.T.);
#40560=ORIENTED_EDGE('',*,*,#31222,.T.);
#40561=ORIENTED_EDGE('',*,*,#31218,.F.);
#40562=ORIENTED_EDGE('',*,*,#31223,.F.);
#40563=ORIENTED_EDGE('',*,*,#31224,.T.);
#40564=ORIENTED_EDGE('',*,*,#31225,.T.);
#40565=ORIENTED_EDGE('',*,*,#31221,.F.);
#40566=ORIENTED_EDGE('',*,*,#31226,.F.);
#40567=ORIENTED_EDGE('',*,*,#31227,.T.);
#40568=ORIENTED_EDGE('',*,*,#31228,.T.);
#40569=ORIENTED_EDGE('',*,*,#31224,.F.);
#40570=ORIENTED_EDGE('',*,*,#31229,.F.);
#40571=ORIENTED_EDGE('',*,*,#31230,.T.);
#40572=ORIENTED_EDGE('',*,*,#31231,.T.);
#40573=ORIENTED_EDGE('',*,*,#31227,.F.);
#40574=ORIENTED_EDGE('',*,*,#31232,.F.);
#40575=ORIENTED_EDGE('',*,*,#31233,.T.);
#40576=ORIENTED_EDGE('',*,*,#31234,.T.);
#40577=ORIENTED_EDGE('',*,*,#31230,.F.);
#40578=ORIENTED_EDGE('',*,*,#31235,.F.);
#40579=ORIENTED_EDGE('',*,*,#31236,.T.);
#40580=ORIENTED_EDGE('',*,*,#31237,.T.);
#40581=ORIENTED_EDGE('',*,*,#31233,.F.);
#40582=ORIENTED_EDGE('',*,*,#31238,.F.);
#40583=ORIENTED_EDGE('',*,*,#31239,.T.);
#40584=ORIENTED_EDGE('',*,*,#31240,.T.);
#40585=ORIENTED_EDGE('',*,*,#31236,.F.);
#40586=ORIENTED_EDGE('',*,*,#31241,.F.);
#40587=ORIENTED_EDGE('',*,*,#31242,.T.);
#40588=ORIENTED_EDGE('',*,*,#31243,.T.);
#40589=ORIENTED_EDGE('',*,*,#31239,.F.);
#40590=ORIENTED_EDGE('',*,*,#31244,.F.);
#40591=ORIENTED_EDGE('',*,*,#31245,.T.);
#40592=ORIENTED_EDGE('',*,*,#31246,.T.);
#40593=ORIENTED_EDGE('',*,*,#31242,.F.);
#40594=ORIENTED_EDGE('',*,*,#31247,.F.);
#40595=ORIENTED_EDGE('',*,*,#31248,.T.);
#40596=ORIENTED_EDGE('',*,*,#31249,.T.);
#40597=ORIENTED_EDGE('',*,*,#31245,.F.);
#40598=ORIENTED_EDGE('',*,*,#31250,.F.);
#40599=ORIENTED_EDGE('',*,*,#31251,.T.);
#40600=ORIENTED_EDGE('',*,*,#31252,.T.);
#40601=ORIENTED_EDGE('',*,*,#31248,.F.);
#40602=ORIENTED_EDGE('',*,*,#31253,.F.);
#40603=ORIENTED_EDGE('',*,*,#31254,.T.);
#40604=ORIENTED_EDGE('',*,*,#31255,.T.);
#40605=ORIENTED_EDGE('',*,*,#31251,.F.);
#40606=ORIENTED_EDGE('',*,*,#31256,.F.);
#40607=ORIENTED_EDGE('',*,*,#31257,.T.);
#40608=ORIENTED_EDGE('',*,*,#31258,.T.);
#40609=ORIENTED_EDGE('',*,*,#31254,.F.);
#40610=ORIENTED_EDGE('',*,*,#31259,.F.);
#40611=ORIENTED_EDGE('',*,*,#31260,.T.);
#40612=ORIENTED_EDGE('',*,*,#31261,.T.);
#40613=ORIENTED_EDGE('',*,*,#31257,.F.);
#40614=ORIENTED_EDGE('',*,*,#31262,.F.);
#40615=ORIENTED_EDGE('',*,*,#31263,.T.);
#40616=ORIENTED_EDGE('',*,*,#31264,.T.);
#40617=ORIENTED_EDGE('',*,*,#31260,.F.);
#40618=ORIENTED_EDGE('',*,*,#31265,.F.);
#40619=ORIENTED_EDGE('',*,*,#31266,.T.);
#40620=ORIENTED_EDGE('',*,*,#31267,.T.);
#40621=ORIENTED_EDGE('',*,*,#31263,.F.);
#40622=ORIENTED_EDGE('',*,*,#31268,.F.);
#40623=ORIENTED_EDGE('',*,*,#31269,.T.);
#40624=ORIENTED_EDGE('',*,*,#31270,.T.);
#40625=ORIENTED_EDGE('',*,*,#31266,.F.);
#40626=ORIENTED_EDGE('',*,*,#31271,.F.);
#40627=ORIENTED_EDGE('',*,*,#31272,.T.);
#40628=ORIENTED_EDGE('',*,*,#31273,.T.);
#40629=ORIENTED_EDGE('',*,*,#31269,.F.);
#40630=ORIENTED_EDGE('',*,*,#31274,.F.);
#40631=ORIENTED_EDGE('',*,*,#31189,.T.);
#40632=ORIENTED_EDGE('',*,*,#31275,.T.);
#40633=ORIENTED_EDGE('',*,*,#31272,.F.);
#40634=ORIENTED_EDGE('',*,*,#31275,.F.);
#40635=ORIENTED_EDGE('',*,*,#31188,.F.);
#40636=ORIENTED_EDGE('',*,*,#31192,.F.);
#40637=ORIENTED_EDGE('',*,*,#31195,.F.);
#40638=ORIENTED_EDGE('',*,*,#31198,.F.);
#40639=ORIENTED_EDGE('',*,*,#31201,.F.);
#40640=ORIENTED_EDGE('',*,*,#31204,.F.);
#40641=ORIENTED_EDGE('',*,*,#31207,.F.);
#40642=ORIENTED_EDGE('',*,*,#31210,.F.);
#40643=ORIENTED_EDGE('',*,*,#31213,.F.);
#40644=ORIENTED_EDGE('',*,*,#31216,.F.);
#40645=ORIENTED_EDGE('',*,*,#31219,.F.);
#40646=ORIENTED_EDGE('',*,*,#31222,.F.);
#40647=ORIENTED_EDGE('',*,*,#31225,.F.);
#40648=ORIENTED_EDGE('',*,*,#31228,.F.);
#40649=ORIENTED_EDGE('',*,*,#31231,.F.);
#40650=ORIENTED_EDGE('',*,*,#31234,.F.);
#40651=ORIENTED_EDGE('',*,*,#31237,.F.);
#40652=ORIENTED_EDGE('',*,*,#31240,.F.);
#40653=ORIENTED_EDGE('',*,*,#31243,.F.);
#40654=ORIENTED_EDGE('',*,*,#31246,.F.);
#40655=ORIENTED_EDGE('',*,*,#31249,.F.);
#40656=ORIENTED_EDGE('',*,*,#31252,.F.);
#40657=ORIENTED_EDGE('',*,*,#31255,.F.);
#40658=ORIENTED_EDGE('',*,*,#31258,.F.);
#40659=ORIENTED_EDGE('',*,*,#31261,.F.);
#40660=ORIENTED_EDGE('',*,*,#31264,.F.);
#40661=ORIENTED_EDGE('',*,*,#31267,.F.);
#40662=ORIENTED_EDGE('',*,*,#31270,.F.);
#40663=ORIENTED_EDGE('',*,*,#31273,.F.);
#40664=ORIENTED_EDGE('',*,*,#31126,.T.);
#40665=ORIENTED_EDGE('',*,*,#31148,.T.);
#40666=ORIENTED_EDGE('',*,*,#31145,.T.);
#40667=ORIENTED_EDGE('',*,*,#31142,.T.);
#40668=ORIENTED_EDGE('',*,*,#31139,.T.);
#40669=ORIENTED_EDGE('',*,*,#31136,.T.);
#40670=ORIENTED_EDGE('',*,*,#31133,.T.);
#40671=ORIENTED_EDGE('',*,*,#31130,.T.);
#40672=ORIENTED_EDGE('',*,*,#31276,.F.);
#40673=ORIENTED_EDGE('',*,*,#31277,.T.);
#40674=ORIENTED_EDGE('',*,*,#31278,.T.);
#40675=ORIENTED_EDGE('',*,*,#31279,.F.);
#40676=ORIENTED_EDGE('',*,*,#31280,.F.);
#40677=ORIENTED_EDGE('',*,*,#31281,.T.);
#40678=ORIENTED_EDGE('',*,*,#31282,.T.);
#40679=ORIENTED_EDGE('',*,*,#31277,.F.);
#40680=ORIENTED_EDGE('',*,*,#31283,.F.);
#40681=ORIENTED_EDGE('',*,*,#31284,.T.);
#40682=ORIENTED_EDGE('',*,*,#31285,.T.);
#40683=ORIENTED_EDGE('',*,*,#31281,.F.);
#40684=ORIENTED_EDGE('',*,*,#31286,.F.);
#40685=ORIENTED_EDGE('',*,*,#31287,.T.);
#40686=ORIENTED_EDGE('',*,*,#31288,.T.);
#40687=ORIENTED_EDGE('',*,*,#31284,.F.);
#40688=ORIENTED_EDGE('',*,*,#31289,.F.);
#40689=ORIENTED_EDGE('',*,*,#31290,.T.);
#40690=ORIENTED_EDGE('',*,*,#31291,.T.);
#40691=ORIENTED_EDGE('',*,*,#31287,.F.);
#40692=ORIENTED_EDGE('',*,*,#31292,.F.);
#40693=ORIENTED_EDGE('',*,*,#31293,.T.);
#40694=ORIENTED_EDGE('',*,*,#31294,.T.);
#40695=ORIENTED_EDGE('',*,*,#31290,.F.);
#40696=ORIENTED_EDGE('',*,*,#31295,.F.);
#40697=ORIENTED_EDGE('',*,*,#31296,.T.);
#40698=ORIENTED_EDGE('',*,*,#31297,.T.);
#40699=ORIENTED_EDGE('',*,*,#31293,.F.);
#40700=ORIENTED_EDGE('',*,*,#31298,.F.);
#40701=ORIENTED_EDGE('',*,*,#31279,.T.);
#40702=ORIENTED_EDGE('',*,*,#31299,.T.);
#40703=ORIENTED_EDGE('',*,*,#31296,.F.);
#40704=ORIENTED_EDGE('',*,*,#31300,.F.);
#40705=ORIENTED_EDGE('',*,*,#31301,.T.);
#40706=ORIENTED_EDGE('',*,*,#31302,.T.);
#40707=ORIENTED_EDGE('',*,*,#31303,.F.);
#40708=ORIENTED_EDGE('',*,*,#31304,.F.);
#40709=ORIENTED_EDGE('',*,*,#31305,.T.);
#40710=ORIENTED_EDGE('',*,*,#31306,.T.);
#40711=ORIENTED_EDGE('',*,*,#31301,.F.);
#40712=ORIENTED_EDGE('',*,*,#31307,.F.);
#40713=ORIENTED_EDGE('',*,*,#31308,.T.);
#40714=ORIENTED_EDGE('',*,*,#31309,.T.);
#40715=ORIENTED_EDGE('',*,*,#31305,.F.);
#40716=ORIENTED_EDGE('',*,*,#31310,.F.);
#40717=ORIENTED_EDGE('',*,*,#31311,.T.);
#40718=ORIENTED_EDGE('',*,*,#31312,.T.);
#40719=ORIENTED_EDGE('',*,*,#31308,.F.);
#40720=ORIENTED_EDGE('',*,*,#31313,.F.);
#40721=ORIENTED_EDGE('',*,*,#31314,.T.);
#40722=ORIENTED_EDGE('',*,*,#31315,.T.);
#40723=ORIENTED_EDGE('',*,*,#31311,.F.);
#40724=ORIENTED_EDGE('',*,*,#31316,.F.);
#40725=ORIENTED_EDGE('',*,*,#31317,.T.);
#40726=ORIENTED_EDGE('',*,*,#31318,.T.);
#40727=ORIENTED_EDGE('',*,*,#31314,.F.);
#40728=ORIENTED_EDGE('',*,*,#31319,.F.);
#40729=ORIENTED_EDGE('',*,*,#31320,.T.);
#40730=ORIENTED_EDGE('',*,*,#31321,.T.);
#40731=ORIENTED_EDGE('',*,*,#31317,.F.);
#40732=ORIENTED_EDGE('',*,*,#31322,.F.);
#40733=ORIENTED_EDGE('',*,*,#31323,.T.);
#40734=ORIENTED_EDGE('',*,*,#31324,.T.);
#40735=ORIENTED_EDGE('',*,*,#31320,.F.);
#40736=ORIENTED_EDGE('',*,*,#31325,.F.);
#40737=ORIENTED_EDGE('',*,*,#31326,.T.);
#40738=ORIENTED_EDGE('',*,*,#31327,.T.);
#40739=ORIENTED_EDGE('',*,*,#31323,.F.);
#40740=ORIENTED_EDGE('',*,*,#31328,.F.);
#40741=ORIENTED_EDGE('',*,*,#31329,.T.);
#40742=ORIENTED_EDGE('',*,*,#31330,.T.);
#40743=ORIENTED_EDGE('',*,*,#31326,.F.);
#40744=ORIENTED_EDGE('',*,*,#31331,.F.);
#40745=ORIENTED_EDGE('',*,*,#31332,.T.);
#40746=ORIENTED_EDGE('',*,*,#31333,.T.);
#40747=ORIENTED_EDGE('',*,*,#31329,.F.);
#40748=ORIENTED_EDGE('',*,*,#31334,.F.);
#40749=ORIENTED_EDGE('',*,*,#31303,.T.);
#40750=ORIENTED_EDGE('',*,*,#31335,.T.);
#40751=ORIENTED_EDGE('',*,*,#31332,.F.);
#40752=ORIENTED_EDGE('',*,*,#31335,.F.);
#40753=ORIENTED_EDGE('',*,*,#31302,.F.);
#40754=ORIENTED_EDGE('',*,*,#31306,.F.);
#40755=ORIENTED_EDGE('',*,*,#31309,.F.);
#40756=ORIENTED_EDGE('',*,*,#31312,.F.);
#40757=ORIENTED_EDGE('',*,*,#31315,.F.);
#40758=ORIENTED_EDGE('',*,*,#31318,.F.);
#40759=ORIENTED_EDGE('',*,*,#31321,.F.);
#40760=ORIENTED_EDGE('',*,*,#31324,.F.);
#40761=ORIENTED_EDGE('',*,*,#31327,.F.);
#40762=ORIENTED_EDGE('',*,*,#31330,.F.);
#40763=ORIENTED_EDGE('',*,*,#31333,.F.);
#40764=ORIENTED_EDGE('',*,*,#31299,.F.);
#40765=ORIENTED_EDGE('',*,*,#31278,.F.);
#40766=ORIENTED_EDGE('',*,*,#31282,.F.);
#40767=ORIENTED_EDGE('',*,*,#31285,.F.);
#40768=ORIENTED_EDGE('',*,*,#31288,.F.);
#40769=ORIENTED_EDGE('',*,*,#31291,.F.);
#40770=ORIENTED_EDGE('',*,*,#31294,.F.);
#40771=ORIENTED_EDGE('',*,*,#31297,.F.);
#40772=ORIENTED_EDGE('',*,*,#31336,.F.);
#40773=ORIENTED_EDGE('',*,*,#31337,.T.);
#40774=ORIENTED_EDGE('',*,*,#31338,.T.);
#40775=ORIENTED_EDGE('',*,*,#31339,.F.);
#40776=ORIENTED_EDGE('',*,*,#31340,.F.);
#40777=ORIENTED_EDGE('',*,*,#31341,.T.);
#40778=ORIENTED_EDGE('',*,*,#31342,.T.);
#40779=ORIENTED_EDGE('',*,*,#31337,.F.);
#40780=ORIENTED_EDGE('',*,*,#31343,.F.);
#40781=ORIENTED_EDGE('',*,*,#31344,.T.);
#40782=ORIENTED_EDGE('',*,*,#31345,.T.);
#40783=ORIENTED_EDGE('',*,*,#31341,.F.);
#40784=ORIENTED_EDGE('',*,*,#31346,.F.);
#40785=ORIENTED_EDGE('',*,*,#31347,.T.);
#40786=ORIENTED_EDGE('',*,*,#31348,.T.);
#40787=ORIENTED_EDGE('',*,*,#31344,.F.);
#40788=ORIENTED_EDGE('',*,*,#31349,.F.);
#40789=ORIENTED_EDGE('',*,*,#31350,.T.);
#40790=ORIENTED_EDGE('',*,*,#31351,.T.);
#40791=ORIENTED_EDGE('',*,*,#31347,.F.);
#40792=ORIENTED_EDGE('',*,*,#31352,.F.);
#40793=ORIENTED_EDGE('',*,*,#31353,.T.);
#40794=ORIENTED_EDGE('',*,*,#31354,.T.);
#40795=ORIENTED_EDGE('',*,*,#31350,.F.);
#40796=ORIENTED_EDGE('',*,*,#31355,.F.);
#40797=ORIENTED_EDGE('',*,*,#31356,.T.);
#40798=ORIENTED_EDGE('',*,*,#31357,.T.);
#40799=ORIENTED_EDGE('',*,*,#31353,.F.);
#40800=ORIENTED_EDGE('',*,*,#31358,.F.);
#40801=ORIENTED_EDGE('',*,*,#31359,.T.);
#40802=ORIENTED_EDGE('',*,*,#31360,.T.);
#40803=ORIENTED_EDGE('',*,*,#31356,.F.);
#40804=ORIENTED_EDGE('',*,*,#31361,.F.);
#40805=ORIENTED_EDGE('',*,*,#31362,.T.);
#40806=ORIENTED_EDGE('',*,*,#31363,.T.);
#40807=ORIENTED_EDGE('',*,*,#31359,.F.);
#40808=ORIENTED_EDGE('',*,*,#31364,.F.);
#40809=ORIENTED_EDGE('',*,*,#31365,.T.);
#40810=ORIENTED_EDGE('',*,*,#31366,.T.);
#40811=ORIENTED_EDGE('',*,*,#31362,.F.);
#40812=ORIENTED_EDGE('',*,*,#31367,.F.);
#40813=ORIENTED_EDGE('',*,*,#31368,.T.);
#40814=ORIENTED_EDGE('',*,*,#31369,.T.);
#40815=ORIENTED_EDGE('',*,*,#31365,.F.);
#40816=ORIENTED_EDGE('',*,*,#31370,.F.);
#40817=ORIENTED_EDGE('',*,*,#31371,.T.);
#40818=ORIENTED_EDGE('',*,*,#31372,.T.);
#40819=ORIENTED_EDGE('',*,*,#31368,.F.);
#40820=ORIENTED_EDGE('',*,*,#31373,.F.);
#40821=ORIENTED_EDGE('',*,*,#31374,.T.);
#40822=ORIENTED_EDGE('',*,*,#31375,.T.);
#40823=ORIENTED_EDGE('',*,*,#31371,.F.);
#40824=ORIENTED_EDGE('',*,*,#31376,.F.);
#40825=ORIENTED_EDGE('',*,*,#31377,.T.);
#40826=ORIENTED_EDGE('',*,*,#31378,.T.);
#40827=ORIENTED_EDGE('',*,*,#31374,.F.);
#40828=ORIENTED_EDGE('',*,*,#31379,.F.);
#40829=ORIENTED_EDGE('',*,*,#31380,.T.);
#40830=ORIENTED_EDGE('',*,*,#31381,.T.);
#40831=ORIENTED_EDGE('',*,*,#31377,.F.);
#40832=ORIENTED_EDGE('',*,*,#31382,.F.);
#40833=ORIENTED_EDGE('',*,*,#31383,.T.);
#40834=ORIENTED_EDGE('',*,*,#31384,.T.);
#40835=ORIENTED_EDGE('',*,*,#31380,.F.);
#40836=ORIENTED_EDGE('',*,*,#31385,.F.);
#40837=ORIENTED_EDGE('',*,*,#31386,.T.);
#40838=ORIENTED_EDGE('',*,*,#31387,.T.);
#40839=ORIENTED_EDGE('',*,*,#31383,.F.);
#40840=ORIENTED_EDGE('',*,*,#31388,.F.);
#40841=ORIENTED_EDGE('',*,*,#31389,.T.);
#40842=ORIENTED_EDGE('',*,*,#31390,.T.);
#40843=ORIENTED_EDGE('',*,*,#31386,.F.);
#40844=ORIENTED_EDGE('',*,*,#31391,.F.);
#40845=ORIENTED_EDGE('',*,*,#31392,.T.);
#40846=ORIENTED_EDGE('',*,*,#31393,.T.);
#40847=ORIENTED_EDGE('',*,*,#31389,.F.);
#40848=ORIENTED_EDGE('',*,*,#31394,.F.);
#40849=ORIENTED_EDGE('',*,*,#31395,.T.);
#40850=ORIENTED_EDGE('',*,*,#31396,.T.);
#40851=ORIENTED_EDGE('',*,*,#31392,.F.);
#40852=ORIENTED_EDGE('',*,*,#31397,.F.);
#40853=ORIENTED_EDGE('',*,*,#31398,.T.);
#40854=ORIENTED_EDGE('',*,*,#31399,.T.);
#40855=ORIENTED_EDGE('',*,*,#31395,.F.);
#40856=ORIENTED_EDGE('',*,*,#31400,.F.);
#40857=ORIENTED_EDGE('',*,*,#31339,.T.);
#40858=ORIENTED_EDGE('',*,*,#31401,.T.);
#40859=ORIENTED_EDGE('',*,*,#31398,.F.);
#40860=ORIENTED_EDGE('',*,*,#31401,.F.);
#40861=ORIENTED_EDGE('',*,*,#31338,.F.);
#40862=ORIENTED_EDGE('',*,*,#31342,.F.);
#40863=ORIENTED_EDGE('',*,*,#31345,.F.);
#40864=ORIENTED_EDGE('',*,*,#31348,.F.);
#40865=ORIENTED_EDGE('',*,*,#31351,.F.);
#40866=ORIENTED_EDGE('',*,*,#31354,.F.);
#40867=ORIENTED_EDGE('',*,*,#31357,.F.);
#40868=ORIENTED_EDGE('',*,*,#31360,.F.);
#40869=ORIENTED_EDGE('',*,*,#31363,.F.);
#40870=ORIENTED_EDGE('',*,*,#31366,.F.);
#40871=ORIENTED_EDGE('',*,*,#31369,.F.);
#40872=ORIENTED_EDGE('',*,*,#31372,.F.);
#40873=ORIENTED_EDGE('',*,*,#31375,.F.);
#40874=ORIENTED_EDGE('',*,*,#31378,.F.);
#40875=ORIENTED_EDGE('',*,*,#31381,.F.);
#40876=ORIENTED_EDGE('',*,*,#31384,.F.);
#40877=ORIENTED_EDGE('',*,*,#31387,.F.);
#40878=ORIENTED_EDGE('',*,*,#31390,.F.);
#40879=ORIENTED_EDGE('',*,*,#31393,.F.);
#40880=ORIENTED_EDGE('',*,*,#31396,.F.);
#40881=ORIENTED_EDGE('',*,*,#31399,.F.);
#40882=ORIENTED_EDGE('',*,*,#31276,.T.);
#40883=ORIENTED_EDGE('',*,*,#31298,.T.);
#40884=ORIENTED_EDGE('',*,*,#31295,.T.);
#40885=ORIENTED_EDGE('',*,*,#31292,.T.);
#40886=ORIENTED_EDGE('',*,*,#31289,.T.);
#40887=ORIENTED_EDGE('',*,*,#31286,.T.);
#40888=ORIENTED_EDGE('',*,*,#31283,.T.);
#40889=ORIENTED_EDGE('',*,*,#31280,.T.);
#40890=ORIENTED_EDGE('',*,*,#31402,.F.);
#40891=ORIENTED_EDGE('',*,*,#31403,.T.);
#40892=ORIENTED_EDGE('',*,*,#31404,.T.);
#40893=ORIENTED_EDGE('',*,*,#31405,.F.);
#40894=ORIENTED_EDGE('',*,*,#31406,.F.);
#40895=ORIENTED_EDGE('',*,*,#31407,.T.);
#40896=ORIENTED_EDGE('',*,*,#31408,.T.);
#40897=ORIENTED_EDGE('',*,*,#31403,.F.);
#40898=ORIENTED_EDGE('',*,*,#31409,.F.);
#40899=ORIENTED_EDGE('',*,*,#31410,.T.);
#40900=ORIENTED_EDGE('',*,*,#31411,.T.);
#40901=ORIENTED_EDGE('',*,*,#31407,.F.);
#40902=ORIENTED_EDGE('',*,*,#31412,.F.);
#40903=ORIENTED_EDGE('',*,*,#31413,.T.);
#40904=ORIENTED_EDGE('',*,*,#31414,.T.);
#40905=ORIENTED_EDGE('',*,*,#31410,.F.);
#40906=ORIENTED_EDGE('',*,*,#31415,.F.);
#40907=ORIENTED_EDGE('',*,*,#31416,.T.);
#40908=ORIENTED_EDGE('',*,*,#31417,.T.);
#40909=ORIENTED_EDGE('',*,*,#31413,.F.);
#40910=ORIENTED_EDGE('',*,*,#31418,.F.);
#40911=ORIENTED_EDGE('',*,*,#31419,.T.);
#40912=ORIENTED_EDGE('',*,*,#31420,.T.);
#40913=ORIENTED_EDGE('',*,*,#31416,.F.);
#40914=ORIENTED_EDGE('',*,*,#31421,.F.);
#40915=ORIENTED_EDGE('',*,*,#31422,.T.);
#40916=ORIENTED_EDGE('',*,*,#31423,.T.);
#40917=ORIENTED_EDGE('',*,*,#31419,.F.);
#40918=ORIENTED_EDGE('',*,*,#31424,.F.);
#40919=ORIENTED_EDGE('',*,*,#31405,.T.);
#40920=ORIENTED_EDGE('',*,*,#31425,.T.);
#40921=ORIENTED_EDGE('',*,*,#31422,.F.);
#40922=ORIENTED_EDGE('',*,*,#31426,.F.);
#40923=ORIENTED_EDGE('',*,*,#31427,.T.);
#40924=ORIENTED_EDGE('',*,*,#31428,.T.);
#40925=ORIENTED_EDGE('',*,*,#31429,.F.);
#40926=ORIENTED_EDGE('',*,*,#31430,.F.);
#40927=ORIENTED_EDGE('',*,*,#31431,.T.);
#40928=ORIENTED_EDGE('',*,*,#31432,.T.);
#40929=ORIENTED_EDGE('',*,*,#31427,.F.);
#40930=ORIENTED_EDGE('',*,*,#31433,.F.);
#40931=ORIENTED_EDGE('',*,*,#31434,.T.);
#40932=ORIENTED_EDGE('',*,*,#31435,.T.);
#40933=ORIENTED_EDGE('',*,*,#31431,.F.);
#40934=ORIENTED_EDGE('',*,*,#31436,.F.);
#40935=ORIENTED_EDGE('',*,*,#31437,.T.);
#40936=ORIENTED_EDGE('',*,*,#31438,.T.);
#40937=ORIENTED_EDGE('',*,*,#31434,.F.);
#40938=ORIENTED_EDGE('',*,*,#31439,.F.);
#40939=ORIENTED_EDGE('',*,*,#31440,.T.);
#40940=ORIENTED_EDGE('',*,*,#31441,.T.);
#40941=ORIENTED_EDGE('',*,*,#31437,.F.);
#40942=ORIENTED_EDGE('',*,*,#31442,.F.);
#40943=ORIENTED_EDGE('',*,*,#31443,.T.);
#40944=ORIENTED_EDGE('',*,*,#31444,.T.);
#40945=ORIENTED_EDGE('',*,*,#31440,.F.);
#40946=ORIENTED_EDGE('',*,*,#31445,.F.);
#40947=ORIENTED_EDGE('',*,*,#31446,.T.);
#40948=ORIENTED_EDGE('',*,*,#31447,.T.);
#40949=ORIENTED_EDGE('',*,*,#31443,.F.);
#40950=ORIENTED_EDGE('',*,*,#31448,.F.);
#40951=ORIENTED_EDGE('',*,*,#31449,.T.);
#40952=ORIENTED_EDGE('',*,*,#31450,.T.);
#40953=ORIENTED_EDGE('',*,*,#31446,.F.);
#40954=ORIENTED_EDGE('',*,*,#31451,.F.);
#40955=ORIENTED_EDGE('',*,*,#31452,.T.);
#40956=ORIENTED_EDGE('',*,*,#31453,.T.);
#40957=ORIENTED_EDGE('',*,*,#31449,.F.);
#40958=ORIENTED_EDGE('',*,*,#31454,.F.);
#40959=ORIENTED_EDGE('',*,*,#31455,.T.);
#40960=ORIENTED_EDGE('',*,*,#31456,.T.);
#40961=ORIENTED_EDGE('',*,*,#31452,.F.);
#40962=ORIENTED_EDGE('',*,*,#31457,.F.);
#40963=ORIENTED_EDGE('',*,*,#31458,.T.);
#40964=ORIENTED_EDGE('',*,*,#31459,.T.);
#40965=ORIENTED_EDGE('',*,*,#31455,.F.);
#40966=ORIENTED_EDGE('',*,*,#31460,.F.);
#40967=ORIENTED_EDGE('',*,*,#31429,.T.);
#40968=ORIENTED_EDGE('',*,*,#31461,.T.);
#40969=ORIENTED_EDGE('',*,*,#31458,.F.);
#40970=ORIENTED_EDGE('',*,*,#31461,.F.);
#40971=ORIENTED_EDGE('',*,*,#31428,.F.);
#40972=ORIENTED_EDGE('',*,*,#31432,.F.);
#40973=ORIENTED_EDGE('',*,*,#31435,.F.);
#40974=ORIENTED_EDGE('',*,*,#31438,.F.);
#40975=ORIENTED_EDGE('',*,*,#31441,.F.);
#40976=ORIENTED_EDGE('',*,*,#31444,.F.);
#40977=ORIENTED_EDGE('',*,*,#31447,.F.);
#40978=ORIENTED_EDGE('',*,*,#31450,.F.);
#40979=ORIENTED_EDGE('',*,*,#31453,.F.);
#40980=ORIENTED_EDGE('',*,*,#31456,.F.);
#40981=ORIENTED_EDGE('',*,*,#31459,.F.);
#40982=ORIENTED_EDGE('',*,*,#31425,.F.);
#40983=ORIENTED_EDGE('',*,*,#31404,.F.);
#40984=ORIENTED_EDGE('',*,*,#31408,.F.);
#40985=ORIENTED_EDGE('',*,*,#31411,.F.);
#40986=ORIENTED_EDGE('',*,*,#31414,.F.);
#40987=ORIENTED_EDGE('',*,*,#31417,.F.);
#40988=ORIENTED_EDGE('',*,*,#31420,.F.);
#40989=ORIENTED_EDGE('',*,*,#31423,.F.);
#40990=ORIENTED_EDGE('',*,*,#31462,.F.);
#40991=ORIENTED_EDGE('',*,*,#31463,.T.);
#40992=ORIENTED_EDGE('',*,*,#31464,.T.);
#40993=ORIENTED_EDGE('',*,*,#31465,.F.);
#40994=ORIENTED_EDGE('',*,*,#31466,.F.);
#40995=ORIENTED_EDGE('',*,*,#31467,.T.);
#40996=ORIENTED_EDGE('',*,*,#31468,.T.);
#40997=ORIENTED_EDGE('',*,*,#31463,.F.);
#40998=ORIENTED_EDGE('',*,*,#31469,.F.);
#40999=ORIENTED_EDGE('',*,*,#31470,.T.);
#41000=ORIENTED_EDGE('',*,*,#31471,.T.);
#41001=ORIENTED_EDGE('',*,*,#31467,.F.);
#41002=ORIENTED_EDGE('',*,*,#31472,.F.);
#41003=ORIENTED_EDGE('',*,*,#31473,.T.);
#41004=ORIENTED_EDGE('',*,*,#31474,.T.);
#41005=ORIENTED_EDGE('',*,*,#31470,.F.);
#41006=ORIENTED_EDGE('',*,*,#31475,.F.);
#41007=ORIENTED_EDGE('',*,*,#31476,.T.);
#41008=ORIENTED_EDGE('',*,*,#31477,.T.);
#41009=ORIENTED_EDGE('',*,*,#31473,.F.);
#41010=ORIENTED_EDGE('',*,*,#31478,.F.);
#41011=ORIENTED_EDGE('',*,*,#31479,.T.);
#41012=ORIENTED_EDGE('',*,*,#31480,.T.);
#41013=ORIENTED_EDGE('',*,*,#31476,.F.);
#41014=ORIENTED_EDGE('',*,*,#31481,.F.);
#41015=ORIENTED_EDGE('',*,*,#31482,.T.);
#41016=ORIENTED_EDGE('',*,*,#31483,.T.);
#41017=ORIENTED_EDGE('',*,*,#31479,.F.);
#41018=ORIENTED_EDGE('',*,*,#31484,.F.);
#41019=ORIENTED_EDGE('',*,*,#31485,.T.);
#41020=ORIENTED_EDGE('',*,*,#31486,.T.);
#41021=ORIENTED_EDGE('',*,*,#31482,.F.);
#41022=ORIENTED_EDGE('',*,*,#31487,.F.);
#41023=ORIENTED_EDGE('',*,*,#31465,.T.);
#41024=ORIENTED_EDGE('',*,*,#31488,.T.);
#41025=ORIENTED_EDGE('',*,*,#31485,.F.);
#41026=ORIENTED_EDGE('',*,*,#31488,.F.);
#41027=ORIENTED_EDGE('',*,*,#31464,.F.);
#41028=ORIENTED_EDGE('',*,*,#31468,.F.);
#41029=ORIENTED_EDGE('',*,*,#31471,.F.);
#41030=ORIENTED_EDGE('',*,*,#31474,.F.);
#41031=ORIENTED_EDGE('',*,*,#31477,.F.);
#41032=ORIENTED_EDGE('',*,*,#31480,.F.);
#41033=ORIENTED_EDGE('',*,*,#31483,.F.);
#41034=ORIENTED_EDGE('',*,*,#31486,.F.);
#41035=ORIENTED_EDGE('',*,*,#31402,.T.);
#41036=ORIENTED_EDGE('',*,*,#31424,.T.);
#41037=ORIENTED_EDGE('',*,*,#31421,.T.);
#41038=ORIENTED_EDGE('',*,*,#31418,.T.);
#41039=ORIENTED_EDGE('',*,*,#31415,.T.);
#41040=ORIENTED_EDGE('',*,*,#31412,.T.);
#41041=ORIENTED_EDGE('',*,*,#31409,.T.);
#41042=ORIENTED_EDGE('',*,*,#31406,.T.);
#41043=ORIENTED_EDGE('',*,*,#31489,.F.);
#41044=ORIENTED_EDGE('',*,*,#31490,.T.);
#41045=ORIENTED_EDGE('',*,*,#31491,.T.);
#41046=ORIENTED_EDGE('',*,*,#31492,.F.);
#41047=ORIENTED_EDGE('',*,*,#31493,.F.);
#41048=ORIENTED_EDGE('',*,*,#31494,.T.);
#41049=ORIENTED_EDGE('',*,*,#31495,.T.);
#41050=ORIENTED_EDGE('',*,*,#31490,.F.);
#41051=ORIENTED_EDGE('',*,*,#31496,.F.);
#41052=ORIENTED_EDGE('',*,*,#31497,.T.);
#41053=ORIENTED_EDGE('',*,*,#31498,.T.);
#41054=ORIENTED_EDGE('',*,*,#31494,.F.);
#41055=ORIENTED_EDGE('',*,*,#31499,.F.);
#41056=ORIENTED_EDGE('',*,*,#31500,.T.);
#41057=ORIENTED_EDGE('',*,*,#31501,.T.);
#41058=ORIENTED_EDGE('',*,*,#31497,.F.);
#41059=ORIENTED_EDGE('',*,*,#31502,.F.);
#41060=ORIENTED_EDGE('',*,*,#31503,.T.);
#41061=ORIENTED_EDGE('',*,*,#31504,.T.);
#41062=ORIENTED_EDGE('',*,*,#31500,.F.);
#41063=ORIENTED_EDGE('',*,*,#31505,.F.);
#41064=ORIENTED_EDGE('',*,*,#31506,.T.);
#41065=ORIENTED_EDGE('',*,*,#31507,.T.);
#41066=ORIENTED_EDGE('',*,*,#31503,.F.);
#41067=ORIENTED_EDGE('',*,*,#31508,.F.);
#41068=ORIENTED_EDGE('',*,*,#31509,.T.);
#41069=ORIENTED_EDGE('',*,*,#31510,.T.);
#41070=ORIENTED_EDGE('',*,*,#31506,.F.);
#41071=ORIENTED_EDGE('',*,*,#31511,.F.);
#41072=ORIENTED_EDGE('',*,*,#31492,.T.);
#41073=ORIENTED_EDGE('',*,*,#31512,.T.);
#41074=ORIENTED_EDGE('',*,*,#31509,.F.);
#41075=ORIENTED_EDGE('',*,*,#31513,.F.);
#41076=ORIENTED_EDGE('',*,*,#31514,.T.);
#41077=ORIENTED_EDGE('',*,*,#31515,.T.);
#41078=ORIENTED_EDGE('',*,*,#31516,.F.);
#41079=ORIENTED_EDGE('',*,*,#31517,.F.);
#41080=ORIENTED_EDGE('',*,*,#31518,.T.);
#41081=ORIENTED_EDGE('',*,*,#31519,.T.);
#41082=ORIENTED_EDGE('',*,*,#31514,.F.);
#41083=ORIENTED_EDGE('',*,*,#31520,.F.);
#41084=ORIENTED_EDGE('',*,*,#31521,.T.);
#41085=ORIENTED_EDGE('',*,*,#31522,.T.);
#41086=ORIENTED_EDGE('',*,*,#31518,.F.);
#41087=ORIENTED_EDGE('',*,*,#31523,.F.);
#41088=ORIENTED_EDGE('',*,*,#31524,.T.);
#41089=ORIENTED_EDGE('',*,*,#31525,.T.);
#41090=ORIENTED_EDGE('',*,*,#31521,.F.);
#41091=ORIENTED_EDGE('',*,*,#31526,.F.);
#41092=ORIENTED_EDGE('',*,*,#31527,.T.);
#41093=ORIENTED_EDGE('',*,*,#31528,.T.);
#41094=ORIENTED_EDGE('',*,*,#31524,.F.);
#41095=ORIENTED_EDGE('',*,*,#31529,.F.);
#41096=ORIENTED_EDGE('',*,*,#31530,.T.);
#41097=ORIENTED_EDGE('',*,*,#31531,.T.);
#41098=ORIENTED_EDGE('',*,*,#31527,.F.);
#41099=ORIENTED_EDGE('',*,*,#31532,.F.);
#41100=ORIENTED_EDGE('',*,*,#31533,.T.);
#41101=ORIENTED_EDGE('',*,*,#31534,.T.);
#41102=ORIENTED_EDGE('',*,*,#31530,.F.);
#41103=ORIENTED_EDGE('',*,*,#31535,.F.);
#41104=ORIENTED_EDGE('',*,*,#31536,.T.);
#41105=ORIENTED_EDGE('',*,*,#31537,.T.);
#41106=ORIENTED_EDGE('',*,*,#31533,.F.);
#41107=ORIENTED_EDGE('',*,*,#31538,.F.);
#41108=ORIENTED_EDGE('',*,*,#31539,.T.);
#41109=ORIENTED_EDGE('',*,*,#31540,.T.);
#41110=ORIENTED_EDGE('',*,*,#31536,.F.);
#41111=ORIENTED_EDGE('',*,*,#31541,.F.);
#41112=ORIENTED_EDGE('',*,*,#31542,.T.);
#41113=ORIENTED_EDGE('',*,*,#31543,.T.);
#41114=ORIENTED_EDGE('',*,*,#31539,.F.);
#41115=ORIENTED_EDGE('',*,*,#31544,.F.);
#41116=ORIENTED_EDGE('',*,*,#31545,.T.);
#41117=ORIENTED_EDGE('',*,*,#31546,.T.);
#41118=ORIENTED_EDGE('',*,*,#31542,.F.);
#41119=ORIENTED_EDGE('',*,*,#31547,.F.);
#41120=ORIENTED_EDGE('',*,*,#31516,.T.);
#41121=ORIENTED_EDGE('',*,*,#31548,.T.);
#41122=ORIENTED_EDGE('',*,*,#31545,.F.);
#41123=ORIENTED_EDGE('',*,*,#31548,.F.);
#41124=ORIENTED_EDGE('',*,*,#31515,.F.);
#41125=ORIENTED_EDGE('',*,*,#31519,.F.);
#41126=ORIENTED_EDGE('',*,*,#31522,.F.);
#41127=ORIENTED_EDGE('',*,*,#31525,.F.);
#41128=ORIENTED_EDGE('',*,*,#31528,.F.);
#41129=ORIENTED_EDGE('',*,*,#31531,.F.);
#41130=ORIENTED_EDGE('',*,*,#31534,.F.);
#41131=ORIENTED_EDGE('',*,*,#31537,.F.);
#41132=ORIENTED_EDGE('',*,*,#31540,.F.);
#41133=ORIENTED_EDGE('',*,*,#31543,.F.);
#41134=ORIENTED_EDGE('',*,*,#31546,.F.);
#41135=ORIENTED_EDGE('',*,*,#31512,.F.);
#41136=ORIENTED_EDGE('',*,*,#31491,.F.);
#41137=ORIENTED_EDGE('',*,*,#31495,.F.);
#41138=ORIENTED_EDGE('',*,*,#31498,.F.);
#41139=ORIENTED_EDGE('',*,*,#31501,.F.);
#41140=ORIENTED_EDGE('',*,*,#31504,.F.);
#41141=ORIENTED_EDGE('',*,*,#31507,.F.);
#41142=ORIENTED_EDGE('',*,*,#31510,.F.);
#41143=ORIENTED_EDGE('',*,*,#31489,.T.);
#41144=ORIENTED_EDGE('',*,*,#31511,.T.);
#41145=ORIENTED_EDGE('',*,*,#31508,.T.);
#41146=ORIENTED_EDGE('',*,*,#31505,.T.);
#41147=ORIENTED_EDGE('',*,*,#31502,.T.);
#41148=ORIENTED_EDGE('',*,*,#31499,.T.);
#41149=ORIENTED_EDGE('',*,*,#31496,.T.);
#41150=ORIENTED_EDGE('',*,*,#31493,.T.);
#41151=ORIENTED_EDGE('',*,*,#31549,.F.);
#41152=ORIENTED_EDGE('',*,*,#31550,.T.);
#41153=ORIENTED_EDGE('',*,*,#31551,.T.);
#41154=ORIENTED_EDGE('',*,*,#31552,.F.);
#41155=ORIENTED_EDGE('',*,*,#31553,.F.);
#41156=ORIENTED_EDGE('',*,*,#31554,.T.);
#41157=ORIENTED_EDGE('',*,*,#31555,.T.);
#41158=ORIENTED_EDGE('',*,*,#31550,.F.);
#41159=ORIENTED_EDGE('',*,*,#31556,.F.);
#41160=ORIENTED_EDGE('',*,*,#31557,.T.);
#41161=ORIENTED_EDGE('',*,*,#31558,.T.);
#41162=ORIENTED_EDGE('',*,*,#31554,.F.);
#41163=ORIENTED_EDGE('',*,*,#31559,.F.);
#41164=ORIENTED_EDGE('',*,*,#31560,.T.);
#41165=ORIENTED_EDGE('',*,*,#31561,.T.);
#41166=ORIENTED_EDGE('',*,*,#31557,.F.);
#41167=ORIENTED_EDGE('',*,*,#31562,.F.);
#41168=ORIENTED_EDGE('',*,*,#31563,.T.);
#41169=ORIENTED_EDGE('',*,*,#31564,.T.);
#41170=ORIENTED_EDGE('',*,*,#31560,.F.);
#41171=ORIENTED_EDGE('',*,*,#31565,.F.);
#41172=ORIENTED_EDGE('',*,*,#31566,.T.);
#41173=ORIENTED_EDGE('',*,*,#31567,.T.);
#41174=ORIENTED_EDGE('',*,*,#31563,.F.);
#41175=ORIENTED_EDGE('',*,*,#31568,.F.);
#41176=ORIENTED_EDGE('',*,*,#31569,.T.);
#41177=ORIENTED_EDGE('',*,*,#31570,.T.);
#41178=ORIENTED_EDGE('',*,*,#31566,.F.);
#41179=ORIENTED_EDGE('',*,*,#31571,.F.);
#41180=ORIENTED_EDGE('',*,*,#31552,.T.);
#41181=ORIENTED_EDGE('',*,*,#31572,.T.);
#41182=ORIENTED_EDGE('',*,*,#31569,.F.);
#41183=ORIENTED_EDGE('',*,*,#31573,.F.);
#41184=ORIENTED_EDGE('',*,*,#31574,.T.);
#41185=ORIENTED_EDGE('',*,*,#31575,.T.);
#41186=ORIENTED_EDGE('',*,*,#31576,.F.);
#41187=ORIENTED_EDGE('',*,*,#31577,.F.);
#41188=ORIENTED_EDGE('',*,*,#31578,.T.);
#41189=ORIENTED_EDGE('',*,*,#31579,.T.);
#41190=ORIENTED_EDGE('',*,*,#31574,.F.);
#41191=ORIENTED_EDGE('',*,*,#31580,.F.);
#41192=ORIENTED_EDGE('',*,*,#31581,.T.);
#41193=ORIENTED_EDGE('',*,*,#31582,.T.);
#41194=ORIENTED_EDGE('',*,*,#31578,.F.);
#41195=ORIENTED_EDGE('',*,*,#31583,.F.);
#41196=ORIENTED_EDGE('',*,*,#31584,.T.);
#41197=ORIENTED_EDGE('',*,*,#31585,.T.);
#41198=ORIENTED_EDGE('',*,*,#31581,.F.);
#41199=ORIENTED_EDGE('',*,*,#31586,.F.);
#41200=ORIENTED_EDGE('',*,*,#31587,.T.);
#41201=ORIENTED_EDGE('',*,*,#31588,.T.);
#41202=ORIENTED_EDGE('',*,*,#31584,.F.);
#41203=ORIENTED_EDGE('',*,*,#31589,.F.);
#41204=ORIENTED_EDGE('',*,*,#31590,.T.);
#41205=ORIENTED_EDGE('',*,*,#31591,.T.);
#41206=ORIENTED_EDGE('',*,*,#31587,.F.);
#41207=ORIENTED_EDGE('',*,*,#31592,.F.);
#41208=ORIENTED_EDGE('',*,*,#31593,.T.);
#41209=ORIENTED_EDGE('',*,*,#31594,.T.);
#41210=ORIENTED_EDGE('',*,*,#31590,.F.);
#41211=ORIENTED_EDGE('',*,*,#31595,.F.);
#41212=ORIENTED_EDGE('',*,*,#31596,.T.);
#41213=ORIENTED_EDGE('',*,*,#31597,.T.);
#41214=ORIENTED_EDGE('',*,*,#31593,.F.);
#41215=ORIENTED_EDGE('',*,*,#31598,.F.);
#41216=ORIENTED_EDGE('',*,*,#31599,.T.);
#41217=ORIENTED_EDGE('',*,*,#31600,.T.);
#41218=ORIENTED_EDGE('',*,*,#31596,.F.);
#41219=ORIENTED_EDGE('',*,*,#31601,.F.);
#41220=ORIENTED_EDGE('',*,*,#31602,.T.);
#41221=ORIENTED_EDGE('',*,*,#31603,.T.);
#41222=ORIENTED_EDGE('',*,*,#31599,.F.);
#41223=ORIENTED_EDGE('',*,*,#31604,.F.);
#41224=ORIENTED_EDGE('',*,*,#31605,.T.);
#41225=ORIENTED_EDGE('',*,*,#31606,.T.);
#41226=ORIENTED_EDGE('',*,*,#31602,.F.);
#41227=ORIENTED_EDGE('',*,*,#31607,.F.);
#41228=ORIENTED_EDGE('',*,*,#31576,.T.);
#41229=ORIENTED_EDGE('',*,*,#31608,.T.);
#41230=ORIENTED_EDGE('',*,*,#31605,.F.);
#41231=ORIENTED_EDGE('',*,*,#31608,.F.);
#41232=ORIENTED_EDGE('',*,*,#31575,.F.);
#41233=ORIENTED_EDGE('',*,*,#31579,.F.);
#41234=ORIENTED_EDGE('',*,*,#31582,.F.);
#41235=ORIENTED_EDGE('',*,*,#31585,.F.);
#41236=ORIENTED_EDGE('',*,*,#31588,.F.);
#41237=ORIENTED_EDGE('',*,*,#31591,.F.);
#41238=ORIENTED_EDGE('',*,*,#31594,.F.);
#41239=ORIENTED_EDGE('',*,*,#31597,.F.);
#41240=ORIENTED_EDGE('',*,*,#31600,.F.);
#41241=ORIENTED_EDGE('',*,*,#31603,.F.);
#41242=ORIENTED_EDGE('',*,*,#31606,.F.);
#41243=ORIENTED_EDGE('',*,*,#31572,.F.);
#41244=ORIENTED_EDGE('',*,*,#31551,.F.);
#41245=ORIENTED_EDGE('',*,*,#31555,.F.);
#41246=ORIENTED_EDGE('',*,*,#31558,.F.);
#41247=ORIENTED_EDGE('',*,*,#31561,.F.);
#41248=ORIENTED_EDGE('',*,*,#31564,.F.);
#41249=ORIENTED_EDGE('',*,*,#31567,.F.);
#41250=ORIENTED_EDGE('',*,*,#31570,.F.);
#41251=ORIENTED_EDGE('',*,*,#31609,.F.);
#41252=ORIENTED_EDGE('',*,*,#31610,.T.);
#41253=ORIENTED_EDGE('',*,*,#31611,.T.);
#41254=ORIENTED_EDGE('',*,*,#31612,.F.);
#41255=ORIENTED_EDGE('',*,*,#31613,.F.);
#41256=ORIENTED_EDGE('',*,*,#31614,.T.);
#41257=ORIENTED_EDGE('',*,*,#31615,.T.);
#41258=ORIENTED_EDGE('',*,*,#31610,.F.);
#41259=ORIENTED_EDGE('',*,*,#31616,.F.);
#41260=ORIENTED_EDGE('',*,*,#31617,.T.);
#41261=ORIENTED_EDGE('',*,*,#31618,.T.);
#41262=ORIENTED_EDGE('',*,*,#31614,.F.);
#41263=ORIENTED_EDGE('',*,*,#31619,.F.);
#41264=ORIENTED_EDGE('',*,*,#31620,.T.);
#41265=ORIENTED_EDGE('',*,*,#31621,.T.);
#41266=ORIENTED_EDGE('',*,*,#31617,.F.);
#41267=ORIENTED_EDGE('',*,*,#31622,.F.);
#41268=ORIENTED_EDGE('',*,*,#31623,.T.);
#41269=ORIENTED_EDGE('',*,*,#31624,.T.);
#41270=ORIENTED_EDGE('',*,*,#31620,.F.);
#41271=ORIENTED_EDGE('',*,*,#31625,.F.);
#41272=ORIENTED_EDGE('',*,*,#31626,.T.);
#41273=ORIENTED_EDGE('',*,*,#31627,.T.);
#41274=ORIENTED_EDGE('',*,*,#31623,.F.);
#41275=ORIENTED_EDGE('',*,*,#31628,.F.);
#41276=ORIENTED_EDGE('',*,*,#31629,.T.);
#41277=ORIENTED_EDGE('',*,*,#31630,.T.);
#41278=ORIENTED_EDGE('',*,*,#31626,.F.);
#41279=ORIENTED_EDGE('',*,*,#31631,.F.);
#41280=ORIENTED_EDGE('',*,*,#31632,.T.);
#41281=ORIENTED_EDGE('',*,*,#31633,.T.);
#41282=ORIENTED_EDGE('',*,*,#31629,.F.);
#41283=ORIENTED_EDGE('',*,*,#31634,.F.);
#41284=ORIENTED_EDGE('',*,*,#31612,.T.);
#41285=ORIENTED_EDGE('',*,*,#31635,.T.);
#41286=ORIENTED_EDGE('',*,*,#31632,.F.);
#41287=ORIENTED_EDGE('',*,*,#31635,.F.);
#41288=ORIENTED_EDGE('',*,*,#31611,.F.);
#41289=ORIENTED_EDGE('',*,*,#31615,.F.);
#41290=ORIENTED_EDGE('',*,*,#31618,.F.);
#41291=ORIENTED_EDGE('',*,*,#31621,.F.);
#41292=ORIENTED_EDGE('',*,*,#31624,.F.);
#41293=ORIENTED_EDGE('',*,*,#31627,.F.);
#41294=ORIENTED_EDGE('',*,*,#31630,.F.);
#41295=ORIENTED_EDGE('',*,*,#31633,.F.);
#41296=ORIENTED_EDGE('',*,*,#31549,.T.);
#41297=ORIENTED_EDGE('',*,*,#31571,.T.);
#41298=ORIENTED_EDGE('',*,*,#31568,.T.);
#41299=ORIENTED_EDGE('',*,*,#31565,.T.);
#41300=ORIENTED_EDGE('',*,*,#31562,.T.);
#41301=ORIENTED_EDGE('',*,*,#31559,.T.);
#41302=ORIENTED_EDGE('',*,*,#31556,.T.);
#41303=ORIENTED_EDGE('',*,*,#31553,.T.);
#41304=ORIENTED_EDGE('',*,*,#31636,.F.);
#41305=ORIENTED_EDGE('',*,*,#31637,.T.);
#41306=ORIENTED_EDGE('',*,*,#31638,.T.);
#41307=ORIENTED_EDGE('',*,*,#31639,.F.);
#41308=ORIENTED_EDGE('',*,*,#31640,.F.);
#41309=ORIENTED_EDGE('',*,*,#31641,.T.);
#41310=ORIENTED_EDGE('',*,*,#31642,.T.);
#41311=ORIENTED_EDGE('',*,*,#31637,.F.);
#41312=ORIENTED_EDGE('',*,*,#31643,.F.);
#41313=ORIENTED_EDGE('',*,*,#31644,.T.);
#41314=ORIENTED_EDGE('',*,*,#31645,.T.);
#41315=ORIENTED_EDGE('',*,*,#31641,.F.);
#41316=ORIENTED_EDGE('',*,*,#31646,.F.);
#41317=ORIENTED_EDGE('',*,*,#31647,.T.);
#41318=ORIENTED_EDGE('',*,*,#31648,.T.);
#41319=ORIENTED_EDGE('',*,*,#31644,.F.);
#41320=ORIENTED_EDGE('',*,*,#31649,.F.);
#41321=ORIENTED_EDGE('',*,*,#31650,.T.);
#41322=ORIENTED_EDGE('',*,*,#31651,.T.);
#41323=ORIENTED_EDGE('',*,*,#31647,.F.);
#41324=ORIENTED_EDGE('',*,*,#31652,.F.);
#41325=ORIENTED_EDGE('',*,*,#31653,.T.);
#41326=ORIENTED_EDGE('',*,*,#31654,.T.);
#41327=ORIENTED_EDGE('',*,*,#31650,.F.);
#41328=ORIENTED_EDGE('',*,*,#31655,.F.);
#41329=ORIENTED_EDGE('',*,*,#31656,.T.);
#41330=ORIENTED_EDGE('',*,*,#31657,.T.);
#41331=ORIENTED_EDGE('',*,*,#31653,.F.);
#41332=ORIENTED_EDGE('',*,*,#31658,.F.);
#41333=ORIENTED_EDGE('',*,*,#31639,.T.);
#41334=ORIENTED_EDGE('',*,*,#31659,.T.);
#41335=ORIENTED_EDGE('',*,*,#31656,.F.);
#41336=ORIENTED_EDGE('',*,*,#31660,.F.);
#41337=ORIENTED_EDGE('',*,*,#31661,.T.);
#41338=ORIENTED_EDGE('',*,*,#31662,.T.);
#41339=ORIENTED_EDGE('',*,*,#31663,.F.);
#41340=ORIENTED_EDGE('',*,*,#31664,.F.);
#41341=ORIENTED_EDGE('',*,*,#31665,.T.);
#41342=ORIENTED_EDGE('',*,*,#31666,.T.);
#41343=ORIENTED_EDGE('',*,*,#31661,.F.);
#41344=ORIENTED_EDGE('',*,*,#31667,.F.);
#41345=ORIENTED_EDGE('',*,*,#31668,.T.);
#41346=ORIENTED_EDGE('',*,*,#31669,.T.);
#41347=ORIENTED_EDGE('',*,*,#31665,.F.);
#41348=ORIENTED_EDGE('',*,*,#31670,.F.);
#41349=ORIENTED_EDGE('',*,*,#31671,.T.);
#41350=ORIENTED_EDGE('',*,*,#31672,.T.);
#41351=ORIENTED_EDGE('',*,*,#31668,.F.);
#41352=ORIENTED_EDGE('',*,*,#31673,.F.);
#41353=ORIENTED_EDGE('',*,*,#31674,.T.);
#41354=ORIENTED_EDGE('',*,*,#31675,.T.);
#41355=ORIENTED_EDGE('',*,*,#31671,.F.);
#41356=ORIENTED_EDGE('',*,*,#31676,.F.);
#41357=ORIENTED_EDGE('',*,*,#31677,.T.);
#41358=ORIENTED_EDGE('',*,*,#31678,.T.);
#41359=ORIENTED_EDGE('',*,*,#31674,.F.);
#41360=ORIENTED_EDGE('',*,*,#31679,.F.);
#41361=ORIENTED_EDGE('',*,*,#31680,.T.);
#41362=ORIENTED_EDGE('',*,*,#31681,.T.);
#41363=ORIENTED_EDGE('',*,*,#31677,.F.);
#41364=ORIENTED_EDGE('',*,*,#31682,.F.);
#41365=ORIENTED_EDGE('',*,*,#31683,.T.);
#41366=ORIENTED_EDGE('',*,*,#31684,.T.);
#41367=ORIENTED_EDGE('',*,*,#31680,.F.);
#41368=ORIENTED_EDGE('',*,*,#31685,.F.);
#41369=ORIENTED_EDGE('',*,*,#31686,.T.);
#41370=ORIENTED_EDGE('',*,*,#31687,.T.);
#41371=ORIENTED_EDGE('',*,*,#31683,.F.);
#41372=ORIENTED_EDGE('',*,*,#31688,.F.);
#41373=ORIENTED_EDGE('',*,*,#31689,.T.);
#41374=ORIENTED_EDGE('',*,*,#31690,.T.);
#41375=ORIENTED_EDGE('',*,*,#31686,.F.);
#41376=ORIENTED_EDGE('',*,*,#31691,.F.);
#41377=ORIENTED_EDGE('',*,*,#31692,.T.);
#41378=ORIENTED_EDGE('',*,*,#31693,.T.);
#41379=ORIENTED_EDGE('',*,*,#31689,.F.);
#41380=ORIENTED_EDGE('',*,*,#31694,.F.);
#41381=ORIENTED_EDGE('',*,*,#31663,.T.);
#41382=ORIENTED_EDGE('',*,*,#31695,.T.);
#41383=ORIENTED_EDGE('',*,*,#31692,.F.);
#41384=ORIENTED_EDGE('',*,*,#31695,.F.);
#41385=ORIENTED_EDGE('',*,*,#31662,.F.);
#41386=ORIENTED_EDGE('',*,*,#31666,.F.);
#41387=ORIENTED_EDGE('',*,*,#31669,.F.);
#41388=ORIENTED_EDGE('',*,*,#31672,.F.);
#41389=ORIENTED_EDGE('',*,*,#31675,.F.);
#41390=ORIENTED_EDGE('',*,*,#31678,.F.);
#41391=ORIENTED_EDGE('',*,*,#31681,.F.);
#41392=ORIENTED_EDGE('',*,*,#31684,.F.);
#41393=ORIENTED_EDGE('',*,*,#31687,.F.);
#41394=ORIENTED_EDGE('',*,*,#31690,.F.);
#41395=ORIENTED_EDGE('',*,*,#31693,.F.);
#41396=ORIENTED_EDGE('',*,*,#31659,.F.);
#41397=ORIENTED_EDGE('',*,*,#31638,.F.);
#41398=ORIENTED_EDGE('',*,*,#31642,.F.);
#41399=ORIENTED_EDGE('',*,*,#31645,.F.);
#41400=ORIENTED_EDGE('',*,*,#31648,.F.);
#41401=ORIENTED_EDGE('',*,*,#31651,.F.);
#41402=ORIENTED_EDGE('',*,*,#31654,.F.);
#41403=ORIENTED_EDGE('',*,*,#31657,.F.);
#41404=ORIENTED_EDGE('',*,*,#31696,.F.);
#41405=ORIENTED_EDGE('',*,*,#31697,.T.);
#41406=ORIENTED_EDGE('',*,*,#31698,.T.);
#41407=ORIENTED_EDGE('',*,*,#31699,.F.);
#41408=ORIENTED_EDGE('',*,*,#31700,.F.);
#41409=ORIENTED_EDGE('',*,*,#31701,.T.);
#41410=ORIENTED_EDGE('',*,*,#31702,.T.);
#41411=ORIENTED_EDGE('',*,*,#31697,.F.);
#41412=ORIENTED_EDGE('',*,*,#31703,.F.);
#41413=ORIENTED_EDGE('',*,*,#31704,.T.);
#41414=ORIENTED_EDGE('',*,*,#31705,.T.);
#41415=ORIENTED_EDGE('',*,*,#31701,.F.);
#41416=ORIENTED_EDGE('',*,*,#31706,.F.);
#41417=ORIENTED_EDGE('',*,*,#31707,.T.);
#41418=ORIENTED_EDGE('',*,*,#31708,.T.);
#41419=ORIENTED_EDGE('',*,*,#31704,.F.);
#41420=ORIENTED_EDGE('',*,*,#31709,.F.);
#41421=ORIENTED_EDGE('',*,*,#31710,.T.);
#41422=ORIENTED_EDGE('',*,*,#31711,.T.);
#41423=ORIENTED_EDGE('',*,*,#31707,.F.);
#41424=ORIENTED_EDGE('',*,*,#31712,.F.);
#41425=ORIENTED_EDGE('',*,*,#31713,.T.);
#41426=ORIENTED_EDGE('',*,*,#31714,.T.);
#41427=ORIENTED_EDGE('',*,*,#31710,.F.);
#41428=ORIENTED_EDGE('',*,*,#31715,.F.);
#41429=ORIENTED_EDGE('',*,*,#31716,.T.);
#41430=ORIENTED_EDGE('',*,*,#31717,.T.);
#41431=ORIENTED_EDGE('',*,*,#31713,.F.);
#41432=ORIENTED_EDGE('',*,*,#31718,.F.);
#41433=ORIENTED_EDGE('',*,*,#31719,.T.);
#41434=ORIENTED_EDGE('',*,*,#31720,.T.);
#41435=ORIENTED_EDGE('',*,*,#31716,.F.);
#41436=ORIENTED_EDGE('',*,*,#31721,.F.);
#41437=ORIENTED_EDGE('',*,*,#31722,.T.);
#41438=ORIENTED_EDGE('',*,*,#31723,.T.);
#41439=ORIENTED_EDGE('',*,*,#31719,.F.);
#41440=ORIENTED_EDGE('',*,*,#31724,.F.);
#41441=ORIENTED_EDGE('',*,*,#31725,.T.);
#41442=ORIENTED_EDGE('',*,*,#31726,.T.);
#41443=ORIENTED_EDGE('',*,*,#31722,.F.);
#41444=ORIENTED_EDGE('',*,*,#31727,.F.);
#41445=ORIENTED_EDGE('',*,*,#31728,.T.);
#41446=ORIENTED_EDGE('',*,*,#31729,.T.);
#41447=ORIENTED_EDGE('',*,*,#31725,.F.);
#41448=ORIENTED_EDGE('',*,*,#31730,.F.);
#41449=ORIENTED_EDGE('',*,*,#31731,.T.);
#41450=ORIENTED_EDGE('',*,*,#31732,.T.);
#41451=ORIENTED_EDGE('',*,*,#31728,.F.);
#41452=ORIENTED_EDGE('',*,*,#31733,.F.);
#41453=ORIENTED_EDGE('',*,*,#31734,.T.);
#41454=ORIENTED_EDGE('',*,*,#31735,.T.);
#41455=ORIENTED_EDGE('',*,*,#31731,.F.);
#41456=ORIENTED_EDGE('',*,*,#31736,.F.);
#41457=ORIENTED_EDGE('',*,*,#31737,.T.);
#41458=ORIENTED_EDGE('',*,*,#31738,.T.);
#41459=ORIENTED_EDGE('',*,*,#31734,.F.);
#41460=ORIENTED_EDGE('',*,*,#31739,.F.);
#41461=ORIENTED_EDGE('',*,*,#31740,.T.);
#41462=ORIENTED_EDGE('',*,*,#31741,.T.);
#41463=ORIENTED_EDGE('',*,*,#31737,.F.);
#41464=ORIENTED_EDGE('',*,*,#31742,.F.);
#41465=ORIENTED_EDGE('',*,*,#31743,.T.);
#41466=ORIENTED_EDGE('',*,*,#31744,.T.);
#41467=ORIENTED_EDGE('',*,*,#31740,.F.);
#41468=ORIENTED_EDGE('',*,*,#31745,.F.);
#41469=ORIENTED_EDGE('',*,*,#31746,.T.);
#41470=ORIENTED_EDGE('',*,*,#31747,.T.);
#41471=ORIENTED_EDGE('',*,*,#31743,.F.);
#41472=ORIENTED_EDGE('',*,*,#31748,.F.);
#41473=ORIENTED_EDGE('',*,*,#31749,.T.);
#41474=ORIENTED_EDGE('',*,*,#31750,.T.);
#41475=ORIENTED_EDGE('',*,*,#31746,.F.);
#41476=ORIENTED_EDGE('',*,*,#31751,.F.);
#41477=ORIENTED_EDGE('',*,*,#31752,.T.);
#41478=ORIENTED_EDGE('',*,*,#31753,.T.);
#41479=ORIENTED_EDGE('',*,*,#31749,.F.);
#41480=ORIENTED_EDGE('',*,*,#31754,.F.);
#41481=ORIENTED_EDGE('',*,*,#31755,.T.);
#41482=ORIENTED_EDGE('',*,*,#31756,.T.);
#41483=ORIENTED_EDGE('',*,*,#31752,.F.);
#41484=ORIENTED_EDGE('',*,*,#31757,.F.);
#41485=ORIENTED_EDGE('',*,*,#31758,.T.);
#41486=ORIENTED_EDGE('',*,*,#31759,.T.);
#41487=ORIENTED_EDGE('',*,*,#31755,.F.);
#41488=ORIENTED_EDGE('',*,*,#31760,.F.);
#41489=ORIENTED_EDGE('',*,*,#31699,.T.);
#41490=ORIENTED_EDGE('',*,*,#31761,.T.);
#41491=ORIENTED_EDGE('',*,*,#31758,.F.);
#41492=ORIENTED_EDGE('',*,*,#31761,.F.);
#41493=ORIENTED_EDGE('',*,*,#31698,.F.);
#41494=ORIENTED_EDGE('',*,*,#31702,.F.);
#41495=ORIENTED_EDGE('',*,*,#31705,.F.);
#41496=ORIENTED_EDGE('',*,*,#31708,.F.);
#41497=ORIENTED_EDGE('',*,*,#31711,.F.);
#41498=ORIENTED_EDGE('',*,*,#31714,.F.);
#41499=ORIENTED_EDGE('',*,*,#31717,.F.);
#41500=ORIENTED_EDGE('',*,*,#31720,.F.);
#41501=ORIENTED_EDGE('',*,*,#31723,.F.);
#41502=ORIENTED_EDGE('',*,*,#31726,.F.);
#41503=ORIENTED_EDGE('',*,*,#31729,.F.);
#41504=ORIENTED_EDGE('',*,*,#31732,.F.);
#41505=ORIENTED_EDGE('',*,*,#31735,.F.);
#41506=ORIENTED_EDGE('',*,*,#31738,.F.);
#41507=ORIENTED_EDGE('',*,*,#31741,.F.);
#41508=ORIENTED_EDGE('',*,*,#31744,.F.);
#41509=ORIENTED_EDGE('',*,*,#31747,.F.);
#41510=ORIENTED_EDGE('',*,*,#31750,.F.);
#41511=ORIENTED_EDGE('',*,*,#31753,.F.);
#41512=ORIENTED_EDGE('',*,*,#31756,.F.);
#41513=ORIENTED_EDGE('',*,*,#31759,.F.);
#41514=ORIENTED_EDGE('',*,*,#31636,.T.);
#41515=ORIENTED_EDGE('',*,*,#31658,.T.);
#41516=ORIENTED_EDGE('',*,*,#31655,.T.);
#41517=ORIENTED_EDGE('',*,*,#31652,.T.);
#41518=ORIENTED_EDGE('',*,*,#31649,.T.);
#41519=ORIENTED_EDGE('',*,*,#31646,.T.);
#41520=ORIENTED_EDGE('',*,*,#31643,.T.);
#41521=ORIENTED_EDGE('',*,*,#31640,.T.);
#41522=ORIENTED_EDGE('',*,*,#31762,.F.);
#41523=ORIENTED_EDGE('',*,*,#31763,.T.);
#41524=ORIENTED_EDGE('',*,*,#31764,.T.);
#41525=ORIENTED_EDGE('',*,*,#31765,.F.);
#41526=ORIENTED_EDGE('',*,*,#31766,.F.);
#41527=ORIENTED_EDGE('',*,*,#31767,.T.);
#41528=ORIENTED_EDGE('',*,*,#31768,.T.);
#41529=ORIENTED_EDGE('',*,*,#31763,.F.);
#41530=ORIENTED_EDGE('',*,*,#31769,.F.);
#41531=ORIENTED_EDGE('',*,*,#31770,.T.);
#41532=ORIENTED_EDGE('',*,*,#31771,.T.);
#41533=ORIENTED_EDGE('',*,*,#31767,.F.);
#41534=ORIENTED_EDGE('',*,*,#31772,.F.);
#41535=ORIENTED_EDGE('',*,*,#31773,.T.);
#41536=ORIENTED_EDGE('',*,*,#31774,.T.);
#41537=ORIENTED_EDGE('',*,*,#31770,.F.);
#41538=ORIENTED_EDGE('',*,*,#31775,.F.);
#41539=ORIENTED_EDGE('',*,*,#31776,.T.);
#41540=ORIENTED_EDGE('',*,*,#31777,.T.);
#41541=ORIENTED_EDGE('',*,*,#31773,.F.);
#41542=ORIENTED_EDGE('',*,*,#31778,.F.);
#41543=ORIENTED_EDGE('',*,*,#31779,.T.);
#41544=ORIENTED_EDGE('',*,*,#31780,.T.);
#41545=ORIENTED_EDGE('',*,*,#31776,.F.);
#41546=ORIENTED_EDGE('',*,*,#31781,.F.);
#41547=ORIENTED_EDGE('',*,*,#31782,.T.);
#41548=ORIENTED_EDGE('',*,*,#31783,.T.);
#41549=ORIENTED_EDGE('',*,*,#31779,.F.);
#41550=ORIENTED_EDGE('',*,*,#31784,.F.);
#41551=ORIENTED_EDGE('',*,*,#31765,.T.);
#41552=ORIENTED_EDGE('',*,*,#31785,.T.);
#41553=ORIENTED_EDGE('',*,*,#31782,.F.);
#41554=ORIENTED_EDGE('',*,*,#31786,.F.);
#41555=ORIENTED_EDGE('',*,*,#31787,.T.);
#41556=ORIENTED_EDGE('',*,*,#31788,.T.);
#41557=ORIENTED_EDGE('',*,*,#31789,.F.);
#41558=ORIENTED_EDGE('',*,*,#31790,.F.);
#41559=ORIENTED_EDGE('',*,*,#31791,.T.);
#41560=ORIENTED_EDGE('',*,*,#31792,.T.);
#41561=ORIENTED_EDGE('',*,*,#31787,.F.);
#41562=ORIENTED_EDGE('',*,*,#31793,.F.);
#41563=ORIENTED_EDGE('',*,*,#31794,.T.);
#41564=ORIENTED_EDGE('',*,*,#31795,.T.);
#41565=ORIENTED_EDGE('',*,*,#31791,.F.);
#41566=ORIENTED_EDGE('',*,*,#31796,.F.);
#41567=ORIENTED_EDGE('',*,*,#31797,.T.);
#41568=ORIENTED_EDGE('',*,*,#31798,.T.);
#41569=ORIENTED_EDGE('',*,*,#31794,.F.);
#41570=ORIENTED_EDGE('',*,*,#31799,.F.);
#41571=ORIENTED_EDGE('',*,*,#31800,.T.);
#41572=ORIENTED_EDGE('',*,*,#31801,.T.);
#41573=ORIENTED_EDGE('',*,*,#31797,.F.);
#41574=ORIENTED_EDGE('',*,*,#31802,.F.);
#41575=ORIENTED_EDGE('',*,*,#31803,.T.);
#41576=ORIENTED_EDGE('',*,*,#31804,.T.);
#41577=ORIENTED_EDGE('',*,*,#31800,.F.);
#41578=ORIENTED_EDGE('',*,*,#31805,.F.);
#41579=ORIENTED_EDGE('',*,*,#31806,.T.);
#41580=ORIENTED_EDGE('',*,*,#31807,.T.);
#41581=ORIENTED_EDGE('',*,*,#31803,.F.);
#41582=ORIENTED_EDGE('',*,*,#31808,.F.);
#41583=ORIENTED_EDGE('',*,*,#31809,.T.);
#41584=ORIENTED_EDGE('',*,*,#31810,.T.);
#41585=ORIENTED_EDGE('',*,*,#31806,.F.);
#41586=ORIENTED_EDGE('',*,*,#31811,.F.);
#41587=ORIENTED_EDGE('',*,*,#31812,.T.);
#41588=ORIENTED_EDGE('',*,*,#31813,.T.);
#41589=ORIENTED_EDGE('',*,*,#31809,.F.);
#41590=ORIENTED_EDGE('',*,*,#31814,.F.);
#41591=ORIENTED_EDGE('',*,*,#31815,.T.);
#41592=ORIENTED_EDGE('',*,*,#31816,.T.);
#41593=ORIENTED_EDGE('',*,*,#31812,.F.);
#41594=ORIENTED_EDGE('',*,*,#31817,.F.);
#41595=ORIENTED_EDGE('',*,*,#31818,.T.);
#41596=ORIENTED_EDGE('',*,*,#31819,.T.);
#41597=ORIENTED_EDGE('',*,*,#31815,.F.);
#41598=ORIENTED_EDGE('',*,*,#31820,.F.);
#41599=ORIENTED_EDGE('',*,*,#31789,.T.);
#41600=ORIENTED_EDGE('',*,*,#31821,.T.);
#41601=ORIENTED_EDGE('',*,*,#31818,.F.);
#41602=ORIENTED_EDGE('',*,*,#31821,.F.);
#41603=ORIENTED_EDGE('',*,*,#31788,.F.);
#41604=ORIENTED_EDGE('',*,*,#31792,.F.);
#41605=ORIENTED_EDGE('',*,*,#31795,.F.);
#41606=ORIENTED_EDGE('',*,*,#31798,.F.);
#41607=ORIENTED_EDGE('',*,*,#31801,.F.);
#41608=ORIENTED_EDGE('',*,*,#31804,.F.);
#41609=ORIENTED_EDGE('',*,*,#31807,.F.);
#41610=ORIENTED_EDGE('',*,*,#31810,.F.);
#41611=ORIENTED_EDGE('',*,*,#31813,.F.);
#41612=ORIENTED_EDGE('',*,*,#31816,.F.);
#41613=ORIENTED_EDGE('',*,*,#31819,.F.);
#41614=ORIENTED_EDGE('',*,*,#31785,.F.);
#41615=ORIENTED_EDGE('',*,*,#31764,.F.);
#41616=ORIENTED_EDGE('',*,*,#31768,.F.);
#41617=ORIENTED_EDGE('',*,*,#31771,.F.);
#41618=ORIENTED_EDGE('',*,*,#31774,.F.);
#41619=ORIENTED_EDGE('',*,*,#31777,.F.);
#41620=ORIENTED_EDGE('',*,*,#31780,.F.);
#41621=ORIENTED_EDGE('',*,*,#31783,.F.);
#41622=ORIENTED_EDGE('',*,*,#31822,.F.);
#41623=ORIENTED_EDGE('',*,*,#31823,.T.);
#41624=ORIENTED_EDGE('',*,*,#31824,.T.);
#41625=ORIENTED_EDGE('',*,*,#31825,.F.);
#41626=ORIENTED_EDGE('',*,*,#31826,.F.);
#41627=ORIENTED_EDGE('',*,*,#31827,.T.);
#41628=ORIENTED_EDGE('',*,*,#31828,.T.);
#41629=ORIENTED_EDGE('',*,*,#31823,.F.);
#41630=ORIENTED_EDGE('',*,*,#31829,.F.);
#41631=ORIENTED_EDGE('',*,*,#31830,.T.);
#41632=ORIENTED_EDGE('',*,*,#31831,.T.);
#41633=ORIENTED_EDGE('',*,*,#31827,.F.);
#41634=ORIENTED_EDGE('',*,*,#31832,.F.);
#41635=ORIENTED_EDGE('',*,*,#31833,.T.);
#41636=ORIENTED_EDGE('',*,*,#31834,.T.);
#41637=ORIENTED_EDGE('',*,*,#31830,.F.);
#41638=ORIENTED_EDGE('',*,*,#31835,.F.);
#41639=ORIENTED_EDGE('',*,*,#31836,.T.);
#41640=ORIENTED_EDGE('',*,*,#31837,.T.);
#41641=ORIENTED_EDGE('',*,*,#31833,.F.);
#41642=ORIENTED_EDGE('',*,*,#31838,.F.);
#41643=ORIENTED_EDGE('',*,*,#31839,.T.);
#41644=ORIENTED_EDGE('',*,*,#31840,.T.);
#41645=ORIENTED_EDGE('',*,*,#31836,.F.);
#41646=ORIENTED_EDGE('',*,*,#31841,.F.);
#41647=ORIENTED_EDGE('',*,*,#31842,.T.);
#41648=ORIENTED_EDGE('',*,*,#31843,.T.);
#41649=ORIENTED_EDGE('',*,*,#31839,.F.);
#41650=ORIENTED_EDGE('',*,*,#31844,.F.);
#41651=ORIENTED_EDGE('',*,*,#31845,.T.);
#41652=ORIENTED_EDGE('',*,*,#31846,.T.);
#41653=ORIENTED_EDGE('',*,*,#31842,.F.);
#41654=ORIENTED_EDGE('',*,*,#31847,.F.);
#41655=ORIENTED_EDGE('',*,*,#31848,.T.);
#41656=ORIENTED_EDGE('',*,*,#31849,.T.);
#41657=ORIENTED_EDGE('',*,*,#31845,.F.);
#41658=ORIENTED_EDGE('',*,*,#31850,.F.);
#41659=ORIENTED_EDGE('',*,*,#31851,.T.);
#41660=ORIENTED_EDGE('',*,*,#31852,.T.);
#41661=ORIENTED_EDGE('',*,*,#31848,.F.);
#41662=ORIENTED_EDGE('',*,*,#31853,.F.);
#41663=ORIENTED_EDGE('',*,*,#31854,.T.);
#41664=ORIENTED_EDGE('',*,*,#31855,.T.);
#41665=ORIENTED_EDGE('',*,*,#31851,.F.);
#41666=ORIENTED_EDGE('',*,*,#31856,.F.);
#41667=ORIENTED_EDGE('',*,*,#31857,.T.);
#41668=ORIENTED_EDGE('',*,*,#31858,.T.);
#41669=ORIENTED_EDGE('',*,*,#31854,.F.);
#41670=ORIENTED_EDGE('',*,*,#31859,.F.);
#41671=ORIENTED_EDGE('',*,*,#31860,.T.);
#41672=ORIENTED_EDGE('',*,*,#31861,.T.);
#41673=ORIENTED_EDGE('',*,*,#31857,.F.);
#41674=ORIENTED_EDGE('',*,*,#31862,.F.);
#41675=ORIENTED_EDGE('',*,*,#31863,.T.);
#41676=ORIENTED_EDGE('',*,*,#31864,.T.);
#41677=ORIENTED_EDGE('',*,*,#31860,.F.);
#41678=ORIENTED_EDGE('',*,*,#31865,.F.);
#41679=ORIENTED_EDGE('',*,*,#31866,.T.);
#41680=ORIENTED_EDGE('',*,*,#31867,.T.);
#41681=ORIENTED_EDGE('',*,*,#31863,.F.);
#41682=ORIENTED_EDGE('',*,*,#31868,.F.);
#41683=ORIENTED_EDGE('',*,*,#31869,.T.);
#41684=ORIENTED_EDGE('',*,*,#31870,.T.);
#41685=ORIENTED_EDGE('',*,*,#31866,.F.);
#41686=ORIENTED_EDGE('',*,*,#31871,.F.);
#41687=ORIENTED_EDGE('',*,*,#31872,.T.);
#41688=ORIENTED_EDGE('',*,*,#31873,.T.);
#41689=ORIENTED_EDGE('',*,*,#31869,.F.);
#41690=ORIENTED_EDGE('',*,*,#31874,.F.);
#41691=ORIENTED_EDGE('',*,*,#31875,.T.);
#41692=ORIENTED_EDGE('',*,*,#31876,.T.);
#41693=ORIENTED_EDGE('',*,*,#31872,.F.);
#41694=ORIENTED_EDGE('',*,*,#31877,.F.);
#41695=ORIENTED_EDGE('',*,*,#31878,.T.);
#41696=ORIENTED_EDGE('',*,*,#31879,.T.);
#41697=ORIENTED_EDGE('',*,*,#31875,.F.);
#41698=ORIENTED_EDGE('',*,*,#31880,.F.);
#41699=ORIENTED_EDGE('',*,*,#31881,.T.);
#41700=ORIENTED_EDGE('',*,*,#31882,.T.);
#41701=ORIENTED_EDGE('',*,*,#31878,.F.);
#41702=ORIENTED_EDGE('',*,*,#31883,.F.);
#41703=ORIENTED_EDGE('',*,*,#31884,.T.);
#41704=ORIENTED_EDGE('',*,*,#31885,.T.);
#41705=ORIENTED_EDGE('',*,*,#31881,.F.);
#41706=ORIENTED_EDGE('',*,*,#31886,.F.);
#41707=ORIENTED_EDGE('',*,*,#31887,.T.);
#41708=ORIENTED_EDGE('',*,*,#31888,.T.);
#41709=ORIENTED_EDGE('',*,*,#31884,.F.);
#41710=ORIENTED_EDGE('',*,*,#31889,.F.);
#41711=ORIENTED_EDGE('',*,*,#31890,.T.);
#41712=ORIENTED_EDGE('',*,*,#31891,.T.);
#41713=ORIENTED_EDGE('',*,*,#31887,.F.);
#41714=ORIENTED_EDGE('',*,*,#31892,.F.);
#41715=ORIENTED_EDGE('',*,*,#31893,.T.);
#41716=ORIENTED_EDGE('',*,*,#31894,.T.);
#41717=ORIENTED_EDGE('',*,*,#31890,.F.);
#41718=ORIENTED_EDGE('',*,*,#31895,.F.);
#41719=ORIENTED_EDGE('',*,*,#31896,.T.);
#41720=ORIENTED_EDGE('',*,*,#31897,.T.);
#41721=ORIENTED_EDGE('',*,*,#31893,.F.);
#41722=ORIENTED_EDGE('',*,*,#31898,.F.);
#41723=ORIENTED_EDGE('',*,*,#31899,.T.);
#41724=ORIENTED_EDGE('',*,*,#31900,.T.);
#41725=ORIENTED_EDGE('',*,*,#31896,.F.);
#41726=ORIENTED_EDGE('',*,*,#31901,.F.);
#41727=ORIENTED_EDGE('',*,*,#31902,.T.);
#41728=ORIENTED_EDGE('',*,*,#31903,.T.);
#41729=ORIENTED_EDGE('',*,*,#31899,.F.);
#41730=ORIENTED_EDGE('',*,*,#31904,.F.);
#41731=ORIENTED_EDGE('',*,*,#31905,.T.);
#41732=ORIENTED_EDGE('',*,*,#31906,.T.);
#41733=ORIENTED_EDGE('',*,*,#31902,.F.);
#41734=ORIENTED_EDGE('',*,*,#31907,.F.);
#41735=ORIENTED_EDGE('',*,*,#31908,.T.);
#41736=ORIENTED_EDGE('',*,*,#31909,.T.);
#41737=ORIENTED_EDGE('',*,*,#31905,.F.);
#41738=ORIENTED_EDGE('',*,*,#31910,.F.);
#41739=ORIENTED_EDGE('',*,*,#31825,.T.);
#41740=ORIENTED_EDGE('',*,*,#31911,.T.);
#41741=ORIENTED_EDGE('',*,*,#31908,.F.);
#41742=ORIENTED_EDGE('',*,*,#31911,.F.);
#41743=ORIENTED_EDGE('',*,*,#31824,.F.);
#41744=ORIENTED_EDGE('',*,*,#31828,.F.);
#41745=ORIENTED_EDGE('',*,*,#31831,.F.);
#41746=ORIENTED_EDGE('',*,*,#31834,.F.);
#41747=ORIENTED_EDGE('',*,*,#31837,.F.);
#41748=ORIENTED_EDGE('',*,*,#31840,.F.);
#41749=ORIENTED_EDGE('',*,*,#31843,.F.);
#41750=ORIENTED_EDGE('',*,*,#31846,.F.);
#41751=ORIENTED_EDGE('',*,*,#31849,.F.);
#41752=ORIENTED_EDGE('',*,*,#31852,.F.);
#41753=ORIENTED_EDGE('',*,*,#31855,.F.);
#41754=ORIENTED_EDGE('',*,*,#31858,.F.);
#41755=ORIENTED_EDGE('',*,*,#31861,.F.);
#41756=ORIENTED_EDGE('',*,*,#31864,.F.);
#41757=ORIENTED_EDGE('',*,*,#31867,.F.);
#41758=ORIENTED_EDGE('',*,*,#31870,.F.);
#41759=ORIENTED_EDGE('',*,*,#31873,.F.);
#41760=ORIENTED_EDGE('',*,*,#31876,.F.);
#41761=ORIENTED_EDGE('',*,*,#31879,.F.);
#41762=ORIENTED_EDGE('',*,*,#31882,.F.);
#41763=ORIENTED_EDGE('',*,*,#31885,.F.);
#41764=ORIENTED_EDGE('',*,*,#31888,.F.);
#41765=ORIENTED_EDGE('',*,*,#31891,.F.);
#41766=ORIENTED_EDGE('',*,*,#31894,.F.);
#41767=ORIENTED_EDGE('',*,*,#31897,.F.);
#41768=ORIENTED_EDGE('',*,*,#31900,.F.);
#41769=ORIENTED_EDGE('',*,*,#31903,.F.);
#41770=ORIENTED_EDGE('',*,*,#31906,.F.);
#41771=ORIENTED_EDGE('',*,*,#31909,.F.);
#41772=ORIENTED_EDGE('',*,*,#31762,.T.);
#41773=ORIENTED_EDGE('',*,*,#31784,.T.);
#41774=ORIENTED_EDGE('',*,*,#31781,.T.);
#41775=ORIENTED_EDGE('',*,*,#31778,.T.);
#41776=ORIENTED_EDGE('',*,*,#31775,.T.);
#41777=ORIENTED_EDGE('',*,*,#31772,.T.);
#41778=ORIENTED_EDGE('',*,*,#31769,.T.);
#41779=ORIENTED_EDGE('',*,*,#31766,.T.);
#41780=ORIENTED_EDGE('',*,*,#31912,.F.);
#41781=ORIENTED_EDGE('',*,*,#31913,.T.);
#41782=ORIENTED_EDGE('',*,*,#31914,.T.);
#41783=ORIENTED_EDGE('',*,*,#31915,.F.);
#41784=ORIENTED_EDGE('',*,*,#31916,.F.);
#41785=ORIENTED_EDGE('',*,*,#31917,.T.);
#41786=ORIENTED_EDGE('',*,*,#31918,.T.);
#41787=ORIENTED_EDGE('',*,*,#31913,.F.);
#41788=ORIENTED_EDGE('',*,*,#31919,.F.);
#41789=ORIENTED_EDGE('',*,*,#31920,.T.);
#41790=ORIENTED_EDGE('',*,*,#31921,.T.);
#41791=ORIENTED_EDGE('',*,*,#31917,.F.);
#41792=ORIENTED_EDGE('',*,*,#31922,.F.);
#41793=ORIENTED_EDGE('',*,*,#31923,.T.);
#41794=ORIENTED_EDGE('',*,*,#31924,.T.);
#41795=ORIENTED_EDGE('',*,*,#31920,.F.);
#41796=ORIENTED_EDGE('',*,*,#31925,.F.);
#41797=ORIENTED_EDGE('',*,*,#31926,.T.);
#41798=ORIENTED_EDGE('',*,*,#31927,.T.);
#41799=ORIENTED_EDGE('',*,*,#31923,.F.);
#41800=ORIENTED_EDGE('',*,*,#31928,.F.);
#41801=ORIENTED_EDGE('',*,*,#31929,.T.);
#41802=ORIENTED_EDGE('',*,*,#31930,.T.);
#41803=ORIENTED_EDGE('',*,*,#31926,.F.);
#41804=ORIENTED_EDGE('',*,*,#31931,.F.);
#41805=ORIENTED_EDGE('',*,*,#31932,.T.);
#41806=ORIENTED_EDGE('',*,*,#31933,.T.);
#41807=ORIENTED_EDGE('',*,*,#31929,.F.);
#41808=ORIENTED_EDGE('',*,*,#31934,.F.);
#41809=ORIENTED_EDGE('',*,*,#31915,.T.);
#41810=ORIENTED_EDGE('',*,*,#31935,.T.);
#41811=ORIENTED_EDGE('',*,*,#31932,.F.);
#41812=ORIENTED_EDGE('',*,*,#31936,.F.);
#41813=ORIENTED_EDGE('',*,*,#31937,.T.);
#41814=ORIENTED_EDGE('',*,*,#31938,.T.);
#41815=ORIENTED_EDGE('',*,*,#31939,.F.);
#41816=ORIENTED_EDGE('',*,*,#31940,.F.);
#41817=ORIENTED_EDGE('',*,*,#31941,.T.);
#41818=ORIENTED_EDGE('',*,*,#31942,.T.);
#41819=ORIENTED_EDGE('',*,*,#31937,.F.);
#41820=ORIENTED_EDGE('',*,*,#31943,.F.);
#41821=ORIENTED_EDGE('',*,*,#31944,.T.);
#41822=ORIENTED_EDGE('',*,*,#31945,.T.);
#41823=ORIENTED_EDGE('',*,*,#31941,.F.);
#41824=ORIENTED_EDGE('',*,*,#31946,.F.);
#41825=ORIENTED_EDGE('',*,*,#31947,.T.);
#41826=ORIENTED_EDGE('',*,*,#31948,.T.);
#41827=ORIENTED_EDGE('',*,*,#31944,.F.);
#41828=ORIENTED_EDGE('',*,*,#31949,.F.);
#41829=ORIENTED_EDGE('',*,*,#31950,.T.);
#41830=ORIENTED_EDGE('',*,*,#31951,.T.);
#41831=ORIENTED_EDGE('',*,*,#31947,.F.);
#41832=ORIENTED_EDGE('',*,*,#31952,.F.);
#41833=ORIENTED_EDGE('',*,*,#31953,.T.);
#41834=ORIENTED_EDGE('',*,*,#31954,.T.);
#41835=ORIENTED_EDGE('',*,*,#31950,.F.);
#41836=ORIENTED_EDGE('',*,*,#31955,.F.);
#41837=ORIENTED_EDGE('',*,*,#31956,.T.);
#41838=ORIENTED_EDGE('',*,*,#31957,.T.);
#41839=ORIENTED_EDGE('',*,*,#31953,.F.);
#41840=ORIENTED_EDGE('',*,*,#31958,.F.);
#41841=ORIENTED_EDGE('',*,*,#31959,.T.);
#41842=ORIENTED_EDGE('',*,*,#31960,.T.);
#41843=ORIENTED_EDGE('',*,*,#31956,.F.);
#41844=ORIENTED_EDGE('',*,*,#31961,.F.);
#41845=ORIENTED_EDGE('',*,*,#31962,.T.);
#41846=ORIENTED_EDGE('',*,*,#31963,.T.);
#41847=ORIENTED_EDGE('',*,*,#31959,.F.);
#41848=ORIENTED_EDGE('',*,*,#31964,.F.);
#41849=ORIENTED_EDGE('',*,*,#31965,.T.);
#41850=ORIENTED_EDGE('',*,*,#31966,.T.);
#41851=ORIENTED_EDGE('',*,*,#31962,.F.);
#41852=ORIENTED_EDGE('',*,*,#31967,.F.);
#41853=ORIENTED_EDGE('',*,*,#31968,.T.);
#41854=ORIENTED_EDGE('',*,*,#31969,.T.);
#41855=ORIENTED_EDGE('',*,*,#31965,.F.);
#41856=ORIENTED_EDGE('',*,*,#31970,.F.);
#41857=ORIENTED_EDGE('',*,*,#31939,.T.);
#41858=ORIENTED_EDGE('',*,*,#31971,.T.);
#41859=ORIENTED_EDGE('',*,*,#31968,.F.);
#41860=ORIENTED_EDGE('',*,*,#31971,.F.);
#41861=ORIENTED_EDGE('',*,*,#31938,.F.);
#41862=ORIENTED_EDGE('',*,*,#31942,.F.);
#41863=ORIENTED_EDGE('',*,*,#31945,.F.);
#41864=ORIENTED_EDGE('',*,*,#31948,.F.);
#41865=ORIENTED_EDGE('',*,*,#31951,.F.);
#41866=ORIENTED_EDGE('',*,*,#31954,.F.);
#41867=ORIENTED_EDGE('',*,*,#31957,.F.);
#41868=ORIENTED_EDGE('',*,*,#31960,.F.);
#41869=ORIENTED_EDGE('',*,*,#31963,.F.);
#41870=ORIENTED_EDGE('',*,*,#31966,.F.);
#41871=ORIENTED_EDGE('',*,*,#31969,.F.);
#41872=ORIENTED_EDGE('',*,*,#31935,.F.);
#41873=ORIENTED_EDGE('',*,*,#31914,.F.);
#41874=ORIENTED_EDGE('',*,*,#31918,.F.);
#41875=ORIENTED_EDGE('',*,*,#31921,.F.);
#41876=ORIENTED_EDGE('',*,*,#31924,.F.);
#41877=ORIENTED_EDGE('',*,*,#31927,.F.);
#41878=ORIENTED_EDGE('',*,*,#31930,.F.);
#41879=ORIENTED_EDGE('',*,*,#31933,.F.);
#41880=ORIENTED_EDGE('',*,*,#31972,.F.);
#41881=ORIENTED_EDGE('',*,*,#31973,.T.);
#41882=ORIENTED_EDGE('',*,*,#31974,.T.);
#41883=ORIENTED_EDGE('',*,*,#31975,.F.);
#41884=ORIENTED_EDGE('',*,*,#31976,.F.);
#41885=ORIENTED_EDGE('',*,*,#31977,.T.);
#41886=ORIENTED_EDGE('',*,*,#31978,.T.);
#41887=ORIENTED_EDGE('',*,*,#31973,.F.);
#41888=ORIENTED_EDGE('',*,*,#31979,.F.);
#41889=ORIENTED_EDGE('',*,*,#31975,.T.);
#41890=ORIENTED_EDGE('',*,*,#31980,.T.);
#41891=ORIENTED_EDGE('',*,*,#31977,.F.);
#41892=ORIENTED_EDGE('',*,*,#31981,.F.);
#41893=ORIENTED_EDGE('',*,*,#31982,.T.);
#41894=ORIENTED_EDGE('',*,*,#31983,.T.);
#41895=ORIENTED_EDGE('',*,*,#31984,.F.);
#41896=ORIENTED_EDGE('',*,*,#31985,.F.);
#41897=ORIENTED_EDGE('',*,*,#31986,.T.);
#41898=ORIENTED_EDGE('',*,*,#31987,.T.);
#41899=ORIENTED_EDGE('',*,*,#31982,.F.);
#41900=ORIENTED_EDGE('',*,*,#31988,.F.);
#41901=ORIENTED_EDGE('',*,*,#31989,.T.);
#41902=ORIENTED_EDGE('',*,*,#31990,.T.);
#41903=ORIENTED_EDGE('',*,*,#31986,.F.);
#41904=ORIENTED_EDGE('',*,*,#31991,.F.);
#41905=ORIENTED_EDGE('',*,*,#31992,.T.);
#41906=ORIENTED_EDGE('',*,*,#31993,.T.);
#41907=ORIENTED_EDGE('',*,*,#31989,.F.);
#41908=ORIENTED_EDGE('',*,*,#31994,.F.);
#41909=ORIENTED_EDGE('',*,*,#31995,.T.);
#41910=ORIENTED_EDGE('',*,*,#31996,.T.);
#41911=ORIENTED_EDGE('',*,*,#31992,.F.);
#41912=ORIENTED_EDGE('',*,*,#31997,.F.);
#41913=ORIENTED_EDGE('',*,*,#31998,.T.);
#41914=ORIENTED_EDGE('',*,*,#31999,.T.);
#41915=ORIENTED_EDGE('',*,*,#31995,.F.);
#41916=ORIENTED_EDGE('',*,*,#32000,.F.);
#41917=ORIENTED_EDGE('',*,*,#32001,.T.);
#41918=ORIENTED_EDGE('',*,*,#32002,.T.);
#41919=ORIENTED_EDGE('',*,*,#31998,.F.);
#41920=ORIENTED_EDGE('',*,*,#32003,.F.);
#41921=ORIENTED_EDGE('',*,*,#32004,.T.);
#41922=ORIENTED_EDGE('',*,*,#32005,.T.);
#41923=ORIENTED_EDGE('',*,*,#32001,.F.);
#41924=ORIENTED_EDGE('',*,*,#32006,.F.);
#41925=ORIENTED_EDGE('',*,*,#32007,.T.);
#41926=ORIENTED_EDGE('',*,*,#32008,.T.);
#41927=ORIENTED_EDGE('',*,*,#32004,.F.);
#41928=ORIENTED_EDGE('',*,*,#32009,.F.);
#41929=ORIENTED_EDGE('',*,*,#32010,.T.);
#41930=ORIENTED_EDGE('',*,*,#32011,.T.);
#41931=ORIENTED_EDGE('',*,*,#32007,.F.);
#41932=ORIENTED_EDGE('',*,*,#32012,.F.);
#41933=ORIENTED_EDGE('',*,*,#31984,.T.);
#41934=ORIENTED_EDGE('',*,*,#32013,.T.);
#41935=ORIENTED_EDGE('',*,*,#32010,.F.);
#41936=ORIENTED_EDGE('',*,*,#32013,.F.);
#41937=ORIENTED_EDGE('',*,*,#31983,.F.);
#41938=ORIENTED_EDGE('',*,*,#31987,.F.);
#41939=ORIENTED_EDGE('',*,*,#31990,.F.);
#41940=ORIENTED_EDGE('',*,*,#31993,.F.);
#41941=ORIENTED_EDGE('',*,*,#31996,.F.);
#41942=ORIENTED_EDGE('',*,*,#31999,.F.);
#41943=ORIENTED_EDGE('',*,*,#32002,.F.);
#41944=ORIENTED_EDGE('',*,*,#32005,.F.);
#41945=ORIENTED_EDGE('',*,*,#32008,.F.);
#41946=ORIENTED_EDGE('',*,*,#32011,.F.);
#41947=ORIENTED_EDGE('',*,*,#31980,.F.);
#41948=ORIENTED_EDGE('',*,*,#31974,.F.);
#41949=ORIENTED_EDGE('',*,*,#31978,.F.);
#41950=ORIENTED_EDGE('',*,*,#31972,.T.);
#41951=ORIENTED_EDGE('',*,*,#31979,.T.);
#41952=ORIENTED_EDGE('',*,*,#31976,.T.);
#41953=ORIENTED_EDGE('',*,*,#31912,.T.);
#41954=ORIENTED_EDGE('',*,*,#31934,.T.);
#41955=ORIENTED_EDGE('',*,*,#31931,.T.);
#41956=ORIENTED_EDGE('',*,*,#31928,.T.);
#41957=ORIENTED_EDGE('',*,*,#31925,.T.);
#41958=ORIENTED_EDGE('',*,*,#31922,.T.);
#41959=ORIENTED_EDGE('',*,*,#31919,.T.);
#41960=ORIENTED_EDGE('',*,*,#31916,.T.);
#41961=ORIENTED_EDGE('',*,*,#32014,.F.);
#41962=ORIENTED_EDGE('',*,*,#32015,.T.);
#41963=ORIENTED_EDGE('',*,*,#32016,.T.);
#41964=ORIENTED_EDGE('',*,*,#32017,.F.);
#41965=ORIENTED_EDGE('',*,*,#32018,.F.);
#41966=ORIENTED_EDGE('',*,*,#32019,.T.);
#41967=ORIENTED_EDGE('',*,*,#32020,.T.);
#41968=ORIENTED_EDGE('',*,*,#32015,.F.);
#41969=ORIENTED_EDGE('',*,*,#32021,.F.);
#41970=ORIENTED_EDGE('',*,*,#32022,.T.);
#41971=ORIENTED_EDGE('',*,*,#32023,.T.);
#41972=ORIENTED_EDGE('',*,*,#32019,.F.);
#41973=ORIENTED_EDGE('',*,*,#32024,.F.);
#41974=ORIENTED_EDGE('',*,*,#32025,.T.);
#41975=ORIENTED_EDGE('',*,*,#32026,.T.);
#41976=ORIENTED_EDGE('',*,*,#32022,.F.);
#41977=ORIENTED_EDGE('',*,*,#32027,.F.);
#41978=ORIENTED_EDGE('',*,*,#32028,.T.);
#41979=ORIENTED_EDGE('',*,*,#32029,.T.);
#41980=ORIENTED_EDGE('',*,*,#32025,.F.);
#41981=ORIENTED_EDGE('',*,*,#32030,.F.);
#41982=ORIENTED_EDGE('',*,*,#32031,.T.);
#41983=ORIENTED_EDGE('',*,*,#32032,.T.);
#41984=ORIENTED_EDGE('',*,*,#32028,.F.);
#41985=ORIENTED_EDGE('',*,*,#32033,.F.);
#41986=ORIENTED_EDGE('',*,*,#32034,.T.);
#41987=ORIENTED_EDGE('',*,*,#32035,.T.);
#41988=ORIENTED_EDGE('',*,*,#32031,.F.);
#41989=ORIENTED_EDGE('',*,*,#32036,.F.);
#41990=ORIENTED_EDGE('',*,*,#32017,.T.);
#41991=ORIENTED_EDGE('',*,*,#32037,.T.);
#41992=ORIENTED_EDGE('',*,*,#32034,.F.);
#41993=ORIENTED_EDGE('',*,*,#32038,.F.);
#41994=ORIENTED_EDGE('',*,*,#32039,.T.);
#41995=ORIENTED_EDGE('',*,*,#32040,.T.);
#41996=ORIENTED_EDGE('',*,*,#32041,.F.);
#41997=ORIENTED_EDGE('',*,*,#32042,.F.);
#41998=ORIENTED_EDGE('',*,*,#32043,.T.);
#41999=ORIENTED_EDGE('',*,*,#32044,.T.);
#42000=ORIENTED_EDGE('',*,*,#32039,.F.);
#42001=ORIENTED_EDGE('',*,*,#32045,.F.);
#42002=ORIENTED_EDGE('',*,*,#32046,.T.);
#42003=ORIENTED_EDGE('',*,*,#32047,.T.);
#42004=ORIENTED_EDGE('',*,*,#32043,.F.);
#42005=ORIENTED_EDGE('',*,*,#32048,.F.);
#42006=ORIENTED_EDGE('',*,*,#32049,.T.);
#42007=ORIENTED_EDGE('',*,*,#32050,.T.);
#42008=ORIENTED_EDGE('',*,*,#32046,.F.);
#42009=ORIENTED_EDGE('',*,*,#32051,.F.);
#42010=ORIENTED_EDGE('',*,*,#32052,.T.);
#42011=ORIENTED_EDGE('',*,*,#32053,.T.);
#42012=ORIENTED_EDGE('',*,*,#32049,.F.);
#42013=ORIENTED_EDGE('',*,*,#32054,.F.);
#42014=ORIENTED_EDGE('',*,*,#32055,.T.);
#42015=ORIENTED_EDGE('',*,*,#32056,.T.);
#42016=ORIENTED_EDGE('',*,*,#32052,.F.);
#42017=ORIENTED_EDGE('',*,*,#32057,.F.);
#42018=ORIENTED_EDGE('',*,*,#32058,.T.);
#42019=ORIENTED_EDGE('',*,*,#32059,.T.);
#42020=ORIENTED_EDGE('',*,*,#32055,.F.);
#42021=ORIENTED_EDGE('',*,*,#32060,.F.);
#42022=ORIENTED_EDGE('',*,*,#32061,.T.);
#42023=ORIENTED_EDGE('',*,*,#32062,.T.);
#42024=ORIENTED_EDGE('',*,*,#32058,.F.);
#42025=ORIENTED_EDGE('',*,*,#32063,.F.);
#42026=ORIENTED_EDGE('',*,*,#32064,.T.);
#42027=ORIENTED_EDGE('',*,*,#32065,.T.);
#42028=ORIENTED_EDGE('',*,*,#32061,.F.);
#42029=ORIENTED_EDGE('',*,*,#32066,.F.);
#42030=ORIENTED_EDGE('',*,*,#32067,.T.);
#42031=ORIENTED_EDGE('',*,*,#32068,.T.);
#42032=ORIENTED_EDGE('',*,*,#32064,.F.);
#42033=ORIENTED_EDGE('',*,*,#32069,.F.);
#42034=ORIENTED_EDGE('',*,*,#32070,.T.);
#42035=ORIENTED_EDGE('',*,*,#32071,.T.);
#42036=ORIENTED_EDGE('',*,*,#32067,.F.);
#42037=ORIENTED_EDGE('',*,*,#32072,.F.);
#42038=ORIENTED_EDGE('',*,*,#32041,.T.);
#42039=ORIENTED_EDGE('',*,*,#32073,.T.);
#42040=ORIENTED_EDGE('',*,*,#32070,.F.);
#42041=ORIENTED_EDGE('',*,*,#32073,.F.);
#42042=ORIENTED_EDGE('',*,*,#32040,.F.);
#42043=ORIENTED_EDGE('',*,*,#32044,.F.);
#42044=ORIENTED_EDGE('',*,*,#32047,.F.);
#42045=ORIENTED_EDGE('',*,*,#32050,.F.);
#42046=ORIENTED_EDGE('',*,*,#32053,.F.);
#42047=ORIENTED_EDGE('',*,*,#32056,.F.);
#42048=ORIENTED_EDGE('',*,*,#32059,.F.);
#42049=ORIENTED_EDGE('',*,*,#32062,.F.);
#42050=ORIENTED_EDGE('',*,*,#32065,.F.);
#42051=ORIENTED_EDGE('',*,*,#32068,.F.);
#42052=ORIENTED_EDGE('',*,*,#32071,.F.);
#42053=ORIENTED_EDGE('',*,*,#32037,.F.);
#42054=ORIENTED_EDGE('',*,*,#32016,.F.);
#42055=ORIENTED_EDGE('',*,*,#32020,.F.);
#42056=ORIENTED_EDGE('',*,*,#32023,.F.);
#42057=ORIENTED_EDGE('',*,*,#32026,.F.);
#42058=ORIENTED_EDGE('',*,*,#32029,.F.);
#42059=ORIENTED_EDGE('',*,*,#32032,.F.);
#42060=ORIENTED_EDGE('',*,*,#32035,.F.);
#42061=ORIENTED_EDGE('',*,*,#32074,.F.);
#42062=ORIENTED_EDGE('',*,*,#32075,.T.);
#42063=ORIENTED_EDGE('',*,*,#32076,.T.);
#42064=ORIENTED_EDGE('',*,*,#32077,.F.);
#42065=ORIENTED_EDGE('',*,*,#32078,.F.);
#42066=ORIENTED_EDGE('',*,*,#32079,.T.);
#42067=ORIENTED_EDGE('',*,*,#32080,.T.);
#42068=ORIENTED_EDGE('',*,*,#32075,.F.);
#42069=ORIENTED_EDGE('',*,*,#32081,.F.);
#42070=ORIENTED_EDGE('',*,*,#32082,.T.);
#42071=ORIENTED_EDGE('',*,*,#32083,.T.);
#42072=ORIENTED_EDGE('',*,*,#32079,.F.);
#42073=ORIENTED_EDGE('',*,*,#32084,.F.);
#42074=ORIENTED_EDGE('',*,*,#32085,.T.);
#42075=ORIENTED_EDGE('',*,*,#32086,.T.);
#42076=ORIENTED_EDGE('',*,*,#32082,.F.);
#42077=ORIENTED_EDGE('',*,*,#32087,.F.);
#42078=ORIENTED_EDGE('',*,*,#32088,.T.);
#42079=ORIENTED_EDGE('',*,*,#32089,.T.);
#42080=ORIENTED_EDGE('',*,*,#32085,.F.);
#42081=ORIENTED_EDGE('',*,*,#32090,.F.);
#42082=ORIENTED_EDGE('',*,*,#32091,.T.);
#42083=ORIENTED_EDGE('',*,*,#32092,.T.);
#42084=ORIENTED_EDGE('',*,*,#32088,.F.);
#42085=ORIENTED_EDGE('',*,*,#32093,.F.);
#42086=ORIENTED_EDGE('',*,*,#32094,.T.);
#42087=ORIENTED_EDGE('',*,*,#32095,.T.);
#42088=ORIENTED_EDGE('',*,*,#32091,.F.);
#42089=ORIENTED_EDGE('',*,*,#32096,.F.);
#42090=ORIENTED_EDGE('',*,*,#32097,.T.);
#42091=ORIENTED_EDGE('',*,*,#32098,.T.);
#42092=ORIENTED_EDGE('',*,*,#32094,.F.);
#42093=ORIENTED_EDGE('',*,*,#32099,.F.);
#42094=ORIENTED_EDGE('',*,*,#32100,.T.);
#42095=ORIENTED_EDGE('',*,*,#32101,.T.);
#42096=ORIENTED_EDGE('',*,*,#32097,.F.);
#42097=ORIENTED_EDGE('',*,*,#32102,.F.);
#42098=ORIENTED_EDGE('',*,*,#32103,.T.);
#42099=ORIENTED_EDGE('',*,*,#32104,.T.);
#42100=ORIENTED_EDGE('',*,*,#32100,.F.);
#42101=ORIENTED_EDGE('',*,*,#32105,.F.);
#42102=ORIENTED_EDGE('',*,*,#32106,.T.);
#42103=ORIENTED_EDGE('',*,*,#32107,.T.);
#42104=ORIENTED_EDGE('',*,*,#32103,.F.);
#42105=ORIENTED_EDGE('',*,*,#32108,.F.);
#42106=ORIENTED_EDGE('',*,*,#32109,.T.);
#42107=ORIENTED_EDGE('',*,*,#32110,.T.);
#42108=ORIENTED_EDGE('',*,*,#32106,.F.);
#42109=ORIENTED_EDGE('',*,*,#32111,.F.);
#42110=ORIENTED_EDGE('',*,*,#32112,.T.);
#42111=ORIENTED_EDGE('',*,*,#32113,.T.);
#42112=ORIENTED_EDGE('',*,*,#32109,.F.);
#42113=ORIENTED_EDGE('',*,*,#32114,.F.);
#42114=ORIENTED_EDGE('',*,*,#32115,.T.);
#42115=ORIENTED_EDGE('',*,*,#32116,.T.);
#42116=ORIENTED_EDGE('',*,*,#32112,.F.);
#42117=ORIENTED_EDGE('',*,*,#32117,.F.);
#42118=ORIENTED_EDGE('',*,*,#32118,.T.);
#42119=ORIENTED_EDGE('',*,*,#32119,.T.);
#42120=ORIENTED_EDGE('',*,*,#32115,.F.);
#42121=ORIENTED_EDGE('',*,*,#32120,.F.);
#42122=ORIENTED_EDGE('',*,*,#32121,.T.);
#42123=ORIENTED_EDGE('',*,*,#32122,.T.);
#42124=ORIENTED_EDGE('',*,*,#32118,.F.);
#42125=ORIENTED_EDGE('',*,*,#32123,.F.);
#42126=ORIENTED_EDGE('',*,*,#32124,.T.);
#42127=ORIENTED_EDGE('',*,*,#32125,.T.);
#42128=ORIENTED_EDGE('',*,*,#32121,.F.);
#42129=ORIENTED_EDGE('',*,*,#32126,.F.);
#42130=ORIENTED_EDGE('',*,*,#32127,.T.);
#42131=ORIENTED_EDGE('',*,*,#32128,.T.);
#42132=ORIENTED_EDGE('',*,*,#32124,.F.);
#42133=ORIENTED_EDGE('',*,*,#32129,.F.);
#42134=ORIENTED_EDGE('',*,*,#32130,.T.);
#42135=ORIENTED_EDGE('',*,*,#32131,.T.);
#42136=ORIENTED_EDGE('',*,*,#32127,.F.);
#42137=ORIENTED_EDGE('',*,*,#32132,.F.);
#42138=ORIENTED_EDGE('',*,*,#32133,.T.);
#42139=ORIENTED_EDGE('',*,*,#32134,.T.);
#42140=ORIENTED_EDGE('',*,*,#32130,.F.);
#42141=ORIENTED_EDGE('',*,*,#32135,.F.);
#42142=ORIENTED_EDGE('',*,*,#32136,.T.);
#42143=ORIENTED_EDGE('',*,*,#32137,.T.);
#42144=ORIENTED_EDGE('',*,*,#32133,.F.);
#42145=ORIENTED_EDGE('',*,*,#32138,.F.);
#42146=ORIENTED_EDGE('',*,*,#32077,.T.);
#42147=ORIENTED_EDGE('',*,*,#32139,.T.);
#42148=ORIENTED_EDGE('',*,*,#32136,.F.);
#42149=ORIENTED_EDGE('',*,*,#32139,.F.);
#42150=ORIENTED_EDGE('',*,*,#32076,.F.);
#42151=ORIENTED_EDGE('',*,*,#32080,.F.);
#42152=ORIENTED_EDGE('',*,*,#32083,.F.);
#42153=ORIENTED_EDGE('',*,*,#32086,.F.);
#42154=ORIENTED_EDGE('',*,*,#32089,.F.);
#42155=ORIENTED_EDGE('',*,*,#32092,.F.);
#42156=ORIENTED_EDGE('',*,*,#32095,.F.);
#42157=ORIENTED_EDGE('',*,*,#32098,.F.);
#42158=ORIENTED_EDGE('',*,*,#32101,.F.);
#42159=ORIENTED_EDGE('',*,*,#32104,.F.);
#42160=ORIENTED_EDGE('',*,*,#32107,.F.);
#42161=ORIENTED_EDGE('',*,*,#32110,.F.);
#42162=ORIENTED_EDGE('',*,*,#32113,.F.);
#42163=ORIENTED_EDGE('',*,*,#32116,.F.);
#42164=ORIENTED_EDGE('',*,*,#32119,.F.);
#42165=ORIENTED_EDGE('',*,*,#32122,.F.);
#42166=ORIENTED_EDGE('',*,*,#32125,.F.);
#42167=ORIENTED_EDGE('',*,*,#32128,.F.);
#42168=ORIENTED_EDGE('',*,*,#32131,.F.);
#42169=ORIENTED_EDGE('',*,*,#32134,.F.);
#42170=ORIENTED_EDGE('',*,*,#32137,.F.);
#42171=ORIENTED_EDGE('',*,*,#32014,.T.);
#42172=ORIENTED_EDGE('',*,*,#32036,.T.);
#42173=ORIENTED_EDGE('',*,*,#32033,.T.);
#42174=ORIENTED_EDGE('',*,*,#32030,.T.);
#42175=ORIENTED_EDGE('',*,*,#32027,.T.);
#42176=ORIENTED_EDGE('',*,*,#32024,.T.);
#42177=ORIENTED_EDGE('',*,*,#32021,.T.);
#42178=ORIENTED_EDGE('',*,*,#32018,.T.);
#42179=ORIENTED_EDGE('',*,*,#32140,.F.);
#42180=ORIENTED_EDGE('',*,*,#32141,.T.);
#42181=ORIENTED_EDGE('',*,*,#32142,.T.);
#42182=ORIENTED_EDGE('',*,*,#32143,.F.);
#42183=ORIENTED_EDGE('',*,*,#32144,.F.);
#42184=ORIENTED_EDGE('',*,*,#32145,.T.);
#42185=ORIENTED_EDGE('',*,*,#32146,.T.);
#42186=ORIENTED_EDGE('',*,*,#32141,.F.);
#42187=ORIENTED_EDGE('',*,*,#32147,.F.);
#42188=ORIENTED_EDGE('',*,*,#32148,.T.);
#42189=ORIENTED_EDGE('',*,*,#32149,.T.);
#42190=ORIENTED_EDGE('',*,*,#32145,.F.);
#42191=ORIENTED_EDGE('',*,*,#32150,.F.);
#42192=ORIENTED_EDGE('',*,*,#32151,.T.);
#42193=ORIENTED_EDGE('',*,*,#32152,.T.);
#42194=ORIENTED_EDGE('',*,*,#32148,.F.);
#42195=ORIENTED_EDGE('',*,*,#32153,.F.);
#42196=ORIENTED_EDGE('',*,*,#32154,.T.);
#42197=ORIENTED_EDGE('',*,*,#32155,.T.);
#42198=ORIENTED_EDGE('',*,*,#32151,.F.);
#42199=ORIENTED_EDGE('',*,*,#32156,.F.);
#42200=ORIENTED_EDGE('',*,*,#32157,.T.);
#42201=ORIENTED_EDGE('',*,*,#32158,.T.);
#42202=ORIENTED_EDGE('',*,*,#32154,.F.);
#42203=ORIENTED_EDGE('',*,*,#32159,.F.);
#42204=ORIENTED_EDGE('',*,*,#32160,.T.);
#42205=ORIENTED_EDGE('',*,*,#32161,.T.);
#42206=ORIENTED_EDGE('',*,*,#32157,.F.);
#42207=ORIENTED_EDGE('',*,*,#32162,.F.);
#42208=ORIENTED_EDGE('',*,*,#32143,.T.);
#42209=ORIENTED_EDGE('',*,*,#32163,.T.);
#42210=ORIENTED_EDGE('',*,*,#32160,.F.);
#42211=ORIENTED_EDGE('',*,*,#32164,.F.);
#42212=ORIENTED_EDGE('',*,*,#32165,.T.);
#42213=ORIENTED_EDGE('',*,*,#32166,.T.);
#42214=ORIENTED_EDGE('',*,*,#32167,.F.);
#42215=ORIENTED_EDGE('',*,*,#32168,.F.);
#42216=ORIENTED_EDGE('',*,*,#32169,.T.);
#42217=ORIENTED_EDGE('',*,*,#32170,.T.);
#42218=ORIENTED_EDGE('',*,*,#32165,.F.);
#42219=ORIENTED_EDGE('',*,*,#32171,.F.);
#42220=ORIENTED_EDGE('',*,*,#32172,.T.);
#42221=ORIENTED_EDGE('',*,*,#32173,.T.);
#42222=ORIENTED_EDGE('',*,*,#32169,.F.);
#42223=ORIENTED_EDGE('',*,*,#32174,.F.);
#42224=ORIENTED_EDGE('',*,*,#32175,.T.);
#42225=ORIENTED_EDGE('',*,*,#32176,.T.);
#42226=ORIENTED_EDGE('',*,*,#32172,.F.);
#42227=ORIENTED_EDGE('',*,*,#32177,.F.);
#42228=ORIENTED_EDGE('',*,*,#32178,.T.);
#42229=ORIENTED_EDGE('',*,*,#32179,.T.);
#42230=ORIENTED_EDGE('',*,*,#32175,.F.);
#42231=ORIENTED_EDGE('',*,*,#32180,.F.);
#42232=ORIENTED_EDGE('',*,*,#32181,.T.);
#42233=ORIENTED_EDGE('',*,*,#32182,.T.);
#42234=ORIENTED_EDGE('',*,*,#32178,.F.);
#42235=ORIENTED_EDGE('',*,*,#32183,.F.);
#42236=ORIENTED_EDGE('',*,*,#32184,.T.);
#42237=ORIENTED_EDGE('',*,*,#32185,.T.);
#42238=ORIENTED_EDGE('',*,*,#32181,.F.);
#42239=ORIENTED_EDGE('',*,*,#32186,.F.);
#42240=ORIENTED_EDGE('',*,*,#32187,.T.);
#42241=ORIENTED_EDGE('',*,*,#32188,.T.);
#42242=ORIENTED_EDGE('',*,*,#32184,.F.);
#42243=ORIENTED_EDGE('',*,*,#32189,.F.);
#42244=ORIENTED_EDGE('',*,*,#32190,.T.);
#42245=ORIENTED_EDGE('',*,*,#32191,.T.);
#42246=ORIENTED_EDGE('',*,*,#32187,.F.);
#42247=ORIENTED_EDGE('',*,*,#32192,.F.);
#42248=ORIENTED_EDGE('',*,*,#32193,.T.);
#42249=ORIENTED_EDGE('',*,*,#32194,.T.);
#42250=ORIENTED_EDGE('',*,*,#32190,.F.);
#42251=ORIENTED_EDGE('',*,*,#32195,.F.);
#42252=ORIENTED_EDGE('',*,*,#32196,.T.);
#42253=ORIENTED_EDGE('',*,*,#32197,.T.);
#42254=ORIENTED_EDGE('',*,*,#32193,.F.);
#42255=ORIENTED_EDGE('',*,*,#32198,.F.);
#42256=ORIENTED_EDGE('',*,*,#32167,.T.);
#42257=ORIENTED_EDGE('',*,*,#32199,.T.);
#42258=ORIENTED_EDGE('',*,*,#32196,.F.);
#42259=ORIENTED_EDGE('',*,*,#32199,.F.);
#42260=ORIENTED_EDGE('',*,*,#32166,.F.);
#42261=ORIENTED_EDGE('',*,*,#32170,.F.);
#42262=ORIENTED_EDGE('',*,*,#32173,.F.);
#42263=ORIENTED_EDGE('',*,*,#32176,.F.);
#42264=ORIENTED_EDGE('',*,*,#32179,.F.);
#42265=ORIENTED_EDGE('',*,*,#32182,.F.);
#42266=ORIENTED_EDGE('',*,*,#32185,.F.);
#42267=ORIENTED_EDGE('',*,*,#32188,.F.);
#42268=ORIENTED_EDGE('',*,*,#32191,.F.);
#42269=ORIENTED_EDGE('',*,*,#32194,.F.);
#42270=ORIENTED_EDGE('',*,*,#32197,.F.);
#42271=ORIENTED_EDGE('',*,*,#32163,.F.);
#42272=ORIENTED_EDGE('',*,*,#32142,.F.);
#42273=ORIENTED_EDGE('',*,*,#32146,.F.);
#42274=ORIENTED_EDGE('',*,*,#32149,.F.);
#42275=ORIENTED_EDGE('',*,*,#32152,.F.);
#42276=ORIENTED_EDGE('',*,*,#32155,.F.);
#42277=ORIENTED_EDGE('',*,*,#32158,.F.);
#42278=ORIENTED_EDGE('',*,*,#32161,.F.);
#42279=ORIENTED_EDGE('',*,*,#32200,.F.);
#42280=ORIENTED_EDGE('',*,*,#32201,.T.);
#42281=ORIENTED_EDGE('',*,*,#32202,.T.);
#42282=ORIENTED_EDGE('',*,*,#32203,.F.);
#42283=ORIENTED_EDGE('',*,*,#32204,.F.);
#42284=ORIENTED_EDGE('',*,*,#32205,.T.);
#42285=ORIENTED_EDGE('',*,*,#32206,.T.);
#42286=ORIENTED_EDGE('',*,*,#32201,.F.);
#42287=ORIENTED_EDGE('',*,*,#32207,.F.);
#42288=ORIENTED_EDGE('',*,*,#32208,.T.);
#42289=ORIENTED_EDGE('',*,*,#32209,.T.);
#42290=ORIENTED_EDGE('',*,*,#32205,.F.);
#42291=ORIENTED_EDGE('',*,*,#32210,.F.);
#42292=ORIENTED_EDGE('',*,*,#32211,.T.);
#42293=ORIENTED_EDGE('',*,*,#32212,.T.);
#42294=ORIENTED_EDGE('',*,*,#32208,.F.);
#42295=ORIENTED_EDGE('',*,*,#32213,.F.);
#42296=ORIENTED_EDGE('',*,*,#32214,.T.);
#42297=ORIENTED_EDGE('',*,*,#32215,.T.);
#42298=ORIENTED_EDGE('',*,*,#32211,.F.);
#42299=ORIENTED_EDGE('',*,*,#32216,.F.);
#42300=ORIENTED_EDGE('',*,*,#32217,.T.);
#42301=ORIENTED_EDGE('',*,*,#32218,.T.);
#42302=ORIENTED_EDGE('',*,*,#32214,.F.);
#42303=ORIENTED_EDGE('',*,*,#32219,.F.);
#42304=ORIENTED_EDGE('',*,*,#32220,.T.);
#42305=ORIENTED_EDGE('',*,*,#32221,.T.);
#42306=ORIENTED_EDGE('',*,*,#32217,.F.);
#42307=ORIENTED_EDGE('',*,*,#32222,.F.);
#42308=ORIENTED_EDGE('',*,*,#32223,.T.);
#42309=ORIENTED_EDGE('',*,*,#32224,.T.);
#42310=ORIENTED_EDGE('',*,*,#32220,.F.);
#42311=ORIENTED_EDGE('',*,*,#32225,.F.);
#42312=ORIENTED_EDGE('',*,*,#32203,.T.);
#42313=ORIENTED_EDGE('',*,*,#32226,.T.);
#42314=ORIENTED_EDGE('',*,*,#32223,.F.);
#42315=ORIENTED_EDGE('',*,*,#32227,.F.);
#42316=ORIENTED_EDGE('',*,*,#32228,.T.);
#42317=ORIENTED_EDGE('',*,*,#32229,.T.);
#42318=ORIENTED_EDGE('',*,*,#32230,.F.);
#42319=ORIENTED_EDGE('',*,*,#32231,.F.);
#42320=ORIENTED_EDGE('',*,*,#32232,.T.);
#42321=ORIENTED_EDGE('',*,*,#32233,.T.);
#42322=ORIENTED_EDGE('',*,*,#32228,.F.);
#42323=ORIENTED_EDGE('',*,*,#32234,.F.);
#42324=ORIENTED_EDGE('',*,*,#32235,.T.);
#42325=ORIENTED_EDGE('',*,*,#32236,.T.);
#42326=ORIENTED_EDGE('',*,*,#32232,.F.);
#42327=ORIENTED_EDGE('',*,*,#32237,.F.);
#42328=ORIENTED_EDGE('',*,*,#32238,.T.);
#42329=ORIENTED_EDGE('',*,*,#32239,.T.);
#42330=ORIENTED_EDGE('',*,*,#32235,.F.);
#42331=ORIENTED_EDGE('',*,*,#32240,.F.);
#42332=ORIENTED_EDGE('',*,*,#32241,.T.);
#42333=ORIENTED_EDGE('',*,*,#32242,.T.);
#42334=ORIENTED_EDGE('',*,*,#32238,.F.);
#42335=ORIENTED_EDGE('',*,*,#32243,.F.);
#42336=ORIENTED_EDGE('',*,*,#32244,.T.);
#42337=ORIENTED_EDGE('',*,*,#32245,.T.);
#42338=ORIENTED_EDGE('',*,*,#32241,.F.);
#42339=ORIENTED_EDGE('',*,*,#32246,.F.);
#42340=ORIENTED_EDGE('',*,*,#32247,.T.);
#42341=ORIENTED_EDGE('',*,*,#32248,.T.);
#42342=ORIENTED_EDGE('',*,*,#32244,.F.);
#42343=ORIENTED_EDGE('',*,*,#32249,.F.);
#42344=ORIENTED_EDGE('',*,*,#32250,.T.);
#42345=ORIENTED_EDGE('',*,*,#32251,.T.);
#42346=ORIENTED_EDGE('',*,*,#32247,.F.);
#42347=ORIENTED_EDGE('',*,*,#32252,.F.);
#42348=ORIENTED_EDGE('',*,*,#32253,.T.);
#42349=ORIENTED_EDGE('',*,*,#32254,.T.);
#42350=ORIENTED_EDGE('',*,*,#32250,.F.);
#42351=ORIENTED_EDGE('',*,*,#32255,.F.);
#42352=ORIENTED_EDGE('',*,*,#32256,.T.);
#42353=ORIENTED_EDGE('',*,*,#32257,.T.);
#42354=ORIENTED_EDGE('',*,*,#32253,.F.);
#42355=ORIENTED_EDGE('',*,*,#32258,.F.);
#42356=ORIENTED_EDGE('',*,*,#32259,.T.);
#42357=ORIENTED_EDGE('',*,*,#32260,.T.);
#42358=ORIENTED_EDGE('',*,*,#32256,.F.);
#42359=ORIENTED_EDGE('',*,*,#32261,.F.);
#42360=ORIENTED_EDGE('',*,*,#32262,.T.);
#42361=ORIENTED_EDGE('',*,*,#32263,.T.);
#42362=ORIENTED_EDGE('',*,*,#32259,.F.);
#42363=ORIENTED_EDGE('',*,*,#32264,.F.);
#42364=ORIENTED_EDGE('',*,*,#32265,.T.);
#42365=ORIENTED_EDGE('',*,*,#32266,.T.);
#42366=ORIENTED_EDGE('',*,*,#32262,.F.);
#42367=ORIENTED_EDGE('',*,*,#32267,.F.);
#42368=ORIENTED_EDGE('',*,*,#32268,.T.);
#42369=ORIENTED_EDGE('',*,*,#32269,.T.);
#42370=ORIENTED_EDGE('',*,*,#32265,.F.);
#42371=ORIENTED_EDGE('',*,*,#32270,.F.);
#42372=ORIENTED_EDGE('',*,*,#32271,.T.);
#42373=ORIENTED_EDGE('',*,*,#32272,.T.);
#42374=ORIENTED_EDGE('',*,*,#32268,.F.);
#42375=ORIENTED_EDGE('',*,*,#32273,.F.);
#42376=ORIENTED_EDGE('',*,*,#32274,.T.);
#42377=ORIENTED_EDGE('',*,*,#32275,.T.);
#42378=ORIENTED_EDGE('',*,*,#32271,.F.);
#42379=ORIENTED_EDGE('',*,*,#32276,.F.);
#42380=ORIENTED_EDGE('',*,*,#32277,.T.);
#42381=ORIENTED_EDGE('',*,*,#32278,.T.);
#42382=ORIENTED_EDGE('',*,*,#32274,.F.);
#42383=ORIENTED_EDGE('',*,*,#32279,.F.);
#42384=ORIENTED_EDGE('',*,*,#32280,.T.);
#42385=ORIENTED_EDGE('',*,*,#32281,.T.);
#42386=ORIENTED_EDGE('',*,*,#32277,.F.);
#42387=ORIENTED_EDGE('',*,*,#32282,.F.);
#42388=ORIENTED_EDGE('',*,*,#32230,.T.);
#42389=ORIENTED_EDGE('',*,*,#32283,.T.);
#42390=ORIENTED_EDGE('',*,*,#32280,.F.);
#42391=ORIENTED_EDGE('',*,*,#32283,.F.);
#42392=ORIENTED_EDGE('',*,*,#32229,.F.);
#42393=ORIENTED_EDGE('',*,*,#32233,.F.);
#42394=ORIENTED_EDGE('',*,*,#32236,.F.);
#42395=ORIENTED_EDGE('',*,*,#32239,.F.);
#42396=ORIENTED_EDGE('',*,*,#32242,.F.);
#42397=ORIENTED_EDGE('',*,*,#32245,.F.);
#42398=ORIENTED_EDGE('',*,*,#32248,.F.);
#42399=ORIENTED_EDGE('',*,*,#32251,.F.);
#42400=ORIENTED_EDGE('',*,*,#32254,.F.);
#42401=ORIENTED_EDGE('',*,*,#32257,.F.);
#42402=ORIENTED_EDGE('',*,*,#32260,.F.);
#42403=ORIENTED_EDGE('',*,*,#32263,.F.);
#42404=ORIENTED_EDGE('',*,*,#32266,.F.);
#42405=ORIENTED_EDGE('',*,*,#32269,.F.);
#42406=ORIENTED_EDGE('',*,*,#32272,.F.);
#42407=ORIENTED_EDGE('',*,*,#32275,.F.);
#42408=ORIENTED_EDGE('',*,*,#32278,.F.);
#42409=ORIENTED_EDGE('',*,*,#32281,.F.);
#42410=ORIENTED_EDGE('',*,*,#32226,.F.);
#42411=ORIENTED_EDGE('',*,*,#32202,.F.);
#42412=ORIENTED_EDGE('',*,*,#32206,.F.);
#42413=ORIENTED_EDGE('',*,*,#32209,.F.);
#42414=ORIENTED_EDGE('',*,*,#32212,.F.);
#42415=ORIENTED_EDGE('',*,*,#32215,.F.);
#42416=ORIENTED_EDGE('',*,*,#32218,.F.);
#42417=ORIENTED_EDGE('',*,*,#32221,.F.);
#42418=ORIENTED_EDGE('',*,*,#32224,.F.);
#42419=ORIENTED_EDGE('',*,*,#32200,.T.);
#42420=ORIENTED_EDGE('',*,*,#32225,.T.);
#42421=ORIENTED_EDGE('',*,*,#32222,.T.);
#42422=ORIENTED_EDGE('',*,*,#32219,.T.);
#42423=ORIENTED_EDGE('',*,*,#32216,.T.);
#42424=ORIENTED_EDGE('',*,*,#32213,.T.);
#42425=ORIENTED_EDGE('',*,*,#32210,.T.);
#42426=ORIENTED_EDGE('',*,*,#32207,.T.);
#42427=ORIENTED_EDGE('',*,*,#32204,.T.);
#42428=ORIENTED_EDGE('',*,*,#32140,.T.);
#42429=ORIENTED_EDGE('',*,*,#32162,.T.);
#42430=ORIENTED_EDGE('',*,*,#32159,.T.);
#42431=ORIENTED_EDGE('',*,*,#32156,.T.);
#42432=ORIENTED_EDGE('',*,*,#32153,.T.);
#42433=ORIENTED_EDGE('',*,*,#32150,.T.);
#42434=ORIENTED_EDGE('',*,*,#32147,.T.);
#42435=ORIENTED_EDGE('',*,*,#32144,.T.);
#42436=ORIENTED_EDGE('',*,*,#32284,.F.);
#42437=ORIENTED_EDGE('',*,*,#32285,.T.);
#42438=ORIENTED_EDGE('',*,*,#32286,.T.);
#42439=ORIENTED_EDGE('',*,*,#32287,.F.);
#42440=ORIENTED_EDGE('',*,*,#32288,.F.);
#42441=ORIENTED_EDGE('',*,*,#32289,.T.);
#42442=ORIENTED_EDGE('',*,*,#32290,.T.);
#42443=ORIENTED_EDGE('',*,*,#32285,.F.);
#42444=ORIENTED_EDGE('',*,*,#32291,.F.);
#42445=ORIENTED_EDGE('',*,*,#32292,.T.);
#42446=ORIENTED_EDGE('',*,*,#32293,.T.);
#42447=ORIENTED_EDGE('',*,*,#32289,.F.);
#42448=ORIENTED_EDGE('',*,*,#32294,.F.);
#42449=ORIENTED_EDGE('',*,*,#32295,.T.);
#42450=ORIENTED_EDGE('',*,*,#32296,.T.);
#42451=ORIENTED_EDGE('',*,*,#32292,.F.);
#42452=ORIENTED_EDGE('',*,*,#32297,.F.);
#42453=ORIENTED_EDGE('',*,*,#32298,.T.);
#42454=ORIENTED_EDGE('',*,*,#32299,.T.);
#42455=ORIENTED_EDGE('',*,*,#32295,.F.);
#42456=ORIENTED_EDGE('',*,*,#32300,.F.);
#42457=ORIENTED_EDGE('',*,*,#32301,.T.);
#42458=ORIENTED_EDGE('',*,*,#32302,.T.);
#42459=ORIENTED_EDGE('',*,*,#32298,.F.);
#42460=ORIENTED_EDGE('',*,*,#32303,.F.);
#42461=ORIENTED_EDGE('',*,*,#32304,.T.);
#42462=ORIENTED_EDGE('',*,*,#32305,.T.);
#42463=ORIENTED_EDGE('',*,*,#32301,.F.);
#42464=ORIENTED_EDGE('',*,*,#32306,.F.);
#42465=ORIENTED_EDGE('',*,*,#32287,.T.);
#42466=ORIENTED_EDGE('',*,*,#32307,.T.);
#42467=ORIENTED_EDGE('',*,*,#32304,.F.);
#42468=ORIENTED_EDGE('',*,*,#32308,.F.);
#42469=ORIENTED_EDGE('',*,*,#32309,.T.);
#42470=ORIENTED_EDGE('',*,*,#32310,.T.);
#42471=ORIENTED_EDGE('',*,*,#32311,.F.);
#42472=ORIENTED_EDGE('',*,*,#32312,.F.);
#42473=ORIENTED_EDGE('',*,*,#32313,.T.);
#42474=ORIENTED_EDGE('',*,*,#32314,.T.);
#42475=ORIENTED_EDGE('',*,*,#32309,.F.);
#42476=ORIENTED_EDGE('',*,*,#32315,.F.);
#42477=ORIENTED_EDGE('',*,*,#32316,.T.);
#42478=ORIENTED_EDGE('',*,*,#32317,.T.);
#42479=ORIENTED_EDGE('',*,*,#32313,.F.);
#42480=ORIENTED_EDGE('',*,*,#32318,.F.);
#42481=ORIENTED_EDGE('',*,*,#32319,.T.);
#42482=ORIENTED_EDGE('',*,*,#32320,.T.);
#42483=ORIENTED_EDGE('',*,*,#32316,.F.);
#42484=ORIENTED_EDGE('',*,*,#32321,.F.);
#42485=ORIENTED_EDGE('',*,*,#32322,.T.);
#42486=ORIENTED_EDGE('',*,*,#32323,.T.);
#42487=ORIENTED_EDGE('',*,*,#32319,.F.);
#42488=ORIENTED_EDGE('',*,*,#32324,.F.);
#42489=ORIENTED_EDGE('',*,*,#32325,.T.);
#42490=ORIENTED_EDGE('',*,*,#32326,.T.);
#42491=ORIENTED_EDGE('',*,*,#32322,.F.);
#42492=ORIENTED_EDGE('',*,*,#32327,.F.);
#42493=ORIENTED_EDGE('',*,*,#32328,.T.);
#42494=ORIENTED_EDGE('',*,*,#32329,.T.);
#42495=ORIENTED_EDGE('',*,*,#32325,.F.);
#42496=ORIENTED_EDGE('',*,*,#32330,.F.);
#42497=ORIENTED_EDGE('',*,*,#32331,.T.);
#42498=ORIENTED_EDGE('',*,*,#32332,.T.);
#42499=ORIENTED_EDGE('',*,*,#32328,.F.);
#42500=ORIENTED_EDGE('',*,*,#32333,.F.);
#42501=ORIENTED_EDGE('',*,*,#32334,.T.);
#42502=ORIENTED_EDGE('',*,*,#32335,.T.);
#42503=ORIENTED_EDGE('',*,*,#32331,.F.);
#42504=ORIENTED_EDGE('',*,*,#32336,.F.);
#42505=ORIENTED_EDGE('',*,*,#32337,.T.);
#42506=ORIENTED_EDGE('',*,*,#32338,.T.);
#42507=ORIENTED_EDGE('',*,*,#32334,.F.);
#42508=ORIENTED_EDGE('',*,*,#32339,.F.);
#42509=ORIENTED_EDGE('',*,*,#32340,.T.);
#42510=ORIENTED_EDGE('',*,*,#32341,.T.);
#42511=ORIENTED_EDGE('',*,*,#32337,.F.);
#42512=ORIENTED_EDGE('',*,*,#32342,.F.);
#42513=ORIENTED_EDGE('',*,*,#32311,.T.);
#42514=ORIENTED_EDGE('',*,*,#32343,.T.);
#42515=ORIENTED_EDGE('',*,*,#32340,.F.);
#42516=ORIENTED_EDGE('',*,*,#32343,.F.);
#42517=ORIENTED_EDGE('',*,*,#32310,.F.);
#42518=ORIENTED_EDGE('',*,*,#32314,.F.);
#42519=ORIENTED_EDGE('',*,*,#32317,.F.);
#42520=ORIENTED_EDGE('',*,*,#32320,.F.);
#42521=ORIENTED_EDGE('',*,*,#32323,.F.);
#42522=ORIENTED_EDGE('',*,*,#32326,.F.);
#42523=ORIENTED_EDGE('',*,*,#32329,.F.);
#42524=ORIENTED_EDGE('',*,*,#32332,.F.);
#42525=ORIENTED_EDGE('',*,*,#32335,.F.);
#42526=ORIENTED_EDGE('',*,*,#32338,.F.);
#42527=ORIENTED_EDGE('',*,*,#32341,.F.);
#42528=ORIENTED_EDGE('',*,*,#32307,.F.);
#42529=ORIENTED_EDGE('',*,*,#32286,.F.);
#42530=ORIENTED_EDGE('',*,*,#32290,.F.);
#42531=ORIENTED_EDGE('',*,*,#32293,.F.);
#42532=ORIENTED_EDGE('',*,*,#32296,.F.);
#42533=ORIENTED_EDGE('',*,*,#32299,.F.);
#42534=ORIENTED_EDGE('',*,*,#32302,.F.);
#42535=ORIENTED_EDGE('',*,*,#32305,.F.);
#42536=ORIENTED_EDGE('',*,*,#32344,.F.);
#42537=ORIENTED_EDGE('',*,*,#32345,.T.);
#42538=ORIENTED_EDGE('',*,*,#32346,.T.);
#42539=ORIENTED_EDGE('',*,*,#32347,.F.);
#42540=ORIENTED_EDGE('',*,*,#32348,.F.);
#42541=ORIENTED_EDGE('',*,*,#32349,.T.);
#42542=ORIENTED_EDGE('',*,*,#32350,.T.);
#42543=ORIENTED_EDGE('',*,*,#32345,.F.);
#42544=ORIENTED_EDGE('',*,*,#32351,.F.);
#42545=ORIENTED_EDGE('',*,*,#32352,.T.);
#42546=ORIENTED_EDGE('',*,*,#32353,.T.);
#42547=ORIENTED_EDGE('',*,*,#32349,.F.);
#42548=ORIENTED_EDGE('',*,*,#32354,.F.);
#42549=ORIENTED_EDGE('',*,*,#32355,.T.);
#42550=ORIENTED_EDGE('',*,*,#32356,.T.);
#42551=ORIENTED_EDGE('',*,*,#32352,.F.);
#42552=ORIENTED_EDGE('',*,*,#32357,.F.);
#42553=ORIENTED_EDGE('',*,*,#32358,.T.);
#42554=ORIENTED_EDGE('',*,*,#32359,.T.);
#42555=ORIENTED_EDGE('',*,*,#32355,.F.);
#42556=ORIENTED_EDGE('',*,*,#32360,.F.);
#42557=ORIENTED_EDGE('',*,*,#32361,.T.);
#42558=ORIENTED_EDGE('',*,*,#32362,.T.);
#42559=ORIENTED_EDGE('',*,*,#32358,.F.);
#42560=ORIENTED_EDGE('',*,*,#32363,.F.);
#42561=ORIENTED_EDGE('',*,*,#32364,.T.);
#42562=ORIENTED_EDGE('',*,*,#32365,.T.);
#42563=ORIENTED_EDGE('',*,*,#32361,.F.);
#42564=ORIENTED_EDGE('',*,*,#32366,.F.);
#42565=ORIENTED_EDGE('',*,*,#32367,.T.);
#42566=ORIENTED_EDGE('',*,*,#32368,.T.);
#42567=ORIENTED_EDGE('',*,*,#32364,.F.);
#42568=ORIENTED_EDGE('',*,*,#32369,.F.);
#42569=ORIENTED_EDGE('',*,*,#32370,.T.);
#42570=ORIENTED_EDGE('',*,*,#32371,.T.);
#42571=ORIENTED_EDGE('',*,*,#32367,.F.);
#42572=ORIENTED_EDGE('',*,*,#32372,.F.);
#42573=ORIENTED_EDGE('',*,*,#32373,.T.);
#42574=ORIENTED_EDGE('',*,*,#32374,.T.);
#42575=ORIENTED_EDGE('',*,*,#32370,.F.);
#42576=ORIENTED_EDGE('',*,*,#32375,.F.);
#42577=ORIENTED_EDGE('',*,*,#32347,.T.);
#42578=ORIENTED_EDGE('',*,*,#32376,.T.);
#42579=ORIENTED_EDGE('',*,*,#32373,.F.);
#42580=ORIENTED_EDGE('',*,*,#32376,.F.);
#42581=ORIENTED_EDGE('',*,*,#32346,.F.);
#42582=ORIENTED_EDGE('',*,*,#32350,.F.);
#42583=ORIENTED_EDGE('',*,*,#32353,.F.);
#42584=ORIENTED_EDGE('',*,*,#32356,.F.);
#42585=ORIENTED_EDGE('',*,*,#32359,.F.);
#42586=ORIENTED_EDGE('',*,*,#32362,.F.);
#42587=ORIENTED_EDGE('',*,*,#32365,.F.);
#42588=ORIENTED_EDGE('',*,*,#32368,.F.);
#42589=ORIENTED_EDGE('',*,*,#32371,.F.);
#42590=ORIENTED_EDGE('',*,*,#32374,.F.);
#42591=ORIENTED_EDGE('',*,*,#32284,.T.);
#42592=ORIENTED_EDGE('',*,*,#32306,.T.);
#42593=ORIENTED_EDGE('',*,*,#32303,.T.);
#42594=ORIENTED_EDGE('',*,*,#32300,.T.);
#42595=ORIENTED_EDGE('',*,*,#32297,.T.);
#42596=ORIENTED_EDGE('',*,*,#32294,.T.);
#42597=ORIENTED_EDGE('',*,*,#32291,.T.);
#42598=ORIENTED_EDGE('',*,*,#32288,.T.);
#42599=ORIENTED_EDGE('',*,*,#32377,.F.);
#42600=ORIENTED_EDGE('',*,*,#32378,.T.);
#42601=ORIENTED_EDGE('',*,*,#32379,.T.);
#42602=ORIENTED_EDGE('',*,*,#32380,.F.);
#42603=ORIENTED_EDGE('',*,*,#32381,.F.);
#42604=ORIENTED_EDGE('',*,*,#32382,.T.);
#42605=ORIENTED_EDGE('',*,*,#32383,.T.);
#42606=ORIENTED_EDGE('',*,*,#32378,.F.);
#42607=ORIENTED_EDGE('',*,*,#32384,.F.);
#42608=ORIENTED_EDGE('',*,*,#32385,.T.);
#42609=ORIENTED_EDGE('',*,*,#32386,.T.);
#42610=ORIENTED_EDGE('',*,*,#32382,.F.);
#42611=ORIENTED_EDGE('',*,*,#32387,.F.);
#42612=ORIENTED_EDGE('',*,*,#32388,.T.);
#42613=ORIENTED_EDGE('',*,*,#32389,.T.);
#42614=ORIENTED_EDGE('',*,*,#32385,.F.);
#42615=ORIENTED_EDGE('',*,*,#32390,.F.);
#42616=ORIENTED_EDGE('',*,*,#32391,.T.);
#42617=ORIENTED_EDGE('',*,*,#32392,.T.);
#42618=ORIENTED_EDGE('',*,*,#32388,.F.);
#42619=ORIENTED_EDGE('',*,*,#32393,.F.);
#42620=ORIENTED_EDGE('',*,*,#32394,.T.);
#42621=ORIENTED_EDGE('',*,*,#32395,.T.);
#42622=ORIENTED_EDGE('',*,*,#32391,.F.);
#42623=ORIENTED_EDGE('',*,*,#32396,.F.);
#42624=ORIENTED_EDGE('',*,*,#32397,.T.);
#42625=ORIENTED_EDGE('',*,*,#32398,.T.);
#42626=ORIENTED_EDGE('',*,*,#32394,.F.);
#42627=ORIENTED_EDGE('',*,*,#32399,.F.);
#42628=ORIENTED_EDGE('',*,*,#32380,.T.);
#42629=ORIENTED_EDGE('',*,*,#32400,.T.);
#42630=ORIENTED_EDGE('',*,*,#32397,.F.);
#42631=ORIENTED_EDGE('',*,*,#32401,.F.);
#42632=ORIENTED_EDGE('',*,*,#32402,.T.);
#42633=ORIENTED_EDGE('',*,*,#32403,.T.);
#42634=ORIENTED_EDGE('',*,*,#32404,.F.);
#42635=ORIENTED_EDGE('',*,*,#32405,.F.);
#42636=ORIENTED_EDGE('',*,*,#32406,.T.);
#42637=ORIENTED_EDGE('',*,*,#32407,.T.);
#42638=ORIENTED_EDGE('',*,*,#32402,.F.);
#42639=ORIENTED_EDGE('',*,*,#32408,.F.);
#42640=ORIENTED_EDGE('',*,*,#32409,.T.);
#42641=ORIENTED_EDGE('',*,*,#32410,.T.);
#42642=ORIENTED_EDGE('',*,*,#32406,.F.);
#42643=ORIENTED_EDGE('',*,*,#32411,.F.);
#42644=ORIENTED_EDGE('',*,*,#32412,.T.);
#42645=ORIENTED_EDGE('',*,*,#32413,.T.);
#42646=ORIENTED_EDGE('',*,*,#32409,.F.);
#42647=ORIENTED_EDGE('',*,*,#32414,.F.);
#42648=ORIENTED_EDGE('',*,*,#32415,.T.);
#42649=ORIENTED_EDGE('',*,*,#32416,.T.);
#42650=ORIENTED_EDGE('',*,*,#32412,.F.);
#42651=ORIENTED_EDGE('',*,*,#32417,.F.);
#42652=ORIENTED_EDGE('',*,*,#32418,.T.);
#42653=ORIENTED_EDGE('',*,*,#32419,.T.);
#42654=ORIENTED_EDGE('',*,*,#32415,.F.);
#42655=ORIENTED_EDGE('',*,*,#32420,.F.);
#42656=ORIENTED_EDGE('',*,*,#32421,.T.);
#42657=ORIENTED_EDGE('',*,*,#32422,.T.);
#42658=ORIENTED_EDGE('',*,*,#32418,.F.);
#42659=ORIENTED_EDGE('',*,*,#32423,.F.);
#42660=ORIENTED_EDGE('',*,*,#32424,.T.);
#42661=ORIENTED_EDGE('',*,*,#32425,.T.);
#42662=ORIENTED_EDGE('',*,*,#32421,.F.);
#42663=ORIENTED_EDGE('',*,*,#32426,.F.);
#42664=ORIENTED_EDGE('',*,*,#32427,.T.);
#42665=ORIENTED_EDGE('',*,*,#32428,.T.);
#42666=ORIENTED_EDGE('',*,*,#32424,.F.);
#42667=ORIENTED_EDGE('',*,*,#32429,.F.);
#42668=ORIENTED_EDGE('',*,*,#32430,.T.);
#42669=ORIENTED_EDGE('',*,*,#32431,.T.);
#42670=ORIENTED_EDGE('',*,*,#32427,.F.);
#42671=ORIENTED_EDGE('',*,*,#32432,.F.);
#42672=ORIENTED_EDGE('',*,*,#32433,.T.);
#42673=ORIENTED_EDGE('',*,*,#32434,.T.);
#42674=ORIENTED_EDGE('',*,*,#32430,.F.);
#42675=ORIENTED_EDGE('',*,*,#32435,.F.);
#42676=ORIENTED_EDGE('',*,*,#32404,.T.);
#42677=ORIENTED_EDGE('',*,*,#32436,.T.);
#42678=ORIENTED_EDGE('',*,*,#32433,.F.);
#42679=ORIENTED_EDGE('',*,*,#32436,.F.);
#42680=ORIENTED_EDGE('',*,*,#32403,.F.);
#42681=ORIENTED_EDGE('',*,*,#32407,.F.);
#42682=ORIENTED_EDGE('',*,*,#32410,.F.);
#42683=ORIENTED_EDGE('',*,*,#32413,.F.);
#42684=ORIENTED_EDGE('',*,*,#32416,.F.);
#42685=ORIENTED_EDGE('',*,*,#32419,.F.);
#42686=ORIENTED_EDGE('',*,*,#32422,.F.);
#42687=ORIENTED_EDGE('',*,*,#32425,.F.);
#42688=ORIENTED_EDGE('',*,*,#32428,.F.);
#42689=ORIENTED_EDGE('',*,*,#32431,.F.);
#42690=ORIENTED_EDGE('',*,*,#32434,.F.);
#42691=ORIENTED_EDGE('',*,*,#32400,.F.);
#42692=ORIENTED_EDGE('',*,*,#32379,.F.);
#42693=ORIENTED_EDGE('',*,*,#32383,.F.);
#42694=ORIENTED_EDGE('',*,*,#32386,.F.);
#42695=ORIENTED_EDGE('',*,*,#32389,.F.);
#42696=ORIENTED_EDGE('',*,*,#32392,.F.);
#42697=ORIENTED_EDGE('',*,*,#32395,.F.);
#42698=ORIENTED_EDGE('',*,*,#32398,.F.);
#42699=ORIENTED_EDGE('',*,*,#32437,.F.);
#42700=ORIENTED_EDGE('',*,*,#32438,.T.);
#42701=ORIENTED_EDGE('',*,*,#32439,.T.);
#42702=ORIENTED_EDGE('',*,*,#32440,.F.);
#42703=ORIENTED_EDGE('',*,*,#32441,.F.);
#42704=ORIENTED_EDGE('',*,*,#32442,.T.);
#42705=ORIENTED_EDGE('',*,*,#32443,.T.);
#42706=ORIENTED_EDGE('',*,*,#32438,.F.);
#42707=ORIENTED_EDGE('',*,*,#32444,.F.);
#42708=ORIENTED_EDGE('',*,*,#32445,.T.);
#42709=ORIENTED_EDGE('',*,*,#32446,.T.);
#42710=ORIENTED_EDGE('',*,*,#32442,.F.);
#42711=ORIENTED_EDGE('',*,*,#32447,.F.);
#42712=ORIENTED_EDGE('',*,*,#32448,.T.);
#42713=ORIENTED_EDGE('',*,*,#32449,.T.);
#42714=ORIENTED_EDGE('',*,*,#32445,.F.);
#42715=ORIENTED_EDGE('',*,*,#32450,.F.);
#42716=ORIENTED_EDGE('',*,*,#32451,.T.);
#42717=ORIENTED_EDGE('',*,*,#32452,.T.);
#42718=ORIENTED_EDGE('',*,*,#32448,.F.);
#42719=ORIENTED_EDGE('',*,*,#32453,.F.);
#42720=ORIENTED_EDGE('',*,*,#32454,.T.);
#42721=ORIENTED_EDGE('',*,*,#32455,.T.);
#42722=ORIENTED_EDGE('',*,*,#32451,.F.);
#42723=ORIENTED_EDGE('',*,*,#32456,.F.);
#42724=ORIENTED_EDGE('',*,*,#32457,.T.);
#42725=ORIENTED_EDGE('',*,*,#32458,.T.);
#42726=ORIENTED_EDGE('',*,*,#32454,.F.);
#42727=ORIENTED_EDGE('',*,*,#32459,.F.);
#42728=ORIENTED_EDGE('',*,*,#32440,.T.);
#42729=ORIENTED_EDGE('',*,*,#32460,.T.);
#42730=ORIENTED_EDGE('',*,*,#32457,.F.);
#42731=ORIENTED_EDGE('',*,*,#32461,.F.);
#42732=ORIENTED_EDGE('',*,*,#32462,.T.);
#42733=ORIENTED_EDGE('',*,*,#32463,.T.);
#42734=ORIENTED_EDGE('',*,*,#32464,.F.);
#42735=ORIENTED_EDGE('',*,*,#32465,.F.);
#42736=ORIENTED_EDGE('',*,*,#32466,.T.);
#42737=ORIENTED_EDGE('',*,*,#32467,.T.);
#42738=ORIENTED_EDGE('',*,*,#32462,.F.);
#42739=ORIENTED_EDGE('',*,*,#32468,.F.);
#42740=ORIENTED_EDGE('',*,*,#32469,.T.);
#42741=ORIENTED_EDGE('',*,*,#32470,.T.);
#42742=ORIENTED_EDGE('',*,*,#32466,.F.);
#42743=ORIENTED_EDGE('',*,*,#32471,.F.);
#42744=ORIENTED_EDGE('',*,*,#32472,.T.);
#42745=ORIENTED_EDGE('',*,*,#32473,.T.);
#42746=ORIENTED_EDGE('',*,*,#32469,.F.);
#42747=ORIENTED_EDGE('',*,*,#32474,.F.);
#42748=ORIENTED_EDGE('',*,*,#32475,.T.);
#42749=ORIENTED_EDGE('',*,*,#32476,.T.);
#42750=ORIENTED_EDGE('',*,*,#32472,.F.);
#42751=ORIENTED_EDGE('',*,*,#32477,.F.);
#42752=ORIENTED_EDGE('',*,*,#32478,.T.);
#42753=ORIENTED_EDGE('',*,*,#32479,.T.);
#42754=ORIENTED_EDGE('',*,*,#32475,.F.);
#42755=ORIENTED_EDGE('',*,*,#32480,.F.);
#42756=ORIENTED_EDGE('',*,*,#32481,.T.);
#42757=ORIENTED_EDGE('',*,*,#32482,.T.);
#42758=ORIENTED_EDGE('',*,*,#32478,.F.);
#42759=ORIENTED_EDGE('',*,*,#32483,.F.);
#42760=ORIENTED_EDGE('',*,*,#32484,.T.);
#42761=ORIENTED_EDGE('',*,*,#32485,.T.);
#42762=ORIENTED_EDGE('',*,*,#32481,.F.);
#42763=ORIENTED_EDGE('',*,*,#32486,.F.);
#42764=ORIENTED_EDGE('',*,*,#32464,.T.);
#42765=ORIENTED_EDGE('',*,*,#32487,.T.);
#42766=ORIENTED_EDGE('',*,*,#32484,.F.);
#42767=ORIENTED_EDGE('',*,*,#32488,.F.);
#42768=ORIENTED_EDGE('',*,*,#32489,.T.);
#42769=ORIENTED_EDGE('',*,*,#32490,.T.);
#42770=ORIENTED_EDGE('',*,*,#32491,.F.);
#42771=ORIENTED_EDGE('',*,*,#32492,.F.);
#42772=ORIENTED_EDGE('',*,*,#32493,.T.);
#42773=ORIENTED_EDGE('',*,*,#32494,.T.);
#42774=ORIENTED_EDGE('',*,*,#32489,.F.);
#42775=ORIENTED_EDGE('',*,*,#32495,.F.);
#42776=ORIENTED_EDGE('',*,*,#32496,.T.);
#42777=ORIENTED_EDGE('',*,*,#32497,.T.);
#42778=ORIENTED_EDGE('',*,*,#32493,.F.);
#42779=ORIENTED_EDGE('',*,*,#32498,.F.);
#42780=ORIENTED_EDGE('',*,*,#32499,.T.);
#42781=ORIENTED_EDGE('',*,*,#32500,.T.);
#42782=ORIENTED_EDGE('',*,*,#32496,.F.);
#42783=ORIENTED_EDGE('',*,*,#32501,.F.);
#42784=ORIENTED_EDGE('',*,*,#32502,.T.);
#42785=ORIENTED_EDGE('',*,*,#32503,.T.);
#42786=ORIENTED_EDGE('',*,*,#32499,.F.);
#42787=ORIENTED_EDGE('',*,*,#32504,.F.);
#42788=ORIENTED_EDGE('',*,*,#32505,.T.);
#42789=ORIENTED_EDGE('',*,*,#32506,.T.);
#42790=ORIENTED_EDGE('',*,*,#32502,.F.);
#42791=ORIENTED_EDGE('',*,*,#32507,.F.);
#42792=ORIENTED_EDGE('',*,*,#32508,.T.);
#42793=ORIENTED_EDGE('',*,*,#32509,.T.);
#42794=ORIENTED_EDGE('',*,*,#32505,.F.);
#42795=ORIENTED_EDGE('',*,*,#32510,.F.);
#42796=ORIENTED_EDGE('',*,*,#32511,.T.);
#42797=ORIENTED_EDGE('',*,*,#32512,.T.);
#42798=ORIENTED_EDGE('',*,*,#32508,.F.);
#42799=ORIENTED_EDGE('',*,*,#32513,.F.);
#42800=ORIENTED_EDGE('',*,*,#32514,.T.);
#42801=ORIENTED_EDGE('',*,*,#32515,.T.);
#42802=ORIENTED_EDGE('',*,*,#32511,.F.);
#42803=ORIENTED_EDGE('',*,*,#32516,.F.);
#42804=ORIENTED_EDGE('',*,*,#32517,.T.);
#42805=ORIENTED_EDGE('',*,*,#32518,.T.);
#42806=ORIENTED_EDGE('',*,*,#32514,.F.);
#42807=ORIENTED_EDGE('',*,*,#32519,.F.);
#42808=ORIENTED_EDGE('',*,*,#32520,.T.);
#42809=ORIENTED_EDGE('',*,*,#32521,.T.);
#42810=ORIENTED_EDGE('',*,*,#32517,.F.);
#42811=ORIENTED_EDGE('',*,*,#32522,.F.);
#42812=ORIENTED_EDGE('',*,*,#32523,.T.);
#42813=ORIENTED_EDGE('',*,*,#32524,.T.);
#42814=ORIENTED_EDGE('',*,*,#32520,.F.);
#42815=ORIENTED_EDGE('',*,*,#32525,.F.);
#42816=ORIENTED_EDGE('',*,*,#32526,.T.);
#42817=ORIENTED_EDGE('',*,*,#32527,.T.);
#42818=ORIENTED_EDGE('',*,*,#32523,.F.);
#42819=ORIENTED_EDGE('',*,*,#32528,.F.);
#42820=ORIENTED_EDGE('',*,*,#32529,.T.);
#42821=ORIENTED_EDGE('',*,*,#32530,.T.);
#42822=ORIENTED_EDGE('',*,*,#32526,.F.);
#42823=ORIENTED_EDGE('',*,*,#32531,.F.);
#42824=ORIENTED_EDGE('',*,*,#32532,.T.);
#42825=ORIENTED_EDGE('',*,*,#32533,.T.);
#42826=ORIENTED_EDGE('',*,*,#32529,.F.);
#42827=ORIENTED_EDGE('',*,*,#32534,.F.);
#42828=ORIENTED_EDGE('',*,*,#32491,.T.);
#42829=ORIENTED_EDGE('',*,*,#32535,.T.);
#42830=ORIENTED_EDGE('',*,*,#32532,.F.);
#42831=ORIENTED_EDGE('',*,*,#32535,.F.);
#42832=ORIENTED_EDGE('',*,*,#32490,.F.);
#42833=ORIENTED_EDGE('',*,*,#32494,.F.);
#42834=ORIENTED_EDGE('',*,*,#32497,.F.);
#42835=ORIENTED_EDGE('',*,*,#32500,.F.);
#42836=ORIENTED_EDGE('',*,*,#32503,.F.);
#42837=ORIENTED_EDGE('',*,*,#32506,.F.);
#42838=ORIENTED_EDGE('',*,*,#32509,.F.);
#42839=ORIENTED_EDGE('',*,*,#32512,.F.);
#42840=ORIENTED_EDGE('',*,*,#32515,.F.);
#42841=ORIENTED_EDGE('',*,*,#32518,.F.);
#42842=ORIENTED_EDGE('',*,*,#32521,.F.);
#42843=ORIENTED_EDGE('',*,*,#32524,.F.);
#42844=ORIENTED_EDGE('',*,*,#32527,.F.);
#42845=ORIENTED_EDGE('',*,*,#32530,.F.);
#42846=ORIENTED_EDGE('',*,*,#32533,.F.);
#42847=ORIENTED_EDGE('',*,*,#32487,.F.);
#42848=ORIENTED_EDGE('',*,*,#32463,.F.);
#42849=ORIENTED_EDGE('',*,*,#32467,.F.);
#42850=ORIENTED_EDGE('',*,*,#32470,.F.);
#42851=ORIENTED_EDGE('',*,*,#32473,.F.);
#42852=ORIENTED_EDGE('',*,*,#32476,.F.);
#42853=ORIENTED_EDGE('',*,*,#32479,.F.);
#42854=ORIENTED_EDGE('',*,*,#32482,.F.);
#42855=ORIENTED_EDGE('',*,*,#32485,.F.);
#42856=ORIENTED_EDGE('',*,*,#32460,.F.);
#42857=ORIENTED_EDGE('',*,*,#32439,.F.);
#42858=ORIENTED_EDGE('',*,*,#32443,.F.);
#42859=ORIENTED_EDGE('',*,*,#32446,.F.);
#42860=ORIENTED_EDGE('',*,*,#32449,.F.);
#42861=ORIENTED_EDGE('',*,*,#32452,.F.);
#42862=ORIENTED_EDGE('',*,*,#32455,.F.);
#42863=ORIENTED_EDGE('',*,*,#32458,.F.);
#42864=ORIENTED_EDGE('',*,*,#32461,.T.);
#42865=ORIENTED_EDGE('',*,*,#32486,.T.);
#42866=ORIENTED_EDGE('',*,*,#32483,.T.);
#42867=ORIENTED_EDGE('',*,*,#32480,.T.);
#42868=ORIENTED_EDGE('',*,*,#32477,.T.);
#42869=ORIENTED_EDGE('',*,*,#32474,.T.);
#42870=ORIENTED_EDGE('',*,*,#32471,.T.);
#42871=ORIENTED_EDGE('',*,*,#32468,.T.);
#42872=ORIENTED_EDGE('',*,*,#32465,.T.);
#42873=ORIENTED_EDGE('',*,*,#32437,.T.);
#42874=ORIENTED_EDGE('',*,*,#32459,.T.);
#42875=ORIENTED_EDGE('',*,*,#32456,.T.);
#42876=ORIENTED_EDGE('',*,*,#32453,.T.);
#42877=ORIENTED_EDGE('',*,*,#32450,.T.);
#42878=ORIENTED_EDGE('',*,*,#32447,.T.);
#42879=ORIENTED_EDGE('',*,*,#32444,.T.);
#42880=ORIENTED_EDGE('',*,*,#32441,.T.);
#42881=ORIENTED_EDGE('',*,*,#32377,.T.);
#42882=ORIENTED_EDGE('',*,*,#32399,.T.);
#42883=ORIENTED_EDGE('',*,*,#32396,.T.);
#42884=ORIENTED_EDGE('',*,*,#32393,.T.);
#42885=ORIENTED_EDGE('',*,*,#32390,.T.);
#42886=ORIENTED_EDGE('',*,*,#32387,.T.);
#42887=ORIENTED_EDGE('',*,*,#32384,.T.);
#42888=ORIENTED_EDGE('',*,*,#32381,.T.);
#42889=ORIENTED_EDGE('',*,*,#32536,.F.);
#42890=ORIENTED_EDGE('',*,*,#32537,.T.);
#42891=ORIENTED_EDGE('',*,*,#32538,.T.);
#42892=ORIENTED_EDGE('',*,*,#32539,.F.);
#42893=ORIENTED_EDGE('',*,*,#32540,.F.);
#42894=ORIENTED_EDGE('',*,*,#32541,.T.);
#42895=ORIENTED_EDGE('',*,*,#32542,.T.);
#42896=ORIENTED_EDGE('',*,*,#32537,.F.);
#42897=ORIENTED_EDGE('',*,*,#32543,.F.);
#42898=ORIENTED_EDGE('',*,*,#32544,.T.);
#42899=ORIENTED_EDGE('',*,*,#32545,.T.);
#42900=ORIENTED_EDGE('',*,*,#32541,.F.);
#42901=ORIENTED_EDGE('',*,*,#32546,.F.);
#42902=ORIENTED_EDGE('',*,*,#32547,.T.);
#42903=ORIENTED_EDGE('',*,*,#32548,.T.);
#42904=ORIENTED_EDGE('',*,*,#32544,.F.);
#42905=ORIENTED_EDGE('',*,*,#32549,.F.);
#42906=ORIENTED_EDGE('',*,*,#32550,.T.);
#42907=ORIENTED_EDGE('',*,*,#32551,.T.);
#42908=ORIENTED_EDGE('',*,*,#32547,.F.);
#42909=ORIENTED_EDGE('',*,*,#32552,.F.);
#42910=ORIENTED_EDGE('',*,*,#32553,.T.);
#42911=ORIENTED_EDGE('',*,*,#32554,.T.);
#42912=ORIENTED_EDGE('',*,*,#32550,.F.);
#42913=ORIENTED_EDGE('',*,*,#32555,.F.);
#42914=ORIENTED_EDGE('',*,*,#32556,.T.);
#42915=ORIENTED_EDGE('',*,*,#32557,.T.);
#42916=ORIENTED_EDGE('',*,*,#32553,.F.);
#42917=ORIENTED_EDGE('',*,*,#32558,.F.);
#42918=ORIENTED_EDGE('',*,*,#32539,.T.);
#42919=ORIENTED_EDGE('',*,*,#32559,.T.);
#42920=ORIENTED_EDGE('',*,*,#32556,.F.);
#42921=ORIENTED_EDGE('',*,*,#32560,.F.);
#42922=ORIENTED_EDGE('',*,*,#32561,.T.);
#42923=ORIENTED_EDGE('',*,*,#32562,.T.);
#42924=ORIENTED_EDGE('',*,*,#32563,.F.);
#42925=ORIENTED_EDGE('',*,*,#32564,.F.);
#42926=ORIENTED_EDGE('',*,*,#32565,.T.);
#42927=ORIENTED_EDGE('',*,*,#32566,.T.);
#42928=ORIENTED_EDGE('',*,*,#32561,.F.);
#42929=ORIENTED_EDGE('',*,*,#32567,.F.);
#42930=ORIENTED_EDGE('',*,*,#32568,.T.);
#42931=ORIENTED_EDGE('',*,*,#32569,.T.);
#42932=ORIENTED_EDGE('',*,*,#32565,.F.);
#42933=ORIENTED_EDGE('',*,*,#32570,.F.);
#42934=ORIENTED_EDGE('',*,*,#32571,.T.);
#42935=ORIENTED_EDGE('',*,*,#32572,.T.);
#42936=ORIENTED_EDGE('',*,*,#32568,.F.);
#42937=ORIENTED_EDGE('',*,*,#32573,.F.);
#42938=ORIENTED_EDGE('',*,*,#32574,.T.);
#42939=ORIENTED_EDGE('',*,*,#32575,.T.);
#42940=ORIENTED_EDGE('',*,*,#32571,.F.);
#42941=ORIENTED_EDGE('',*,*,#32576,.F.);
#42942=ORIENTED_EDGE('',*,*,#32577,.T.);
#42943=ORIENTED_EDGE('',*,*,#32578,.T.);
#42944=ORIENTED_EDGE('',*,*,#32574,.F.);
#42945=ORIENTED_EDGE('',*,*,#32579,.F.);
#42946=ORIENTED_EDGE('',*,*,#32580,.T.);
#42947=ORIENTED_EDGE('',*,*,#32581,.T.);
#42948=ORIENTED_EDGE('',*,*,#32577,.F.);
#42949=ORIENTED_EDGE('',*,*,#32582,.F.);
#42950=ORIENTED_EDGE('',*,*,#32583,.T.);
#42951=ORIENTED_EDGE('',*,*,#32584,.T.);
#42952=ORIENTED_EDGE('',*,*,#32580,.F.);
#42953=ORIENTED_EDGE('',*,*,#32585,.F.);
#42954=ORIENTED_EDGE('',*,*,#32586,.T.);
#42955=ORIENTED_EDGE('',*,*,#32587,.T.);
#42956=ORIENTED_EDGE('',*,*,#32583,.F.);
#42957=ORIENTED_EDGE('',*,*,#32588,.F.);
#42958=ORIENTED_EDGE('',*,*,#32589,.T.);
#42959=ORIENTED_EDGE('',*,*,#32590,.T.);
#42960=ORIENTED_EDGE('',*,*,#32586,.F.);
#42961=ORIENTED_EDGE('',*,*,#32591,.F.);
#42962=ORIENTED_EDGE('',*,*,#32592,.T.);
#42963=ORIENTED_EDGE('',*,*,#32593,.T.);
#42964=ORIENTED_EDGE('',*,*,#32589,.F.);
#42965=ORIENTED_EDGE('',*,*,#32594,.F.);
#42966=ORIENTED_EDGE('',*,*,#32563,.T.);
#42967=ORIENTED_EDGE('',*,*,#32595,.T.);
#42968=ORIENTED_EDGE('',*,*,#32592,.F.);
#42969=ORIENTED_EDGE('',*,*,#32595,.F.);
#42970=ORIENTED_EDGE('',*,*,#32562,.F.);
#42971=ORIENTED_EDGE('',*,*,#32566,.F.);
#42972=ORIENTED_EDGE('',*,*,#32569,.F.);
#42973=ORIENTED_EDGE('',*,*,#32572,.F.);
#42974=ORIENTED_EDGE('',*,*,#32575,.F.);
#42975=ORIENTED_EDGE('',*,*,#32578,.F.);
#42976=ORIENTED_EDGE('',*,*,#32581,.F.);
#42977=ORIENTED_EDGE('',*,*,#32584,.F.);
#42978=ORIENTED_EDGE('',*,*,#32587,.F.);
#42979=ORIENTED_EDGE('',*,*,#32590,.F.);
#42980=ORIENTED_EDGE('',*,*,#32593,.F.);
#42981=ORIENTED_EDGE('',*,*,#32559,.F.);
#42982=ORIENTED_EDGE('',*,*,#32538,.F.);
#42983=ORIENTED_EDGE('',*,*,#32542,.F.);
#42984=ORIENTED_EDGE('',*,*,#32545,.F.);
#42985=ORIENTED_EDGE('',*,*,#32548,.F.);
#42986=ORIENTED_EDGE('',*,*,#32551,.F.);
#42987=ORIENTED_EDGE('',*,*,#32554,.F.);
#42988=ORIENTED_EDGE('',*,*,#32557,.F.);
#42989=ORIENTED_EDGE('',*,*,#32596,.F.);
#42990=ORIENTED_EDGE('',*,*,#32597,.T.);
#42991=ORIENTED_EDGE('',*,*,#32598,.T.);
#42992=ORIENTED_EDGE('',*,*,#32599,.F.);
#42993=ORIENTED_EDGE('',*,*,#32600,.F.);
#42994=ORIENTED_EDGE('',*,*,#32601,.T.);
#42995=ORIENTED_EDGE('',*,*,#32602,.T.);
#42996=ORIENTED_EDGE('',*,*,#32597,.F.);
#42997=ORIENTED_EDGE('',*,*,#32603,.F.);
#42998=ORIENTED_EDGE('',*,*,#32604,.T.);
#42999=ORIENTED_EDGE('',*,*,#32605,.T.);
#43000=ORIENTED_EDGE('',*,*,#32601,.F.);
#43001=ORIENTED_EDGE('',*,*,#32606,.F.);
#43002=ORIENTED_EDGE('',*,*,#32607,.T.);
#43003=ORIENTED_EDGE('',*,*,#32608,.T.);
#43004=ORIENTED_EDGE('',*,*,#32604,.F.);
#43005=ORIENTED_EDGE('',*,*,#32609,.F.);
#43006=ORIENTED_EDGE('',*,*,#32610,.T.);
#43007=ORIENTED_EDGE('',*,*,#32611,.T.);
#43008=ORIENTED_EDGE('',*,*,#32607,.F.);
#43009=ORIENTED_EDGE('',*,*,#32612,.F.);
#43010=ORIENTED_EDGE('',*,*,#32613,.T.);
#43011=ORIENTED_EDGE('',*,*,#32614,.T.);
#43012=ORIENTED_EDGE('',*,*,#32610,.F.);
#43013=ORIENTED_EDGE('',*,*,#32615,.F.);
#43014=ORIENTED_EDGE('',*,*,#32616,.T.);
#43015=ORIENTED_EDGE('',*,*,#32617,.T.);
#43016=ORIENTED_EDGE('',*,*,#32613,.F.);
#43017=ORIENTED_EDGE('',*,*,#32618,.F.);
#43018=ORIENTED_EDGE('',*,*,#32599,.T.);
#43019=ORIENTED_EDGE('',*,*,#32619,.T.);
#43020=ORIENTED_EDGE('',*,*,#32616,.F.);
#43021=ORIENTED_EDGE('',*,*,#32620,.F.);
#43022=ORIENTED_EDGE('',*,*,#32621,.T.);
#43023=ORIENTED_EDGE('',*,*,#32622,.T.);
#43024=ORIENTED_EDGE('',*,*,#32623,.F.);
#43025=ORIENTED_EDGE('',*,*,#32624,.F.);
#43026=ORIENTED_EDGE('',*,*,#32625,.T.);
#43027=ORIENTED_EDGE('',*,*,#32626,.T.);
#43028=ORIENTED_EDGE('',*,*,#32621,.F.);
#43029=ORIENTED_EDGE('',*,*,#32627,.F.);
#43030=ORIENTED_EDGE('',*,*,#32628,.T.);
#43031=ORIENTED_EDGE('',*,*,#32629,.T.);
#43032=ORIENTED_EDGE('',*,*,#32625,.F.);
#43033=ORIENTED_EDGE('',*,*,#32630,.F.);
#43034=ORIENTED_EDGE('',*,*,#32631,.T.);
#43035=ORIENTED_EDGE('',*,*,#32632,.T.);
#43036=ORIENTED_EDGE('',*,*,#32628,.F.);
#43037=ORIENTED_EDGE('',*,*,#32633,.F.);
#43038=ORIENTED_EDGE('',*,*,#32634,.T.);
#43039=ORIENTED_EDGE('',*,*,#32635,.T.);
#43040=ORIENTED_EDGE('',*,*,#32631,.F.);
#43041=ORIENTED_EDGE('',*,*,#32636,.F.);
#43042=ORIENTED_EDGE('',*,*,#32637,.T.);
#43043=ORIENTED_EDGE('',*,*,#32638,.T.);
#43044=ORIENTED_EDGE('',*,*,#32634,.F.);
#43045=ORIENTED_EDGE('',*,*,#32639,.F.);
#43046=ORIENTED_EDGE('',*,*,#32640,.T.);
#43047=ORIENTED_EDGE('',*,*,#32641,.T.);
#43048=ORIENTED_EDGE('',*,*,#32637,.F.);
#43049=ORIENTED_EDGE('',*,*,#32642,.F.);
#43050=ORIENTED_EDGE('',*,*,#32643,.T.);
#43051=ORIENTED_EDGE('',*,*,#32644,.T.);
#43052=ORIENTED_EDGE('',*,*,#32640,.F.);
#43053=ORIENTED_EDGE('',*,*,#32645,.F.);
#43054=ORIENTED_EDGE('',*,*,#32646,.T.);
#43055=ORIENTED_EDGE('',*,*,#32647,.T.);
#43056=ORIENTED_EDGE('',*,*,#32643,.F.);
#43057=ORIENTED_EDGE('',*,*,#32648,.F.);
#43058=ORIENTED_EDGE('',*,*,#32649,.T.);
#43059=ORIENTED_EDGE('',*,*,#32650,.T.);
#43060=ORIENTED_EDGE('',*,*,#32646,.F.);
#43061=ORIENTED_EDGE('',*,*,#32651,.F.);
#43062=ORIENTED_EDGE('',*,*,#32652,.T.);
#43063=ORIENTED_EDGE('',*,*,#32653,.T.);
#43064=ORIENTED_EDGE('',*,*,#32649,.F.);
#43065=ORIENTED_EDGE('',*,*,#32654,.F.);
#43066=ORIENTED_EDGE('',*,*,#32655,.T.);
#43067=ORIENTED_EDGE('',*,*,#32656,.T.);
#43068=ORIENTED_EDGE('',*,*,#32652,.F.);
#43069=ORIENTED_EDGE('',*,*,#32657,.F.);
#43070=ORIENTED_EDGE('',*,*,#32658,.T.);
#43071=ORIENTED_EDGE('',*,*,#32659,.T.);
#43072=ORIENTED_EDGE('',*,*,#32655,.F.);
#43073=ORIENTED_EDGE('',*,*,#32660,.F.);
#43074=ORIENTED_EDGE('',*,*,#32661,.T.);
#43075=ORIENTED_EDGE('',*,*,#32662,.T.);
#43076=ORIENTED_EDGE('',*,*,#32658,.F.);
#43077=ORIENTED_EDGE('',*,*,#32663,.F.);
#43078=ORIENTED_EDGE('',*,*,#32664,.T.);
#43079=ORIENTED_EDGE('',*,*,#32665,.T.);
#43080=ORIENTED_EDGE('',*,*,#32661,.F.);
#43081=ORIENTED_EDGE('',*,*,#32666,.F.);
#43082=ORIENTED_EDGE('',*,*,#32667,.T.);
#43083=ORIENTED_EDGE('',*,*,#32668,.T.);
#43084=ORIENTED_EDGE('',*,*,#32664,.F.);
#43085=ORIENTED_EDGE('',*,*,#32669,.F.);
#43086=ORIENTED_EDGE('',*,*,#32670,.T.);
#43087=ORIENTED_EDGE('',*,*,#32671,.T.);
#43088=ORIENTED_EDGE('',*,*,#32667,.F.);
#43089=ORIENTED_EDGE('',*,*,#32672,.F.);
#43090=ORIENTED_EDGE('',*,*,#32673,.T.);
#43091=ORIENTED_EDGE('',*,*,#32674,.T.);
#43092=ORIENTED_EDGE('',*,*,#32670,.F.);
#43093=ORIENTED_EDGE('',*,*,#32675,.F.);
#43094=ORIENTED_EDGE('',*,*,#32676,.T.);
#43095=ORIENTED_EDGE('',*,*,#32677,.T.);
#43096=ORIENTED_EDGE('',*,*,#32673,.F.);
#43097=ORIENTED_EDGE('',*,*,#32678,.F.);
#43098=ORIENTED_EDGE('',*,*,#32679,.T.);
#43099=ORIENTED_EDGE('',*,*,#32680,.T.);
#43100=ORIENTED_EDGE('',*,*,#32676,.F.);
#43101=ORIENTED_EDGE('',*,*,#32681,.F.);
#43102=ORIENTED_EDGE('',*,*,#32682,.T.);
#43103=ORIENTED_EDGE('',*,*,#32683,.T.);
#43104=ORIENTED_EDGE('',*,*,#32679,.F.);
#43105=ORIENTED_EDGE('',*,*,#32684,.F.);
#43106=ORIENTED_EDGE('',*,*,#32623,.T.);
#43107=ORIENTED_EDGE('',*,*,#32685,.T.);
#43108=ORIENTED_EDGE('',*,*,#32682,.F.);
#43109=ORIENTED_EDGE('',*,*,#32685,.F.);
#43110=ORIENTED_EDGE('',*,*,#32622,.F.);
#43111=ORIENTED_EDGE('',*,*,#32626,.F.);
#43112=ORIENTED_EDGE('',*,*,#32629,.F.);
#43113=ORIENTED_EDGE('',*,*,#32632,.F.);
#43114=ORIENTED_EDGE('',*,*,#32635,.F.);
#43115=ORIENTED_EDGE('',*,*,#32638,.F.);
#43116=ORIENTED_EDGE('',*,*,#32641,.F.);
#43117=ORIENTED_EDGE('',*,*,#32644,.F.);
#43118=ORIENTED_EDGE('',*,*,#32647,.F.);
#43119=ORIENTED_EDGE('',*,*,#32650,.F.);
#43120=ORIENTED_EDGE('',*,*,#32653,.F.);
#43121=ORIENTED_EDGE('',*,*,#32656,.F.);
#43122=ORIENTED_EDGE('',*,*,#32659,.F.);
#43123=ORIENTED_EDGE('',*,*,#32662,.F.);
#43124=ORIENTED_EDGE('',*,*,#32665,.F.);
#43125=ORIENTED_EDGE('',*,*,#32668,.F.);
#43126=ORIENTED_EDGE('',*,*,#32671,.F.);
#43127=ORIENTED_EDGE('',*,*,#32674,.F.);
#43128=ORIENTED_EDGE('',*,*,#32677,.F.);
#43129=ORIENTED_EDGE('',*,*,#32680,.F.);
#43130=ORIENTED_EDGE('',*,*,#32683,.F.);
#43131=ORIENTED_EDGE('',*,*,#32619,.F.);
#43132=ORIENTED_EDGE('',*,*,#32598,.F.);
#43133=ORIENTED_EDGE('',*,*,#32602,.F.);
#43134=ORIENTED_EDGE('',*,*,#32605,.F.);
#43135=ORIENTED_EDGE('',*,*,#32608,.F.);
#43136=ORIENTED_EDGE('',*,*,#32611,.F.);
#43137=ORIENTED_EDGE('',*,*,#32614,.F.);
#43138=ORIENTED_EDGE('',*,*,#32617,.F.);
#43139=ORIENTED_EDGE('',*,*,#32596,.T.);
#43140=ORIENTED_EDGE('',*,*,#32618,.T.);
#43141=ORIENTED_EDGE('',*,*,#32615,.T.);
#43142=ORIENTED_EDGE('',*,*,#32612,.T.);
#43143=ORIENTED_EDGE('',*,*,#32609,.T.);
#43144=ORIENTED_EDGE('',*,*,#32606,.T.);
#43145=ORIENTED_EDGE('',*,*,#32603,.T.);
#43146=ORIENTED_EDGE('',*,*,#32600,.T.);
#43147=ORIENTED_EDGE('',*,*,#32536,.T.);
#43148=ORIENTED_EDGE('',*,*,#32558,.T.);
#43149=ORIENTED_EDGE('',*,*,#32555,.T.);
#43150=ORIENTED_EDGE('',*,*,#32552,.T.);
#43151=ORIENTED_EDGE('',*,*,#32549,.T.);
#43152=ORIENTED_EDGE('',*,*,#32546,.T.);
#43153=ORIENTED_EDGE('',*,*,#32543,.T.);
#43154=ORIENTED_EDGE('',*,*,#32540,.T.);
#43155=ORIENTED_EDGE('',*,*,#32686,.F.);
#43156=ORIENTED_EDGE('',*,*,#32687,.T.);
#43157=ORIENTED_EDGE('',*,*,#32688,.T.);
#43158=ORIENTED_EDGE('',*,*,#32689,.F.);
#43159=ORIENTED_EDGE('',*,*,#32690,.F.);
#43160=ORIENTED_EDGE('',*,*,#32691,.T.);
#43161=ORIENTED_EDGE('',*,*,#32692,.T.);
#43162=ORIENTED_EDGE('',*,*,#32687,.F.);
#43163=ORIENTED_EDGE('',*,*,#32693,.F.);
#43164=ORIENTED_EDGE('',*,*,#32694,.T.);
#43165=ORIENTED_EDGE('',*,*,#32695,.T.);
#43166=ORIENTED_EDGE('',*,*,#32691,.F.);
#43167=ORIENTED_EDGE('',*,*,#32696,.F.);
#43168=ORIENTED_EDGE('',*,*,#32689,.T.);
#43169=ORIENTED_EDGE('',*,*,#32697,.T.);
#43170=ORIENTED_EDGE('',*,*,#32694,.F.);
#43171=ORIENTED_EDGE('',*,*,#32697,.F.);
#43172=ORIENTED_EDGE('',*,*,#32688,.F.);
#43173=ORIENTED_EDGE('',*,*,#32692,.F.);
#43174=ORIENTED_EDGE('',*,*,#32695,.F.);
#43175=ORIENTED_EDGE('',*,*,#32698,.F.);
#43176=ORIENTED_EDGE('',*,*,#32699,.T.);
#43177=ORIENTED_EDGE('',*,*,#32700,.T.);
#43178=ORIENTED_EDGE('',*,*,#32701,.F.);
#43179=ORIENTED_EDGE('',*,*,#32702,.F.);
#43180=ORIENTED_EDGE('',*,*,#32703,.T.);
#43181=ORIENTED_EDGE('',*,*,#32704,.T.);
#43182=ORIENTED_EDGE('',*,*,#32699,.F.);
#43183=ORIENTED_EDGE('',*,*,#32705,.F.);
#43184=ORIENTED_EDGE('',*,*,#32706,.T.);
#43185=ORIENTED_EDGE('',*,*,#32707,.T.);
#43186=ORIENTED_EDGE('',*,*,#32703,.F.);
#43187=ORIENTED_EDGE('',*,*,#32708,.F.);
#43188=ORIENTED_EDGE('',*,*,#32701,.T.);
#43189=ORIENTED_EDGE('',*,*,#32709,.T.);
#43190=ORIENTED_EDGE('',*,*,#32706,.F.);
#43191=ORIENTED_EDGE('',*,*,#32709,.F.);
#43192=ORIENTED_EDGE('',*,*,#32700,.F.);
#43193=ORIENTED_EDGE('',*,*,#32704,.F.);
#43194=ORIENTED_EDGE('',*,*,#32707,.F.);
#43195=ORIENTED_EDGE('',*,*,#32710,.F.);
#43196=ORIENTED_EDGE('',*,*,#32711,.T.);
#43197=ORIENTED_EDGE('',*,*,#32712,.T.);
#43198=ORIENTED_EDGE('',*,*,#32713,.F.);
#43199=ORIENTED_EDGE('',*,*,#32714,.F.);
#43200=ORIENTED_EDGE('',*,*,#32715,.T.);
#43201=ORIENTED_EDGE('',*,*,#32716,.T.);
#43202=ORIENTED_EDGE('',*,*,#32711,.F.);
#43203=ORIENTED_EDGE('',*,*,#32717,.F.);
#43204=ORIENTED_EDGE('',*,*,#32718,.T.);
#43205=ORIENTED_EDGE('',*,*,#32719,.T.);
#43206=ORIENTED_EDGE('',*,*,#32715,.F.);
#43207=ORIENTED_EDGE('',*,*,#32720,.F.);
#43208=ORIENTED_EDGE('',*,*,#32713,.T.);
#43209=ORIENTED_EDGE('',*,*,#32721,.T.);
#43210=ORIENTED_EDGE('',*,*,#32718,.F.);
#43211=ORIENTED_EDGE('',*,*,#32721,.F.);
#43212=ORIENTED_EDGE('',*,*,#32712,.F.);
#43213=ORIENTED_EDGE('',*,*,#32716,.F.);
#43214=ORIENTED_EDGE('',*,*,#32719,.F.);
#43215=ORIENTED_EDGE('',*,*,#32722,.F.);
#43216=ORIENTED_EDGE('',*,*,#32723,.T.);
#43217=ORIENTED_EDGE('',*,*,#32724,.T.);
#43218=ORIENTED_EDGE('',*,*,#32725,.F.);
#43219=ORIENTED_EDGE('',*,*,#32726,.F.);
#43220=ORIENTED_EDGE('',*,*,#32727,.T.);
#43221=ORIENTED_EDGE('',*,*,#32728,.T.);
#43222=ORIENTED_EDGE('',*,*,#32723,.F.);
#43223=ORIENTED_EDGE('',*,*,#32729,.F.);
#43224=ORIENTED_EDGE('',*,*,#32730,.T.);
#43225=ORIENTED_EDGE('',*,*,#32731,.T.);
#43226=ORIENTED_EDGE('',*,*,#32727,.F.);
#43227=ORIENTED_EDGE('',*,*,#32732,.F.);
#43228=ORIENTED_EDGE('',*,*,#32725,.T.);
#43229=ORIENTED_EDGE('',*,*,#32733,.T.);
#43230=ORIENTED_EDGE('',*,*,#32730,.F.);
#43231=ORIENTED_EDGE('',*,*,#32733,.F.);
#43232=ORIENTED_EDGE('',*,*,#32724,.F.);
#43233=ORIENTED_EDGE('',*,*,#32728,.F.);
#43234=ORIENTED_EDGE('',*,*,#32731,.F.);
#43235=ORIENTED_EDGE('',*,*,#32734,.F.);
#43236=ORIENTED_EDGE('',*,*,#32735,.T.);
#43237=ORIENTED_EDGE('',*,*,#32736,.T.);
#43238=ORIENTED_EDGE('',*,*,#32737,.F.);
#43239=ORIENTED_EDGE('',*,*,#32738,.F.);
#43240=ORIENTED_EDGE('',*,*,#32739,.T.);
#43241=ORIENTED_EDGE('',*,*,#32740,.T.);
#43242=ORIENTED_EDGE('',*,*,#32735,.F.);
#43243=ORIENTED_EDGE('',*,*,#32741,.F.);
#43244=ORIENTED_EDGE('',*,*,#32742,.T.);
#43245=ORIENTED_EDGE('',*,*,#32743,.T.);
#43246=ORIENTED_EDGE('',*,*,#32739,.F.);
#43247=ORIENTED_EDGE('',*,*,#32744,.F.);
#43248=ORIENTED_EDGE('',*,*,#32737,.T.);
#43249=ORIENTED_EDGE('',*,*,#32745,.T.);
#43250=ORIENTED_EDGE('',*,*,#32742,.F.);
#43251=ORIENTED_EDGE('',*,*,#32745,.F.);
#43252=ORIENTED_EDGE('',*,*,#32736,.F.);
#43253=ORIENTED_EDGE('',*,*,#32740,.F.);
#43254=ORIENTED_EDGE('',*,*,#32743,.F.);
#43255=ORIENTED_EDGE('',*,*,#32746,.F.);
#43256=ORIENTED_EDGE('',*,*,#32747,.T.);
#43257=ORIENTED_EDGE('',*,*,#32748,.T.);
#43258=ORIENTED_EDGE('',*,*,#32749,.F.);
#43259=ORIENTED_EDGE('',*,*,#32750,.F.);
#43260=ORIENTED_EDGE('',*,*,#32751,.T.);
#43261=ORIENTED_EDGE('',*,*,#32752,.T.);
#43262=ORIENTED_EDGE('',*,*,#32747,.F.);
#43263=ORIENTED_EDGE('',*,*,#32753,.F.);
#43264=ORIENTED_EDGE('',*,*,#32754,.T.);
#43265=ORIENTED_EDGE('',*,*,#32755,.T.);
#43266=ORIENTED_EDGE('',*,*,#32751,.F.);
#43267=ORIENTED_EDGE('',*,*,#32756,.F.);
#43268=ORIENTED_EDGE('',*,*,#32749,.T.);
#43269=ORIENTED_EDGE('',*,*,#32757,.T.);
#43270=ORIENTED_EDGE('',*,*,#32754,.F.);
#43271=ORIENTED_EDGE('',*,*,#32757,.F.);
#43272=ORIENTED_EDGE('',*,*,#32748,.F.);
#43273=ORIENTED_EDGE('',*,*,#32752,.F.);
#43274=ORIENTED_EDGE('',*,*,#32755,.F.);
#43275=ORIENTED_EDGE('',*,*,#32758,.F.);
#43276=ORIENTED_EDGE('',*,*,#32759,.T.);
#43277=ORIENTED_EDGE('',*,*,#32760,.T.);
#43278=ORIENTED_EDGE('',*,*,#32761,.F.);
#43279=ORIENTED_EDGE('',*,*,#32762,.F.);
#43280=ORIENTED_EDGE('',*,*,#32763,.T.);
#43281=ORIENTED_EDGE('',*,*,#32764,.T.);
#43282=ORIENTED_EDGE('',*,*,#32759,.F.);
#43283=ORIENTED_EDGE('',*,*,#32765,.F.);
#43284=ORIENTED_EDGE('',*,*,#32766,.T.);
#43285=ORIENTED_EDGE('',*,*,#32767,.T.);
#43286=ORIENTED_EDGE('',*,*,#32763,.F.);
#43287=ORIENTED_EDGE('',*,*,#32768,.F.);
#43288=ORIENTED_EDGE('',*,*,#32761,.T.);
#43289=ORIENTED_EDGE('',*,*,#32769,.T.);
#43290=ORIENTED_EDGE('',*,*,#32766,.F.);
#43291=ORIENTED_EDGE('',*,*,#32769,.F.);
#43292=ORIENTED_EDGE('',*,*,#32760,.F.);
#43293=ORIENTED_EDGE('',*,*,#32764,.F.);
#43294=ORIENTED_EDGE('',*,*,#32767,.F.);
#43295=ORIENTED_EDGE('',*,*,#32770,.F.);
#43296=ORIENTED_EDGE('',*,*,#32771,.T.);
#43297=ORIENTED_EDGE('',*,*,#32772,.T.);
#43298=ORIENTED_EDGE('',*,*,#32773,.F.);
#43299=ORIENTED_EDGE('',*,*,#32774,.F.);
#43300=ORIENTED_EDGE('',*,*,#32775,.T.);
#43301=ORIENTED_EDGE('',*,*,#32776,.T.);
#43302=ORIENTED_EDGE('',*,*,#32771,.F.);
#43303=ORIENTED_EDGE('',*,*,#32777,.F.);
#43304=ORIENTED_EDGE('',*,*,#32778,.T.);
#43305=ORIENTED_EDGE('',*,*,#32779,.T.);
#43306=ORIENTED_EDGE('',*,*,#32775,.F.);
#43307=ORIENTED_EDGE('',*,*,#32780,.F.);
#43308=ORIENTED_EDGE('',*,*,#32773,.T.);
#43309=ORIENTED_EDGE('',*,*,#32781,.T.);
#43310=ORIENTED_EDGE('',*,*,#32778,.F.);
#43311=ORIENTED_EDGE('',*,*,#32781,.F.);
#43312=ORIENTED_EDGE('',*,*,#32772,.F.);
#43313=ORIENTED_EDGE('',*,*,#32776,.F.);
#43314=ORIENTED_EDGE('',*,*,#32779,.F.);
#43315=ORIENTED_EDGE('',*,*,#32782,.F.);
#43316=ORIENTED_EDGE('',*,*,#32783,.T.);
#43317=ORIENTED_EDGE('',*,*,#32784,.T.);
#43318=ORIENTED_EDGE('',*,*,#32785,.F.);
#43319=ORIENTED_EDGE('',*,*,#32786,.F.);
#43320=ORIENTED_EDGE('',*,*,#32787,.T.);
#43321=ORIENTED_EDGE('',*,*,#32788,.T.);
#43322=ORIENTED_EDGE('',*,*,#32783,.F.);
#43323=ORIENTED_EDGE('',*,*,#32789,.F.);
#43324=ORIENTED_EDGE('',*,*,#32790,.T.);
#43325=ORIENTED_EDGE('',*,*,#32791,.T.);
#43326=ORIENTED_EDGE('',*,*,#32787,.F.);
#43327=ORIENTED_EDGE('',*,*,#32792,.F.);
#43328=ORIENTED_EDGE('',*,*,#32785,.T.);
#43329=ORIENTED_EDGE('',*,*,#32793,.T.);
#43330=ORIENTED_EDGE('',*,*,#32790,.F.);
#43331=ORIENTED_EDGE('',*,*,#32793,.F.);
#43332=ORIENTED_EDGE('',*,*,#32784,.F.);
#43333=ORIENTED_EDGE('',*,*,#32788,.F.);
#43334=ORIENTED_EDGE('',*,*,#32791,.F.);
#43335=ORIENTED_EDGE('',*,*,#32794,.F.);
#43336=ORIENTED_EDGE('',*,*,#32795,.T.);
#43337=ORIENTED_EDGE('',*,*,#32796,.T.);
#43338=ORIENTED_EDGE('',*,*,#32797,.F.);
#43339=ORIENTED_EDGE('',*,*,#32798,.F.);
#43340=ORIENTED_EDGE('',*,*,#32799,.T.);
#43341=ORIENTED_EDGE('',*,*,#32800,.T.);
#43342=ORIENTED_EDGE('',*,*,#32795,.F.);
#43343=ORIENTED_EDGE('',*,*,#32801,.F.);
#43344=ORIENTED_EDGE('',*,*,#32802,.T.);
#43345=ORIENTED_EDGE('',*,*,#32803,.T.);
#43346=ORIENTED_EDGE('',*,*,#32799,.F.);
#43347=ORIENTED_EDGE('',*,*,#32804,.F.);
#43348=ORIENTED_EDGE('',*,*,#32797,.T.);
#43349=ORIENTED_EDGE('',*,*,#32805,.T.);
#43350=ORIENTED_EDGE('',*,*,#32802,.F.);
#43351=ORIENTED_EDGE('',*,*,#32805,.F.);
#43352=ORIENTED_EDGE('',*,*,#32796,.F.);
#43353=ORIENTED_EDGE('',*,*,#32800,.F.);
#43354=ORIENTED_EDGE('',*,*,#32803,.F.);
#43355=ORIENTED_EDGE('',*,*,#32806,.F.);
#43356=ORIENTED_EDGE('',*,*,#32807,.T.);
#43357=ORIENTED_EDGE('',*,*,#32808,.T.);
#43358=ORIENTED_EDGE('',*,*,#32809,.F.);
#43359=ORIENTED_EDGE('',*,*,#32810,.F.);
#43360=ORIENTED_EDGE('',*,*,#32811,.T.);
#43361=ORIENTED_EDGE('',*,*,#32812,.T.);
#43362=ORIENTED_EDGE('',*,*,#32807,.F.);
#43363=ORIENTED_EDGE('',*,*,#32813,.F.);
#43364=ORIENTED_EDGE('',*,*,#32814,.T.);
#43365=ORIENTED_EDGE('',*,*,#32815,.T.);
#43366=ORIENTED_EDGE('',*,*,#32811,.F.);
#43367=ORIENTED_EDGE('',*,*,#32816,.F.);
#43368=ORIENTED_EDGE('',*,*,#32809,.T.);
#43369=ORIENTED_EDGE('',*,*,#32817,.T.);
#43370=ORIENTED_EDGE('',*,*,#32814,.F.);
#43371=ORIENTED_EDGE('',*,*,#32817,.F.);
#43372=ORIENTED_EDGE('',*,*,#32808,.F.);
#43373=ORIENTED_EDGE('',*,*,#32812,.F.);
#43374=ORIENTED_EDGE('',*,*,#32815,.F.);
#43375=ORIENTED_EDGE('',*,*,#32818,.F.);
#43376=ORIENTED_EDGE('',*,*,#32819,.T.);
#43377=ORIENTED_EDGE('',*,*,#32820,.T.);
#43378=ORIENTED_EDGE('',*,*,#32821,.F.);
#43379=ORIENTED_EDGE('',*,*,#32822,.F.);
#43380=ORIENTED_EDGE('',*,*,#32823,.T.);
#43381=ORIENTED_EDGE('',*,*,#32824,.T.);
#43382=ORIENTED_EDGE('',*,*,#32819,.F.);
#43383=ORIENTED_EDGE('',*,*,#32825,.F.);
#43384=ORIENTED_EDGE('',*,*,#32826,.T.);
#43385=ORIENTED_EDGE('',*,*,#32827,.T.);
#43386=ORIENTED_EDGE('',*,*,#32823,.F.);
#43387=ORIENTED_EDGE('',*,*,#32828,.F.);
#43388=ORIENTED_EDGE('',*,*,#32821,.T.);
#43389=ORIENTED_EDGE('',*,*,#32829,.T.);
#43390=ORIENTED_EDGE('',*,*,#32826,.F.);
#43391=ORIENTED_EDGE('',*,*,#32829,.F.);
#43392=ORIENTED_EDGE('',*,*,#32820,.F.);
#43393=ORIENTED_EDGE('',*,*,#32824,.F.);
#43394=ORIENTED_EDGE('',*,*,#32827,.F.);
#43395=ORIENTED_EDGE('',*,*,#32830,.F.);
#43396=ORIENTED_EDGE('',*,*,#32831,.T.);
#43397=ORIENTED_EDGE('',*,*,#32832,.T.);
#43398=ORIENTED_EDGE('',*,*,#32833,.F.);
#43399=ORIENTED_EDGE('',*,*,#32834,.F.);
#43400=ORIENTED_EDGE('',*,*,#32835,.T.);
#43401=ORIENTED_EDGE('',*,*,#32836,.T.);
#43402=ORIENTED_EDGE('',*,*,#32831,.F.);
#43403=ORIENTED_EDGE('',*,*,#32837,.F.);
#43404=ORIENTED_EDGE('',*,*,#32838,.T.);
#43405=ORIENTED_EDGE('',*,*,#32839,.T.);
#43406=ORIENTED_EDGE('',*,*,#32835,.F.);
#43407=ORIENTED_EDGE('',*,*,#32840,.F.);
#43408=ORIENTED_EDGE('',*,*,#32833,.T.);
#43409=ORIENTED_EDGE('',*,*,#32841,.T.);
#43410=ORIENTED_EDGE('',*,*,#32838,.F.);
#43411=ORIENTED_EDGE('',*,*,#32841,.F.);
#43412=ORIENTED_EDGE('',*,*,#32832,.F.);
#43413=ORIENTED_EDGE('',*,*,#32836,.F.);
#43414=ORIENTED_EDGE('',*,*,#32839,.F.);
#43415=ORIENTED_EDGE('',*,*,#32842,.F.);
#43416=ORIENTED_EDGE('',*,*,#32843,.T.);
#43417=ORIENTED_EDGE('',*,*,#32844,.T.);
#43418=ORIENTED_EDGE('',*,*,#32845,.F.);
#43419=ORIENTED_EDGE('',*,*,#32846,.F.);
#43420=ORIENTED_EDGE('',*,*,#32847,.T.);
#43421=ORIENTED_EDGE('',*,*,#32848,.T.);
#43422=ORIENTED_EDGE('',*,*,#32843,.F.);
#43423=ORIENTED_EDGE('',*,*,#32849,.F.);
#43424=ORIENTED_EDGE('',*,*,#32850,.T.);
#43425=ORIENTED_EDGE('',*,*,#32851,.T.);
#43426=ORIENTED_EDGE('',*,*,#32847,.F.);
#43427=ORIENTED_EDGE('',*,*,#32852,.F.);
#43428=ORIENTED_EDGE('',*,*,#32845,.T.);
#43429=ORIENTED_EDGE('',*,*,#32853,.T.);
#43430=ORIENTED_EDGE('',*,*,#32850,.F.);
#43431=ORIENTED_EDGE('',*,*,#32853,.F.);
#43432=ORIENTED_EDGE('',*,*,#32844,.F.);
#43433=ORIENTED_EDGE('',*,*,#32848,.F.);
#43434=ORIENTED_EDGE('',*,*,#32851,.F.);
#43435=ORIENTED_EDGE('',*,*,#32854,.F.);
#43436=ORIENTED_EDGE('',*,*,#32855,.T.);
#43437=ORIENTED_EDGE('',*,*,#32856,.T.);
#43438=ORIENTED_EDGE('',*,*,#32857,.F.);
#43439=ORIENTED_EDGE('',*,*,#32858,.F.);
#43440=ORIENTED_EDGE('',*,*,#32859,.T.);
#43441=ORIENTED_EDGE('',*,*,#32860,.T.);
#43442=ORIENTED_EDGE('',*,*,#32855,.F.);
#43443=ORIENTED_EDGE('',*,*,#32861,.F.);
#43444=ORIENTED_EDGE('',*,*,#32862,.T.);
#43445=ORIENTED_EDGE('',*,*,#32863,.T.);
#43446=ORIENTED_EDGE('',*,*,#32859,.F.);
#43447=ORIENTED_EDGE('',*,*,#32864,.F.);
#43448=ORIENTED_EDGE('',*,*,#32857,.T.);
#43449=ORIENTED_EDGE('',*,*,#32865,.T.);
#43450=ORIENTED_EDGE('',*,*,#32862,.F.);
#43451=ORIENTED_EDGE('',*,*,#32865,.F.);
#43452=ORIENTED_EDGE('',*,*,#32856,.F.);
#43453=ORIENTED_EDGE('',*,*,#32860,.F.);
#43454=ORIENTED_EDGE('',*,*,#32863,.F.);
#43455=ORIENTED_EDGE('',*,*,#32866,.F.);
#43456=ORIENTED_EDGE('',*,*,#32867,.T.);
#43457=ORIENTED_EDGE('',*,*,#32868,.T.);
#43458=ORIENTED_EDGE('',*,*,#32869,.F.);
#43459=ORIENTED_EDGE('',*,*,#32870,.F.);
#43460=ORIENTED_EDGE('',*,*,#32871,.T.);
#43461=ORIENTED_EDGE('',*,*,#32872,.T.);
#43462=ORIENTED_EDGE('',*,*,#32867,.F.);
#43463=ORIENTED_EDGE('',*,*,#32873,.F.);
#43464=ORIENTED_EDGE('',*,*,#32874,.T.);
#43465=ORIENTED_EDGE('',*,*,#32875,.T.);
#43466=ORIENTED_EDGE('',*,*,#32871,.F.);
#43467=ORIENTED_EDGE('',*,*,#32876,.F.);
#43468=ORIENTED_EDGE('',*,*,#32869,.T.);
#43469=ORIENTED_EDGE('',*,*,#32877,.T.);
#43470=ORIENTED_EDGE('',*,*,#32874,.F.);
#43471=ORIENTED_EDGE('',*,*,#32877,.F.);
#43472=ORIENTED_EDGE('',*,*,#32868,.F.);
#43473=ORIENTED_EDGE('',*,*,#32872,.F.);
#43474=ORIENTED_EDGE('',*,*,#32875,.F.);
#43475=ORIENTED_EDGE('',*,*,#32878,.F.);
#43476=ORIENTED_EDGE('',*,*,#32879,.T.);
#43477=ORIENTED_EDGE('',*,*,#32880,.T.);
#43478=ORIENTED_EDGE('',*,*,#32881,.F.);
#43479=ORIENTED_EDGE('',*,*,#32882,.F.);
#43480=ORIENTED_EDGE('',*,*,#32883,.T.);
#43481=ORIENTED_EDGE('',*,*,#32884,.T.);
#43482=ORIENTED_EDGE('',*,*,#32879,.F.);
#43483=ORIENTED_EDGE('',*,*,#32885,.F.);
#43484=ORIENTED_EDGE('',*,*,#32886,.T.);
#43485=ORIENTED_EDGE('',*,*,#32887,.T.);
#43486=ORIENTED_EDGE('',*,*,#32883,.F.);
#43487=ORIENTED_EDGE('',*,*,#32888,.F.);
#43488=ORIENTED_EDGE('',*,*,#32881,.T.);
#43489=ORIENTED_EDGE('',*,*,#32889,.T.);
#43490=ORIENTED_EDGE('',*,*,#32886,.F.);
#43491=ORIENTED_EDGE('',*,*,#32889,.F.);
#43492=ORIENTED_EDGE('',*,*,#32880,.F.);
#43493=ORIENTED_EDGE('',*,*,#32884,.F.);
#43494=ORIENTED_EDGE('',*,*,#32887,.F.);
#43495=ORIENTED_EDGE('',*,*,#32890,.F.);
#43496=ORIENTED_EDGE('',*,*,#32891,.T.);
#43497=ORIENTED_EDGE('',*,*,#32892,.T.);
#43498=ORIENTED_EDGE('',*,*,#32893,.F.);
#43499=ORIENTED_EDGE('',*,*,#32894,.F.);
#43500=ORIENTED_EDGE('',*,*,#32895,.T.);
#43501=ORIENTED_EDGE('',*,*,#32896,.T.);
#43502=ORIENTED_EDGE('',*,*,#32891,.F.);
#43503=ORIENTED_EDGE('',*,*,#32897,.F.);
#43504=ORIENTED_EDGE('',*,*,#32898,.T.);
#43505=ORIENTED_EDGE('',*,*,#32899,.T.);
#43506=ORIENTED_EDGE('',*,*,#32895,.F.);
#43507=ORIENTED_EDGE('',*,*,#32900,.F.);
#43508=ORIENTED_EDGE('',*,*,#32893,.T.);
#43509=ORIENTED_EDGE('',*,*,#32901,.T.);
#43510=ORIENTED_EDGE('',*,*,#32898,.F.);
#43511=ORIENTED_EDGE('',*,*,#32901,.F.);
#43512=ORIENTED_EDGE('',*,*,#32892,.F.);
#43513=ORIENTED_EDGE('',*,*,#32896,.F.);
#43514=ORIENTED_EDGE('',*,*,#32899,.F.);
#43515=ORIENTED_EDGE('',*,*,#32902,.F.);
#43516=ORIENTED_EDGE('',*,*,#32903,.T.);
#43517=ORIENTED_EDGE('',*,*,#32904,.T.);
#43518=ORIENTED_EDGE('',*,*,#32905,.F.);
#43519=ORIENTED_EDGE('',*,*,#32906,.F.);
#43520=ORIENTED_EDGE('',*,*,#32907,.T.);
#43521=ORIENTED_EDGE('',*,*,#32908,.T.);
#43522=ORIENTED_EDGE('',*,*,#32903,.F.);
#43523=ORIENTED_EDGE('',*,*,#32909,.F.);
#43524=ORIENTED_EDGE('',*,*,#32910,.T.);
#43525=ORIENTED_EDGE('',*,*,#32911,.T.);
#43526=ORIENTED_EDGE('',*,*,#32907,.F.);
#43527=ORIENTED_EDGE('',*,*,#32912,.F.);
#43528=ORIENTED_EDGE('',*,*,#32905,.T.);
#43529=ORIENTED_EDGE('',*,*,#32913,.T.);
#43530=ORIENTED_EDGE('',*,*,#32910,.F.);
#43531=ORIENTED_EDGE('',*,*,#32913,.F.);
#43532=ORIENTED_EDGE('',*,*,#32904,.F.);
#43533=ORIENTED_EDGE('',*,*,#32908,.F.);
#43534=ORIENTED_EDGE('',*,*,#32911,.F.);
#43535=ORIENTED_EDGE('',*,*,#32914,.F.);
#43536=ORIENTED_EDGE('',*,*,#32915,.T.);
#43537=ORIENTED_EDGE('',*,*,#32916,.T.);
#43538=ORIENTED_EDGE('',*,*,#32917,.F.);
#43539=ORIENTED_EDGE('',*,*,#32918,.F.);
#43540=ORIENTED_EDGE('',*,*,#32919,.T.);
#43541=ORIENTED_EDGE('',*,*,#32920,.T.);
#43542=ORIENTED_EDGE('',*,*,#32915,.F.);
#43543=ORIENTED_EDGE('',*,*,#32921,.F.);
#43544=ORIENTED_EDGE('',*,*,#32922,.T.);
#43545=ORIENTED_EDGE('',*,*,#32923,.T.);
#43546=ORIENTED_EDGE('',*,*,#32919,.F.);
#43547=ORIENTED_EDGE('',*,*,#32924,.F.);
#43548=ORIENTED_EDGE('',*,*,#32917,.T.);
#43549=ORIENTED_EDGE('',*,*,#32925,.T.);
#43550=ORIENTED_EDGE('',*,*,#32922,.F.);
#43551=ORIENTED_EDGE('',*,*,#32925,.F.);
#43552=ORIENTED_EDGE('',*,*,#32916,.F.);
#43553=ORIENTED_EDGE('',*,*,#32920,.F.);
#43554=ORIENTED_EDGE('',*,*,#32923,.F.);
#43555=ORIENTED_EDGE('',*,*,#32926,.F.);
#43556=ORIENTED_EDGE('',*,*,#32927,.T.);
#43557=ORIENTED_EDGE('',*,*,#32928,.T.);
#43558=ORIENTED_EDGE('',*,*,#32929,.F.);
#43559=ORIENTED_EDGE('',*,*,#32930,.F.);
#43560=ORIENTED_EDGE('',*,*,#32931,.T.);
#43561=ORIENTED_EDGE('',*,*,#32932,.T.);
#43562=ORIENTED_EDGE('',*,*,#32927,.F.);
#43563=ORIENTED_EDGE('',*,*,#32933,.F.);
#43564=ORIENTED_EDGE('',*,*,#32934,.T.);
#43565=ORIENTED_EDGE('',*,*,#32935,.T.);
#43566=ORIENTED_EDGE('',*,*,#32931,.F.);
#43567=ORIENTED_EDGE('',*,*,#32936,.F.);
#43568=ORIENTED_EDGE('',*,*,#32929,.T.);
#43569=ORIENTED_EDGE('',*,*,#32937,.T.);
#43570=ORIENTED_EDGE('',*,*,#32934,.F.);
#43571=ORIENTED_EDGE('',*,*,#32937,.F.);
#43572=ORIENTED_EDGE('',*,*,#32928,.F.);
#43573=ORIENTED_EDGE('',*,*,#32932,.F.);
#43574=ORIENTED_EDGE('',*,*,#32935,.F.);
#43575=ORIENTED_EDGE('',*,*,#32938,.F.);
#43576=ORIENTED_EDGE('',*,*,#32939,.T.);
#43577=ORIENTED_EDGE('',*,*,#32940,.T.);
#43578=ORIENTED_EDGE('',*,*,#32941,.F.);
#43579=ORIENTED_EDGE('',*,*,#32942,.F.);
#43580=ORIENTED_EDGE('',*,*,#32943,.T.);
#43581=ORIENTED_EDGE('',*,*,#32944,.T.);
#43582=ORIENTED_EDGE('',*,*,#32939,.F.);
#43583=ORIENTED_EDGE('',*,*,#32945,.F.);
#43584=ORIENTED_EDGE('',*,*,#32946,.T.);
#43585=ORIENTED_EDGE('',*,*,#32947,.T.);
#43586=ORIENTED_EDGE('',*,*,#32943,.F.);
#43587=ORIENTED_EDGE('',*,*,#32948,.F.);
#43588=ORIENTED_EDGE('',*,*,#32941,.T.);
#43589=ORIENTED_EDGE('',*,*,#32949,.T.);
#43590=ORIENTED_EDGE('',*,*,#32946,.F.);
#43591=ORIENTED_EDGE('',*,*,#32949,.F.);
#43592=ORIENTED_EDGE('',*,*,#32940,.F.);
#43593=ORIENTED_EDGE('',*,*,#32944,.F.);
#43594=ORIENTED_EDGE('',*,*,#32947,.F.);
#43595=ORIENTED_EDGE('',*,*,#32950,.F.);
#43596=ORIENTED_EDGE('',*,*,#32951,.T.);
#43597=ORIENTED_EDGE('',*,*,#32952,.T.);
#43598=ORIENTED_EDGE('',*,*,#32953,.F.);
#43599=ORIENTED_EDGE('',*,*,#32954,.F.);
#43600=ORIENTED_EDGE('',*,*,#32955,.T.);
#43601=ORIENTED_EDGE('',*,*,#32956,.T.);
#43602=ORIENTED_EDGE('',*,*,#32951,.F.);
#43603=ORIENTED_EDGE('',*,*,#32957,.F.);
#43604=ORIENTED_EDGE('',*,*,#32958,.T.);
#43605=ORIENTED_EDGE('',*,*,#32959,.T.);
#43606=ORIENTED_EDGE('',*,*,#32955,.F.);
#43607=ORIENTED_EDGE('',*,*,#32960,.F.);
#43608=ORIENTED_EDGE('',*,*,#32953,.T.);
#43609=ORIENTED_EDGE('',*,*,#32961,.T.);
#43610=ORIENTED_EDGE('',*,*,#32958,.F.);
#43611=ORIENTED_EDGE('',*,*,#32961,.F.);
#43612=ORIENTED_EDGE('',*,*,#32952,.F.);
#43613=ORIENTED_EDGE('',*,*,#32956,.F.);
#43614=ORIENTED_EDGE('',*,*,#32959,.F.);
#43615=ORIENTED_EDGE('',*,*,#32962,.F.);
#43616=ORIENTED_EDGE('',*,*,#32963,.T.);
#43617=ORIENTED_EDGE('',*,*,#32964,.T.);
#43618=ORIENTED_EDGE('',*,*,#32965,.F.);
#43619=ORIENTED_EDGE('',*,*,#32966,.F.);
#43620=ORIENTED_EDGE('',*,*,#32967,.T.);
#43621=ORIENTED_EDGE('',*,*,#32968,.T.);
#43622=ORIENTED_EDGE('',*,*,#32963,.F.);
#43623=ORIENTED_EDGE('',*,*,#32969,.F.);
#43624=ORIENTED_EDGE('',*,*,#32970,.T.);
#43625=ORIENTED_EDGE('',*,*,#32971,.T.);
#43626=ORIENTED_EDGE('',*,*,#32967,.F.);
#43627=ORIENTED_EDGE('',*,*,#32972,.F.);
#43628=ORIENTED_EDGE('',*,*,#32965,.T.);
#43629=ORIENTED_EDGE('',*,*,#32973,.T.);
#43630=ORIENTED_EDGE('',*,*,#32970,.F.);
#43631=ORIENTED_EDGE('',*,*,#32973,.F.);
#43632=ORIENTED_EDGE('',*,*,#32964,.F.);
#43633=ORIENTED_EDGE('',*,*,#32968,.F.);
#43634=ORIENTED_EDGE('',*,*,#32971,.F.);
#43635=ORIENTED_EDGE('',*,*,#32974,.F.);
#43636=ORIENTED_EDGE('',*,*,#32975,.T.);
#43637=ORIENTED_EDGE('',*,*,#32976,.T.);
#43638=ORIENTED_EDGE('',*,*,#32977,.F.);
#43639=ORIENTED_EDGE('',*,*,#32978,.F.);
#43640=ORIENTED_EDGE('',*,*,#32979,.T.);
#43641=ORIENTED_EDGE('',*,*,#32980,.T.);
#43642=ORIENTED_EDGE('',*,*,#32975,.F.);
#43643=ORIENTED_EDGE('',*,*,#32981,.F.);
#43644=ORIENTED_EDGE('',*,*,#32982,.T.);
#43645=ORIENTED_EDGE('',*,*,#32983,.T.);
#43646=ORIENTED_EDGE('',*,*,#32979,.F.);
#43647=ORIENTED_EDGE('',*,*,#32984,.F.);
#43648=ORIENTED_EDGE('',*,*,#32977,.T.);
#43649=ORIENTED_EDGE('',*,*,#32985,.T.);
#43650=ORIENTED_EDGE('',*,*,#32982,.F.);
#43651=ORIENTED_EDGE('',*,*,#32985,.F.);
#43652=ORIENTED_EDGE('',*,*,#32976,.F.);
#43653=ORIENTED_EDGE('',*,*,#32980,.F.);
#43654=ORIENTED_EDGE('',*,*,#32983,.F.);
#43655=ORIENTED_EDGE('',*,*,#32986,.F.);
#43656=ORIENTED_EDGE('',*,*,#32987,.T.);
#43657=ORIENTED_EDGE('',*,*,#32988,.T.);
#43658=ORIENTED_EDGE('',*,*,#32989,.F.);
#43659=ORIENTED_EDGE('',*,*,#32990,.F.);
#43660=ORIENTED_EDGE('',*,*,#32991,.T.);
#43661=ORIENTED_EDGE('',*,*,#32992,.T.);
#43662=ORIENTED_EDGE('',*,*,#32987,.F.);
#43663=ORIENTED_EDGE('',*,*,#32993,.F.);
#43664=ORIENTED_EDGE('',*,*,#32994,.T.);
#43665=ORIENTED_EDGE('',*,*,#32995,.T.);
#43666=ORIENTED_EDGE('',*,*,#32991,.F.);
#43667=ORIENTED_EDGE('',*,*,#32996,.F.);
#43668=ORIENTED_EDGE('',*,*,#32989,.T.);
#43669=ORIENTED_EDGE('',*,*,#32997,.T.);
#43670=ORIENTED_EDGE('',*,*,#32994,.F.);
#43671=ORIENTED_EDGE('',*,*,#32997,.F.);
#43672=ORIENTED_EDGE('',*,*,#32988,.F.);
#43673=ORIENTED_EDGE('',*,*,#32992,.F.);
#43674=ORIENTED_EDGE('',*,*,#32995,.F.);
#43675=ORIENTED_EDGE('',*,*,#32998,.F.);
#43676=ORIENTED_EDGE('',*,*,#32999,.T.);
#43677=ORIENTED_EDGE('',*,*,#33000,.T.);
#43678=ORIENTED_EDGE('',*,*,#33001,.F.);
#43679=ORIENTED_EDGE('',*,*,#33002,.F.);
#43680=ORIENTED_EDGE('',*,*,#33003,.T.);
#43681=ORIENTED_EDGE('',*,*,#33004,.T.);
#43682=ORIENTED_EDGE('',*,*,#32999,.F.);
#43683=ORIENTED_EDGE('',*,*,#33005,.F.);
#43684=ORIENTED_EDGE('',*,*,#33006,.T.);
#43685=ORIENTED_EDGE('',*,*,#33007,.T.);
#43686=ORIENTED_EDGE('',*,*,#33003,.F.);
#43687=ORIENTED_EDGE('',*,*,#33008,.F.);
#43688=ORIENTED_EDGE('',*,*,#33001,.T.);
#43689=ORIENTED_EDGE('',*,*,#33009,.T.);
#43690=ORIENTED_EDGE('',*,*,#33006,.F.);
#43691=ORIENTED_EDGE('',*,*,#33009,.F.);
#43692=ORIENTED_EDGE('',*,*,#33000,.F.);
#43693=ORIENTED_EDGE('',*,*,#33004,.F.);
#43694=ORIENTED_EDGE('',*,*,#33007,.F.);
#43695=ORIENTED_EDGE('',*,*,#33010,.F.);
#43696=ORIENTED_EDGE('',*,*,#33011,.T.);
#43697=ORIENTED_EDGE('',*,*,#33012,.T.);
#43698=ORIENTED_EDGE('',*,*,#33013,.F.);
#43699=ORIENTED_EDGE('',*,*,#33014,.F.);
#43700=ORIENTED_EDGE('',*,*,#33015,.T.);
#43701=ORIENTED_EDGE('',*,*,#33016,.T.);
#43702=ORIENTED_EDGE('',*,*,#33011,.F.);
#43703=ORIENTED_EDGE('',*,*,#33017,.F.);
#43704=ORIENTED_EDGE('',*,*,#33018,.T.);
#43705=ORIENTED_EDGE('',*,*,#33019,.T.);
#43706=ORIENTED_EDGE('',*,*,#33015,.F.);
#43707=ORIENTED_EDGE('',*,*,#33020,.F.);
#43708=ORIENTED_EDGE('',*,*,#33013,.T.);
#43709=ORIENTED_EDGE('',*,*,#33021,.T.);
#43710=ORIENTED_EDGE('',*,*,#33018,.F.);
#43711=ORIENTED_EDGE('',*,*,#33021,.F.);
#43712=ORIENTED_EDGE('',*,*,#33012,.F.);
#43713=ORIENTED_EDGE('',*,*,#33016,.F.);
#43714=ORIENTED_EDGE('',*,*,#33019,.F.);
#43715=ORIENTED_EDGE('',*,*,#33022,.F.);
#43716=ORIENTED_EDGE('',*,*,#33023,.T.);
#43717=ORIENTED_EDGE('',*,*,#33024,.T.);
#43718=ORIENTED_EDGE('',*,*,#33025,.F.);
#43719=ORIENTED_EDGE('',*,*,#33026,.F.);
#43720=ORIENTED_EDGE('',*,*,#33027,.T.);
#43721=ORIENTED_EDGE('',*,*,#33028,.T.);
#43722=ORIENTED_EDGE('',*,*,#33023,.F.);
#43723=ORIENTED_EDGE('',*,*,#33029,.F.);
#43724=ORIENTED_EDGE('',*,*,#33030,.T.);
#43725=ORIENTED_EDGE('',*,*,#33031,.T.);
#43726=ORIENTED_EDGE('',*,*,#33027,.F.);
#43727=ORIENTED_EDGE('',*,*,#33032,.F.);
#43728=ORIENTED_EDGE('',*,*,#33025,.T.);
#43729=ORIENTED_EDGE('',*,*,#33033,.T.);
#43730=ORIENTED_EDGE('',*,*,#33030,.F.);
#43731=ORIENTED_EDGE('',*,*,#33033,.F.);
#43732=ORIENTED_EDGE('',*,*,#33024,.F.);
#43733=ORIENTED_EDGE('',*,*,#33028,.F.);
#43734=ORIENTED_EDGE('',*,*,#33031,.F.);
#43735=ORIENTED_EDGE('',*,*,#33034,.F.);
#43736=ORIENTED_EDGE('',*,*,#33035,.T.);
#43737=ORIENTED_EDGE('',*,*,#33036,.T.);
#43738=ORIENTED_EDGE('',*,*,#33037,.F.);
#43739=ORIENTED_EDGE('',*,*,#33038,.F.);
#43740=ORIENTED_EDGE('',*,*,#33039,.T.);
#43741=ORIENTED_EDGE('',*,*,#33040,.T.);
#43742=ORIENTED_EDGE('',*,*,#33035,.F.);
#43743=ORIENTED_EDGE('',*,*,#33041,.F.);
#43744=ORIENTED_EDGE('',*,*,#33042,.T.);
#43745=ORIENTED_EDGE('',*,*,#33043,.T.);
#43746=ORIENTED_EDGE('',*,*,#33039,.F.);
#43747=ORIENTED_EDGE('',*,*,#33044,.F.);
#43748=ORIENTED_EDGE('',*,*,#33037,.T.);
#43749=ORIENTED_EDGE('',*,*,#33045,.T.);
#43750=ORIENTED_EDGE('',*,*,#33042,.F.);
#43751=ORIENTED_EDGE('',*,*,#33045,.F.);
#43752=ORIENTED_EDGE('',*,*,#33036,.F.);
#43753=ORIENTED_EDGE('',*,*,#33040,.F.);
#43754=ORIENTED_EDGE('',*,*,#33043,.F.);
#43755=ORIENTED_EDGE('',*,*,#33046,.F.);
#43756=ORIENTED_EDGE('',*,*,#33047,.T.);
#43757=ORIENTED_EDGE('',*,*,#33048,.T.);
#43758=ORIENTED_EDGE('',*,*,#33049,.F.);
#43759=ORIENTED_EDGE('',*,*,#33050,.F.);
#43760=ORIENTED_EDGE('',*,*,#33051,.T.);
#43761=ORIENTED_EDGE('',*,*,#33052,.T.);
#43762=ORIENTED_EDGE('',*,*,#33047,.F.);
#43763=ORIENTED_EDGE('',*,*,#33053,.F.);
#43764=ORIENTED_EDGE('',*,*,#33054,.T.);
#43765=ORIENTED_EDGE('',*,*,#33055,.T.);
#43766=ORIENTED_EDGE('',*,*,#33051,.F.);
#43767=ORIENTED_EDGE('',*,*,#33056,.F.);
#43768=ORIENTED_EDGE('',*,*,#33049,.T.);
#43769=ORIENTED_EDGE('',*,*,#33057,.T.);
#43770=ORIENTED_EDGE('',*,*,#33054,.F.);
#43771=ORIENTED_EDGE('',*,*,#33057,.F.);
#43772=ORIENTED_EDGE('',*,*,#33048,.F.);
#43773=ORIENTED_EDGE('',*,*,#33052,.F.);
#43774=ORIENTED_EDGE('',*,*,#33055,.F.);
#43775=ORIENTED_EDGE('',*,*,#33058,.F.);
#43776=ORIENTED_EDGE('',*,*,#33059,.T.);
#43777=ORIENTED_EDGE('',*,*,#33060,.T.);
#43778=ORIENTED_EDGE('',*,*,#33061,.F.);
#43779=ORIENTED_EDGE('',*,*,#33062,.F.);
#43780=ORIENTED_EDGE('',*,*,#33063,.T.);
#43781=ORIENTED_EDGE('',*,*,#33064,.T.);
#43782=ORIENTED_EDGE('',*,*,#33059,.F.);
#43783=ORIENTED_EDGE('',*,*,#33065,.F.);
#43784=ORIENTED_EDGE('',*,*,#33066,.T.);
#43785=ORIENTED_EDGE('',*,*,#33067,.T.);
#43786=ORIENTED_EDGE('',*,*,#33063,.F.);
#43787=ORIENTED_EDGE('',*,*,#33068,.F.);
#43788=ORIENTED_EDGE('',*,*,#33061,.T.);
#43789=ORIENTED_EDGE('',*,*,#33069,.T.);
#43790=ORIENTED_EDGE('',*,*,#33066,.F.);
#43791=ORIENTED_EDGE('',*,*,#33069,.F.);
#43792=ORIENTED_EDGE('',*,*,#33060,.F.);
#43793=ORIENTED_EDGE('',*,*,#33064,.F.);
#43794=ORIENTED_EDGE('',*,*,#33067,.F.);
#43795=ORIENTED_EDGE('',*,*,#33070,.F.);
#43796=ORIENTED_EDGE('',*,*,#33071,.T.);
#43797=ORIENTED_EDGE('',*,*,#33072,.T.);
#43798=ORIENTED_EDGE('',*,*,#33073,.F.);
#43799=ORIENTED_EDGE('',*,*,#33074,.F.);
#43800=ORIENTED_EDGE('',*,*,#33075,.T.);
#43801=ORIENTED_EDGE('',*,*,#33076,.T.);
#43802=ORIENTED_EDGE('',*,*,#33071,.F.);
#43803=ORIENTED_EDGE('',*,*,#33077,.F.);
#43804=ORIENTED_EDGE('',*,*,#33078,.T.);
#43805=ORIENTED_EDGE('',*,*,#33079,.T.);
#43806=ORIENTED_EDGE('',*,*,#33075,.F.);
#43807=ORIENTED_EDGE('',*,*,#33080,.F.);
#43808=ORIENTED_EDGE('',*,*,#33073,.T.);
#43809=ORIENTED_EDGE('',*,*,#33081,.T.);
#43810=ORIENTED_EDGE('',*,*,#33078,.F.);
#43811=ORIENTED_EDGE('',*,*,#33081,.F.);
#43812=ORIENTED_EDGE('',*,*,#33072,.F.);
#43813=ORIENTED_EDGE('',*,*,#33076,.F.);
#43814=ORIENTED_EDGE('',*,*,#33079,.F.);
#43815=ORIENTED_EDGE('',*,*,#33082,.F.);
#43816=ORIENTED_EDGE('',*,*,#33083,.T.);
#43817=ORIENTED_EDGE('',*,*,#33084,.T.);
#43818=ORIENTED_EDGE('',*,*,#33085,.F.);
#43819=ORIENTED_EDGE('',*,*,#33086,.F.);
#43820=ORIENTED_EDGE('',*,*,#33087,.T.);
#43821=ORIENTED_EDGE('',*,*,#33088,.T.);
#43822=ORIENTED_EDGE('',*,*,#33083,.F.);
#43823=ORIENTED_EDGE('',*,*,#33089,.F.);
#43824=ORIENTED_EDGE('',*,*,#33090,.T.);
#43825=ORIENTED_EDGE('',*,*,#33091,.T.);
#43826=ORIENTED_EDGE('',*,*,#33087,.F.);
#43827=ORIENTED_EDGE('',*,*,#33092,.F.);
#43828=ORIENTED_EDGE('',*,*,#33085,.T.);
#43829=ORIENTED_EDGE('',*,*,#33093,.T.);
#43830=ORIENTED_EDGE('',*,*,#33090,.F.);
#43831=ORIENTED_EDGE('',*,*,#33093,.F.);
#43832=ORIENTED_EDGE('',*,*,#33084,.F.);
#43833=ORIENTED_EDGE('',*,*,#33088,.F.);
#43834=ORIENTED_EDGE('',*,*,#33091,.F.);
#43835=ORIENTED_EDGE('',*,*,#33094,.F.);
#43836=ORIENTED_EDGE('',*,*,#33095,.T.);
#43837=ORIENTED_EDGE('',*,*,#33096,.T.);
#43838=ORIENTED_EDGE('',*,*,#33097,.F.);
#43839=ORIENTED_EDGE('',*,*,#33098,.F.);
#43840=ORIENTED_EDGE('',*,*,#33099,.T.);
#43841=ORIENTED_EDGE('',*,*,#33100,.T.);
#43842=ORIENTED_EDGE('',*,*,#33095,.F.);
#43843=ORIENTED_EDGE('',*,*,#33101,.F.);
#43844=ORIENTED_EDGE('',*,*,#33102,.T.);
#43845=ORIENTED_EDGE('',*,*,#33103,.T.);
#43846=ORIENTED_EDGE('',*,*,#33099,.F.);
#43847=ORIENTED_EDGE('',*,*,#33104,.F.);
#43848=ORIENTED_EDGE('',*,*,#33097,.T.);
#43849=ORIENTED_EDGE('',*,*,#33105,.T.);
#43850=ORIENTED_EDGE('',*,*,#33102,.F.);
#43851=ORIENTED_EDGE('',*,*,#33105,.F.);
#43852=ORIENTED_EDGE('',*,*,#33096,.F.);
#43853=ORIENTED_EDGE('',*,*,#33100,.F.);
#43854=ORIENTED_EDGE('',*,*,#33103,.F.);
#43855=ORIENTED_EDGE('',*,*,#33106,.F.);
#43856=ORIENTED_EDGE('',*,*,#33107,.T.);
#43857=ORIENTED_EDGE('',*,*,#33108,.T.);
#43858=ORIENTED_EDGE('',*,*,#33109,.F.);
#43859=ORIENTED_EDGE('',*,*,#33110,.F.);
#43860=ORIENTED_EDGE('',*,*,#33111,.T.);
#43861=ORIENTED_EDGE('',*,*,#33112,.T.);
#43862=ORIENTED_EDGE('',*,*,#33107,.F.);
#43863=ORIENTED_EDGE('',*,*,#33113,.F.);
#43864=ORIENTED_EDGE('',*,*,#33114,.T.);
#43865=ORIENTED_EDGE('',*,*,#33115,.T.);
#43866=ORIENTED_EDGE('',*,*,#33111,.F.);
#43867=ORIENTED_EDGE('',*,*,#33116,.F.);
#43868=ORIENTED_EDGE('',*,*,#33109,.T.);
#43869=ORIENTED_EDGE('',*,*,#33117,.T.);
#43870=ORIENTED_EDGE('',*,*,#33114,.F.);
#43871=ORIENTED_EDGE('',*,*,#33117,.F.);
#43872=ORIENTED_EDGE('',*,*,#33108,.F.);
#43873=ORIENTED_EDGE('',*,*,#33112,.F.);
#43874=ORIENTED_EDGE('',*,*,#33115,.F.);
#43875=ORIENTED_EDGE('',*,*,#33118,.F.);
#43876=ORIENTED_EDGE('',*,*,#33119,.T.);
#43877=ORIENTED_EDGE('',*,*,#33120,.T.);
#43878=ORIENTED_EDGE('',*,*,#33121,.F.);
#43879=ORIENTED_EDGE('',*,*,#33122,.F.);
#43880=ORIENTED_EDGE('',*,*,#33123,.T.);
#43881=ORIENTED_EDGE('',*,*,#33124,.T.);
#43882=ORIENTED_EDGE('',*,*,#33119,.F.);
#43883=ORIENTED_EDGE('',*,*,#33125,.F.);
#43884=ORIENTED_EDGE('',*,*,#33126,.T.);
#43885=ORIENTED_EDGE('',*,*,#33127,.T.);
#43886=ORIENTED_EDGE('',*,*,#33123,.F.);
#43887=ORIENTED_EDGE('',*,*,#33128,.F.);
#43888=ORIENTED_EDGE('',*,*,#33121,.T.);
#43889=ORIENTED_EDGE('',*,*,#33129,.T.);
#43890=ORIENTED_EDGE('',*,*,#33126,.F.);
#43891=ORIENTED_EDGE('',*,*,#33129,.F.);
#43892=ORIENTED_EDGE('',*,*,#33120,.F.);
#43893=ORIENTED_EDGE('',*,*,#33124,.F.);
#43894=ORIENTED_EDGE('',*,*,#33127,.F.);
#43895=ORIENTED_EDGE('',*,*,#33130,.F.);
#43896=ORIENTED_EDGE('',*,*,#33131,.T.);
#43897=ORIENTED_EDGE('',*,*,#33132,.T.);
#43898=ORIENTED_EDGE('',*,*,#33133,.F.);
#43899=ORIENTED_EDGE('',*,*,#33134,.F.);
#43900=ORIENTED_EDGE('',*,*,#33135,.T.);
#43901=ORIENTED_EDGE('',*,*,#33136,.T.);
#43902=ORIENTED_EDGE('',*,*,#33131,.F.);
#43903=ORIENTED_EDGE('',*,*,#33137,.F.);
#43904=ORIENTED_EDGE('',*,*,#33138,.T.);
#43905=ORIENTED_EDGE('',*,*,#33139,.T.);
#43906=ORIENTED_EDGE('',*,*,#33135,.F.);
#43907=ORIENTED_EDGE('',*,*,#33140,.F.);
#43908=ORIENTED_EDGE('',*,*,#33133,.T.);
#43909=ORIENTED_EDGE('',*,*,#33141,.T.);
#43910=ORIENTED_EDGE('',*,*,#33138,.F.);
#43911=ORIENTED_EDGE('',*,*,#33141,.F.);
#43912=ORIENTED_EDGE('',*,*,#33132,.F.);
#43913=ORIENTED_EDGE('',*,*,#33136,.F.);
#43914=ORIENTED_EDGE('',*,*,#33139,.F.);
#43915=ORIENTED_EDGE('',*,*,#33142,.F.);
#43916=ORIENTED_EDGE('',*,*,#33143,.T.);
#43917=ORIENTED_EDGE('',*,*,#33144,.T.);
#43918=ORIENTED_EDGE('',*,*,#33145,.F.);
#43919=ORIENTED_EDGE('',*,*,#33146,.F.);
#43920=ORIENTED_EDGE('',*,*,#33147,.T.);
#43921=ORIENTED_EDGE('',*,*,#33148,.T.);
#43922=ORIENTED_EDGE('',*,*,#33143,.F.);
#43923=ORIENTED_EDGE('',*,*,#33149,.F.);
#43924=ORIENTED_EDGE('',*,*,#33150,.T.);
#43925=ORIENTED_EDGE('',*,*,#33151,.T.);
#43926=ORIENTED_EDGE('',*,*,#33147,.F.);
#43927=ORIENTED_EDGE('',*,*,#33152,.F.);
#43928=ORIENTED_EDGE('',*,*,#33145,.T.);
#43929=ORIENTED_EDGE('',*,*,#33153,.T.);
#43930=ORIENTED_EDGE('',*,*,#33150,.F.);
#43931=ORIENTED_EDGE('',*,*,#33153,.F.);
#43932=ORIENTED_EDGE('',*,*,#33144,.F.);
#43933=ORIENTED_EDGE('',*,*,#33148,.F.);
#43934=ORIENTED_EDGE('',*,*,#33151,.F.);
#43935=ORIENTED_EDGE('',*,*,#33154,.F.);
#43936=ORIENTED_EDGE('',*,*,#33155,.T.);
#43937=ORIENTED_EDGE('',*,*,#33156,.T.);
#43938=ORIENTED_EDGE('',*,*,#33157,.F.);
#43939=ORIENTED_EDGE('',*,*,#33158,.F.);
#43940=ORIENTED_EDGE('',*,*,#33159,.T.);
#43941=ORIENTED_EDGE('',*,*,#33160,.T.);
#43942=ORIENTED_EDGE('',*,*,#33155,.F.);
#43943=ORIENTED_EDGE('',*,*,#33161,.F.);
#43944=ORIENTED_EDGE('',*,*,#33162,.T.);
#43945=ORIENTED_EDGE('',*,*,#33163,.T.);
#43946=ORIENTED_EDGE('',*,*,#33159,.F.);
#43947=ORIENTED_EDGE('',*,*,#33164,.F.);
#43948=ORIENTED_EDGE('',*,*,#33157,.T.);
#43949=ORIENTED_EDGE('',*,*,#33165,.T.);
#43950=ORIENTED_EDGE('',*,*,#33162,.F.);
#43951=ORIENTED_EDGE('',*,*,#33165,.F.);
#43952=ORIENTED_EDGE('',*,*,#33156,.F.);
#43953=ORIENTED_EDGE('',*,*,#33160,.F.);
#43954=ORIENTED_EDGE('',*,*,#33163,.F.);
#43955=ORIENTED_EDGE('',*,*,#33166,.F.);
#43956=ORIENTED_EDGE('',*,*,#33167,.T.);
#43957=ORIENTED_EDGE('',*,*,#33168,.T.);
#43958=ORIENTED_EDGE('',*,*,#33169,.F.);
#43959=ORIENTED_EDGE('',*,*,#33170,.F.);
#43960=ORIENTED_EDGE('',*,*,#33171,.T.);
#43961=ORIENTED_EDGE('',*,*,#33172,.T.);
#43962=ORIENTED_EDGE('',*,*,#33167,.F.);
#43963=ORIENTED_EDGE('',*,*,#33173,.F.);
#43964=ORIENTED_EDGE('',*,*,#33174,.T.);
#43965=ORIENTED_EDGE('',*,*,#33175,.T.);
#43966=ORIENTED_EDGE('',*,*,#33171,.F.);
#43967=ORIENTED_EDGE('',*,*,#33176,.F.);
#43968=ORIENTED_EDGE('',*,*,#33169,.T.);
#43969=ORIENTED_EDGE('',*,*,#33177,.T.);
#43970=ORIENTED_EDGE('',*,*,#33174,.F.);
#43971=ORIENTED_EDGE('',*,*,#33177,.F.);
#43972=ORIENTED_EDGE('',*,*,#33168,.F.);
#43973=ORIENTED_EDGE('',*,*,#33172,.F.);
#43974=ORIENTED_EDGE('',*,*,#33175,.F.);
#43975=ORIENTED_EDGE('',*,*,#33178,.F.);
#43976=ORIENTED_EDGE('',*,*,#33179,.T.);
#43977=ORIENTED_EDGE('',*,*,#33180,.T.);
#43978=ORIENTED_EDGE('',*,*,#33181,.F.);
#43979=ORIENTED_EDGE('',*,*,#33182,.F.);
#43980=ORIENTED_EDGE('',*,*,#33183,.T.);
#43981=ORIENTED_EDGE('',*,*,#33184,.T.);
#43982=ORIENTED_EDGE('',*,*,#33179,.F.);
#43983=ORIENTED_EDGE('',*,*,#33185,.F.);
#43984=ORIENTED_EDGE('',*,*,#33186,.T.);
#43985=ORIENTED_EDGE('',*,*,#33187,.T.);
#43986=ORIENTED_EDGE('',*,*,#33183,.F.);
#43987=ORIENTED_EDGE('',*,*,#33188,.F.);
#43988=ORIENTED_EDGE('',*,*,#33181,.T.);
#43989=ORIENTED_EDGE('',*,*,#33189,.T.);
#43990=ORIENTED_EDGE('',*,*,#33186,.F.);
#43991=ORIENTED_EDGE('',*,*,#33189,.F.);
#43992=ORIENTED_EDGE('',*,*,#33180,.F.);
#43993=ORIENTED_EDGE('',*,*,#33184,.F.);
#43994=ORIENTED_EDGE('',*,*,#33187,.F.);
#43995=ORIENTED_EDGE('',*,*,#33190,.F.);
#43996=ORIENTED_EDGE('',*,*,#33191,.T.);
#43997=ORIENTED_EDGE('',*,*,#33192,.T.);
#43998=ORIENTED_EDGE('',*,*,#33193,.F.);
#43999=ORIENTED_EDGE('',*,*,#33194,.F.);
#44000=ORIENTED_EDGE('',*,*,#33195,.T.);
#44001=ORIENTED_EDGE('',*,*,#33196,.T.);
#44002=ORIENTED_EDGE('',*,*,#33191,.F.);
#44003=ORIENTED_EDGE('',*,*,#33197,.F.);
#44004=ORIENTED_EDGE('',*,*,#33198,.T.);
#44005=ORIENTED_EDGE('',*,*,#33199,.T.);
#44006=ORIENTED_EDGE('',*,*,#33195,.F.);
#44007=ORIENTED_EDGE('',*,*,#33200,.F.);
#44008=ORIENTED_EDGE('',*,*,#33193,.T.);
#44009=ORIENTED_EDGE('',*,*,#33201,.T.);
#44010=ORIENTED_EDGE('',*,*,#33198,.F.);
#44011=ORIENTED_EDGE('',*,*,#33201,.F.);
#44012=ORIENTED_EDGE('',*,*,#33192,.F.);
#44013=ORIENTED_EDGE('',*,*,#33196,.F.);
#44014=ORIENTED_EDGE('',*,*,#33199,.F.);
#44015=ORIENTED_EDGE('',*,*,#33202,.F.);
#44016=ORIENTED_EDGE('',*,*,#33203,.T.);
#44017=ORIENTED_EDGE('',*,*,#33204,.T.);
#44018=ORIENTED_EDGE('',*,*,#33205,.F.);
#44019=ORIENTED_EDGE('',*,*,#33206,.F.);
#44020=ORIENTED_EDGE('',*,*,#33207,.T.);
#44021=ORIENTED_EDGE('',*,*,#33208,.T.);
#44022=ORIENTED_EDGE('',*,*,#33203,.F.);
#44023=ORIENTED_EDGE('',*,*,#33209,.F.);
#44024=ORIENTED_EDGE('',*,*,#33210,.T.);
#44025=ORIENTED_EDGE('',*,*,#33211,.T.);
#44026=ORIENTED_EDGE('',*,*,#33207,.F.);
#44027=ORIENTED_EDGE('',*,*,#33212,.F.);
#44028=ORIENTED_EDGE('',*,*,#33205,.T.);
#44029=ORIENTED_EDGE('',*,*,#33213,.T.);
#44030=ORIENTED_EDGE('',*,*,#33210,.F.);
#44031=ORIENTED_EDGE('',*,*,#33213,.F.);
#44032=ORIENTED_EDGE('',*,*,#33204,.F.);
#44033=ORIENTED_EDGE('',*,*,#33208,.F.);
#44034=ORIENTED_EDGE('',*,*,#33211,.F.);
#44035=ORIENTED_EDGE('',*,*,#33214,.F.);
#44036=ORIENTED_EDGE('',*,*,#33215,.T.);
#44037=ORIENTED_EDGE('',*,*,#33216,.T.);
#44038=ORIENTED_EDGE('',*,*,#33217,.F.);
#44039=ORIENTED_EDGE('',*,*,#33218,.F.);
#44040=ORIENTED_EDGE('',*,*,#33219,.T.);
#44041=ORIENTED_EDGE('',*,*,#33220,.T.);
#44042=ORIENTED_EDGE('',*,*,#33215,.F.);
#44043=ORIENTED_EDGE('',*,*,#33221,.F.);
#44044=ORIENTED_EDGE('',*,*,#33222,.T.);
#44045=ORIENTED_EDGE('',*,*,#33223,.T.);
#44046=ORIENTED_EDGE('',*,*,#33219,.F.);
#44047=ORIENTED_EDGE('',*,*,#33224,.F.);
#44048=ORIENTED_EDGE('',*,*,#33217,.T.);
#44049=ORIENTED_EDGE('',*,*,#33225,.T.);
#44050=ORIENTED_EDGE('',*,*,#33222,.F.);
#44051=ORIENTED_EDGE('',*,*,#33225,.F.);
#44052=ORIENTED_EDGE('',*,*,#33216,.F.);
#44053=ORIENTED_EDGE('',*,*,#33220,.F.);
#44054=ORIENTED_EDGE('',*,*,#33223,.F.);
#44055=ORIENTED_EDGE('',*,*,#33226,.F.);
#44056=ORIENTED_EDGE('',*,*,#33227,.T.);
#44057=ORIENTED_EDGE('',*,*,#33228,.T.);
#44058=ORIENTED_EDGE('',*,*,#33229,.F.);
#44059=ORIENTED_EDGE('',*,*,#33230,.F.);
#44060=ORIENTED_EDGE('',*,*,#33231,.T.);
#44061=ORIENTED_EDGE('',*,*,#33232,.T.);
#44062=ORIENTED_EDGE('',*,*,#33227,.F.);
#44063=ORIENTED_EDGE('',*,*,#33233,.F.);
#44064=ORIENTED_EDGE('',*,*,#33234,.T.);
#44065=ORIENTED_EDGE('',*,*,#33235,.T.);
#44066=ORIENTED_EDGE('',*,*,#33231,.F.);
#44067=ORIENTED_EDGE('',*,*,#33236,.F.);
#44068=ORIENTED_EDGE('',*,*,#33229,.T.);
#44069=ORIENTED_EDGE('',*,*,#33237,.T.);
#44070=ORIENTED_EDGE('',*,*,#33234,.F.);
#44071=ORIENTED_EDGE('',*,*,#33237,.F.);
#44072=ORIENTED_EDGE('',*,*,#33228,.F.);
#44073=ORIENTED_EDGE('',*,*,#33232,.F.);
#44074=ORIENTED_EDGE('',*,*,#33235,.F.);
#44075=ORIENTED_EDGE('',*,*,#33238,.F.);
#44076=ORIENTED_EDGE('',*,*,#33239,.T.);
#44077=ORIENTED_EDGE('',*,*,#33240,.T.);
#44078=ORIENTED_EDGE('',*,*,#33241,.F.);
#44079=ORIENTED_EDGE('',*,*,#33242,.F.);
#44080=ORIENTED_EDGE('',*,*,#33243,.T.);
#44081=ORIENTED_EDGE('',*,*,#33244,.T.);
#44082=ORIENTED_EDGE('',*,*,#33239,.F.);
#44083=ORIENTED_EDGE('',*,*,#33245,.F.);
#44084=ORIENTED_EDGE('',*,*,#33246,.T.);
#44085=ORIENTED_EDGE('',*,*,#33247,.T.);
#44086=ORIENTED_EDGE('',*,*,#33243,.F.);
#44087=ORIENTED_EDGE('',*,*,#33248,.F.);
#44088=ORIENTED_EDGE('',*,*,#33241,.T.);
#44089=ORIENTED_EDGE('',*,*,#33249,.T.);
#44090=ORIENTED_EDGE('',*,*,#33246,.F.);
#44091=ORIENTED_EDGE('',*,*,#33249,.F.);
#44092=ORIENTED_EDGE('',*,*,#33240,.F.);
#44093=ORIENTED_EDGE('',*,*,#33244,.F.);
#44094=ORIENTED_EDGE('',*,*,#33247,.F.);
#44095=ORIENTED_EDGE('',*,*,#33250,.F.);
#44096=ORIENTED_EDGE('',*,*,#33251,.T.);
#44097=ORIENTED_EDGE('',*,*,#33252,.T.);
#44098=ORIENTED_EDGE('',*,*,#33253,.F.);
#44099=ORIENTED_EDGE('',*,*,#33254,.F.);
#44100=ORIENTED_EDGE('',*,*,#33255,.T.);
#44101=ORIENTED_EDGE('',*,*,#33256,.T.);
#44102=ORIENTED_EDGE('',*,*,#33251,.F.);
#44103=ORIENTED_EDGE('',*,*,#33257,.F.);
#44104=ORIENTED_EDGE('',*,*,#33258,.T.);
#44105=ORIENTED_EDGE('',*,*,#33259,.T.);
#44106=ORIENTED_EDGE('',*,*,#33255,.F.);
#44107=ORIENTED_EDGE('',*,*,#33260,.F.);
#44108=ORIENTED_EDGE('',*,*,#33253,.T.);
#44109=ORIENTED_EDGE('',*,*,#33261,.T.);
#44110=ORIENTED_EDGE('',*,*,#33258,.F.);
#44111=ORIENTED_EDGE('',*,*,#33261,.F.);
#44112=ORIENTED_EDGE('',*,*,#33252,.F.);
#44113=ORIENTED_EDGE('',*,*,#33256,.F.);
#44114=ORIENTED_EDGE('',*,*,#33259,.F.);
#44115=ORIENTED_EDGE('',*,*,#33262,.F.);
#44116=ORIENTED_EDGE('',*,*,#33263,.T.);
#44117=ORIENTED_EDGE('',*,*,#33264,.T.);
#44118=ORIENTED_EDGE('',*,*,#33265,.F.);
#44119=ORIENTED_EDGE('',*,*,#33266,.F.);
#44120=ORIENTED_EDGE('',*,*,#33267,.T.);
#44121=ORIENTED_EDGE('',*,*,#33268,.T.);
#44122=ORIENTED_EDGE('',*,*,#33263,.F.);
#44123=ORIENTED_EDGE('',*,*,#33269,.F.);
#44124=ORIENTED_EDGE('',*,*,#33270,.T.);
#44125=ORIENTED_EDGE('',*,*,#33271,.T.);
#44126=ORIENTED_EDGE('',*,*,#33267,.F.);
#44127=ORIENTED_EDGE('',*,*,#33272,.F.);
#44128=ORIENTED_EDGE('',*,*,#33265,.T.);
#44129=ORIENTED_EDGE('',*,*,#33273,.T.);
#44130=ORIENTED_EDGE('',*,*,#33270,.F.);
#44131=ORIENTED_EDGE('',*,*,#33273,.F.);
#44132=ORIENTED_EDGE('',*,*,#33264,.F.);
#44133=ORIENTED_EDGE('',*,*,#33268,.F.);
#44134=ORIENTED_EDGE('',*,*,#33271,.F.);
#44135=ORIENTED_EDGE('',*,*,#33274,.F.);
#44136=ORIENTED_EDGE('',*,*,#33275,.T.);
#44137=ORIENTED_EDGE('',*,*,#33276,.T.);
#44138=ORIENTED_EDGE('',*,*,#33277,.F.);
#44139=ORIENTED_EDGE('',*,*,#33278,.F.);
#44140=ORIENTED_EDGE('',*,*,#33279,.T.);
#44141=ORIENTED_EDGE('',*,*,#33280,.T.);
#44142=ORIENTED_EDGE('',*,*,#33275,.F.);
#44143=ORIENTED_EDGE('',*,*,#33281,.F.);
#44144=ORIENTED_EDGE('',*,*,#33282,.T.);
#44145=ORIENTED_EDGE('',*,*,#33283,.T.);
#44146=ORIENTED_EDGE('',*,*,#33279,.F.);
#44147=ORIENTED_EDGE('',*,*,#33284,.F.);
#44148=ORIENTED_EDGE('',*,*,#33277,.T.);
#44149=ORIENTED_EDGE('',*,*,#33285,.T.);
#44150=ORIENTED_EDGE('',*,*,#33282,.F.);
#44151=ORIENTED_EDGE('',*,*,#33285,.F.);
#44152=ORIENTED_EDGE('',*,*,#33276,.F.);
#44153=ORIENTED_EDGE('',*,*,#33280,.F.);
#44154=ORIENTED_EDGE('',*,*,#33283,.F.);
#44155=ORIENTED_EDGE('',*,*,#33286,.F.);
#44156=ORIENTED_EDGE('',*,*,#33287,.T.);
#44157=ORIENTED_EDGE('',*,*,#33288,.T.);
#44158=ORIENTED_EDGE('',*,*,#33289,.F.);
#44159=ORIENTED_EDGE('',*,*,#33290,.F.);
#44160=ORIENTED_EDGE('',*,*,#33291,.T.);
#44161=ORIENTED_EDGE('',*,*,#33292,.T.);
#44162=ORIENTED_EDGE('',*,*,#33287,.F.);
#44163=ORIENTED_EDGE('',*,*,#33293,.F.);
#44164=ORIENTED_EDGE('',*,*,#33294,.T.);
#44165=ORIENTED_EDGE('',*,*,#33295,.T.);
#44166=ORIENTED_EDGE('',*,*,#33291,.F.);
#44167=ORIENTED_EDGE('',*,*,#33296,.F.);
#44168=ORIENTED_EDGE('',*,*,#33289,.T.);
#44169=ORIENTED_EDGE('',*,*,#33297,.T.);
#44170=ORIENTED_EDGE('',*,*,#33294,.F.);
#44171=ORIENTED_EDGE('',*,*,#33297,.F.);
#44172=ORIENTED_EDGE('',*,*,#33288,.F.);
#44173=ORIENTED_EDGE('',*,*,#33292,.F.);
#44174=ORIENTED_EDGE('',*,*,#33295,.F.);
#44175=ORIENTED_EDGE('',*,*,#33298,.F.);
#44176=ORIENTED_EDGE('',*,*,#33299,.T.);
#44177=ORIENTED_EDGE('',*,*,#33300,.T.);
#44178=ORIENTED_EDGE('',*,*,#33301,.F.);
#44179=ORIENTED_EDGE('',*,*,#33302,.F.);
#44180=ORIENTED_EDGE('',*,*,#33303,.T.);
#44181=ORIENTED_EDGE('',*,*,#33304,.T.);
#44182=ORIENTED_EDGE('',*,*,#33299,.F.);
#44183=ORIENTED_EDGE('',*,*,#33305,.F.);
#44184=ORIENTED_EDGE('',*,*,#33306,.T.);
#44185=ORIENTED_EDGE('',*,*,#33307,.T.);
#44186=ORIENTED_EDGE('',*,*,#33303,.F.);
#44187=ORIENTED_EDGE('',*,*,#33308,.F.);
#44188=ORIENTED_EDGE('',*,*,#33301,.T.);
#44189=ORIENTED_EDGE('',*,*,#33309,.T.);
#44190=ORIENTED_EDGE('',*,*,#33306,.F.);
#44191=ORIENTED_EDGE('',*,*,#33309,.F.);
#44192=ORIENTED_EDGE('',*,*,#33300,.F.);
#44193=ORIENTED_EDGE('',*,*,#33304,.F.);
#44194=ORIENTED_EDGE('',*,*,#33307,.F.);
#44195=ORIENTED_EDGE('',*,*,#33310,.F.);
#44196=ORIENTED_EDGE('',*,*,#33311,.T.);
#44197=ORIENTED_EDGE('',*,*,#33312,.T.);
#44198=ORIENTED_EDGE('',*,*,#33313,.F.);
#44199=ORIENTED_EDGE('',*,*,#33314,.F.);
#44200=ORIENTED_EDGE('',*,*,#33315,.T.);
#44201=ORIENTED_EDGE('',*,*,#33316,.T.);
#44202=ORIENTED_EDGE('',*,*,#33311,.F.);
#44203=ORIENTED_EDGE('',*,*,#33317,.F.);
#44204=ORIENTED_EDGE('',*,*,#33318,.T.);
#44205=ORIENTED_EDGE('',*,*,#33319,.T.);
#44206=ORIENTED_EDGE('',*,*,#33315,.F.);
#44207=ORIENTED_EDGE('',*,*,#33320,.F.);
#44208=ORIENTED_EDGE('',*,*,#33313,.T.);
#44209=ORIENTED_EDGE('',*,*,#33321,.T.);
#44210=ORIENTED_EDGE('',*,*,#33318,.F.);
#44211=ORIENTED_EDGE('',*,*,#33321,.F.);
#44212=ORIENTED_EDGE('',*,*,#33312,.F.);
#44213=ORIENTED_EDGE('',*,*,#33316,.F.);
#44214=ORIENTED_EDGE('',*,*,#33319,.F.);
#44215=ORIENTED_EDGE('',*,*,#33322,.F.);
#44216=ORIENTED_EDGE('',*,*,#33323,.T.);
#44217=ORIENTED_EDGE('',*,*,#33324,.T.);
#44218=ORIENTED_EDGE('',*,*,#33325,.F.);
#44219=ORIENTED_EDGE('',*,*,#33326,.F.);
#44220=ORIENTED_EDGE('',*,*,#33327,.T.);
#44221=ORIENTED_EDGE('',*,*,#33328,.T.);
#44222=ORIENTED_EDGE('',*,*,#33323,.F.);
#44223=ORIENTED_EDGE('',*,*,#33329,.F.);
#44224=ORIENTED_EDGE('',*,*,#33330,.T.);
#44225=ORIENTED_EDGE('',*,*,#33331,.T.);
#44226=ORIENTED_EDGE('',*,*,#33327,.F.);
#44227=ORIENTED_EDGE('',*,*,#33332,.F.);
#44228=ORIENTED_EDGE('',*,*,#33325,.T.);
#44229=ORIENTED_EDGE('',*,*,#33333,.T.);
#44230=ORIENTED_EDGE('',*,*,#33330,.F.);
#44231=ORIENTED_EDGE('',*,*,#33333,.F.);
#44232=ORIENTED_EDGE('',*,*,#33324,.F.);
#44233=ORIENTED_EDGE('',*,*,#33328,.F.);
#44234=ORIENTED_EDGE('',*,*,#33331,.F.);
#44235=ORIENTED_EDGE('',*,*,#33334,.F.);
#44236=ORIENTED_EDGE('',*,*,#33335,.T.);
#44237=ORIENTED_EDGE('',*,*,#33336,.T.);
#44238=ORIENTED_EDGE('',*,*,#33337,.F.);
#44239=ORIENTED_EDGE('',*,*,#33338,.F.);
#44240=ORIENTED_EDGE('',*,*,#33339,.T.);
#44241=ORIENTED_EDGE('',*,*,#33340,.T.);
#44242=ORIENTED_EDGE('',*,*,#33335,.F.);
#44243=ORIENTED_EDGE('',*,*,#33341,.F.);
#44244=ORIENTED_EDGE('',*,*,#33342,.T.);
#44245=ORIENTED_EDGE('',*,*,#33343,.T.);
#44246=ORIENTED_EDGE('',*,*,#33339,.F.);
#44247=ORIENTED_EDGE('',*,*,#33344,.F.);
#44248=ORIENTED_EDGE('',*,*,#33337,.T.);
#44249=ORIENTED_EDGE('',*,*,#33345,.T.);
#44250=ORIENTED_EDGE('',*,*,#33342,.F.);
#44251=ORIENTED_EDGE('',*,*,#33345,.F.);
#44252=ORIENTED_EDGE('',*,*,#33336,.F.);
#44253=ORIENTED_EDGE('',*,*,#33340,.F.);
#44254=ORIENTED_EDGE('',*,*,#33343,.F.);
#44255=ORIENTED_EDGE('',*,*,#33346,.F.);
#44256=ORIENTED_EDGE('',*,*,#33347,.T.);
#44257=ORIENTED_EDGE('',*,*,#33348,.T.);
#44258=ORIENTED_EDGE('',*,*,#33349,.F.);
#44259=ORIENTED_EDGE('',*,*,#33350,.F.);
#44260=ORIENTED_EDGE('',*,*,#33351,.T.);
#44261=ORIENTED_EDGE('',*,*,#33352,.T.);
#44262=ORIENTED_EDGE('',*,*,#33347,.F.);
#44263=ORIENTED_EDGE('',*,*,#33353,.F.);
#44264=ORIENTED_EDGE('',*,*,#33354,.T.);
#44265=ORIENTED_EDGE('',*,*,#33355,.T.);
#44266=ORIENTED_EDGE('',*,*,#33351,.F.);
#44267=ORIENTED_EDGE('',*,*,#33356,.F.);
#44268=ORIENTED_EDGE('',*,*,#33349,.T.);
#44269=ORIENTED_EDGE('',*,*,#33357,.T.);
#44270=ORIENTED_EDGE('',*,*,#33354,.F.);
#44271=ORIENTED_EDGE('',*,*,#33357,.F.);
#44272=ORIENTED_EDGE('',*,*,#33348,.F.);
#44273=ORIENTED_EDGE('',*,*,#33352,.F.);
#44274=ORIENTED_EDGE('',*,*,#33355,.F.);
#44275=ORIENTED_EDGE('',*,*,#33358,.F.);
#44276=ORIENTED_EDGE('',*,*,#33359,.T.);
#44277=ORIENTED_EDGE('',*,*,#33360,.T.);
#44278=ORIENTED_EDGE('',*,*,#33361,.F.);
#44279=ORIENTED_EDGE('',*,*,#33362,.F.);
#44280=ORIENTED_EDGE('',*,*,#33363,.T.);
#44281=ORIENTED_EDGE('',*,*,#33364,.T.);
#44282=ORIENTED_EDGE('',*,*,#33359,.F.);
#44283=ORIENTED_EDGE('',*,*,#33365,.F.);
#44284=ORIENTED_EDGE('',*,*,#33366,.T.);
#44285=ORIENTED_EDGE('',*,*,#33367,.T.);
#44286=ORIENTED_EDGE('',*,*,#33363,.F.);
#44287=ORIENTED_EDGE('',*,*,#33368,.F.);
#44288=ORIENTED_EDGE('',*,*,#33361,.T.);
#44289=ORIENTED_EDGE('',*,*,#33369,.T.);
#44290=ORIENTED_EDGE('',*,*,#33366,.F.);
#44291=ORIENTED_EDGE('',*,*,#33369,.F.);
#44292=ORIENTED_EDGE('',*,*,#33360,.F.);
#44293=ORIENTED_EDGE('',*,*,#33364,.F.);
#44294=ORIENTED_EDGE('',*,*,#33367,.F.);
#44295=ORIENTED_EDGE('',*,*,#33370,.F.);
#44296=ORIENTED_EDGE('',*,*,#33371,.T.);
#44297=ORIENTED_EDGE('',*,*,#33372,.T.);
#44298=ORIENTED_EDGE('',*,*,#33373,.F.);
#44299=ORIENTED_EDGE('',*,*,#33374,.F.);
#44300=ORIENTED_EDGE('',*,*,#33375,.T.);
#44301=ORIENTED_EDGE('',*,*,#33376,.T.);
#44302=ORIENTED_EDGE('',*,*,#33371,.F.);
#44303=ORIENTED_EDGE('',*,*,#33377,.F.);
#44304=ORIENTED_EDGE('',*,*,#33378,.T.);
#44305=ORIENTED_EDGE('',*,*,#33379,.T.);
#44306=ORIENTED_EDGE('',*,*,#33375,.F.);
#44307=ORIENTED_EDGE('',*,*,#33380,.F.);
#44308=ORIENTED_EDGE('',*,*,#33373,.T.);
#44309=ORIENTED_EDGE('',*,*,#33381,.T.);
#44310=ORIENTED_EDGE('',*,*,#33378,.F.);
#44311=ORIENTED_EDGE('',*,*,#33381,.F.);
#44312=ORIENTED_EDGE('',*,*,#33372,.F.);
#44313=ORIENTED_EDGE('',*,*,#33376,.F.);
#44314=ORIENTED_EDGE('',*,*,#33379,.F.);
#44315=ORIENTED_EDGE('',*,*,#33382,.F.);
#44316=ORIENTED_EDGE('',*,*,#33383,.T.);
#44317=ORIENTED_EDGE('',*,*,#33384,.T.);
#44318=ORIENTED_EDGE('',*,*,#33385,.F.);
#44319=ORIENTED_EDGE('',*,*,#33386,.F.);
#44320=ORIENTED_EDGE('',*,*,#33387,.T.);
#44321=ORIENTED_EDGE('',*,*,#33388,.T.);
#44322=ORIENTED_EDGE('',*,*,#33383,.F.);
#44323=ORIENTED_EDGE('',*,*,#33389,.F.);
#44324=ORIENTED_EDGE('',*,*,#33390,.T.);
#44325=ORIENTED_EDGE('',*,*,#33391,.T.);
#44326=ORIENTED_EDGE('',*,*,#33387,.F.);
#44327=ORIENTED_EDGE('',*,*,#33392,.F.);
#44328=ORIENTED_EDGE('',*,*,#33385,.T.);
#44329=ORIENTED_EDGE('',*,*,#33393,.T.);
#44330=ORIENTED_EDGE('',*,*,#33390,.F.);
#44331=ORIENTED_EDGE('',*,*,#33393,.F.);
#44332=ORIENTED_EDGE('',*,*,#33384,.F.);
#44333=ORIENTED_EDGE('',*,*,#33388,.F.);
#44334=ORIENTED_EDGE('',*,*,#33391,.F.);
#44335=ORIENTED_EDGE('',*,*,#33394,.F.);
#44336=ORIENTED_EDGE('',*,*,#33395,.T.);
#44337=ORIENTED_EDGE('',*,*,#33396,.T.);
#44338=ORIENTED_EDGE('',*,*,#33397,.F.);
#44339=ORIENTED_EDGE('',*,*,#33398,.F.);
#44340=ORIENTED_EDGE('',*,*,#33399,.T.);
#44341=ORIENTED_EDGE('',*,*,#33400,.T.);
#44342=ORIENTED_EDGE('',*,*,#33395,.F.);
#44343=ORIENTED_EDGE('',*,*,#33401,.F.);
#44344=ORIENTED_EDGE('',*,*,#33402,.T.);
#44345=ORIENTED_EDGE('',*,*,#33403,.T.);
#44346=ORIENTED_EDGE('',*,*,#33399,.F.);
#44347=ORIENTED_EDGE('',*,*,#33404,.F.);
#44348=ORIENTED_EDGE('',*,*,#33397,.T.);
#44349=ORIENTED_EDGE('',*,*,#33405,.T.);
#44350=ORIENTED_EDGE('',*,*,#33402,.F.);
#44351=ORIENTED_EDGE('',*,*,#33405,.F.);
#44352=ORIENTED_EDGE('',*,*,#33396,.F.);
#44353=ORIENTED_EDGE('',*,*,#33400,.F.);
#44354=ORIENTED_EDGE('',*,*,#33403,.F.);
#44355=ORIENTED_EDGE('',*,*,#33406,.F.);
#44356=ORIENTED_EDGE('',*,*,#33407,.T.);
#44357=ORIENTED_EDGE('',*,*,#33408,.T.);
#44358=ORIENTED_EDGE('',*,*,#33409,.F.);
#44359=ORIENTED_EDGE('',*,*,#33410,.F.);
#44360=ORIENTED_EDGE('',*,*,#33411,.T.);
#44361=ORIENTED_EDGE('',*,*,#33412,.T.);
#44362=ORIENTED_EDGE('',*,*,#33407,.F.);
#44363=ORIENTED_EDGE('',*,*,#33413,.F.);
#44364=ORIENTED_EDGE('',*,*,#33414,.T.);
#44365=ORIENTED_EDGE('',*,*,#33415,.T.);
#44366=ORIENTED_EDGE('',*,*,#33411,.F.);
#44367=ORIENTED_EDGE('',*,*,#33416,.F.);
#44368=ORIENTED_EDGE('',*,*,#33409,.T.);
#44369=ORIENTED_EDGE('',*,*,#33417,.T.);
#44370=ORIENTED_EDGE('',*,*,#33414,.F.);
#44371=ORIENTED_EDGE('',*,*,#33417,.F.);
#44372=ORIENTED_EDGE('',*,*,#33408,.F.);
#44373=ORIENTED_EDGE('',*,*,#33412,.F.);
#44374=ORIENTED_EDGE('',*,*,#33415,.F.);
#44375=ORIENTED_EDGE('',*,*,#33418,.F.);
#44376=ORIENTED_EDGE('',*,*,#33419,.T.);
#44377=ORIENTED_EDGE('',*,*,#33420,.T.);
#44378=ORIENTED_EDGE('',*,*,#33421,.F.);
#44379=ORIENTED_EDGE('',*,*,#33422,.F.);
#44380=ORIENTED_EDGE('',*,*,#33423,.T.);
#44381=ORIENTED_EDGE('',*,*,#33424,.T.);
#44382=ORIENTED_EDGE('',*,*,#33419,.F.);
#44383=ORIENTED_EDGE('',*,*,#33425,.F.);
#44384=ORIENTED_EDGE('',*,*,#33426,.T.);
#44385=ORIENTED_EDGE('',*,*,#33427,.T.);
#44386=ORIENTED_EDGE('',*,*,#33423,.F.);
#44387=ORIENTED_EDGE('',*,*,#33428,.F.);
#44388=ORIENTED_EDGE('',*,*,#33421,.T.);
#44389=ORIENTED_EDGE('',*,*,#33429,.T.);
#44390=ORIENTED_EDGE('',*,*,#33426,.F.);
#44391=ORIENTED_EDGE('',*,*,#33429,.F.);
#44392=ORIENTED_EDGE('',*,*,#33420,.F.);
#44393=ORIENTED_EDGE('',*,*,#33424,.F.);
#44394=ORIENTED_EDGE('',*,*,#33427,.F.);
#44395=ORIENTED_EDGE('',*,*,#33430,.F.);
#44396=ORIENTED_EDGE('',*,*,#33431,.T.);
#44397=ORIENTED_EDGE('',*,*,#33432,.T.);
#44398=ORIENTED_EDGE('',*,*,#33433,.F.);
#44399=ORIENTED_EDGE('',*,*,#33434,.F.);
#44400=ORIENTED_EDGE('',*,*,#33435,.T.);
#44401=ORIENTED_EDGE('',*,*,#33436,.T.);
#44402=ORIENTED_EDGE('',*,*,#33431,.F.);
#44403=ORIENTED_EDGE('',*,*,#33437,.F.);
#44404=ORIENTED_EDGE('',*,*,#33438,.T.);
#44405=ORIENTED_EDGE('',*,*,#33439,.T.);
#44406=ORIENTED_EDGE('',*,*,#33435,.F.);
#44407=ORIENTED_EDGE('',*,*,#33440,.F.);
#44408=ORIENTED_EDGE('',*,*,#33433,.T.);
#44409=ORIENTED_EDGE('',*,*,#33441,.T.);
#44410=ORIENTED_EDGE('',*,*,#33438,.F.);
#44411=ORIENTED_EDGE('',*,*,#33441,.F.);
#44412=ORIENTED_EDGE('',*,*,#33432,.F.);
#44413=ORIENTED_EDGE('',*,*,#33436,.F.);
#44414=ORIENTED_EDGE('',*,*,#33439,.F.);
#44415=ORIENTED_EDGE('',*,*,#33442,.F.);
#44416=ORIENTED_EDGE('',*,*,#33443,.T.);
#44417=ORIENTED_EDGE('',*,*,#33444,.T.);
#44418=ORIENTED_EDGE('',*,*,#33445,.F.);
#44419=ORIENTED_EDGE('',*,*,#33446,.F.);
#44420=ORIENTED_EDGE('',*,*,#33447,.T.);
#44421=ORIENTED_EDGE('',*,*,#33448,.T.);
#44422=ORIENTED_EDGE('',*,*,#33443,.F.);
#44423=ORIENTED_EDGE('',*,*,#33449,.F.);
#44424=ORIENTED_EDGE('',*,*,#33450,.T.);
#44425=ORIENTED_EDGE('',*,*,#33451,.T.);
#44426=ORIENTED_EDGE('',*,*,#33447,.F.);
#44427=ORIENTED_EDGE('',*,*,#33452,.F.);
#44428=ORIENTED_EDGE('',*,*,#33445,.T.);
#44429=ORIENTED_EDGE('',*,*,#33453,.T.);
#44430=ORIENTED_EDGE('',*,*,#33450,.F.);
#44431=ORIENTED_EDGE('',*,*,#33453,.F.);
#44432=ORIENTED_EDGE('',*,*,#33444,.F.);
#44433=ORIENTED_EDGE('',*,*,#33448,.F.);
#44434=ORIENTED_EDGE('',*,*,#33451,.F.);
#44435=ORIENTED_EDGE('',*,*,#33454,.F.);
#44436=ORIENTED_EDGE('',*,*,#33455,.T.);
#44437=ORIENTED_EDGE('',*,*,#33456,.T.);
#44438=ORIENTED_EDGE('',*,*,#33457,.F.);
#44439=ORIENTED_EDGE('',*,*,#33458,.F.);
#44440=ORIENTED_EDGE('',*,*,#33459,.T.);
#44441=ORIENTED_EDGE('',*,*,#33460,.T.);
#44442=ORIENTED_EDGE('',*,*,#33455,.F.);
#44443=ORIENTED_EDGE('',*,*,#33461,.F.);
#44444=ORIENTED_EDGE('',*,*,#33462,.T.);
#44445=ORIENTED_EDGE('',*,*,#33463,.T.);
#44446=ORIENTED_EDGE('',*,*,#33459,.F.);
#44447=ORIENTED_EDGE('',*,*,#33464,.F.);
#44448=ORIENTED_EDGE('',*,*,#33457,.T.);
#44449=ORIENTED_EDGE('',*,*,#33465,.T.);
#44450=ORIENTED_EDGE('',*,*,#33462,.F.);
#44451=ORIENTED_EDGE('',*,*,#33465,.F.);
#44452=ORIENTED_EDGE('',*,*,#33456,.F.);
#44453=ORIENTED_EDGE('',*,*,#33460,.F.);
#44454=ORIENTED_EDGE('',*,*,#33463,.F.);
#44455=ORIENTED_EDGE('',*,*,#33466,.F.);
#44456=ORIENTED_EDGE('',*,*,#33467,.T.);
#44457=ORIENTED_EDGE('',*,*,#33468,.T.);
#44458=ORIENTED_EDGE('',*,*,#33469,.F.);
#44459=ORIENTED_EDGE('',*,*,#33470,.F.);
#44460=ORIENTED_EDGE('',*,*,#33471,.T.);
#44461=ORIENTED_EDGE('',*,*,#33472,.T.);
#44462=ORIENTED_EDGE('',*,*,#33467,.F.);
#44463=ORIENTED_EDGE('',*,*,#33473,.F.);
#44464=ORIENTED_EDGE('',*,*,#33474,.T.);
#44465=ORIENTED_EDGE('',*,*,#33475,.T.);
#44466=ORIENTED_EDGE('',*,*,#33471,.F.);
#44467=ORIENTED_EDGE('',*,*,#33476,.F.);
#44468=ORIENTED_EDGE('',*,*,#33469,.T.);
#44469=ORIENTED_EDGE('',*,*,#33477,.T.);
#44470=ORIENTED_EDGE('',*,*,#33474,.F.);
#44471=ORIENTED_EDGE('',*,*,#33477,.F.);
#44472=ORIENTED_EDGE('',*,*,#33468,.F.);
#44473=ORIENTED_EDGE('',*,*,#33472,.F.);
#44474=ORIENTED_EDGE('',*,*,#33475,.F.);
#44475=ORIENTED_EDGE('',*,*,#33478,.F.);
#44476=ORIENTED_EDGE('',*,*,#33479,.T.);
#44477=ORIENTED_EDGE('',*,*,#33480,.T.);
#44478=ORIENTED_EDGE('',*,*,#33481,.F.);
#44479=ORIENTED_EDGE('',*,*,#33482,.F.);
#44480=ORIENTED_EDGE('',*,*,#33483,.T.);
#44481=ORIENTED_EDGE('',*,*,#33484,.T.);
#44482=ORIENTED_EDGE('',*,*,#33479,.F.);
#44483=ORIENTED_EDGE('',*,*,#33485,.F.);
#44484=ORIENTED_EDGE('',*,*,#33486,.T.);
#44485=ORIENTED_EDGE('',*,*,#33487,.T.);
#44486=ORIENTED_EDGE('',*,*,#33483,.F.);
#44487=ORIENTED_EDGE('',*,*,#33488,.F.);
#44488=ORIENTED_EDGE('',*,*,#33481,.T.);
#44489=ORIENTED_EDGE('',*,*,#33489,.T.);
#44490=ORIENTED_EDGE('',*,*,#33486,.F.);
#44491=ORIENTED_EDGE('',*,*,#33489,.F.);
#44492=ORIENTED_EDGE('',*,*,#33480,.F.);
#44493=ORIENTED_EDGE('',*,*,#33484,.F.);
#44494=ORIENTED_EDGE('',*,*,#33487,.F.);
#44495=ORIENTED_EDGE('',*,*,#33490,.F.);
#44496=ORIENTED_EDGE('',*,*,#33491,.T.);
#44497=ORIENTED_EDGE('',*,*,#33492,.T.);
#44498=ORIENTED_EDGE('',*,*,#33493,.F.);
#44499=ORIENTED_EDGE('',*,*,#33494,.F.);
#44500=ORIENTED_EDGE('',*,*,#33495,.T.);
#44501=ORIENTED_EDGE('',*,*,#33496,.T.);
#44502=ORIENTED_EDGE('',*,*,#33491,.F.);
#44503=ORIENTED_EDGE('',*,*,#33497,.F.);
#44504=ORIENTED_EDGE('',*,*,#33498,.T.);
#44505=ORIENTED_EDGE('',*,*,#33499,.T.);
#44506=ORIENTED_EDGE('',*,*,#33495,.F.);
#44507=ORIENTED_EDGE('',*,*,#33500,.F.);
#44508=ORIENTED_EDGE('',*,*,#33493,.T.);
#44509=ORIENTED_EDGE('',*,*,#33501,.T.);
#44510=ORIENTED_EDGE('',*,*,#33498,.F.);
#44511=ORIENTED_EDGE('',*,*,#33501,.F.);
#44512=ORIENTED_EDGE('',*,*,#33492,.F.);
#44513=ORIENTED_EDGE('',*,*,#33496,.F.);
#44514=ORIENTED_EDGE('',*,*,#33499,.F.);
#44515=ORIENTED_EDGE('',*,*,#33502,.F.);
#44516=ORIENTED_EDGE('',*,*,#33503,.T.);
#44517=ORIENTED_EDGE('',*,*,#33504,.T.);
#44518=ORIENTED_EDGE('',*,*,#33505,.F.);
#44519=ORIENTED_EDGE('',*,*,#33506,.F.);
#44520=ORIENTED_EDGE('',*,*,#33507,.T.);
#44521=ORIENTED_EDGE('',*,*,#33508,.T.);
#44522=ORIENTED_EDGE('',*,*,#33503,.F.);
#44523=ORIENTED_EDGE('',*,*,#33509,.F.);
#44524=ORIENTED_EDGE('',*,*,#33510,.T.);
#44525=ORIENTED_EDGE('',*,*,#33511,.T.);
#44526=ORIENTED_EDGE('',*,*,#33507,.F.);
#44527=ORIENTED_EDGE('',*,*,#33512,.F.);
#44528=ORIENTED_EDGE('',*,*,#33505,.T.);
#44529=ORIENTED_EDGE('',*,*,#33513,.T.);
#44530=ORIENTED_EDGE('',*,*,#33510,.F.);
#44531=ORIENTED_EDGE('',*,*,#33513,.F.);
#44532=ORIENTED_EDGE('',*,*,#33504,.F.);
#44533=ORIENTED_EDGE('',*,*,#33508,.F.);
#44534=ORIENTED_EDGE('',*,*,#33511,.F.);
#44535=ORIENTED_EDGE('',*,*,#33514,.F.);
#44536=ORIENTED_EDGE('',*,*,#33515,.T.);
#44537=ORIENTED_EDGE('',*,*,#33516,.T.);
#44538=ORIENTED_EDGE('',*,*,#33517,.F.);
#44539=ORIENTED_EDGE('',*,*,#33518,.F.);
#44540=ORIENTED_EDGE('',*,*,#33519,.T.);
#44541=ORIENTED_EDGE('',*,*,#33520,.T.);
#44542=ORIENTED_EDGE('',*,*,#33515,.F.);
#44543=ORIENTED_EDGE('',*,*,#33521,.F.);
#44544=ORIENTED_EDGE('',*,*,#33522,.T.);
#44545=ORIENTED_EDGE('',*,*,#33523,.T.);
#44546=ORIENTED_EDGE('',*,*,#33519,.F.);
#44547=ORIENTED_EDGE('',*,*,#33524,.F.);
#44548=ORIENTED_EDGE('',*,*,#33517,.T.);
#44549=ORIENTED_EDGE('',*,*,#33525,.T.);
#44550=ORIENTED_EDGE('',*,*,#33522,.F.);
#44551=ORIENTED_EDGE('',*,*,#33525,.F.);
#44552=ORIENTED_EDGE('',*,*,#33516,.F.);
#44553=ORIENTED_EDGE('',*,*,#33520,.F.);
#44554=ORIENTED_EDGE('',*,*,#33523,.F.);
#44555=ORIENTED_EDGE('',*,*,#33526,.F.);
#44556=ORIENTED_EDGE('',*,*,#33527,.T.);
#44557=ORIENTED_EDGE('',*,*,#33528,.T.);
#44558=ORIENTED_EDGE('',*,*,#33529,.F.);
#44559=ORIENTED_EDGE('',*,*,#33530,.F.);
#44560=ORIENTED_EDGE('',*,*,#33531,.T.);
#44561=ORIENTED_EDGE('',*,*,#33532,.T.);
#44562=ORIENTED_EDGE('',*,*,#33527,.F.);
#44563=ORIENTED_EDGE('',*,*,#33533,.F.);
#44564=ORIENTED_EDGE('',*,*,#33534,.T.);
#44565=ORIENTED_EDGE('',*,*,#33535,.T.);
#44566=ORIENTED_EDGE('',*,*,#33531,.F.);
#44567=ORIENTED_EDGE('',*,*,#33536,.F.);
#44568=ORIENTED_EDGE('',*,*,#33529,.T.);
#44569=ORIENTED_EDGE('',*,*,#33537,.T.);
#44570=ORIENTED_EDGE('',*,*,#33534,.F.);
#44571=ORIENTED_EDGE('',*,*,#33537,.F.);
#44572=ORIENTED_EDGE('',*,*,#33528,.F.);
#44573=ORIENTED_EDGE('',*,*,#33532,.F.);
#44574=ORIENTED_EDGE('',*,*,#33535,.F.);
#44575=ORIENTED_EDGE('',*,*,#33538,.F.);
#44576=ORIENTED_EDGE('',*,*,#33539,.T.);
#44577=ORIENTED_EDGE('',*,*,#33540,.T.);
#44578=ORIENTED_EDGE('',*,*,#33541,.F.);
#44579=ORIENTED_EDGE('',*,*,#33542,.F.);
#44580=ORIENTED_EDGE('',*,*,#33543,.T.);
#44581=ORIENTED_EDGE('',*,*,#33544,.T.);
#44582=ORIENTED_EDGE('',*,*,#33539,.F.);
#44583=ORIENTED_EDGE('',*,*,#33545,.F.);
#44584=ORIENTED_EDGE('',*,*,#33546,.T.);
#44585=ORIENTED_EDGE('',*,*,#33547,.T.);
#44586=ORIENTED_EDGE('',*,*,#33543,.F.);
#44587=ORIENTED_EDGE('',*,*,#33548,.F.);
#44588=ORIENTED_EDGE('',*,*,#33541,.T.);
#44589=ORIENTED_EDGE('',*,*,#33549,.T.);
#44590=ORIENTED_EDGE('',*,*,#33546,.F.);
#44591=ORIENTED_EDGE('',*,*,#33549,.F.);
#44592=ORIENTED_EDGE('',*,*,#33540,.F.);
#44593=ORIENTED_EDGE('',*,*,#33544,.F.);
#44594=ORIENTED_EDGE('',*,*,#33547,.F.);
#44595=ORIENTED_EDGE('',*,*,#33550,.F.);
#44596=ORIENTED_EDGE('',*,*,#33551,.T.);
#44597=ORIENTED_EDGE('',*,*,#33552,.T.);
#44598=ORIENTED_EDGE('',*,*,#33553,.F.);
#44599=ORIENTED_EDGE('',*,*,#33554,.F.);
#44600=ORIENTED_EDGE('',*,*,#33555,.T.);
#44601=ORIENTED_EDGE('',*,*,#33556,.T.);
#44602=ORIENTED_EDGE('',*,*,#33551,.F.);
#44603=ORIENTED_EDGE('',*,*,#33557,.F.);
#44604=ORIENTED_EDGE('',*,*,#33558,.T.);
#44605=ORIENTED_EDGE('',*,*,#33559,.T.);
#44606=ORIENTED_EDGE('',*,*,#33555,.F.);
#44607=ORIENTED_EDGE('',*,*,#33560,.F.);
#44608=ORIENTED_EDGE('',*,*,#33553,.T.);
#44609=ORIENTED_EDGE('',*,*,#33561,.T.);
#44610=ORIENTED_EDGE('',*,*,#33558,.F.);
#44611=ORIENTED_EDGE('',*,*,#33561,.F.);
#44612=ORIENTED_EDGE('',*,*,#33552,.F.);
#44613=ORIENTED_EDGE('',*,*,#33556,.F.);
#44614=ORIENTED_EDGE('',*,*,#33559,.F.);
#44615=ORIENTED_EDGE('',*,*,#33562,.F.);
#44616=ORIENTED_EDGE('',*,*,#33563,.T.);
#44617=ORIENTED_EDGE('',*,*,#33564,.T.);
#44618=ORIENTED_EDGE('',*,*,#33565,.F.);
#44619=ORIENTED_EDGE('',*,*,#33566,.F.);
#44620=ORIENTED_EDGE('',*,*,#33567,.T.);
#44621=ORIENTED_EDGE('',*,*,#33568,.T.);
#44622=ORIENTED_EDGE('',*,*,#33563,.F.);
#44623=ORIENTED_EDGE('',*,*,#33569,.F.);
#44624=ORIENTED_EDGE('',*,*,#33570,.T.);
#44625=ORIENTED_EDGE('',*,*,#33571,.T.);
#44626=ORIENTED_EDGE('',*,*,#33567,.F.);
#44627=ORIENTED_EDGE('',*,*,#33572,.F.);
#44628=ORIENTED_EDGE('',*,*,#33565,.T.);
#44629=ORIENTED_EDGE('',*,*,#33573,.T.);
#44630=ORIENTED_EDGE('',*,*,#33570,.F.);
#44631=ORIENTED_EDGE('',*,*,#33573,.F.);
#44632=ORIENTED_EDGE('',*,*,#33564,.F.);
#44633=ORIENTED_EDGE('',*,*,#33568,.F.);
#44634=ORIENTED_EDGE('',*,*,#33571,.F.);
#44635=ORIENTED_EDGE('',*,*,#33574,.F.);
#44636=ORIENTED_EDGE('',*,*,#33575,.T.);
#44637=ORIENTED_EDGE('',*,*,#33576,.T.);
#44638=ORIENTED_EDGE('',*,*,#33577,.F.);
#44639=ORIENTED_EDGE('',*,*,#33578,.F.);
#44640=ORIENTED_EDGE('',*,*,#33579,.T.);
#44641=ORIENTED_EDGE('',*,*,#33580,.T.);
#44642=ORIENTED_EDGE('',*,*,#33575,.F.);
#44643=ORIENTED_EDGE('',*,*,#33581,.F.);
#44644=ORIENTED_EDGE('',*,*,#33582,.T.);
#44645=ORIENTED_EDGE('',*,*,#33583,.T.);
#44646=ORIENTED_EDGE('',*,*,#33579,.F.);
#44647=ORIENTED_EDGE('',*,*,#33584,.F.);
#44648=ORIENTED_EDGE('',*,*,#33577,.T.);
#44649=ORIENTED_EDGE('',*,*,#33585,.T.);
#44650=ORIENTED_EDGE('',*,*,#33582,.F.);
#44651=ORIENTED_EDGE('',*,*,#33585,.F.);
#44652=ORIENTED_EDGE('',*,*,#33576,.F.);
#44653=ORIENTED_EDGE('',*,*,#33580,.F.);
#44654=ORIENTED_EDGE('',*,*,#33583,.F.);
#44655=ORIENTED_EDGE('',*,*,#33586,.F.);
#44656=ORIENTED_EDGE('',*,*,#33587,.T.);
#44657=ORIENTED_EDGE('',*,*,#33588,.T.);
#44658=ORIENTED_EDGE('',*,*,#33589,.F.);
#44659=ORIENTED_EDGE('',*,*,#33590,.F.);
#44660=ORIENTED_EDGE('',*,*,#33591,.T.);
#44661=ORIENTED_EDGE('',*,*,#33592,.T.);
#44662=ORIENTED_EDGE('',*,*,#33587,.F.);
#44663=ORIENTED_EDGE('',*,*,#33593,.F.);
#44664=ORIENTED_EDGE('',*,*,#33594,.T.);
#44665=ORIENTED_EDGE('',*,*,#33595,.T.);
#44666=ORIENTED_EDGE('',*,*,#33591,.F.);
#44667=ORIENTED_EDGE('',*,*,#33596,.F.);
#44668=ORIENTED_EDGE('',*,*,#33589,.T.);
#44669=ORIENTED_EDGE('',*,*,#33597,.T.);
#44670=ORIENTED_EDGE('',*,*,#33594,.F.);
#44671=ORIENTED_EDGE('',*,*,#33597,.F.);
#44672=ORIENTED_EDGE('',*,*,#33588,.F.);
#44673=ORIENTED_EDGE('',*,*,#33592,.F.);
#44674=ORIENTED_EDGE('',*,*,#33595,.F.);
#44675=ORIENTED_EDGE('',*,*,#33598,.F.);
#44676=ORIENTED_EDGE('',*,*,#33599,.T.);
#44677=ORIENTED_EDGE('',*,*,#33600,.T.);
#44678=ORIENTED_EDGE('',*,*,#33601,.F.);
#44679=ORIENTED_EDGE('',*,*,#33602,.F.);
#44680=ORIENTED_EDGE('',*,*,#33603,.T.);
#44681=ORIENTED_EDGE('',*,*,#33604,.T.);
#44682=ORIENTED_EDGE('',*,*,#33599,.F.);
#44683=ORIENTED_EDGE('',*,*,#33605,.F.);
#44684=ORIENTED_EDGE('',*,*,#33606,.T.);
#44685=ORIENTED_EDGE('',*,*,#33607,.T.);
#44686=ORIENTED_EDGE('',*,*,#33603,.F.);
#44687=ORIENTED_EDGE('',*,*,#33608,.F.);
#44688=ORIENTED_EDGE('',*,*,#33601,.T.);
#44689=ORIENTED_EDGE('',*,*,#33609,.T.);
#44690=ORIENTED_EDGE('',*,*,#33606,.F.);
#44691=ORIENTED_EDGE('',*,*,#33609,.F.);
#44692=ORIENTED_EDGE('',*,*,#33600,.F.);
#44693=ORIENTED_EDGE('',*,*,#33604,.F.);
#44694=ORIENTED_EDGE('',*,*,#33607,.F.);
#44695=ORIENTED_EDGE('',*,*,#33610,.F.);
#44696=ORIENTED_EDGE('',*,*,#33611,.T.);
#44697=ORIENTED_EDGE('',*,*,#33612,.T.);
#44698=ORIENTED_EDGE('',*,*,#33613,.F.);
#44699=ORIENTED_EDGE('',*,*,#33614,.F.);
#44700=ORIENTED_EDGE('',*,*,#33615,.T.);
#44701=ORIENTED_EDGE('',*,*,#33616,.T.);
#44702=ORIENTED_EDGE('',*,*,#33611,.F.);
#44703=ORIENTED_EDGE('',*,*,#33617,.F.);
#44704=ORIENTED_EDGE('',*,*,#33618,.T.);
#44705=ORIENTED_EDGE('',*,*,#33619,.T.);
#44706=ORIENTED_EDGE('',*,*,#33615,.F.);
#44707=ORIENTED_EDGE('',*,*,#33620,.F.);
#44708=ORIENTED_EDGE('',*,*,#33613,.T.);
#44709=ORIENTED_EDGE('',*,*,#33621,.T.);
#44710=ORIENTED_EDGE('',*,*,#33618,.F.);
#44711=ORIENTED_EDGE('',*,*,#33621,.F.);
#44712=ORIENTED_EDGE('',*,*,#33612,.F.);
#44713=ORIENTED_EDGE('',*,*,#33616,.F.);
#44714=ORIENTED_EDGE('',*,*,#33619,.F.);
#44715=ORIENTED_EDGE('',*,*,#33622,.F.);
#44716=ORIENTED_EDGE('',*,*,#33623,.T.);
#44717=ORIENTED_EDGE('',*,*,#33624,.T.);
#44718=ORIENTED_EDGE('',*,*,#33625,.F.);
#44719=ORIENTED_EDGE('',*,*,#33626,.F.);
#44720=ORIENTED_EDGE('',*,*,#33627,.T.);
#44721=ORIENTED_EDGE('',*,*,#33628,.T.);
#44722=ORIENTED_EDGE('',*,*,#33623,.F.);
#44723=ORIENTED_EDGE('',*,*,#33629,.F.);
#44724=ORIENTED_EDGE('',*,*,#33630,.T.);
#44725=ORIENTED_EDGE('',*,*,#33631,.T.);
#44726=ORIENTED_EDGE('',*,*,#33627,.F.);
#44727=ORIENTED_EDGE('',*,*,#33632,.F.);
#44728=ORIENTED_EDGE('',*,*,#33625,.T.);
#44729=ORIENTED_EDGE('',*,*,#33633,.T.);
#44730=ORIENTED_EDGE('',*,*,#33630,.F.);
#44731=ORIENTED_EDGE('',*,*,#33633,.F.);
#44732=ORIENTED_EDGE('',*,*,#33624,.F.);
#44733=ORIENTED_EDGE('',*,*,#33628,.F.);
#44734=ORIENTED_EDGE('',*,*,#33631,.F.);
#44735=ORIENTED_EDGE('',*,*,#33634,.F.);
#44736=ORIENTED_EDGE('',*,*,#33635,.T.);
#44737=ORIENTED_EDGE('',*,*,#33636,.T.);
#44738=ORIENTED_EDGE('',*,*,#33637,.F.);
#44739=ORIENTED_EDGE('',*,*,#33638,.F.);
#44740=ORIENTED_EDGE('',*,*,#33639,.T.);
#44741=ORIENTED_EDGE('',*,*,#33640,.T.);
#44742=ORIENTED_EDGE('',*,*,#33635,.F.);
#44743=ORIENTED_EDGE('',*,*,#33641,.F.);
#44744=ORIENTED_EDGE('',*,*,#33642,.T.);
#44745=ORIENTED_EDGE('',*,*,#33643,.T.);
#44746=ORIENTED_EDGE('',*,*,#33639,.F.);
#44747=ORIENTED_EDGE('',*,*,#33644,.F.);
#44748=ORIENTED_EDGE('',*,*,#33637,.T.);
#44749=ORIENTED_EDGE('',*,*,#33645,.T.);
#44750=ORIENTED_EDGE('',*,*,#33642,.F.);
#44751=ORIENTED_EDGE('',*,*,#33645,.F.);
#44752=ORIENTED_EDGE('',*,*,#33636,.F.);
#44753=ORIENTED_EDGE('',*,*,#33640,.F.);
#44754=ORIENTED_EDGE('',*,*,#33643,.F.);
#44755=ORIENTED_EDGE('',*,*,#33646,.F.);
#44756=ORIENTED_EDGE('',*,*,#33647,.T.);
#44757=ORIENTED_EDGE('',*,*,#33648,.T.);
#44758=ORIENTED_EDGE('',*,*,#33649,.F.);
#44759=ORIENTED_EDGE('',*,*,#33650,.F.);
#44760=ORIENTED_EDGE('',*,*,#33651,.T.);
#44761=ORIENTED_EDGE('',*,*,#33652,.T.);
#44762=ORIENTED_EDGE('',*,*,#33647,.F.);
#44763=ORIENTED_EDGE('',*,*,#33653,.F.);
#44764=ORIENTED_EDGE('',*,*,#33654,.T.);
#44765=ORIENTED_EDGE('',*,*,#33655,.T.);
#44766=ORIENTED_EDGE('',*,*,#33651,.F.);
#44767=ORIENTED_EDGE('',*,*,#33656,.F.);
#44768=ORIENTED_EDGE('',*,*,#33649,.T.);
#44769=ORIENTED_EDGE('',*,*,#33657,.T.);
#44770=ORIENTED_EDGE('',*,*,#33654,.F.);
#44771=ORIENTED_EDGE('',*,*,#33657,.F.);
#44772=ORIENTED_EDGE('',*,*,#33648,.F.);
#44773=ORIENTED_EDGE('',*,*,#33652,.F.);
#44774=ORIENTED_EDGE('',*,*,#33655,.F.);
#44775=ORIENTED_EDGE('',*,*,#33658,.F.);
#44776=ORIENTED_EDGE('',*,*,#33659,.T.);
#44777=ORIENTED_EDGE('',*,*,#33660,.T.);
#44778=ORIENTED_EDGE('',*,*,#33661,.F.);
#44779=ORIENTED_EDGE('',*,*,#33662,.F.);
#44780=ORIENTED_EDGE('',*,*,#33663,.T.);
#44781=ORIENTED_EDGE('',*,*,#33664,.T.);
#44782=ORIENTED_EDGE('',*,*,#33659,.F.);
#44783=ORIENTED_EDGE('',*,*,#33665,.F.);
#44784=ORIENTED_EDGE('',*,*,#33666,.T.);
#44785=ORIENTED_EDGE('',*,*,#33667,.T.);
#44786=ORIENTED_EDGE('',*,*,#33663,.F.);
#44787=ORIENTED_EDGE('',*,*,#33668,.F.);
#44788=ORIENTED_EDGE('',*,*,#33661,.T.);
#44789=ORIENTED_EDGE('',*,*,#33669,.T.);
#44790=ORIENTED_EDGE('',*,*,#33666,.F.);
#44791=ORIENTED_EDGE('',*,*,#33669,.F.);
#44792=ORIENTED_EDGE('',*,*,#33660,.F.);
#44793=ORIENTED_EDGE('',*,*,#33664,.F.);
#44794=ORIENTED_EDGE('',*,*,#33667,.F.);
#44795=ORIENTED_EDGE('',*,*,#33670,.F.);
#44796=ORIENTED_EDGE('',*,*,#33671,.T.);
#44797=ORIENTED_EDGE('',*,*,#33672,.T.);
#44798=ORIENTED_EDGE('',*,*,#33673,.F.);
#44799=ORIENTED_EDGE('',*,*,#33674,.F.);
#44800=ORIENTED_EDGE('',*,*,#33675,.T.);
#44801=ORIENTED_EDGE('',*,*,#33676,.T.);
#44802=ORIENTED_EDGE('',*,*,#33671,.F.);
#44803=ORIENTED_EDGE('',*,*,#33677,.F.);
#44804=ORIENTED_EDGE('',*,*,#33678,.T.);
#44805=ORIENTED_EDGE('',*,*,#33679,.T.);
#44806=ORIENTED_EDGE('',*,*,#33675,.F.);
#44807=ORIENTED_EDGE('',*,*,#33680,.F.);
#44808=ORIENTED_EDGE('',*,*,#33673,.T.);
#44809=ORIENTED_EDGE('',*,*,#33681,.T.);
#44810=ORIENTED_EDGE('',*,*,#33678,.F.);
#44811=ORIENTED_EDGE('',*,*,#33681,.F.);
#44812=ORIENTED_EDGE('',*,*,#33672,.F.);
#44813=ORIENTED_EDGE('',*,*,#33676,.F.);
#44814=ORIENTED_EDGE('',*,*,#33679,.F.);
#44815=ORIENTED_EDGE('',*,*,#33682,.F.);
#44816=ORIENTED_EDGE('',*,*,#33683,.T.);
#44817=ORIENTED_EDGE('',*,*,#33684,.T.);
#44818=ORIENTED_EDGE('',*,*,#33685,.F.);
#44819=ORIENTED_EDGE('',*,*,#33686,.F.);
#44820=ORIENTED_EDGE('',*,*,#33687,.T.);
#44821=ORIENTED_EDGE('',*,*,#33688,.T.);
#44822=ORIENTED_EDGE('',*,*,#33683,.F.);
#44823=ORIENTED_EDGE('',*,*,#33689,.F.);
#44824=ORIENTED_EDGE('',*,*,#33690,.T.);
#44825=ORIENTED_EDGE('',*,*,#33691,.T.);
#44826=ORIENTED_EDGE('',*,*,#33687,.F.);
#44827=ORIENTED_EDGE('',*,*,#33692,.F.);
#44828=ORIENTED_EDGE('',*,*,#33685,.T.);
#44829=ORIENTED_EDGE('',*,*,#33693,.T.);
#44830=ORIENTED_EDGE('',*,*,#33690,.F.);
#44831=ORIENTED_EDGE('',*,*,#33693,.F.);
#44832=ORIENTED_EDGE('',*,*,#33684,.F.);
#44833=ORIENTED_EDGE('',*,*,#33688,.F.);
#44834=ORIENTED_EDGE('',*,*,#33691,.F.);
#44835=ORIENTED_EDGE('',*,*,#33694,.F.);
#44836=ORIENTED_EDGE('',*,*,#33695,.T.);
#44837=ORIENTED_EDGE('',*,*,#33696,.T.);
#44838=ORIENTED_EDGE('',*,*,#33697,.F.);
#44839=ORIENTED_EDGE('',*,*,#33698,.F.);
#44840=ORIENTED_EDGE('',*,*,#33699,.T.);
#44841=ORIENTED_EDGE('',*,*,#33700,.T.);
#44842=ORIENTED_EDGE('',*,*,#33695,.F.);
#44843=ORIENTED_EDGE('',*,*,#33701,.F.);
#44844=ORIENTED_EDGE('',*,*,#33702,.T.);
#44845=ORIENTED_EDGE('',*,*,#33703,.T.);
#44846=ORIENTED_EDGE('',*,*,#33699,.F.);
#44847=ORIENTED_EDGE('',*,*,#33704,.F.);
#44848=ORIENTED_EDGE('',*,*,#33697,.T.);
#44849=ORIENTED_EDGE('',*,*,#33705,.T.);
#44850=ORIENTED_EDGE('',*,*,#33702,.F.);
#44851=ORIENTED_EDGE('',*,*,#33705,.F.);
#44852=ORIENTED_EDGE('',*,*,#33696,.F.);
#44853=ORIENTED_EDGE('',*,*,#33700,.F.);
#44854=ORIENTED_EDGE('',*,*,#33703,.F.);
#44855=ORIENTED_EDGE('',*,*,#33706,.F.);
#44856=ORIENTED_EDGE('',*,*,#33707,.T.);
#44857=ORIENTED_EDGE('',*,*,#33708,.T.);
#44858=ORIENTED_EDGE('',*,*,#33709,.F.);
#44859=ORIENTED_EDGE('',*,*,#33710,.F.);
#44860=ORIENTED_EDGE('',*,*,#33711,.T.);
#44861=ORIENTED_EDGE('',*,*,#33712,.T.);
#44862=ORIENTED_EDGE('',*,*,#33707,.F.);
#44863=ORIENTED_EDGE('',*,*,#33713,.F.);
#44864=ORIENTED_EDGE('',*,*,#33714,.T.);
#44865=ORIENTED_EDGE('',*,*,#33715,.T.);
#44866=ORIENTED_EDGE('',*,*,#33711,.F.);
#44867=ORIENTED_EDGE('',*,*,#33716,.F.);
#44868=ORIENTED_EDGE('',*,*,#33709,.T.);
#44869=ORIENTED_EDGE('',*,*,#33717,.T.);
#44870=ORIENTED_EDGE('',*,*,#33714,.F.);
#44871=ORIENTED_EDGE('',*,*,#33717,.F.);
#44872=ORIENTED_EDGE('',*,*,#33708,.F.);
#44873=ORIENTED_EDGE('',*,*,#33712,.F.);
#44874=ORIENTED_EDGE('',*,*,#33715,.F.);
#44875=ORIENTED_EDGE('',*,*,#33718,.F.);
#44876=ORIENTED_EDGE('',*,*,#33719,.T.);
#44877=ORIENTED_EDGE('',*,*,#33720,.T.);
#44878=ORIENTED_EDGE('',*,*,#33721,.F.);
#44879=ORIENTED_EDGE('',*,*,#33722,.F.);
#44880=ORIENTED_EDGE('',*,*,#33723,.T.);
#44881=ORIENTED_EDGE('',*,*,#33724,.T.);
#44882=ORIENTED_EDGE('',*,*,#33719,.F.);
#44883=ORIENTED_EDGE('',*,*,#33725,.F.);
#44884=ORIENTED_EDGE('',*,*,#33726,.T.);
#44885=ORIENTED_EDGE('',*,*,#33727,.T.);
#44886=ORIENTED_EDGE('',*,*,#33723,.F.);
#44887=ORIENTED_EDGE('',*,*,#33728,.F.);
#44888=ORIENTED_EDGE('',*,*,#33721,.T.);
#44889=ORIENTED_EDGE('',*,*,#33729,.T.);
#44890=ORIENTED_EDGE('',*,*,#33726,.F.);
#44891=ORIENTED_EDGE('',*,*,#33729,.F.);
#44892=ORIENTED_EDGE('',*,*,#33720,.F.);
#44893=ORIENTED_EDGE('',*,*,#33724,.F.);
#44894=ORIENTED_EDGE('',*,*,#33727,.F.);
#44895=ORIENTED_EDGE('',*,*,#33730,.F.);
#44896=ORIENTED_EDGE('',*,*,#33731,.T.);
#44897=ORIENTED_EDGE('',*,*,#33732,.T.);
#44898=ORIENTED_EDGE('',*,*,#33733,.F.);
#44899=ORIENTED_EDGE('',*,*,#33734,.F.);
#44900=ORIENTED_EDGE('',*,*,#33735,.T.);
#44901=ORIENTED_EDGE('',*,*,#33736,.T.);
#44902=ORIENTED_EDGE('',*,*,#33731,.F.);
#44903=ORIENTED_EDGE('',*,*,#33737,.F.);
#44904=ORIENTED_EDGE('',*,*,#33738,.T.);
#44905=ORIENTED_EDGE('',*,*,#33739,.T.);
#44906=ORIENTED_EDGE('',*,*,#33735,.F.);
#44907=ORIENTED_EDGE('',*,*,#33740,.F.);
#44908=ORIENTED_EDGE('',*,*,#33733,.T.);
#44909=ORIENTED_EDGE('',*,*,#33741,.T.);
#44910=ORIENTED_EDGE('',*,*,#33738,.F.);
#44911=ORIENTED_EDGE('',*,*,#33741,.F.);
#44912=ORIENTED_EDGE('',*,*,#33732,.F.);
#44913=ORIENTED_EDGE('',*,*,#33736,.F.);
#44914=ORIENTED_EDGE('',*,*,#33739,.F.);
#44915=ORIENTED_EDGE('',*,*,#33742,.F.);
#44916=ORIENTED_EDGE('',*,*,#33743,.T.);
#44917=ORIENTED_EDGE('',*,*,#33744,.T.);
#44918=ORIENTED_EDGE('',*,*,#33745,.F.);
#44919=ORIENTED_EDGE('',*,*,#33746,.F.);
#44920=ORIENTED_EDGE('',*,*,#33747,.T.);
#44921=ORIENTED_EDGE('',*,*,#33748,.T.);
#44922=ORIENTED_EDGE('',*,*,#33743,.F.);
#44923=ORIENTED_EDGE('',*,*,#33749,.F.);
#44924=ORIENTED_EDGE('',*,*,#33750,.T.);
#44925=ORIENTED_EDGE('',*,*,#33751,.T.);
#44926=ORIENTED_EDGE('',*,*,#33747,.F.);
#44927=ORIENTED_EDGE('',*,*,#33752,.F.);
#44928=ORIENTED_EDGE('',*,*,#33745,.T.);
#44929=ORIENTED_EDGE('',*,*,#33753,.T.);
#44930=ORIENTED_EDGE('',*,*,#33750,.F.);
#44931=ORIENTED_EDGE('',*,*,#33753,.F.);
#44932=ORIENTED_EDGE('',*,*,#33744,.F.);
#44933=ORIENTED_EDGE('',*,*,#33748,.F.);
#44934=ORIENTED_EDGE('',*,*,#33751,.F.);
#44935=ORIENTED_EDGE('',*,*,#33754,.F.);
#44936=ORIENTED_EDGE('',*,*,#33755,.T.);
#44937=ORIENTED_EDGE('',*,*,#33756,.T.);
#44938=ORIENTED_EDGE('',*,*,#33757,.F.);
#44939=ORIENTED_EDGE('',*,*,#33758,.F.);
#44940=ORIENTED_EDGE('',*,*,#33759,.T.);
#44941=ORIENTED_EDGE('',*,*,#33760,.T.);
#44942=ORIENTED_EDGE('',*,*,#33755,.F.);
#44943=ORIENTED_EDGE('',*,*,#33761,.F.);
#44944=ORIENTED_EDGE('',*,*,#33762,.T.);
#44945=ORIENTED_EDGE('',*,*,#33763,.T.);
#44946=ORIENTED_EDGE('',*,*,#33759,.F.);
#44947=ORIENTED_EDGE('',*,*,#33764,.F.);
#44948=ORIENTED_EDGE('',*,*,#33757,.T.);
#44949=ORIENTED_EDGE('',*,*,#33765,.T.);
#44950=ORIENTED_EDGE('',*,*,#33762,.F.);
#44951=ORIENTED_EDGE('',*,*,#33765,.F.);
#44952=ORIENTED_EDGE('',*,*,#33756,.F.);
#44953=ORIENTED_EDGE('',*,*,#33760,.F.);
#44954=ORIENTED_EDGE('',*,*,#33763,.F.);
#44955=ORIENTED_EDGE('',*,*,#33766,.F.);
#44956=ORIENTED_EDGE('',*,*,#33767,.T.);
#44957=ORIENTED_EDGE('',*,*,#33768,.T.);
#44958=ORIENTED_EDGE('',*,*,#33769,.F.);
#44959=ORIENTED_EDGE('',*,*,#33770,.F.);
#44960=ORIENTED_EDGE('',*,*,#33771,.T.);
#44961=ORIENTED_EDGE('',*,*,#33772,.T.);
#44962=ORIENTED_EDGE('',*,*,#33767,.F.);
#44963=ORIENTED_EDGE('',*,*,#33773,.F.);
#44964=ORIENTED_EDGE('',*,*,#33774,.T.);
#44965=ORIENTED_EDGE('',*,*,#33775,.T.);
#44966=ORIENTED_EDGE('',*,*,#33771,.F.);
#44967=ORIENTED_EDGE('',*,*,#33776,.F.);
#44968=ORIENTED_EDGE('',*,*,#33769,.T.);
#44969=ORIENTED_EDGE('',*,*,#33777,.T.);
#44970=ORIENTED_EDGE('',*,*,#33774,.F.);
#44971=ORIENTED_EDGE('',*,*,#33777,.F.);
#44972=ORIENTED_EDGE('',*,*,#33768,.F.);
#44973=ORIENTED_EDGE('',*,*,#33772,.F.);
#44974=ORIENTED_EDGE('',*,*,#33775,.F.);
#44975=ORIENTED_EDGE('',*,*,#33778,.F.);
#44976=ORIENTED_EDGE('',*,*,#33779,.T.);
#44977=ORIENTED_EDGE('',*,*,#33780,.T.);
#44978=ORIENTED_EDGE('',*,*,#33781,.F.);
#44979=ORIENTED_EDGE('',*,*,#33782,.F.);
#44980=ORIENTED_EDGE('',*,*,#33783,.T.);
#44981=ORIENTED_EDGE('',*,*,#33784,.T.);
#44982=ORIENTED_EDGE('',*,*,#33779,.F.);
#44983=ORIENTED_EDGE('',*,*,#33785,.F.);
#44984=ORIENTED_EDGE('',*,*,#33786,.T.);
#44985=ORIENTED_EDGE('',*,*,#33787,.T.);
#44986=ORIENTED_EDGE('',*,*,#33783,.F.);
#44987=ORIENTED_EDGE('',*,*,#33788,.F.);
#44988=ORIENTED_EDGE('',*,*,#33781,.T.);
#44989=ORIENTED_EDGE('',*,*,#33789,.T.);
#44990=ORIENTED_EDGE('',*,*,#33786,.F.);
#44991=ORIENTED_EDGE('',*,*,#33789,.F.);
#44992=ORIENTED_EDGE('',*,*,#33780,.F.);
#44993=ORIENTED_EDGE('',*,*,#33784,.F.);
#44994=ORIENTED_EDGE('',*,*,#33787,.F.);
#44995=ORIENTED_EDGE('',*,*,#33790,.F.);
#44996=ORIENTED_EDGE('',*,*,#33791,.T.);
#44997=ORIENTED_EDGE('',*,*,#33792,.T.);
#44998=ORIENTED_EDGE('',*,*,#33793,.F.);
#44999=ORIENTED_EDGE('',*,*,#33794,.F.);
#45000=ORIENTED_EDGE('',*,*,#33795,.T.);
#45001=ORIENTED_EDGE('',*,*,#33796,.T.);
#45002=ORIENTED_EDGE('',*,*,#33791,.F.);
#45003=ORIENTED_EDGE('',*,*,#33797,.F.);
#45004=ORIENTED_EDGE('',*,*,#33798,.T.);
#45005=ORIENTED_EDGE('',*,*,#33799,.T.);
#45006=ORIENTED_EDGE('',*,*,#33795,.F.);
#45007=ORIENTED_EDGE('',*,*,#33800,.F.);
#45008=ORIENTED_EDGE('',*,*,#33793,.T.);
#45009=ORIENTED_EDGE('',*,*,#33801,.T.);
#45010=ORIENTED_EDGE('',*,*,#33798,.F.);
#45011=ORIENTED_EDGE('',*,*,#33801,.F.);
#45012=ORIENTED_EDGE('',*,*,#33792,.F.);
#45013=ORIENTED_EDGE('',*,*,#33796,.F.);
#45014=ORIENTED_EDGE('',*,*,#33799,.F.);
#45015=ORIENTED_EDGE('',*,*,#33802,.F.);
#45016=ORIENTED_EDGE('',*,*,#33803,.T.);
#45017=ORIENTED_EDGE('',*,*,#33804,.T.);
#45018=ORIENTED_EDGE('',*,*,#33805,.F.);
#45019=ORIENTED_EDGE('',*,*,#33806,.F.);
#45020=ORIENTED_EDGE('',*,*,#33807,.T.);
#45021=ORIENTED_EDGE('',*,*,#33808,.T.);
#45022=ORIENTED_EDGE('',*,*,#33803,.F.);
#45023=ORIENTED_EDGE('',*,*,#33809,.F.);
#45024=ORIENTED_EDGE('',*,*,#33810,.T.);
#45025=ORIENTED_EDGE('',*,*,#33811,.T.);
#45026=ORIENTED_EDGE('',*,*,#33807,.F.);
#45027=ORIENTED_EDGE('',*,*,#33812,.F.);
#45028=ORIENTED_EDGE('',*,*,#33805,.T.);
#45029=ORIENTED_EDGE('',*,*,#33813,.T.);
#45030=ORIENTED_EDGE('',*,*,#33810,.F.);
#45031=ORIENTED_EDGE('',*,*,#33813,.F.);
#45032=ORIENTED_EDGE('',*,*,#33804,.F.);
#45033=ORIENTED_EDGE('',*,*,#33808,.F.);
#45034=ORIENTED_EDGE('',*,*,#33811,.F.);
#45035=ORIENTED_EDGE('',*,*,#33814,.F.);
#45036=ORIENTED_EDGE('',*,*,#33815,.T.);
#45037=ORIENTED_EDGE('',*,*,#33816,.T.);
#45038=ORIENTED_EDGE('',*,*,#33817,.F.);
#45039=ORIENTED_EDGE('',*,*,#33818,.F.);
#45040=ORIENTED_EDGE('',*,*,#33819,.T.);
#45041=ORIENTED_EDGE('',*,*,#33820,.T.);
#45042=ORIENTED_EDGE('',*,*,#33815,.F.);
#45043=ORIENTED_EDGE('',*,*,#33821,.F.);
#45044=ORIENTED_EDGE('',*,*,#33822,.T.);
#45045=ORIENTED_EDGE('',*,*,#33823,.T.);
#45046=ORIENTED_EDGE('',*,*,#33819,.F.);
#45047=ORIENTED_EDGE('',*,*,#33824,.F.);
#45048=ORIENTED_EDGE('',*,*,#33817,.T.);
#45049=ORIENTED_EDGE('',*,*,#33825,.T.);
#45050=ORIENTED_EDGE('',*,*,#33822,.F.);
#45051=ORIENTED_EDGE('',*,*,#33825,.F.);
#45052=ORIENTED_EDGE('',*,*,#33816,.F.);
#45053=ORIENTED_EDGE('',*,*,#33820,.F.);
#45054=ORIENTED_EDGE('',*,*,#33823,.F.);
#45055=ORIENTED_EDGE('',*,*,#33826,.F.);
#45056=ORIENTED_EDGE('',*,*,#33827,.T.);
#45057=ORIENTED_EDGE('',*,*,#33828,.T.);
#45058=ORIENTED_EDGE('',*,*,#33829,.F.);
#45059=ORIENTED_EDGE('',*,*,#33830,.F.);
#45060=ORIENTED_EDGE('',*,*,#33831,.T.);
#45061=ORIENTED_EDGE('',*,*,#33832,.T.);
#45062=ORIENTED_EDGE('',*,*,#33827,.F.);
#45063=ORIENTED_EDGE('',*,*,#33833,.F.);
#45064=ORIENTED_EDGE('',*,*,#33834,.T.);
#45065=ORIENTED_EDGE('',*,*,#33835,.T.);
#45066=ORIENTED_EDGE('',*,*,#33831,.F.);
#45067=ORIENTED_EDGE('',*,*,#33836,.F.);
#45068=ORIENTED_EDGE('',*,*,#33829,.T.);
#45069=ORIENTED_EDGE('',*,*,#33837,.T.);
#45070=ORIENTED_EDGE('',*,*,#33834,.F.);
#45071=ORIENTED_EDGE('',*,*,#33837,.F.);
#45072=ORIENTED_EDGE('',*,*,#33828,.F.);
#45073=ORIENTED_EDGE('',*,*,#33832,.F.);
#45074=ORIENTED_EDGE('',*,*,#33835,.F.);
#45075=ORIENTED_EDGE('',*,*,#33838,.F.);
#45076=ORIENTED_EDGE('',*,*,#33839,.T.);
#45077=ORIENTED_EDGE('',*,*,#33840,.T.);
#45078=ORIENTED_EDGE('',*,*,#33841,.F.);
#45079=ORIENTED_EDGE('',*,*,#33842,.F.);
#45080=ORIENTED_EDGE('',*,*,#33843,.T.);
#45081=ORIENTED_EDGE('',*,*,#33844,.T.);
#45082=ORIENTED_EDGE('',*,*,#33839,.F.);
#45083=ORIENTED_EDGE('',*,*,#33845,.F.);
#45084=ORIENTED_EDGE('',*,*,#33846,.T.);
#45085=ORIENTED_EDGE('',*,*,#33847,.T.);
#45086=ORIENTED_EDGE('',*,*,#33843,.F.);
#45087=ORIENTED_EDGE('',*,*,#33848,.F.);
#45088=ORIENTED_EDGE('',*,*,#33841,.T.);
#45089=ORIENTED_EDGE('',*,*,#33849,.T.);
#45090=ORIENTED_EDGE('',*,*,#33846,.F.);
#45091=ORIENTED_EDGE('',*,*,#33849,.F.);
#45092=ORIENTED_EDGE('',*,*,#33840,.F.);
#45093=ORIENTED_EDGE('',*,*,#33844,.F.);
#45094=ORIENTED_EDGE('',*,*,#33847,.F.);
#45095=ORIENTED_EDGE('',*,*,#33850,.F.);
#45096=ORIENTED_EDGE('',*,*,#33851,.T.);
#45097=ORIENTED_EDGE('',*,*,#33852,.T.);
#45098=ORIENTED_EDGE('',*,*,#33853,.F.);
#45099=ORIENTED_EDGE('',*,*,#33854,.F.);
#45100=ORIENTED_EDGE('',*,*,#33855,.T.);
#45101=ORIENTED_EDGE('',*,*,#33856,.T.);
#45102=ORIENTED_EDGE('',*,*,#33851,.F.);
#45103=ORIENTED_EDGE('',*,*,#33857,.F.);
#45104=ORIENTED_EDGE('',*,*,#33858,.T.);
#45105=ORIENTED_EDGE('',*,*,#33859,.T.);
#45106=ORIENTED_EDGE('',*,*,#33855,.F.);
#45107=ORIENTED_EDGE('',*,*,#33860,.F.);
#45108=ORIENTED_EDGE('',*,*,#33853,.T.);
#45109=ORIENTED_EDGE('',*,*,#33861,.T.);
#45110=ORIENTED_EDGE('',*,*,#33858,.F.);
#45111=ORIENTED_EDGE('',*,*,#33861,.F.);
#45112=ORIENTED_EDGE('',*,*,#33852,.F.);
#45113=ORIENTED_EDGE('',*,*,#33856,.F.);
#45114=ORIENTED_EDGE('',*,*,#33859,.F.);
#45115=ORIENTED_EDGE('',*,*,#33862,.F.);
#45116=ORIENTED_EDGE('',*,*,#33863,.T.);
#45117=ORIENTED_EDGE('',*,*,#33864,.T.);
#45118=ORIENTED_EDGE('',*,*,#33865,.F.);
#45119=ORIENTED_EDGE('',*,*,#33866,.F.);
#45120=ORIENTED_EDGE('',*,*,#33867,.T.);
#45121=ORIENTED_EDGE('',*,*,#33868,.T.);
#45122=ORIENTED_EDGE('',*,*,#33863,.F.);
#45123=ORIENTED_EDGE('',*,*,#33869,.F.);
#45124=ORIENTED_EDGE('',*,*,#33870,.T.);
#45125=ORIENTED_EDGE('',*,*,#33871,.T.);
#45126=ORIENTED_EDGE('',*,*,#33867,.F.);
#45127=ORIENTED_EDGE('',*,*,#33872,.F.);
#45128=ORIENTED_EDGE('',*,*,#33865,.T.);
#45129=ORIENTED_EDGE('',*,*,#33873,.T.);
#45130=ORIENTED_EDGE('',*,*,#33870,.F.);
#45131=ORIENTED_EDGE('',*,*,#33873,.F.);
#45132=ORIENTED_EDGE('',*,*,#33864,.F.);
#45133=ORIENTED_EDGE('',*,*,#33868,.F.);
#45134=ORIENTED_EDGE('',*,*,#33871,.F.);
#45135=ORIENTED_EDGE('',*,*,#33874,.F.);
#45136=ORIENTED_EDGE('',*,*,#33875,.T.);
#45137=ORIENTED_EDGE('',*,*,#33876,.T.);
#45138=ORIENTED_EDGE('',*,*,#33877,.F.);
#45139=ORIENTED_EDGE('',*,*,#33878,.F.);
#45140=ORIENTED_EDGE('',*,*,#33879,.T.);
#45141=ORIENTED_EDGE('',*,*,#33880,.T.);
#45142=ORIENTED_EDGE('',*,*,#33875,.F.);
#45143=ORIENTED_EDGE('',*,*,#33881,.F.);
#45144=ORIENTED_EDGE('',*,*,#33882,.T.);
#45145=ORIENTED_EDGE('',*,*,#33883,.T.);
#45146=ORIENTED_EDGE('',*,*,#33879,.F.);
#45147=ORIENTED_EDGE('',*,*,#33884,.F.);
#45148=ORIENTED_EDGE('',*,*,#33877,.T.);
#45149=ORIENTED_EDGE('',*,*,#33885,.T.);
#45150=ORIENTED_EDGE('',*,*,#33882,.F.);
#45151=ORIENTED_EDGE('',*,*,#33885,.F.);
#45152=ORIENTED_EDGE('',*,*,#33876,.F.);
#45153=ORIENTED_EDGE('',*,*,#33880,.F.);
#45154=ORIENTED_EDGE('',*,*,#33883,.F.);
#45155=ORIENTED_EDGE('',*,*,#33886,.F.);
#45156=ORIENTED_EDGE('',*,*,#33887,.T.);
#45157=ORIENTED_EDGE('',*,*,#33888,.T.);
#45158=ORIENTED_EDGE('',*,*,#33889,.F.);
#45159=ORIENTED_EDGE('',*,*,#33890,.F.);
#45160=ORIENTED_EDGE('',*,*,#33891,.T.);
#45161=ORIENTED_EDGE('',*,*,#33892,.T.);
#45162=ORIENTED_EDGE('',*,*,#33887,.F.);
#45163=ORIENTED_EDGE('',*,*,#33893,.F.);
#45164=ORIENTED_EDGE('',*,*,#33894,.T.);
#45165=ORIENTED_EDGE('',*,*,#33895,.T.);
#45166=ORIENTED_EDGE('',*,*,#33891,.F.);
#45167=ORIENTED_EDGE('',*,*,#33896,.F.);
#45168=ORIENTED_EDGE('',*,*,#33889,.T.);
#45169=ORIENTED_EDGE('',*,*,#33897,.T.);
#45170=ORIENTED_EDGE('',*,*,#33894,.F.);
#45171=ORIENTED_EDGE('',*,*,#33897,.F.);
#45172=ORIENTED_EDGE('',*,*,#33888,.F.);
#45173=ORIENTED_EDGE('',*,*,#33892,.F.);
#45174=ORIENTED_EDGE('',*,*,#33895,.F.);
#45175=ORIENTED_EDGE('',*,*,#33898,.F.);
#45176=ORIENTED_EDGE('',*,*,#33899,.T.);
#45177=ORIENTED_EDGE('',*,*,#33900,.T.);
#45178=ORIENTED_EDGE('',*,*,#33901,.F.);
#45179=ORIENTED_EDGE('',*,*,#33902,.F.);
#45180=ORIENTED_EDGE('',*,*,#33903,.T.);
#45181=ORIENTED_EDGE('',*,*,#33904,.T.);
#45182=ORIENTED_EDGE('',*,*,#33899,.F.);
#45183=ORIENTED_EDGE('',*,*,#33905,.F.);
#45184=ORIENTED_EDGE('',*,*,#33906,.T.);
#45185=ORIENTED_EDGE('',*,*,#33907,.T.);
#45186=ORIENTED_EDGE('',*,*,#33903,.F.);
#45187=ORIENTED_EDGE('',*,*,#33908,.F.);
#45188=ORIENTED_EDGE('',*,*,#33901,.T.);
#45189=ORIENTED_EDGE('',*,*,#33909,.T.);
#45190=ORIENTED_EDGE('',*,*,#33906,.F.);
#45191=ORIENTED_EDGE('',*,*,#33909,.F.);
#45192=ORIENTED_EDGE('',*,*,#33900,.F.);
#45193=ORIENTED_EDGE('',*,*,#33904,.F.);
#45194=ORIENTED_EDGE('',*,*,#33907,.F.);
#45195=ORIENTED_EDGE('',*,*,#33910,.F.);
#45196=ORIENTED_EDGE('',*,*,#33911,.T.);
#45197=ORIENTED_EDGE('',*,*,#33912,.T.);
#45198=ORIENTED_EDGE('',*,*,#33913,.F.);
#45199=ORIENTED_EDGE('',*,*,#33914,.F.);
#45200=ORIENTED_EDGE('',*,*,#33915,.T.);
#45201=ORIENTED_EDGE('',*,*,#33916,.T.);
#45202=ORIENTED_EDGE('',*,*,#33911,.F.);
#45203=ORIENTED_EDGE('',*,*,#33917,.F.);
#45204=ORIENTED_EDGE('',*,*,#33918,.T.);
#45205=ORIENTED_EDGE('',*,*,#33919,.T.);
#45206=ORIENTED_EDGE('',*,*,#33915,.F.);
#45207=ORIENTED_EDGE('',*,*,#33920,.F.);
#45208=ORIENTED_EDGE('',*,*,#33913,.T.);
#45209=ORIENTED_EDGE('',*,*,#33921,.T.);
#45210=ORIENTED_EDGE('',*,*,#33918,.F.);
#45211=ORIENTED_EDGE('',*,*,#33921,.F.);
#45212=ORIENTED_EDGE('',*,*,#33912,.F.);
#45213=ORIENTED_EDGE('',*,*,#33916,.F.);
#45214=ORIENTED_EDGE('',*,*,#33919,.F.);
#45215=ORIENTED_EDGE('',*,*,#33922,.F.);
#45216=ORIENTED_EDGE('',*,*,#33923,.T.);
#45217=ORIENTED_EDGE('',*,*,#33924,.T.);
#45218=ORIENTED_EDGE('',*,*,#33925,.F.);
#45219=ORIENTED_EDGE('',*,*,#33926,.F.);
#45220=ORIENTED_EDGE('',*,*,#33927,.T.);
#45221=ORIENTED_EDGE('',*,*,#33928,.T.);
#45222=ORIENTED_EDGE('',*,*,#33923,.F.);
#45223=ORIENTED_EDGE('',*,*,#33929,.F.);
#45224=ORIENTED_EDGE('',*,*,#33930,.T.);
#45225=ORIENTED_EDGE('',*,*,#33931,.T.);
#45226=ORIENTED_EDGE('',*,*,#33927,.F.);
#45227=ORIENTED_EDGE('',*,*,#33932,.F.);
#45228=ORIENTED_EDGE('',*,*,#33925,.T.);
#45229=ORIENTED_EDGE('',*,*,#33933,.T.);
#45230=ORIENTED_EDGE('',*,*,#33930,.F.);
#45231=ORIENTED_EDGE('',*,*,#33933,.F.);
#45232=ORIENTED_EDGE('',*,*,#33924,.F.);
#45233=ORIENTED_EDGE('',*,*,#33928,.F.);
#45234=ORIENTED_EDGE('',*,*,#33931,.F.);
#45235=ORIENTED_EDGE('',*,*,#33934,.F.);
#45236=ORIENTED_EDGE('',*,*,#33935,.T.);
#45237=ORIENTED_EDGE('',*,*,#33936,.T.);
#45238=ORIENTED_EDGE('',*,*,#33937,.F.);
#45239=ORIENTED_EDGE('',*,*,#33938,.F.);
#45240=ORIENTED_EDGE('',*,*,#33939,.T.);
#45241=ORIENTED_EDGE('',*,*,#33940,.T.);
#45242=ORIENTED_EDGE('',*,*,#33935,.F.);
#45243=ORIENTED_EDGE('',*,*,#33941,.F.);
#45244=ORIENTED_EDGE('',*,*,#33942,.T.);
#45245=ORIENTED_EDGE('',*,*,#33943,.T.);
#45246=ORIENTED_EDGE('',*,*,#33939,.F.);
#45247=ORIENTED_EDGE('',*,*,#33944,.F.);
#45248=ORIENTED_EDGE('',*,*,#33937,.T.);
#45249=ORIENTED_EDGE('',*,*,#33945,.T.);
#45250=ORIENTED_EDGE('',*,*,#33942,.F.);
#45251=ORIENTED_EDGE('',*,*,#33945,.F.);
#45252=ORIENTED_EDGE('',*,*,#33936,.F.);
#45253=ORIENTED_EDGE('',*,*,#33940,.F.);
#45254=ORIENTED_EDGE('',*,*,#33943,.F.);
#45255=ORIENTED_EDGE('',*,*,#33946,.F.);
#45256=ORIENTED_EDGE('',*,*,#33947,.T.);
#45257=ORIENTED_EDGE('',*,*,#33948,.T.);
#45258=ORIENTED_EDGE('',*,*,#33949,.F.);
#45259=ORIENTED_EDGE('',*,*,#33950,.F.);
#45260=ORIENTED_EDGE('',*,*,#33951,.T.);
#45261=ORIENTED_EDGE('',*,*,#33952,.T.);
#45262=ORIENTED_EDGE('',*,*,#33947,.F.);
#45263=ORIENTED_EDGE('',*,*,#33953,.F.);
#45264=ORIENTED_EDGE('',*,*,#33954,.T.);
#45265=ORIENTED_EDGE('',*,*,#33955,.T.);
#45266=ORIENTED_EDGE('',*,*,#33951,.F.);
#45267=ORIENTED_EDGE('',*,*,#33956,.F.);
#45268=ORIENTED_EDGE('',*,*,#33949,.T.);
#45269=ORIENTED_EDGE('',*,*,#33957,.T.);
#45270=ORIENTED_EDGE('',*,*,#33954,.F.);
#45271=ORIENTED_EDGE('',*,*,#33957,.F.);
#45272=ORIENTED_EDGE('',*,*,#33948,.F.);
#45273=ORIENTED_EDGE('',*,*,#33952,.F.);
#45274=ORIENTED_EDGE('',*,*,#33955,.F.);
#45275=ORIENTED_EDGE('',*,*,#33958,.F.);
#45276=ORIENTED_EDGE('',*,*,#33959,.T.);
#45277=ORIENTED_EDGE('',*,*,#33960,.T.);
#45278=ORIENTED_EDGE('',*,*,#33961,.F.);
#45279=ORIENTED_EDGE('',*,*,#33962,.F.);
#45280=ORIENTED_EDGE('',*,*,#33963,.T.);
#45281=ORIENTED_EDGE('',*,*,#33964,.T.);
#45282=ORIENTED_EDGE('',*,*,#33959,.F.);
#45283=ORIENTED_EDGE('',*,*,#33965,.F.);
#45284=ORIENTED_EDGE('',*,*,#33966,.T.);
#45285=ORIENTED_EDGE('',*,*,#33967,.T.);
#45286=ORIENTED_EDGE('',*,*,#33963,.F.);
#45287=ORIENTED_EDGE('',*,*,#33968,.F.);
#45288=ORIENTED_EDGE('',*,*,#33961,.T.);
#45289=ORIENTED_EDGE('',*,*,#33969,.T.);
#45290=ORIENTED_EDGE('',*,*,#33966,.F.);
#45291=ORIENTED_EDGE('',*,*,#33969,.F.);
#45292=ORIENTED_EDGE('',*,*,#33960,.F.);
#45293=ORIENTED_EDGE('',*,*,#33964,.F.);
#45294=ORIENTED_EDGE('',*,*,#33967,.F.);
#45295=ORIENTED_EDGE('',*,*,#33970,.F.);
#45296=ORIENTED_EDGE('',*,*,#33971,.T.);
#45297=ORIENTED_EDGE('',*,*,#33972,.T.);
#45298=ORIENTED_EDGE('',*,*,#33973,.F.);
#45299=ORIENTED_EDGE('',*,*,#33974,.F.);
#45300=ORIENTED_EDGE('',*,*,#33975,.T.);
#45301=ORIENTED_EDGE('',*,*,#33976,.T.);
#45302=ORIENTED_EDGE('',*,*,#33971,.F.);
#45303=ORIENTED_EDGE('',*,*,#33977,.F.);
#45304=ORIENTED_EDGE('',*,*,#33978,.T.);
#45305=ORIENTED_EDGE('',*,*,#33979,.T.);
#45306=ORIENTED_EDGE('',*,*,#33975,.F.);
#45307=ORIENTED_EDGE('',*,*,#33980,.F.);
#45308=ORIENTED_EDGE('',*,*,#33973,.T.);
#45309=ORIENTED_EDGE('',*,*,#33981,.T.);
#45310=ORIENTED_EDGE('',*,*,#33978,.F.);
#45311=ORIENTED_EDGE('',*,*,#33981,.F.);
#45312=ORIENTED_EDGE('',*,*,#33972,.F.);
#45313=ORIENTED_EDGE('',*,*,#33976,.F.);
#45314=ORIENTED_EDGE('',*,*,#33979,.F.);
#45315=ORIENTED_EDGE('',*,*,#33982,.F.);
#45316=ORIENTED_EDGE('',*,*,#33983,.T.);
#45317=ORIENTED_EDGE('',*,*,#33984,.T.);
#45318=ORIENTED_EDGE('',*,*,#33985,.F.);
#45319=ORIENTED_EDGE('',*,*,#33986,.F.);
#45320=ORIENTED_EDGE('',*,*,#33987,.T.);
#45321=ORIENTED_EDGE('',*,*,#33988,.T.);
#45322=ORIENTED_EDGE('',*,*,#33983,.F.);
#45323=ORIENTED_EDGE('',*,*,#33989,.F.);
#45324=ORIENTED_EDGE('',*,*,#33990,.T.);
#45325=ORIENTED_EDGE('',*,*,#33991,.T.);
#45326=ORIENTED_EDGE('',*,*,#33987,.F.);
#45327=ORIENTED_EDGE('',*,*,#33992,.F.);
#45328=ORIENTED_EDGE('',*,*,#33985,.T.);
#45329=ORIENTED_EDGE('',*,*,#33993,.T.);
#45330=ORIENTED_EDGE('',*,*,#33990,.F.);
#45331=ORIENTED_EDGE('',*,*,#33993,.F.);
#45332=ORIENTED_EDGE('',*,*,#33984,.F.);
#45333=ORIENTED_EDGE('',*,*,#33988,.F.);
#45334=ORIENTED_EDGE('',*,*,#33991,.F.);
#45335=ORIENTED_EDGE('',*,*,#33994,.F.);
#45336=ORIENTED_EDGE('',*,*,#33995,.T.);
#45337=ORIENTED_EDGE('',*,*,#33996,.T.);
#45338=ORIENTED_EDGE('',*,*,#33997,.F.);
#45339=ORIENTED_EDGE('',*,*,#33998,.F.);
#45340=ORIENTED_EDGE('',*,*,#33999,.T.);
#45341=ORIENTED_EDGE('',*,*,#34000,.T.);
#45342=ORIENTED_EDGE('',*,*,#33995,.F.);
#45343=ORIENTED_EDGE('',*,*,#34001,.F.);
#45344=ORIENTED_EDGE('',*,*,#34002,.T.);
#45345=ORIENTED_EDGE('',*,*,#34003,.T.);
#45346=ORIENTED_EDGE('',*,*,#33999,.F.);
#45347=ORIENTED_EDGE('',*,*,#34004,.F.);
#45348=ORIENTED_EDGE('',*,*,#33997,.T.);
#45349=ORIENTED_EDGE('',*,*,#34005,.T.);
#45350=ORIENTED_EDGE('',*,*,#34002,.F.);
#45351=ORIENTED_EDGE('',*,*,#34005,.F.);
#45352=ORIENTED_EDGE('',*,*,#33996,.F.);
#45353=ORIENTED_EDGE('',*,*,#34000,.F.);
#45354=ORIENTED_EDGE('',*,*,#34003,.F.);
#45355=ORIENTED_EDGE('',*,*,#34006,.F.);
#45356=ORIENTED_EDGE('',*,*,#34007,.T.);
#45357=ORIENTED_EDGE('',*,*,#34008,.T.);
#45358=ORIENTED_EDGE('',*,*,#34009,.F.);
#45359=ORIENTED_EDGE('',*,*,#34010,.F.);
#45360=ORIENTED_EDGE('',*,*,#34011,.T.);
#45361=ORIENTED_EDGE('',*,*,#34012,.T.);
#45362=ORIENTED_EDGE('',*,*,#34007,.F.);
#45363=ORIENTED_EDGE('',*,*,#34013,.F.);
#45364=ORIENTED_EDGE('',*,*,#34014,.T.);
#45365=ORIENTED_EDGE('',*,*,#34015,.T.);
#45366=ORIENTED_EDGE('',*,*,#34011,.F.);
#45367=ORIENTED_EDGE('',*,*,#34016,.F.);
#45368=ORIENTED_EDGE('',*,*,#34009,.T.);
#45369=ORIENTED_EDGE('',*,*,#34017,.T.);
#45370=ORIENTED_EDGE('',*,*,#34014,.F.);
#45371=ORIENTED_EDGE('',*,*,#34017,.F.);
#45372=ORIENTED_EDGE('',*,*,#34008,.F.);
#45373=ORIENTED_EDGE('',*,*,#34012,.F.);
#45374=ORIENTED_EDGE('',*,*,#34015,.F.);
#45375=ORIENTED_EDGE('',*,*,#34018,.F.);
#45376=ORIENTED_EDGE('',*,*,#34019,.T.);
#45377=ORIENTED_EDGE('',*,*,#34020,.T.);
#45378=ORIENTED_EDGE('',*,*,#34021,.F.);
#45379=ORIENTED_EDGE('',*,*,#34022,.F.);
#45380=ORIENTED_EDGE('',*,*,#34023,.T.);
#45381=ORIENTED_EDGE('',*,*,#34024,.T.);
#45382=ORIENTED_EDGE('',*,*,#34019,.F.);
#45383=ORIENTED_EDGE('',*,*,#34025,.F.);
#45384=ORIENTED_EDGE('',*,*,#34026,.T.);
#45385=ORIENTED_EDGE('',*,*,#34027,.T.);
#45386=ORIENTED_EDGE('',*,*,#34023,.F.);
#45387=ORIENTED_EDGE('',*,*,#34028,.F.);
#45388=ORIENTED_EDGE('',*,*,#34021,.T.);
#45389=ORIENTED_EDGE('',*,*,#34029,.T.);
#45390=ORIENTED_EDGE('',*,*,#34026,.F.);
#45391=ORIENTED_EDGE('',*,*,#34029,.F.);
#45392=ORIENTED_EDGE('',*,*,#34020,.F.);
#45393=ORIENTED_EDGE('',*,*,#34024,.F.);
#45394=ORIENTED_EDGE('',*,*,#34027,.F.);
#45395=ORIENTED_EDGE('',*,*,#34030,.F.);
#45396=ORIENTED_EDGE('',*,*,#34031,.T.);
#45397=ORIENTED_EDGE('',*,*,#34032,.T.);
#45398=ORIENTED_EDGE('',*,*,#34033,.F.);
#45399=ORIENTED_EDGE('',*,*,#34034,.F.);
#45400=ORIENTED_EDGE('',*,*,#34035,.T.);
#45401=ORIENTED_EDGE('',*,*,#34036,.T.);
#45402=ORIENTED_EDGE('',*,*,#34031,.F.);
#45403=ORIENTED_EDGE('',*,*,#34037,.F.);
#45404=ORIENTED_EDGE('',*,*,#34038,.T.);
#45405=ORIENTED_EDGE('',*,*,#34039,.T.);
#45406=ORIENTED_EDGE('',*,*,#34035,.F.);
#45407=ORIENTED_EDGE('',*,*,#34040,.F.);
#45408=ORIENTED_EDGE('',*,*,#34033,.T.);
#45409=ORIENTED_EDGE('',*,*,#34041,.T.);
#45410=ORIENTED_EDGE('',*,*,#34038,.F.);
#45411=ORIENTED_EDGE('',*,*,#34041,.F.);
#45412=ORIENTED_EDGE('',*,*,#34032,.F.);
#45413=ORIENTED_EDGE('',*,*,#34036,.F.);
#45414=ORIENTED_EDGE('',*,*,#34039,.F.);
#45415=ORIENTED_EDGE('',*,*,#34042,.F.);
#45416=ORIENTED_EDGE('',*,*,#34043,.T.);
#45417=ORIENTED_EDGE('',*,*,#34044,.T.);
#45418=ORIENTED_EDGE('',*,*,#34045,.F.);
#45419=ORIENTED_EDGE('',*,*,#34046,.F.);
#45420=ORIENTED_EDGE('',*,*,#34047,.T.);
#45421=ORIENTED_EDGE('',*,*,#34048,.T.);
#45422=ORIENTED_EDGE('',*,*,#34043,.F.);
#45423=ORIENTED_EDGE('',*,*,#34049,.F.);
#45424=ORIENTED_EDGE('',*,*,#34050,.T.);
#45425=ORIENTED_EDGE('',*,*,#34051,.T.);
#45426=ORIENTED_EDGE('',*,*,#34047,.F.);
#45427=ORIENTED_EDGE('',*,*,#34052,.F.);
#45428=ORIENTED_EDGE('',*,*,#34045,.T.);
#45429=ORIENTED_EDGE('',*,*,#34053,.T.);
#45430=ORIENTED_EDGE('',*,*,#34050,.F.);
#45431=ORIENTED_EDGE('',*,*,#34053,.F.);
#45432=ORIENTED_EDGE('',*,*,#34044,.F.);
#45433=ORIENTED_EDGE('',*,*,#34048,.F.);
#45434=ORIENTED_EDGE('',*,*,#34051,.F.);
#45435=ORIENTED_EDGE('',*,*,#34054,.F.);
#45436=ORIENTED_EDGE('',*,*,#34055,.T.);
#45437=ORIENTED_EDGE('',*,*,#34056,.T.);
#45438=ORIENTED_EDGE('',*,*,#34057,.F.);
#45439=ORIENTED_EDGE('',*,*,#34058,.F.);
#45440=ORIENTED_EDGE('',*,*,#34059,.T.);
#45441=ORIENTED_EDGE('',*,*,#34060,.T.);
#45442=ORIENTED_EDGE('',*,*,#34055,.F.);
#45443=ORIENTED_EDGE('',*,*,#34061,.F.);
#45444=ORIENTED_EDGE('',*,*,#34062,.T.);
#45445=ORIENTED_EDGE('',*,*,#34063,.T.);
#45446=ORIENTED_EDGE('',*,*,#34059,.F.);
#45447=ORIENTED_EDGE('',*,*,#34064,.F.);
#45448=ORIENTED_EDGE('',*,*,#34057,.T.);
#45449=ORIENTED_EDGE('',*,*,#34065,.T.);
#45450=ORIENTED_EDGE('',*,*,#34062,.F.);
#45451=ORIENTED_EDGE('',*,*,#34065,.F.);
#45452=ORIENTED_EDGE('',*,*,#34056,.F.);
#45453=ORIENTED_EDGE('',*,*,#34060,.F.);
#45454=ORIENTED_EDGE('',*,*,#34063,.F.);
#45455=ORIENTED_EDGE('',*,*,#34066,.F.);
#45456=ORIENTED_EDGE('',*,*,#34067,.T.);
#45457=ORIENTED_EDGE('',*,*,#34068,.T.);
#45458=ORIENTED_EDGE('',*,*,#34069,.F.);
#45459=ORIENTED_EDGE('',*,*,#34070,.F.);
#45460=ORIENTED_EDGE('',*,*,#34071,.T.);
#45461=ORIENTED_EDGE('',*,*,#34072,.T.);
#45462=ORIENTED_EDGE('',*,*,#34067,.F.);
#45463=ORIENTED_EDGE('',*,*,#34073,.F.);
#45464=ORIENTED_EDGE('',*,*,#34074,.T.);
#45465=ORIENTED_EDGE('',*,*,#34075,.T.);
#45466=ORIENTED_EDGE('',*,*,#34071,.F.);
#45467=ORIENTED_EDGE('',*,*,#34076,.F.);
#45468=ORIENTED_EDGE('',*,*,#34069,.T.);
#45469=ORIENTED_EDGE('',*,*,#34077,.T.);
#45470=ORIENTED_EDGE('',*,*,#34074,.F.);
#45471=ORIENTED_EDGE('',*,*,#34077,.F.);
#45472=ORIENTED_EDGE('',*,*,#34068,.F.);
#45473=ORIENTED_EDGE('',*,*,#34072,.F.);
#45474=ORIENTED_EDGE('',*,*,#34075,.F.);
#45475=ORIENTED_EDGE('',*,*,#34078,.F.);
#45476=ORIENTED_EDGE('',*,*,#34079,.T.);
#45477=ORIENTED_EDGE('',*,*,#34080,.T.);
#45478=ORIENTED_EDGE('',*,*,#34081,.F.);
#45479=ORIENTED_EDGE('',*,*,#34082,.F.);
#45480=ORIENTED_EDGE('',*,*,#34083,.T.);
#45481=ORIENTED_EDGE('',*,*,#34084,.T.);
#45482=ORIENTED_EDGE('',*,*,#34079,.F.);
#45483=ORIENTED_EDGE('',*,*,#34085,.F.);
#45484=ORIENTED_EDGE('',*,*,#34086,.T.);
#45485=ORIENTED_EDGE('',*,*,#34087,.T.);
#45486=ORIENTED_EDGE('',*,*,#34083,.F.);
#45487=ORIENTED_EDGE('',*,*,#34088,.F.);
#45488=ORIENTED_EDGE('',*,*,#34081,.T.);
#45489=ORIENTED_EDGE('',*,*,#34089,.T.);
#45490=ORIENTED_EDGE('',*,*,#34086,.F.);
#45491=ORIENTED_EDGE('',*,*,#34089,.F.);
#45492=ORIENTED_EDGE('',*,*,#34080,.F.);
#45493=ORIENTED_EDGE('',*,*,#34084,.F.);
#45494=ORIENTED_EDGE('',*,*,#34087,.F.);
#45495=ORIENTED_EDGE('',*,*,#34090,.F.);
#45496=ORIENTED_EDGE('',*,*,#34091,.T.);
#45497=ORIENTED_EDGE('',*,*,#34092,.T.);
#45498=ORIENTED_EDGE('',*,*,#34093,.F.);
#45499=ORIENTED_EDGE('',*,*,#34094,.F.);
#45500=ORIENTED_EDGE('',*,*,#34095,.T.);
#45501=ORIENTED_EDGE('',*,*,#34096,.T.);
#45502=ORIENTED_EDGE('',*,*,#34091,.F.);
#45503=ORIENTED_EDGE('',*,*,#34097,.F.);
#45504=ORIENTED_EDGE('',*,*,#34098,.T.);
#45505=ORIENTED_EDGE('',*,*,#34099,.T.);
#45506=ORIENTED_EDGE('',*,*,#34095,.F.);
#45507=ORIENTED_EDGE('',*,*,#34100,.F.);
#45508=ORIENTED_EDGE('',*,*,#34093,.T.);
#45509=ORIENTED_EDGE('',*,*,#34101,.T.);
#45510=ORIENTED_EDGE('',*,*,#34098,.F.);
#45511=ORIENTED_EDGE('',*,*,#34101,.F.);
#45512=ORIENTED_EDGE('',*,*,#34092,.F.);
#45513=ORIENTED_EDGE('',*,*,#34096,.F.);
#45514=ORIENTED_EDGE('',*,*,#34099,.F.);
#45515=ORIENTED_EDGE('',*,*,#34102,.F.);
#45516=ORIENTED_EDGE('',*,*,#34103,.T.);
#45517=ORIENTED_EDGE('',*,*,#34104,.T.);
#45518=ORIENTED_EDGE('',*,*,#34105,.F.);
#45519=ORIENTED_EDGE('',*,*,#34106,.F.);
#45520=ORIENTED_EDGE('',*,*,#34107,.T.);
#45521=ORIENTED_EDGE('',*,*,#34108,.T.);
#45522=ORIENTED_EDGE('',*,*,#34103,.F.);
#45523=ORIENTED_EDGE('',*,*,#34109,.F.);
#45524=ORIENTED_EDGE('',*,*,#34110,.T.);
#45525=ORIENTED_EDGE('',*,*,#34111,.T.);
#45526=ORIENTED_EDGE('',*,*,#34107,.F.);
#45527=ORIENTED_EDGE('',*,*,#34112,.F.);
#45528=ORIENTED_EDGE('',*,*,#34105,.T.);
#45529=ORIENTED_EDGE('',*,*,#34113,.T.);
#45530=ORIENTED_EDGE('',*,*,#34110,.F.);
#45531=ORIENTED_EDGE('',*,*,#34113,.F.);
#45532=ORIENTED_EDGE('',*,*,#34104,.F.);
#45533=ORIENTED_EDGE('',*,*,#34108,.F.);
#45534=ORIENTED_EDGE('',*,*,#34111,.F.);
#45535=ORIENTED_EDGE('',*,*,#34114,.F.);
#45536=ORIENTED_EDGE('',*,*,#34115,.T.);
#45537=ORIENTED_EDGE('',*,*,#34116,.T.);
#45538=ORIENTED_EDGE('',*,*,#34117,.F.);
#45539=ORIENTED_EDGE('',*,*,#34118,.F.);
#45540=ORIENTED_EDGE('',*,*,#34119,.T.);
#45541=ORIENTED_EDGE('',*,*,#34120,.T.);
#45542=ORIENTED_EDGE('',*,*,#34115,.F.);
#45543=ORIENTED_EDGE('',*,*,#34121,.F.);
#45544=ORIENTED_EDGE('',*,*,#34122,.T.);
#45545=ORIENTED_EDGE('',*,*,#34123,.T.);
#45546=ORIENTED_EDGE('',*,*,#34119,.F.);
#45547=ORIENTED_EDGE('',*,*,#34124,.F.);
#45548=ORIENTED_EDGE('',*,*,#34117,.T.);
#45549=ORIENTED_EDGE('',*,*,#34125,.T.);
#45550=ORIENTED_EDGE('',*,*,#34122,.F.);
#45551=ORIENTED_EDGE('',*,*,#34125,.F.);
#45552=ORIENTED_EDGE('',*,*,#34116,.F.);
#45553=ORIENTED_EDGE('',*,*,#34120,.F.);
#45554=ORIENTED_EDGE('',*,*,#34123,.F.);
#45555=ORIENTED_EDGE('',*,*,#34126,.F.);
#45556=ORIENTED_EDGE('',*,*,#34127,.T.);
#45557=ORIENTED_EDGE('',*,*,#34128,.T.);
#45558=ORIENTED_EDGE('',*,*,#34129,.F.);
#45559=ORIENTED_EDGE('',*,*,#34130,.F.);
#45560=ORIENTED_EDGE('',*,*,#34131,.T.);
#45561=ORIENTED_EDGE('',*,*,#34132,.T.);
#45562=ORIENTED_EDGE('',*,*,#34127,.F.);
#45563=ORIENTED_EDGE('',*,*,#34133,.F.);
#45564=ORIENTED_EDGE('',*,*,#34134,.T.);
#45565=ORIENTED_EDGE('',*,*,#34135,.T.);
#45566=ORIENTED_EDGE('',*,*,#34131,.F.);
#45567=ORIENTED_EDGE('',*,*,#34136,.F.);
#45568=ORIENTED_EDGE('',*,*,#34129,.T.);
#45569=ORIENTED_EDGE('',*,*,#34137,.T.);
#45570=ORIENTED_EDGE('',*,*,#34134,.F.);
#45571=ORIENTED_EDGE('',*,*,#34137,.F.);
#45572=ORIENTED_EDGE('',*,*,#34128,.F.);
#45573=ORIENTED_EDGE('',*,*,#34132,.F.);
#45574=ORIENTED_EDGE('',*,*,#34135,.F.);
#45575=ORIENTED_EDGE('',*,*,#34138,.F.);
#45576=ORIENTED_EDGE('',*,*,#34139,.T.);
#45577=ORIENTED_EDGE('',*,*,#34140,.T.);
#45578=ORIENTED_EDGE('',*,*,#34141,.F.);
#45579=ORIENTED_EDGE('',*,*,#34142,.F.);
#45580=ORIENTED_EDGE('',*,*,#34143,.T.);
#45581=ORIENTED_EDGE('',*,*,#34144,.T.);
#45582=ORIENTED_EDGE('',*,*,#34139,.F.);
#45583=ORIENTED_EDGE('',*,*,#34145,.F.);
#45584=ORIENTED_EDGE('',*,*,#34146,.T.);
#45585=ORIENTED_EDGE('',*,*,#34147,.T.);
#45586=ORIENTED_EDGE('',*,*,#34143,.F.);
#45587=ORIENTED_EDGE('',*,*,#34148,.F.);
#45588=ORIENTED_EDGE('',*,*,#34141,.T.);
#45589=ORIENTED_EDGE('',*,*,#34149,.T.);
#45590=ORIENTED_EDGE('',*,*,#34146,.F.);
#45591=ORIENTED_EDGE('',*,*,#34149,.F.);
#45592=ORIENTED_EDGE('',*,*,#34140,.F.);
#45593=ORIENTED_EDGE('',*,*,#34144,.F.);
#45594=ORIENTED_EDGE('',*,*,#34147,.F.);
#45595=ORIENTED_EDGE('',*,*,#34150,.F.);
#45596=ORIENTED_EDGE('',*,*,#34151,.T.);
#45597=ORIENTED_EDGE('',*,*,#34152,.T.);
#45598=ORIENTED_EDGE('',*,*,#34153,.F.);
#45599=ORIENTED_EDGE('',*,*,#34154,.F.);
#45600=ORIENTED_EDGE('',*,*,#34155,.T.);
#45601=ORIENTED_EDGE('',*,*,#34156,.T.);
#45602=ORIENTED_EDGE('',*,*,#34151,.F.);
#45603=ORIENTED_EDGE('',*,*,#34157,.F.);
#45604=ORIENTED_EDGE('',*,*,#34158,.T.);
#45605=ORIENTED_EDGE('',*,*,#34159,.T.);
#45606=ORIENTED_EDGE('',*,*,#34155,.F.);
#45607=ORIENTED_EDGE('',*,*,#34160,.F.);
#45608=ORIENTED_EDGE('',*,*,#34153,.T.);
#45609=ORIENTED_EDGE('',*,*,#34161,.T.);
#45610=ORIENTED_EDGE('',*,*,#34158,.F.);
#45611=ORIENTED_EDGE('',*,*,#34161,.F.);
#45612=ORIENTED_EDGE('',*,*,#34152,.F.);
#45613=ORIENTED_EDGE('',*,*,#34156,.F.);
#45614=ORIENTED_EDGE('',*,*,#34159,.F.);
#45615=ORIENTED_EDGE('',*,*,#34162,.F.);
#45616=ORIENTED_EDGE('',*,*,#34163,.T.);
#45617=ORIENTED_EDGE('',*,*,#34164,.T.);
#45618=ORIENTED_EDGE('',*,*,#34165,.F.);
#45619=ORIENTED_EDGE('',*,*,#34166,.F.);
#45620=ORIENTED_EDGE('',*,*,#34167,.T.);
#45621=ORIENTED_EDGE('',*,*,#34168,.T.);
#45622=ORIENTED_EDGE('',*,*,#34163,.F.);
#45623=ORIENTED_EDGE('',*,*,#34169,.F.);
#45624=ORIENTED_EDGE('',*,*,#34170,.T.);
#45625=ORIENTED_EDGE('',*,*,#34171,.T.);
#45626=ORIENTED_EDGE('',*,*,#34167,.F.);
#45627=ORIENTED_EDGE('',*,*,#34172,.F.);
#45628=ORIENTED_EDGE('',*,*,#34165,.T.);
#45629=ORIENTED_EDGE('',*,*,#34173,.T.);
#45630=ORIENTED_EDGE('',*,*,#34170,.F.);
#45631=ORIENTED_EDGE('',*,*,#34173,.F.);
#45632=ORIENTED_EDGE('',*,*,#34164,.F.);
#45633=ORIENTED_EDGE('',*,*,#34168,.F.);
#45634=ORIENTED_EDGE('',*,*,#34171,.F.);
#45635=ORIENTED_EDGE('',*,*,#34174,.F.);
#45636=ORIENTED_EDGE('',*,*,#34175,.T.);
#45637=ORIENTED_EDGE('',*,*,#34176,.T.);
#45638=ORIENTED_EDGE('',*,*,#34177,.F.);
#45639=ORIENTED_EDGE('',*,*,#34178,.F.);
#45640=ORIENTED_EDGE('',*,*,#34179,.T.);
#45641=ORIENTED_EDGE('',*,*,#34180,.T.);
#45642=ORIENTED_EDGE('',*,*,#34175,.F.);
#45643=ORIENTED_EDGE('',*,*,#34181,.F.);
#45644=ORIENTED_EDGE('',*,*,#34182,.T.);
#45645=ORIENTED_EDGE('',*,*,#34183,.T.);
#45646=ORIENTED_EDGE('',*,*,#34179,.F.);
#45647=ORIENTED_EDGE('',*,*,#34184,.F.);
#45648=ORIENTED_EDGE('',*,*,#34177,.T.);
#45649=ORIENTED_EDGE('',*,*,#34185,.T.);
#45650=ORIENTED_EDGE('',*,*,#34182,.F.);
#45651=ORIENTED_EDGE('',*,*,#34185,.F.);
#45652=ORIENTED_EDGE('',*,*,#34176,.F.);
#45653=ORIENTED_EDGE('',*,*,#34180,.F.);
#45654=ORIENTED_EDGE('',*,*,#34183,.F.);
#45655=ORIENTED_EDGE('',*,*,#34186,.F.);
#45656=ORIENTED_EDGE('',*,*,#34187,.T.);
#45657=ORIENTED_EDGE('',*,*,#34188,.T.);
#45658=ORIENTED_EDGE('',*,*,#34189,.F.);
#45659=ORIENTED_EDGE('',*,*,#34190,.F.);
#45660=ORIENTED_EDGE('',*,*,#34191,.T.);
#45661=ORIENTED_EDGE('',*,*,#34192,.T.);
#45662=ORIENTED_EDGE('',*,*,#34187,.F.);
#45663=ORIENTED_EDGE('',*,*,#34193,.F.);
#45664=ORIENTED_EDGE('',*,*,#34194,.T.);
#45665=ORIENTED_EDGE('',*,*,#34195,.T.);
#45666=ORIENTED_EDGE('',*,*,#34191,.F.);
#45667=ORIENTED_EDGE('',*,*,#34196,.F.);
#45668=ORIENTED_EDGE('',*,*,#34189,.T.);
#45669=ORIENTED_EDGE('',*,*,#34197,.T.);
#45670=ORIENTED_EDGE('',*,*,#34194,.F.);
#45671=ORIENTED_EDGE('',*,*,#34197,.F.);
#45672=ORIENTED_EDGE('',*,*,#34188,.F.);
#45673=ORIENTED_EDGE('',*,*,#34192,.F.);
#45674=ORIENTED_EDGE('',*,*,#34195,.F.);
#45675=ORIENTED_EDGE('',*,*,#34198,.F.);
#45676=ORIENTED_EDGE('',*,*,#34199,.T.);
#45677=ORIENTED_EDGE('',*,*,#34200,.T.);
#45678=ORIENTED_EDGE('',*,*,#34201,.F.);
#45679=ORIENTED_EDGE('',*,*,#34202,.F.);
#45680=ORIENTED_EDGE('',*,*,#34203,.T.);
#45681=ORIENTED_EDGE('',*,*,#34204,.T.);
#45682=ORIENTED_EDGE('',*,*,#34199,.F.);
#45683=ORIENTED_EDGE('',*,*,#34205,.F.);
#45684=ORIENTED_EDGE('',*,*,#34206,.T.);
#45685=ORIENTED_EDGE('',*,*,#34207,.T.);
#45686=ORIENTED_EDGE('',*,*,#34203,.F.);
#45687=ORIENTED_EDGE('',*,*,#34208,.F.);
#45688=ORIENTED_EDGE('',*,*,#34201,.T.);
#45689=ORIENTED_EDGE('',*,*,#34209,.T.);
#45690=ORIENTED_EDGE('',*,*,#34206,.F.);
#45691=ORIENTED_EDGE('',*,*,#34209,.F.);
#45692=ORIENTED_EDGE('',*,*,#34200,.F.);
#45693=ORIENTED_EDGE('',*,*,#34204,.F.);
#45694=ORIENTED_EDGE('',*,*,#34207,.F.);
#45695=ORIENTED_EDGE('',*,*,#34210,.F.);
#45696=ORIENTED_EDGE('',*,*,#34211,.T.);
#45697=ORIENTED_EDGE('',*,*,#34212,.T.);
#45698=ORIENTED_EDGE('',*,*,#34213,.F.);
#45699=ORIENTED_EDGE('',*,*,#34214,.F.);
#45700=ORIENTED_EDGE('',*,*,#34215,.T.);
#45701=ORIENTED_EDGE('',*,*,#34216,.T.);
#45702=ORIENTED_EDGE('',*,*,#34211,.F.);
#45703=ORIENTED_EDGE('',*,*,#34217,.F.);
#45704=ORIENTED_EDGE('',*,*,#34218,.T.);
#45705=ORIENTED_EDGE('',*,*,#34219,.T.);
#45706=ORIENTED_EDGE('',*,*,#34215,.F.);
#45707=ORIENTED_EDGE('',*,*,#34220,.F.);
#45708=ORIENTED_EDGE('',*,*,#34213,.T.);
#45709=ORIENTED_EDGE('',*,*,#34221,.T.);
#45710=ORIENTED_EDGE('',*,*,#34218,.F.);
#45711=ORIENTED_EDGE('',*,*,#34221,.F.);
#45712=ORIENTED_EDGE('',*,*,#34212,.F.);
#45713=ORIENTED_EDGE('',*,*,#34216,.F.);
#45714=ORIENTED_EDGE('',*,*,#34219,.F.);
#45715=ORIENTED_EDGE('',*,*,#34222,.F.);
#45716=ORIENTED_EDGE('',*,*,#34223,.T.);
#45717=ORIENTED_EDGE('',*,*,#34224,.T.);
#45718=ORIENTED_EDGE('',*,*,#34225,.F.);
#45719=ORIENTED_EDGE('',*,*,#34226,.F.);
#45720=ORIENTED_EDGE('',*,*,#34227,.T.);
#45721=ORIENTED_EDGE('',*,*,#34228,.T.);
#45722=ORIENTED_EDGE('',*,*,#34223,.F.);
#45723=ORIENTED_EDGE('',*,*,#34229,.F.);
#45724=ORIENTED_EDGE('',*,*,#34230,.T.);
#45725=ORIENTED_EDGE('',*,*,#34231,.T.);
#45726=ORIENTED_EDGE('',*,*,#34227,.F.);
#45727=ORIENTED_EDGE('',*,*,#34232,.F.);
#45728=ORIENTED_EDGE('',*,*,#34225,.T.);
#45729=ORIENTED_EDGE('',*,*,#34233,.T.);
#45730=ORIENTED_EDGE('',*,*,#34230,.F.);
#45731=ORIENTED_EDGE('',*,*,#34233,.F.);
#45732=ORIENTED_EDGE('',*,*,#34224,.F.);
#45733=ORIENTED_EDGE('',*,*,#34228,.F.);
#45734=ORIENTED_EDGE('',*,*,#34231,.F.);
#45735=ORIENTED_EDGE('',*,*,#34234,.F.);
#45736=ORIENTED_EDGE('',*,*,#34235,.T.);
#45737=ORIENTED_EDGE('',*,*,#34236,.T.);
#45738=ORIENTED_EDGE('',*,*,#34237,.F.);
#45739=ORIENTED_EDGE('',*,*,#34238,.F.);
#45740=ORIENTED_EDGE('',*,*,#34239,.T.);
#45741=ORIENTED_EDGE('',*,*,#34240,.T.);
#45742=ORIENTED_EDGE('',*,*,#34235,.F.);
#45743=ORIENTED_EDGE('',*,*,#34241,.F.);
#45744=ORIENTED_EDGE('',*,*,#34242,.T.);
#45745=ORIENTED_EDGE('',*,*,#34243,.T.);
#45746=ORIENTED_EDGE('',*,*,#34239,.F.);
#45747=ORIENTED_EDGE('',*,*,#34244,.F.);
#45748=ORIENTED_EDGE('',*,*,#34237,.T.);
#45749=ORIENTED_EDGE('',*,*,#34245,.T.);
#45750=ORIENTED_EDGE('',*,*,#34242,.F.);
#45751=ORIENTED_EDGE('',*,*,#34245,.F.);
#45752=ORIENTED_EDGE('',*,*,#34236,.F.);
#45753=ORIENTED_EDGE('',*,*,#34240,.F.);
#45754=ORIENTED_EDGE('',*,*,#34243,.F.);
#45755=ORIENTED_EDGE('',*,*,#34246,.F.);
#45756=ORIENTED_EDGE('',*,*,#34247,.T.);
#45757=ORIENTED_EDGE('',*,*,#34248,.T.);
#45758=ORIENTED_EDGE('',*,*,#34249,.F.);
#45759=ORIENTED_EDGE('',*,*,#34250,.F.);
#45760=ORIENTED_EDGE('',*,*,#34251,.T.);
#45761=ORIENTED_EDGE('',*,*,#34252,.T.);
#45762=ORIENTED_EDGE('',*,*,#34247,.F.);
#45763=ORIENTED_EDGE('',*,*,#34253,.F.);
#45764=ORIENTED_EDGE('',*,*,#34254,.T.);
#45765=ORIENTED_EDGE('',*,*,#34255,.T.);
#45766=ORIENTED_EDGE('',*,*,#34251,.F.);
#45767=ORIENTED_EDGE('',*,*,#34256,.F.);
#45768=ORIENTED_EDGE('',*,*,#34249,.T.);
#45769=ORIENTED_EDGE('',*,*,#34257,.T.);
#45770=ORIENTED_EDGE('',*,*,#34254,.F.);
#45771=ORIENTED_EDGE('',*,*,#34257,.F.);
#45772=ORIENTED_EDGE('',*,*,#34248,.F.);
#45773=ORIENTED_EDGE('',*,*,#34252,.F.);
#45774=ORIENTED_EDGE('',*,*,#34255,.F.);
#45775=ORIENTED_EDGE('',*,*,#34258,.F.);
#45776=ORIENTED_EDGE('',*,*,#34259,.T.);
#45777=ORIENTED_EDGE('',*,*,#34260,.T.);
#45778=ORIENTED_EDGE('',*,*,#34261,.F.);
#45779=ORIENTED_EDGE('',*,*,#34262,.F.);
#45780=ORIENTED_EDGE('',*,*,#34263,.T.);
#45781=ORIENTED_EDGE('',*,*,#34264,.T.);
#45782=ORIENTED_EDGE('',*,*,#34259,.F.);
#45783=ORIENTED_EDGE('',*,*,#34265,.F.);
#45784=ORIENTED_EDGE('',*,*,#34266,.T.);
#45785=ORIENTED_EDGE('',*,*,#34267,.T.);
#45786=ORIENTED_EDGE('',*,*,#34263,.F.);
#45787=ORIENTED_EDGE('',*,*,#34268,.F.);
#45788=ORIENTED_EDGE('',*,*,#34261,.T.);
#45789=ORIENTED_EDGE('',*,*,#34269,.T.);
#45790=ORIENTED_EDGE('',*,*,#34266,.F.);
#45791=ORIENTED_EDGE('',*,*,#34269,.F.);
#45792=ORIENTED_EDGE('',*,*,#34260,.F.);
#45793=ORIENTED_EDGE('',*,*,#34264,.F.);
#45794=ORIENTED_EDGE('',*,*,#34267,.F.);
#45795=ORIENTED_EDGE('',*,*,#34270,.F.);
#45796=ORIENTED_EDGE('',*,*,#34271,.T.);
#45797=ORIENTED_EDGE('',*,*,#34272,.T.);
#45798=ORIENTED_EDGE('',*,*,#34273,.F.);
#45799=ORIENTED_EDGE('',*,*,#34274,.F.);
#45800=ORIENTED_EDGE('',*,*,#34275,.T.);
#45801=ORIENTED_EDGE('',*,*,#34276,.T.);
#45802=ORIENTED_EDGE('',*,*,#34271,.F.);
#45803=ORIENTED_EDGE('',*,*,#34277,.F.);
#45804=ORIENTED_EDGE('',*,*,#34278,.T.);
#45805=ORIENTED_EDGE('',*,*,#34279,.T.);
#45806=ORIENTED_EDGE('',*,*,#34275,.F.);
#45807=ORIENTED_EDGE('',*,*,#34280,.F.);
#45808=ORIENTED_EDGE('',*,*,#34273,.T.);
#45809=ORIENTED_EDGE('',*,*,#34281,.T.);
#45810=ORIENTED_EDGE('',*,*,#34278,.F.);
#45811=ORIENTED_EDGE('',*,*,#34281,.F.);
#45812=ORIENTED_EDGE('',*,*,#34272,.F.);
#45813=ORIENTED_EDGE('',*,*,#34276,.F.);
#45814=ORIENTED_EDGE('',*,*,#34279,.F.);
#45815=ORIENTED_EDGE('',*,*,#34282,.F.);
#45816=ORIENTED_EDGE('',*,*,#34283,.T.);
#45817=ORIENTED_EDGE('',*,*,#34284,.T.);
#45818=ORIENTED_EDGE('',*,*,#34285,.F.);
#45819=ORIENTED_EDGE('',*,*,#34286,.F.);
#45820=ORIENTED_EDGE('',*,*,#34287,.T.);
#45821=ORIENTED_EDGE('',*,*,#34288,.T.);
#45822=ORIENTED_EDGE('',*,*,#34283,.F.);
#45823=ORIENTED_EDGE('',*,*,#34289,.F.);
#45824=ORIENTED_EDGE('',*,*,#34290,.T.);
#45825=ORIENTED_EDGE('',*,*,#34291,.T.);
#45826=ORIENTED_EDGE('',*,*,#34287,.F.);
#45827=ORIENTED_EDGE('',*,*,#34292,.F.);
#45828=ORIENTED_EDGE('',*,*,#34285,.T.);
#45829=ORIENTED_EDGE('',*,*,#34293,.T.);
#45830=ORIENTED_EDGE('',*,*,#34290,.F.);
#45831=ORIENTED_EDGE('',*,*,#34293,.F.);
#45832=ORIENTED_EDGE('',*,*,#34284,.F.);
#45833=ORIENTED_EDGE('',*,*,#34288,.F.);
#45834=ORIENTED_EDGE('',*,*,#34291,.F.);
#45835=ORIENTED_EDGE('',*,*,#34294,.F.);
#45836=ORIENTED_EDGE('',*,*,#34295,.T.);
#45837=ORIENTED_EDGE('',*,*,#34296,.T.);
#45838=ORIENTED_EDGE('',*,*,#34297,.F.);
#45839=ORIENTED_EDGE('',*,*,#34298,.F.);
#45840=ORIENTED_EDGE('',*,*,#34299,.T.);
#45841=ORIENTED_EDGE('',*,*,#34300,.T.);
#45842=ORIENTED_EDGE('',*,*,#34295,.F.);
#45843=ORIENTED_EDGE('',*,*,#34301,.F.);
#45844=ORIENTED_EDGE('',*,*,#34302,.T.);
#45845=ORIENTED_EDGE('',*,*,#34303,.T.);
#45846=ORIENTED_EDGE('',*,*,#34299,.F.);
#45847=ORIENTED_EDGE('',*,*,#34304,.F.);
#45848=ORIENTED_EDGE('',*,*,#34297,.T.);
#45849=ORIENTED_EDGE('',*,*,#34305,.T.);
#45850=ORIENTED_EDGE('',*,*,#34302,.F.);
#45851=ORIENTED_EDGE('',*,*,#34305,.F.);
#45852=ORIENTED_EDGE('',*,*,#34296,.F.);
#45853=ORIENTED_EDGE('',*,*,#34300,.F.);
#45854=ORIENTED_EDGE('',*,*,#34303,.F.);
#45855=ORIENTED_EDGE('',*,*,#34306,.F.);
#45856=ORIENTED_EDGE('',*,*,#34307,.T.);
#45857=ORIENTED_EDGE('',*,*,#34308,.T.);
#45858=ORIENTED_EDGE('',*,*,#34309,.F.);
#45859=ORIENTED_EDGE('',*,*,#34310,.F.);
#45860=ORIENTED_EDGE('',*,*,#34311,.T.);
#45861=ORIENTED_EDGE('',*,*,#34312,.T.);
#45862=ORIENTED_EDGE('',*,*,#34307,.F.);
#45863=ORIENTED_EDGE('',*,*,#34313,.F.);
#45864=ORIENTED_EDGE('',*,*,#34314,.T.);
#45865=ORIENTED_EDGE('',*,*,#34315,.T.);
#45866=ORIENTED_EDGE('',*,*,#34311,.F.);
#45867=ORIENTED_EDGE('',*,*,#34316,.F.);
#45868=ORIENTED_EDGE('',*,*,#34309,.T.);
#45869=ORIENTED_EDGE('',*,*,#34317,.T.);
#45870=ORIENTED_EDGE('',*,*,#34314,.F.);
#45871=ORIENTED_EDGE('',*,*,#34317,.F.);
#45872=ORIENTED_EDGE('',*,*,#34308,.F.);
#45873=ORIENTED_EDGE('',*,*,#34312,.F.);
#45874=ORIENTED_EDGE('',*,*,#34315,.F.);
#45875=ORIENTED_EDGE('',*,*,#34318,.F.);
#45876=ORIENTED_EDGE('',*,*,#34319,.T.);
#45877=ORIENTED_EDGE('',*,*,#34320,.T.);
#45878=ORIENTED_EDGE('',*,*,#34321,.F.);
#45879=ORIENTED_EDGE('',*,*,#34322,.F.);
#45880=ORIENTED_EDGE('',*,*,#34323,.T.);
#45881=ORIENTED_EDGE('',*,*,#34324,.T.);
#45882=ORIENTED_EDGE('',*,*,#34319,.F.);
#45883=ORIENTED_EDGE('',*,*,#34325,.F.);
#45884=ORIENTED_EDGE('',*,*,#34326,.T.);
#45885=ORIENTED_EDGE('',*,*,#34327,.T.);
#45886=ORIENTED_EDGE('',*,*,#34323,.F.);
#45887=ORIENTED_EDGE('',*,*,#34328,.F.);
#45888=ORIENTED_EDGE('',*,*,#34321,.T.);
#45889=ORIENTED_EDGE('',*,*,#34329,.T.);
#45890=ORIENTED_EDGE('',*,*,#34326,.F.);
#45891=ORIENTED_EDGE('',*,*,#34329,.F.);
#45892=ORIENTED_EDGE('',*,*,#34320,.F.);
#45893=ORIENTED_EDGE('',*,*,#34324,.F.);
#45894=ORIENTED_EDGE('',*,*,#34327,.F.);
#45895=ORIENTED_EDGE('',*,*,#34330,.F.);
#45896=ORIENTED_EDGE('',*,*,#34331,.T.);
#45897=ORIENTED_EDGE('',*,*,#34332,.T.);
#45898=ORIENTED_EDGE('',*,*,#34333,.F.);
#45899=ORIENTED_EDGE('',*,*,#34334,.F.);
#45900=ORIENTED_EDGE('',*,*,#34335,.T.);
#45901=ORIENTED_EDGE('',*,*,#34336,.T.);
#45902=ORIENTED_EDGE('',*,*,#34331,.F.);
#45903=ORIENTED_EDGE('',*,*,#34337,.F.);
#45904=ORIENTED_EDGE('',*,*,#34338,.T.);
#45905=ORIENTED_EDGE('',*,*,#34339,.T.);
#45906=ORIENTED_EDGE('',*,*,#34335,.F.);
#45907=ORIENTED_EDGE('',*,*,#34340,.F.);
#45908=ORIENTED_EDGE('',*,*,#34333,.T.);
#45909=ORIENTED_EDGE('',*,*,#34341,.T.);
#45910=ORIENTED_EDGE('',*,*,#34338,.F.);
#45911=ORIENTED_EDGE('',*,*,#34341,.F.);
#45912=ORIENTED_EDGE('',*,*,#34332,.F.);
#45913=ORIENTED_EDGE('',*,*,#34336,.F.);
#45914=ORIENTED_EDGE('',*,*,#34339,.F.);
#45915=ORIENTED_EDGE('',*,*,#34342,.F.);
#45916=ORIENTED_EDGE('',*,*,#34343,.T.);
#45917=ORIENTED_EDGE('',*,*,#34344,.T.);
#45918=ORIENTED_EDGE('',*,*,#34345,.F.);
#45919=ORIENTED_EDGE('',*,*,#34346,.F.);
#45920=ORIENTED_EDGE('',*,*,#34347,.T.);
#45921=ORIENTED_EDGE('',*,*,#34348,.T.);
#45922=ORIENTED_EDGE('',*,*,#34343,.F.);
#45923=ORIENTED_EDGE('',*,*,#34349,.F.);
#45924=ORIENTED_EDGE('',*,*,#34350,.T.);
#45925=ORIENTED_EDGE('',*,*,#34351,.T.);
#45926=ORIENTED_EDGE('',*,*,#34347,.F.);
#45927=ORIENTED_EDGE('',*,*,#34352,.F.);
#45928=ORIENTED_EDGE('',*,*,#34345,.T.);
#45929=ORIENTED_EDGE('',*,*,#34353,.T.);
#45930=ORIENTED_EDGE('',*,*,#34350,.F.);
#45931=ORIENTED_EDGE('',*,*,#34353,.F.);
#45932=ORIENTED_EDGE('',*,*,#34344,.F.);
#45933=ORIENTED_EDGE('',*,*,#34348,.F.);
#45934=ORIENTED_EDGE('',*,*,#34351,.F.);
#45935=ORIENTED_EDGE('',*,*,#34354,.F.);
#45936=ORIENTED_EDGE('',*,*,#34355,.T.);
#45937=ORIENTED_EDGE('',*,*,#34356,.T.);
#45938=ORIENTED_EDGE('',*,*,#34357,.F.);
#45939=ORIENTED_EDGE('',*,*,#34358,.F.);
#45940=ORIENTED_EDGE('',*,*,#34359,.T.);
#45941=ORIENTED_EDGE('',*,*,#34360,.T.);
#45942=ORIENTED_EDGE('',*,*,#34355,.F.);
#45943=ORIENTED_EDGE('',*,*,#34361,.F.);
#45944=ORIENTED_EDGE('',*,*,#34362,.T.);
#45945=ORIENTED_EDGE('',*,*,#34363,.T.);
#45946=ORIENTED_EDGE('',*,*,#34359,.F.);
#45947=ORIENTED_EDGE('',*,*,#34364,.F.);
#45948=ORIENTED_EDGE('',*,*,#34357,.T.);
#45949=ORIENTED_EDGE('',*,*,#34365,.T.);
#45950=ORIENTED_EDGE('',*,*,#34362,.F.);
#45951=ORIENTED_EDGE('',*,*,#34365,.F.);
#45952=ORIENTED_EDGE('',*,*,#34356,.F.);
#45953=ORIENTED_EDGE('',*,*,#34360,.F.);
#45954=ORIENTED_EDGE('',*,*,#34363,.F.);
#45955=ORIENTED_EDGE('',*,*,#34366,.F.);
#45956=ORIENTED_EDGE('',*,*,#34367,.T.);
#45957=ORIENTED_EDGE('',*,*,#34368,.T.);
#45958=ORIENTED_EDGE('',*,*,#34369,.F.);
#45959=ORIENTED_EDGE('',*,*,#34370,.F.);
#45960=ORIENTED_EDGE('',*,*,#34371,.T.);
#45961=ORIENTED_EDGE('',*,*,#34372,.T.);
#45962=ORIENTED_EDGE('',*,*,#34367,.F.);
#45963=ORIENTED_EDGE('',*,*,#34373,.F.);
#45964=ORIENTED_EDGE('',*,*,#34374,.T.);
#45965=ORIENTED_EDGE('',*,*,#34375,.T.);
#45966=ORIENTED_EDGE('',*,*,#34371,.F.);
#45967=ORIENTED_EDGE('',*,*,#34376,.F.);
#45968=ORIENTED_EDGE('',*,*,#34369,.T.);
#45969=ORIENTED_EDGE('',*,*,#34377,.T.);
#45970=ORIENTED_EDGE('',*,*,#34374,.F.);
#45971=ORIENTED_EDGE('',*,*,#34377,.F.);
#45972=ORIENTED_EDGE('',*,*,#34368,.F.);
#45973=ORIENTED_EDGE('',*,*,#34372,.F.);
#45974=ORIENTED_EDGE('',*,*,#34375,.F.);
#45975=ORIENTED_EDGE('',*,*,#34378,.F.);
#45976=ORIENTED_EDGE('',*,*,#34379,.T.);
#45977=ORIENTED_EDGE('',*,*,#34380,.T.);
#45978=ORIENTED_EDGE('',*,*,#34381,.F.);
#45979=ORIENTED_EDGE('',*,*,#34382,.F.);
#45980=ORIENTED_EDGE('',*,*,#34383,.T.);
#45981=ORIENTED_EDGE('',*,*,#34384,.T.);
#45982=ORIENTED_EDGE('',*,*,#34379,.F.);
#45983=ORIENTED_EDGE('',*,*,#34385,.F.);
#45984=ORIENTED_EDGE('',*,*,#34386,.T.);
#45985=ORIENTED_EDGE('',*,*,#34387,.T.);
#45986=ORIENTED_EDGE('',*,*,#34383,.F.);
#45987=ORIENTED_EDGE('',*,*,#34388,.F.);
#45988=ORIENTED_EDGE('',*,*,#34381,.T.);
#45989=ORIENTED_EDGE('',*,*,#34389,.T.);
#45990=ORIENTED_EDGE('',*,*,#34386,.F.);
#45991=ORIENTED_EDGE('',*,*,#34389,.F.);
#45992=ORIENTED_EDGE('',*,*,#34380,.F.);
#45993=ORIENTED_EDGE('',*,*,#34384,.F.);
#45994=ORIENTED_EDGE('',*,*,#34387,.F.);
#45995=ORIENTED_EDGE('',*,*,#34390,.F.);
#45996=ORIENTED_EDGE('',*,*,#34391,.T.);
#45997=ORIENTED_EDGE('',*,*,#34392,.T.);
#45998=ORIENTED_EDGE('',*,*,#34393,.F.);
#45999=ORIENTED_EDGE('',*,*,#34394,.F.);
#46000=ORIENTED_EDGE('',*,*,#34395,.T.);
#46001=ORIENTED_EDGE('',*,*,#34396,.T.);
#46002=ORIENTED_EDGE('',*,*,#34391,.F.);
#46003=ORIENTED_EDGE('',*,*,#34397,.F.);
#46004=ORIENTED_EDGE('',*,*,#34398,.T.);
#46005=ORIENTED_EDGE('',*,*,#34399,.T.);
#46006=ORIENTED_EDGE('',*,*,#34395,.F.);
#46007=ORIENTED_EDGE('',*,*,#34400,.F.);
#46008=ORIENTED_EDGE('',*,*,#34393,.T.);
#46009=ORIENTED_EDGE('',*,*,#34401,.T.);
#46010=ORIENTED_EDGE('',*,*,#34398,.F.);
#46011=ORIENTED_EDGE('',*,*,#34401,.F.);
#46012=ORIENTED_EDGE('',*,*,#34392,.F.);
#46013=ORIENTED_EDGE('',*,*,#34396,.F.);
#46014=ORIENTED_EDGE('',*,*,#34399,.F.);
#46015=ORIENTED_EDGE('',*,*,#34402,.F.);
#46016=ORIENTED_EDGE('',*,*,#34403,.T.);
#46017=ORIENTED_EDGE('',*,*,#34404,.T.);
#46018=ORIENTED_EDGE('',*,*,#34405,.F.);
#46019=ORIENTED_EDGE('',*,*,#34406,.F.);
#46020=ORIENTED_EDGE('',*,*,#34407,.T.);
#46021=ORIENTED_EDGE('',*,*,#34408,.T.);
#46022=ORIENTED_EDGE('',*,*,#34403,.F.);
#46023=ORIENTED_EDGE('',*,*,#34409,.F.);
#46024=ORIENTED_EDGE('',*,*,#34410,.T.);
#46025=ORIENTED_EDGE('',*,*,#34411,.T.);
#46026=ORIENTED_EDGE('',*,*,#34407,.F.);
#46027=ORIENTED_EDGE('',*,*,#34412,.F.);
#46028=ORIENTED_EDGE('',*,*,#34405,.T.);
#46029=ORIENTED_EDGE('',*,*,#34413,.T.);
#46030=ORIENTED_EDGE('',*,*,#34410,.F.);
#46031=ORIENTED_EDGE('',*,*,#34413,.F.);
#46032=ORIENTED_EDGE('',*,*,#34404,.F.);
#46033=ORIENTED_EDGE('',*,*,#34408,.F.);
#46034=ORIENTED_EDGE('',*,*,#34411,.F.);
#46035=ORIENTED_EDGE('',*,*,#34414,.F.);
#46036=ORIENTED_EDGE('',*,*,#34415,.T.);
#46037=ORIENTED_EDGE('',*,*,#34416,.T.);
#46038=ORIENTED_EDGE('',*,*,#34417,.F.);
#46039=ORIENTED_EDGE('',*,*,#34418,.F.);
#46040=ORIENTED_EDGE('',*,*,#34419,.T.);
#46041=ORIENTED_EDGE('',*,*,#34420,.T.);
#46042=ORIENTED_EDGE('',*,*,#34415,.F.);
#46043=ORIENTED_EDGE('',*,*,#34421,.F.);
#46044=ORIENTED_EDGE('',*,*,#34422,.T.);
#46045=ORIENTED_EDGE('',*,*,#34423,.T.);
#46046=ORIENTED_EDGE('',*,*,#34419,.F.);
#46047=ORIENTED_EDGE('',*,*,#34424,.F.);
#46048=ORIENTED_EDGE('',*,*,#34417,.T.);
#46049=ORIENTED_EDGE('',*,*,#34425,.T.);
#46050=ORIENTED_EDGE('',*,*,#34422,.F.);
#46051=ORIENTED_EDGE('',*,*,#34425,.F.);
#46052=ORIENTED_EDGE('',*,*,#34416,.F.);
#46053=ORIENTED_EDGE('',*,*,#34420,.F.);
#46054=ORIENTED_EDGE('',*,*,#34423,.F.);
#46055=ORIENTED_EDGE('',*,*,#34426,.F.);
#46056=ORIENTED_EDGE('',*,*,#34427,.T.);
#46057=ORIENTED_EDGE('',*,*,#34428,.T.);
#46058=ORIENTED_EDGE('',*,*,#34429,.F.);
#46059=ORIENTED_EDGE('',*,*,#34430,.F.);
#46060=ORIENTED_EDGE('',*,*,#34431,.T.);
#46061=ORIENTED_EDGE('',*,*,#34432,.T.);
#46062=ORIENTED_EDGE('',*,*,#34427,.F.);
#46063=ORIENTED_EDGE('',*,*,#34433,.F.);
#46064=ORIENTED_EDGE('',*,*,#34434,.T.);
#46065=ORIENTED_EDGE('',*,*,#34435,.T.);
#46066=ORIENTED_EDGE('',*,*,#34431,.F.);
#46067=ORIENTED_EDGE('',*,*,#34436,.F.);
#46068=ORIENTED_EDGE('',*,*,#34429,.T.);
#46069=ORIENTED_EDGE('',*,*,#34437,.T.);
#46070=ORIENTED_EDGE('',*,*,#34434,.F.);
#46071=ORIENTED_EDGE('',*,*,#34437,.F.);
#46072=ORIENTED_EDGE('',*,*,#34428,.F.);
#46073=ORIENTED_EDGE('',*,*,#34432,.F.);
#46074=ORIENTED_EDGE('',*,*,#34435,.F.);
#46075=ORIENTED_EDGE('',*,*,#34438,.F.);
#46076=ORIENTED_EDGE('',*,*,#34439,.T.);
#46077=ORIENTED_EDGE('',*,*,#34440,.T.);
#46078=ORIENTED_EDGE('',*,*,#34441,.F.);
#46079=ORIENTED_EDGE('',*,*,#34442,.F.);
#46080=ORIENTED_EDGE('',*,*,#34443,.T.);
#46081=ORIENTED_EDGE('',*,*,#34444,.T.);
#46082=ORIENTED_EDGE('',*,*,#34439,.F.);
#46083=ORIENTED_EDGE('',*,*,#34445,.F.);
#46084=ORIENTED_EDGE('',*,*,#34446,.T.);
#46085=ORIENTED_EDGE('',*,*,#34447,.T.);
#46086=ORIENTED_EDGE('',*,*,#34443,.F.);
#46087=ORIENTED_EDGE('',*,*,#34448,.F.);
#46088=ORIENTED_EDGE('',*,*,#34441,.T.);
#46089=ORIENTED_EDGE('',*,*,#34449,.T.);
#46090=ORIENTED_EDGE('',*,*,#34446,.F.);
#46091=ORIENTED_EDGE('',*,*,#34449,.F.);
#46092=ORIENTED_EDGE('',*,*,#34440,.F.);
#46093=ORIENTED_EDGE('',*,*,#34444,.F.);
#46094=ORIENTED_EDGE('',*,*,#34447,.F.);
#46095=ORIENTED_EDGE('',*,*,#34450,.F.);
#46096=ORIENTED_EDGE('',*,*,#34451,.T.);
#46097=ORIENTED_EDGE('',*,*,#34452,.T.);
#46098=ORIENTED_EDGE('',*,*,#34453,.F.);
#46099=ORIENTED_EDGE('',*,*,#34454,.F.);
#46100=ORIENTED_EDGE('',*,*,#34455,.T.);
#46101=ORIENTED_EDGE('',*,*,#34456,.T.);
#46102=ORIENTED_EDGE('',*,*,#34451,.F.);
#46103=ORIENTED_EDGE('',*,*,#34457,.F.);
#46104=ORIENTED_EDGE('',*,*,#34458,.T.);
#46105=ORIENTED_EDGE('',*,*,#34459,.T.);
#46106=ORIENTED_EDGE('',*,*,#34455,.F.);
#46107=ORIENTED_EDGE('',*,*,#34460,.F.);
#46108=ORIENTED_EDGE('',*,*,#34453,.T.);
#46109=ORIENTED_EDGE('',*,*,#34461,.T.);
#46110=ORIENTED_EDGE('',*,*,#34458,.F.);
#46111=ORIENTED_EDGE('',*,*,#34461,.F.);
#46112=ORIENTED_EDGE('',*,*,#34452,.F.);
#46113=ORIENTED_EDGE('',*,*,#34456,.F.);
#46114=ORIENTED_EDGE('',*,*,#34459,.F.);
#46115=ORIENTED_EDGE('',*,*,#34462,.F.);
#46116=ORIENTED_EDGE('',*,*,#34463,.T.);
#46117=ORIENTED_EDGE('',*,*,#34464,.T.);
#46118=ORIENTED_EDGE('',*,*,#34465,.F.);
#46119=ORIENTED_EDGE('',*,*,#34466,.F.);
#46120=ORIENTED_EDGE('',*,*,#34467,.T.);
#46121=ORIENTED_EDGE('',*,*,#34468,.T.);
#46122=ORIENTED_EDGE('',*,*,#34463,.F.);
#46123=ORIENTED_EDGE('',*,*,#34469,.F.);
#46124=ORIENTED_EDGE('',*,*,#34470,.T.);
#46125=ORIENTED_EDGE('',*,*,#34471,.T.);
#46126=ORIENTED_EDGE('',*,*,#34467,.F.);
#46127=ORIENTED_EDGE('',*,*,#34472,.F.);
#46128=ORIENTED_EDGE('',*,*,#34465,.T.);
#46129=ORIENTED_EDGE('',*,*,#34473,.T.);
#46130=ORIENTED_EDGE('',*,*,#34470,.F.);
#46131=ORIENTED_EDGE('',*,*,#34473,.F.);
#46132=ORIENTED_EDGE('',*,*,#34464,.F.);
#46133=ORIENTED_EDGE('',*,*,#34468,.F.);
#46134=ORIENTED_EDGE('',*,*,#34471,.F.);
#46135=ORIENTED_EDGE('',*,*,#34474,.F.);
#46136=ORIENTED_EDGE('',*,*,#34475,.T.);
#46137=ORIENTED_EDGE('',*,*,#34476,.T.);
#46138=ORIENTED_EDGE('',*,*,#34477,.F.);
#46139=ORIENTED_EDGE('',*,*,#34478,.F.);
#46140=ORIENTED_EDGE('',*,*,#34479,.T.);
#46141=ORIENTED_EDGE('',*,*,#34480,.T.);
#46142=ORIENTED_EDGE('',*,*,#34475,.F.);
#46143=ORIENTED_EDGE('',*,*,#34481,.F.);
#46144=ORIENTED_EDGE('',*,*,#34482,.T.);
#46145=ORIENTED_EDGE('',*,*,#34483,.T.);
#46146=ORIENTED_EDGE('',*,*,#34479,.F.);
#46147=ORIENTED_EDGE('',*,*,#34484,.F.);
#46148=ORIENTED_EDGE('',*,*,#34477,.T.);
#46149=ORIENTED_EDGE('',*,*,#34485,.T.);
#46150=ORIENTED_EDGE('',*,*,#34482,.F.);
#46151=ORIENTED_EDGE('',*,*,#34485,.F.);
#46152=ORIENTED_EDGE('',*,*,#34476,.F.);
#46153=ORIENTED_EDGE('',*,*,#34480,.F.);
#46154=ORIENTED_EDGE('',*,*,#34483,.F.);
#46155=ORIENTED_EDGE('',*,*,#34486,.F.);
#46156=ORIENTED_EDGE('',*,*,#34487,.T.);
#46157=ORIENTED_EDGE('',*,*,#34488,.T.);
#46158=ORIENTED_EDGE('',*,*,#34489,.F.);
#46159=ORIENTED_EDGE('',*,*,#34490,.F.);
#46160=ORIENTED_EDGE('',*,*,#34491,.T.);
#46161=ORIENTED_EDGE('',*,*,#34492,.T.);
#46162=ORIENTED_EDGE('',*,*,#34487,.F.);
#46163=ORIENTED_EDGE('',*,*,#34493,.F.);
#46164=ORIENTED_EDGE('',*,*,#34494,.T.);
#46165=ORIENTED_EDGE('',*,*,#34495,.T.);
#46166=ORIENTED_EDGE('',*,*,#34491,.F.);
#46167=ORIENTED_EDGE('',*,*,#34496,.F.);
#46168=ORIENTED_EDGE('',*,*,#34489,.T.);
#46169=ORIENTED_EDGE('',*,*,#34497,.T.);
#46170=ORIENTED_EDGE('',*,*,#34494,.F.);
#46171=ORIENTED_EDGE('',*,*,#34497,.F.);
#46172=ORIENTED_EDGE('',*,*,#34488,.F.);
#46173=ORIENTED_EDGE('',*,*,#34492,.F.);
#46174=ORIENTED_EDGE('',*,*,#34495,.F.);
#46175=ORIENTED_EDGE('',*,*,#34498,.F.);
#46176=ORIENTED_EDGE('',*,*,#34499,.T.);
#46177=ORIENTED_EDGE('',*,*,#34500,.T.);
#46178=ORIENTED_EDGE('',*,*,#34501,.F.);
#46179=ORIENTED_EDGE('',*,*,#34502,.F.);
#46180=ORIENTED_EDGE('',*,*,#34503,.T.);
#46181=ORIENTED_EDGE('',*,*,#34504,.T.);
#46182=ORIENTED_EDGE('',*,*,#34499,.F.);
#46183=ORIENTED_EDGE('',*,*,#34505,.F.);
#46184=ORIENTED_EDGE('',*,*,#34506,.T.);
#46185=ORIENTED_EDGE('',*,*,#34507,.T.);
#46186=ORIENTED_EDGE('',*,*,#34503,.F.);
#46187=ORIENTED_EDGE('',*,*,#34508,.F.);
#46188=ORIENTED_EDGE('',*,*,#34501,.T.);
#46189=ORIENTED_EDGE('',*,*,#34509,.T.);
#46190=ORIENTED_EDGE('',*,*,#34506,.F.);
#46191=ORIENTED_EDGE('',*,*,#34509,.F.);
#46192=ORIENTED_EDGE('',*,*,#34500,.F.);
#46193=ORIENTED_EDGE('',*,*,#34504,.F.);
#46194=ORIENTED_EDGE('',*,*,#34507,.F.);
#46195=ORIENTED_EDGE('',*,*,#34510,.F.);
#46196=ORIENTED_EDGE('',*,*,#34511,.T.);
#46197=ORIENTED_EDGE('',*,*,#34512,.T.);
#46198=ORIENTED_EDGE('',*,*,#34513,.F.);
#46199=ORIENTED_EDGE('',*,*,#34514,.F.);
#46200=ORIENTED_EDGE('',*,*,#34515,.T.);
#46201=ORIENTED_EDGE('',*,*,#34516,.T.);
#46202=ORIENTED_EDGE('',*,*,#34511,.F.);
#46203=ORIENTED_EDGE('',*,*,#34517,.F.);
#46204=ORIENTED_EDGE('',*,*,#34518,.T.);
#46205=ORIENTED_EDGE('',*,*,#34519,.T.);
#46206=ORIENTED_EDGE('',*,*,#34515,.F.);
#46207=ORIENTED_EDGE('',*,*,#34520,.F.);
#46208=ORIENTED_EDGE('',*,*,#34513,.T.);
#46209=ORIENTED_EDGE('',*,*,#34521,.T.);
#46210=ORIENTED_EDGE('',*,*,#34518,.F.);
#46211=ORIENTED_EDGE('',*,*,#34521,.F.);
#46212=ORIENTED_EDGE('',*,*,#34512,.F.);
#46213=ORIENTED_EDGE('',*,*,#34516,.F.);
#46214=ORIENTED_EDGE('',*,*,#34519,.F.);
#46215=ORIENTED_EDGE('',*,*,#34522,.F.);
#46216=ORIENTED_EDGE('',*,*,#34523,.T.);
#46217=ORIENTED_EDGE('',*,*,#34524,.T.);
#46218=ORIENTED_EDGE('',*,*,#34525,.F.);
#46219=ORIENTED_EDGE('',*,*,#34526,.F.);
#46220=ORIENTED_EDGE('',*,*,#34527,.T.);
#46221=ORIENTED_EDGE('',*,*,#34528,.T.);
#46222=ORIENTED_EDGE('',*,*,#34523,.F.);
#46223=ORIENTED_EDGE('',*,*,#34529,.F.);
#46224=ORIENTED_EDGE('',*,*,#34530,.T.);
#46225=ORIENTED_EDGE('',*,*,#34531,.T.);
#46226=ORIENTED_EDGE('',*,*,#34527,.F.);
#46227=ORIENTED_EDGE('',*,*,#34532,.F.);
#46228=ORIENTED_EDGE('',*,*,#34525,.T.);
#46229=ORIENTED_EDGE('',*,*,#34533,.T.);
#46230=ORIENTED_EDGE('',*,*,#34530,.F.);
#46231=ORIENTED_EDGE('',*,*,#34533,.F.);
#46232=ORIENTED_EDGE('',*,*,#34524,.F.);
#46233=ORIENTED_EDGE('',*,*,#34528,.F.);
#46234=ORIENTED_EDGE('',*,*,#34531,.F.);
#46235=ORIENTED_EDGE('',*,*,#34534,.F.);
#46236=ORIENTED_EDGE('',*,*,#34535,.T.);
#46237=ORIENTED_EDGE('',*,*,#34536,.T.);
#46238=ORIENTED_EDGE('',*,*,#34537,.F.);
#46239=ORIENTED_EDGE('',*,*,#34538,.F.);
#46240=ORIENTED_EDGE('',*,*,#34539,.T.);
#46241=ORIENTED_EDGE('',*,*,#34540,.T.);
#46242=ORIENTED_EDGE('',*,*,#34535,.F.);
#46243=ORIENTED_EDGE('',*,*,#34541,.F.);
#46244=ORIENTED_EDGE('',*,*,#34542,.T.);
#46245=ORIENTED_EDGE('',*,*,#34543,.T.);
#46246=ORIENTED_EDGE('',*,*,#34539,.F.);
#46247=ORIENTED_EDGE('',*,*,#34544,.F.);
#46248=ORIENTED_EDGE('',*,*,#34537,.T.);
#46249=ORIENTED_EDGE('',*,*,#34545,.T.);
#46250=ORIENTED_EDGE('',*,*,#34542,.F.);
#46251=ORIENTED_EDGE('',*,*,#34545,.F.);
#46252=ORIENTED_EDGE('',*,*,#34536,.F.);
#46253=ORIENTED_EDGE('',*,*,#34540,.F.);
#46254=ORIENTED_EDGE('',*,*,#34543,.F.);
#46255=ORIENTED_EDGE('',*,*,#34546,.F.);
#46256=ORIENTED_EDGE('',*,*,#34547,.T.);
#46257=ORIENTED_EDGE('',*,*,#34548,.T.);
#46258=ORIENTED_EDGE('',*,*,#34549,.F.);
#46259=ORIENTED_EDGE('',*,*,#34550,.F.);
#46260=ORIENTED_EDGE('',*,*,#34551,.T.);
#46261=ORIENTED_EDGE('',*,*,#34552,.T.);
#46262=ORIENTED_EDGE('',*,*,#34547,.F.);
#46263=ORIENTED_EDGE('',*,*,#34553,.F.);
#46264=ORIENTED_EDGE('',*,*,#34554,.T.);
#46265=ORIENTED_EDGE('',*,*,#34555,.T.);
#46266=ORIENTED_EDGE('',*,*,#34551,.F.);
#46267=ORIENTED_EDGE('',*,*,#34556,.F.);
#46268=ORIENTED_EDGE('',*,*,#34549,.T.);
#46269=ORIENTED_EDGE('',*,*,#34557,.T.);
#46270=ORIENTED_EDGE('',*,*,#34554,.F.);
#46271=ORIENTED_EDGE('',*,*,#34557,.F.);
#46272=ORIENTED_EDGE('',*,*,#34548,.F.);
#46273=ORIENTED_EDGE('',*,*,#34552,.F.);
#46274=ORIENTED_EDGE('',*,*,#34555,.F.);
#46275=ORIENTED_EDGE('',*,*,#34558,.F.);
#46276=ORIENTED_EDGE('',*,*,#34559,.T.);
#46277=ORIENTED_EDGE('',*,*,#34560,.T.);
#46278=ORIENTED_EDGE('',*,*,#34561,.F.);
#46279=ORIENTED_EDGE('',*,*,#34562,.F.);
#46280=ORIENTED_EDGE('',*,*,#34563,.T.);
#46281=ORIENTED_EDGE('',*,*,#34564,.T.);
#46282=ORIENTED_EDGE('',*,*,#34559,.F.);
#46283=ORIENTED_EDGE('',*,*,#34565,.F.);
#46284=ORIENTED_EDGE('',*,*,#34566,.T.);
#46285=ORIENTED_EDGE('',*,*,#34567,.T.);
#46286=ORIENTED_EDGE('',*,*,#34563,.F.);
#46287=ORIENTED_EDGE('',*,*,#34568,.F.);
#46288=ORIENTED_EDGE('',*,*,#34561,.T.);
#46289=ORIENTED_EDGE('',*,*,#34569,.T.);
#46290=ORIENTED_EDGE('',*,*,#34566,.F.);
#46291=ORIENTED_EDGE('',*,*,#34569,.F.);
#46292=ORIENTED_EDGE('',*,*,#34560,.F.);
#46293=ORIENTED_EDGE('',*,*,#34564,.F.);
#46294=ORIENTED_EDGE('',*,*,#34567,.F.);
#46295=ORIENTED_EDGE('',*,*,#34570,.F.);
#46296=ORIENTED_EDGE('',*,*,#34571,.T.);
#46297=ORIENTED_EDGE('',*,*,#34572,.T.);
#46298=ORIENTED_EDGE('',*,*,#34573,.F.);
#46299=ORIENTED_EDGE('',*,*,#34574,.F.);
#46300=ORIENTED_EDGE('',*,*,#34575,.T.);
#46301=ORIENTED_EDGE('',*,*,#34576,.T.);
#46302=ORIENTED_EDGE('',*,*,#34571,.F.);
#46303=ORIENTED_EDGE('',*,*,#34577,.F.);
#46304=ORIENTED_EDGE('',*,*,#34578,.T.);
#46305=ORIENTED_EDGE('',*,*,#34579,.T.);
#46306=ORIENTED_EDGE('',*,*,#34575,.F.);
#46307=ORIENTED_EDGE('',*,*,#34580,.F.);
#46308=ORIENTED_EDGE('',*,*,#34573,.T.);
#46309=ORIENTED_EDGE('',*,*,#34581,.T.);
#46310=ORIENTED_EDGE('',*,*,#34578,.F.);
#46311=ORIENTED_EDGE('',*,*,#34581,.F.);
#46312=ORIENTED_EDGE('',*,*,#34572,.F.);
#46313=ORIENTED_EDGE('',*,*,#34576,.F.);
#46314=ORIENTED_EDGE('',*,*,#34579,.F.);
#46315=ORIENTED_EDGE('',*,*,#34582,.F.);
#46316=ORIENTED_EDGE('',*,*,#34583,.T.);
#46317=ORIENTED_EDGE('',*,*,#34584,.T.);
#46318=ORIENTED_EDGE('',*,*,#34585,.F.);
#46319=ORIENTED_EDGE('',*,*,#34586,.F.);
#46320=ORIENTED_EDGE('',*,*,#34587,.T.);
#46321=ORIENTED_EDGE('',*,*,#34588,.T.);
#46322=ORIENTED_EDGE('',*,*,#34583,.F.);
#46323=ORIENTED_EDGE('',*,*,#34589,.F.);
#46324=ORIENTED_EDGE('',*,*,#34590,.T.);
#46325=ORIENTED_EDGE('',*,*,#34591,.T.);
#46326=ORIENTED_EDGE('',*,*,#34587,.F.);
#46327=ORIENTED_EDGE('',*,*,#34592,.F.);
#46328=ORIENTED_EDGE('',*,*,#34585,.T.);
#46329=ORIENTED_EDGE('',*,*,#34593,.T.);
#46330=ORIENTED_EDGE('',*,*,#34590,.F.);
#46331=ORIENTED_EDGE('',*,*,#34593,.F.);
#46332=ORIENTED_EDGE('',*,*,#34584,.F.);
#46333=ORIENTED_EDGE('',*,*,#34588,.F.);
#46334=ORIENTED_EDGE('',*,*,#34591,.F.);
#46335=ORIENTED_EDGE('',*,*,#34594,.F.);
#46336=ORIENTED_EDGE('',*,*,#34595,.T.);
#46337=ORIENTED_EDGE('',*,*,#34596,.T.);
#46338=ORIENTED_EDGE('',*,*,#34597,.F.);
#46339=ORIENTED_EDGE('',*,*,#34598,.F.);
#46340=ORIENTED_EDGE('',*,*,#34599,.T.);
#46341=ORIENTED_EDGE('',*,*,#34600,.T.);
#46342=ORIENTED_EDGE('',*,*,#34595,.F.);
#46343=ORIENTED_EDGE('',*,*,#34601,.F.);
#46344=ORIENTED_EDGE('',*,*,#34602,.T.);
#46345=ORIENTED_EDGE('',*,*,#34603,.T.);
#46346=ORIENTED_EDGE('',*,*,#34599,.F.);
#46347=ORIENTED_EDGE('',*,*,#34604,.F.);
#46348=ORIENTED_EDGE('',*,*,#34597,.T.);
#46349=ORIENTED_EDGE('',*,*,#34605,.T.);
#46350=ORIENTED_EDGE('',*,*,#34602,.F.);
#46351=ORIENTED_EDGE('',*,*,#34605,.F.);
#46352=ORIENTED_EDGE('',*,*,#34596,.F.);
#46353=ORIENTED_EDGE('',*,*,#34600,.F.);
#46354=ORIENTED_EDGE('',*,*,#34603,.F.);
#46355=ORIENTED_EDGE('',*,*,#34606,.F.);
#46356=ORIENTED_EDGE('',*,*,#34607,.T.);
#46357=ORIENTED_EDGE('',*,*,#34608,.T.);
#46358=ORIENTED_EDGE('',*,*,#34609,.F.);
#46359=ORIENTED_EDGE('',*,*,#34610,.F.);
#46360=ORIENTED_EDGE('',*,*,#34611,.T.);
#46361=ORIENTED_EDGE('',*,*,#34612,.T.);
#46362=ORIENTED_EDGE('',*,*,#34607,.F.);
#46363=ORIENTED_EDGE('',*,*,#34613,.F.);
#46364=ORIENTED_EDGE('',*,*,#34614,.T.);
#46365=ORIENTED_EDGE('',*,*,#34615,.T.);
#46366=ORIENTED_EDGE('',*,*,#34611,.F.);
#46367=ORIENTED_EDGE('',*,*,#34616,.F.);
#46368=ORIENTED_EDGE('',*,*,#34609,.T.);
#46369=ORIENTED_EDGE('',*,*,#34617,.T.);
#46370=ORIENTED_EDGE('',*,*,#34614,.F.);
#46371=ORIENTED_EDGE('',*,*,#34617,.F.);
#46372=ORIENTED_EDGE('',*,*,#34608,.F.);
#46373=ORIENTED_EDGE('',*,*,#34612,.F.);
#46374=ORIENTED_EDGE('',*,*,#34615,.F.);
#46375=ORIENTED_EDGE('',*,*,#34618,.F.);
#46376=ORIENTED_EDGE('',*,*,#34619,.T.);
#46377=ORIENTED_EDGE('',*,*,#34620,.T.);
#46378=ORIENTED_EDGE('',*,*,#34621,.F.);
#46379=ORIENTED_EDGE('',*,*,#34622,.F.);
#46380=ORIENTED_EDGE('',*,*,#34623,.T.);
#46381=ORIENTED_EDGE('',*,*,#34624,.T.);
#46382=ORIENTED_EDGE('',*,*,#34619,.F.);
#46383=ORIENTED_EDGE('',*,*,#34625,.F.);
#46384=ORIENTED_EDGE('',*,*,#34626,.T.);
#46385=ORIENTED_EDGE('',*,*,#34627,.T.);
#46386=ORIENTED_EDGE('',*,*,#34623,.F.);
#46387=ORIENTED_EDGE('',*,*,#34628,.F.);
#46388=ORIENTED_EDGE('',*,*,#34621,.T.);
#46389=ORIENTED_EDGE('',*,*,#34629,.T.);
#46390=ORIENTED_EDGE('',*,*,#34626,.F.);
#46391=ORIENTED_EDGE('',*,*,#34629,.F.);
#46392=ORIENTED_EDGE('',*,*,#34620,.F.);
#46393=ORIENTED_EDGE('',*,*,#34624,.F.);
#46394=ORIENTED_EDGE('',*,*,#34627,.F.);
#46395=ORIENTED_EDGE('',*,*,#34630,.F.);
#46396=ORIENTED_EDGE('',*,*,#34631,.T.);
#46397=ORIENTED_EDGE('',*,*,#34632,.T.);
#46398=ORIENTED_EDGE('',*,*,#34633,.F.);
#46399=ORIENTED_EDGE('',*,*,#34634,.F.);
#46400=ORIENTED_EDGE('',*,*,#34635,.T.);
#46401=ORIENTED_EDGE('',*,*,#34636,.T.);
#46402=ORIENTED_EDGE('',*,*,#34631,.F.);
#46403=ORIENTED_EDGE('',*,*,#34637,.F.);
#46404=ORIENTED_EDGE('',*,*,#34638,.T.);
#46405=ORIENTED_EDGE('',*,*,#34639,.T.);
#46406=ORIENTED_EDGE('',*,*,#34635,.F.);
#46407=ORIENTED_EDGE('',*,*,#34640,.F.);
#46408=ORIENTED_EDGE('',*,*,#34633,.T.);
#46409=ORIENTED_EDGE('',*,*,#34641,.T.);
#46410=ORIENTED_EDGE('',*,*,#34638,.F.);
#46411=ORIENTED_EDGE('',*,*,#34641,.F.);
#46412=ORIENTED_EDGE('',*,*,#34632,.F.);
#46413=ORIENTED_EDGE('',*,*,#34636,.F.);
#46414=ORIENTED_EDGE('',*,*,#34639,.F.);
#46415=ORIENTED_EDGE('',*,*,#34642,.F.);
#46416=ORIENTED_EDGE('',*,*,#34643,.T.);
#46417=ORIENTED_EDGE('',*,*,#34644,.T.);
#46418=ORIENTED_EDGE('',*,*,#34645,.F.);
#46419=ORIENTED_EDGE('',*,*,#34646,.F.);
#46420=ORIENTED_EDGE('',*,*,#34647,.T.);
#46421=ORIENTED_EDGE('',*,*,#34648,.T.);
#46422=ORIENTED_EDGE('',*,*,#34643,.F.);
#46423=ORIENTED_EDGE('',*,*,#34649,.F.);
#46424=ORIENTED_EDGE('',*,*,#34650,.T.);
#46425=ORIENTED_EDGE('',*,*,#34651,.T.);
#46426=ORIENTED_EDGE('',*,*,#34647,.F.);
#46427=ORIENTED_EDGE('',*,*,#34652,.F.);
#46428=ORIENTED_EDGE('',*,*,#34645,.T.);
#46429=ORIENTED_EDGE('',*,*,#34653,.T.);
#46430=ORIENTED_EDGE('',*,*,#34650,.F.);
#46431=ORIENTED_EDGE('',*,*,#34653,.F.);
#46432=ORIENTED_EDGE('',*,*,#34644,.F.);
#46433=ORIENTED_EDGE('',*,*,#34648,.F.);
#46434=ORIENTED_EDGE('',*,*,#34651,.F.);
#46435=ORIENTED_EDGE('',*,*,#34654,.F.);
#46436=ORIENTED_EDGE('',*,*,#34655,.T.);
#46437=ORIENTED_EDGE('',*,*,#34656,.T.);
#46438=ORIENTED_EDGE('',*,*,#34657,.F.);
#46439=ORIENTED_EDGE('',*,*,#34658,.F.);
#46440=ORIENTED_EDGE('',*,*,#34659,.T.);
#46441=ORIENTED_EDGE('',*,*,#34660,.T.);
#46442=ORIENTED_EDGE('',*,*,#34655,.F.);
#46443=ORIENTED_EDGE('',*,*,#34661,.F.);
#46444=ORIENTED_EDGE('',*,*,#34662,.T.);
#46445=ORIENTED_EDGE('',*,*,#34663,.T.);
#46446=ORIENTED_EDGE('',*,*,#34659,.F.);
#46447=ORIENTED_EDGE('',*,*,#34664,.F.);
#46448=ORIENTED_EDGE('',*,*,#34657,.T.);
#46449=ORIENTED_EDGE('',*,*,#34665,.T.);
#46450=ORIENTED_EDGE('',*,*,#34662,.F.);
#46451=ORIENTED_EDGE('',*,*,#34665,.F.);
#46452=ORIENTED_EDGE('',*,*,#34656,.F.);
#46453=ORIENTED_EDGE('',*,*,#34660,.F.);
#46454=ORIENTED_EDGE('',*,*,#34663,.F.);
#46455=ORIENTED_EDGE('',*,*,#34666,.F.);
#46456=ORIENTED_EDGE('',*,*,#34667,.T.);
#46457=ORIENTED_EDGE('',*,*,#34668,.T.);
#46458=ORIENTED_EDGE('',*,*,#34669,.F.);
#46459=ORIENTED_EDGE('',*,*,#34670,.F.);
#46460=ORIENTED_EDGE('',*,*,#34671,.T.);
#46461=ORIENTED_EDGE('',*,*,#34672,.T.);
#46462=ORIENTED_EDGE('',*,*,#34667,.F.);
#46463=ORIENTED_EDGE('',*,*,#34673,.F.);
#46464=ORIENTED_EDGE('',*,*,#34674,.T.);
#46465=ORIENTED_EDGE('',*,*,#34675,.T.);
#46466=ORIENTED_EDGE('',*,*,#34671,.F.);
#46467=ORIENTED_EDGE('',*,*,#34676,.F.);
#46468=ORIENTED_EDGE('',*,*,#34669,.T.);
#46469=ORIENTED_EDGE('',*,*,#34677,.T.);
#46470=ORIENTED_EDGE('',*,*,#34674,.F.);
#46471=ORIENTED_EDGE('',*,*,#34677,.F.);
#46472=ORIENTED_EDGE('',*,*,#34668,.F.);
#46473=ORIENTED_EDGE('',*,*,#34672,.F.);
#46474=ORIENTED_EDGE('',*,*,#34675,.F.);
#46475=ORIENTED_EDGE('',*,*,#34678,.F.);
#46476=ORIENTED_EDGE('',*,*,#34679,.T.);
#46477=ORIENTED_EDGE('',*,*,#34680,.T.);
#46478=ORIENTED_EDGE('',*,*,#34681,.F.);
#46479=ORIENTED_EDGE('',*,*,#34682,.F.);
#46480=ORIENTED_EDGE('',*,*,#34683,.T.);
#46481=ORIENTED_EDGE('',*,*,#34684,.T.);
#46482=ORIENTED_EDGE('',*,*,#34679,.F.);
#46483=ORIENTED_EDGE('',*,*,#34685,.F.);
#46484=ORIENTED_EDGE('',*,*,#34686,.T.);
#46485=ORIENTED_EDGE('',*,*,#34687,.T.);
#46486=ORIENTED_EDGE('',*,*,#34683,.F.);
#46487=ORIENTED_EDGE('',*,*,#34688,.F.);
#46488=ORIENTED_EDGE('',*,*,#34681,.T.);
#46489=ORIENTED_EDGE('',*,*,#34689,.T.);
#46490=ORIENTED_EDGE('',*,*,#34686,.F.);
#46491=ORIENTED_EDGE('',*,*,#34689,.F.);
#46492=ORIENTED_EDGE('',*,*,#34680,.F.);
#46493=ORIENTED_EDGE('',*,*,#34684,.F.);
#46494=ORIENTED_EDGE('',*,*,#34687,.F.);
#46495=ORIENTED_EDGE('',*,*,#34690,.F.);
#46496=ORIENTED_EDGE('',*,*,#34691,.T.);
#46497=ORIENTED_EDGE('',*,*,#34692,.T.);
#46498=ORIENTED_EDGE('',*,*,#34693,.F.);
#46499=ORIENTED_EDGE('',*,*,#34694,.F.);
#46500=ORIENTED_EDGE('',*,*,#34695,.T.);
#46501=ORIENTED_EDGE('',*,*,#34696,.T.);
#46502=ORIENTED_EDGE('',*,*,#34691,.F.);
#46503=ORIENTED_EDGE('',*,*,#34697,.F.);
#46504=ORIENTED_EDGE('',*,*,#34698,.T.);
#46505=ORIENTED_EDGE('',*,*,#34699,.T.);
#46506=ORIENTED_EDGE('',*,*,#34695,.F.);
#46507=ORIENTED_EDGE('',*,*,#34700,.F.);
#46508=ORIENTED_EDGE('',*,*,#34693,.T.);
#46509=ORIENTED_EDGE('',*,*,#34701,.T.);
#46510=ORIENTED_EDGE('',*,*,#34698,.F.);
#46511=ORIENTED_EDGE('',*,*,#34701,.F.);
#46512=ORIENTED_EDGE('',*,*,#34692,.F.);
#46513=ORIENTED_EDGE('',*,*,#34696,.F.);
#46514=ORIENTED_EDGE('',*,*,#34699,.F.);
#46515=ORIENTED_EDGE('',*,*,#34702,.F.);
#46516=ORIENTED_EDGE('',*,*,#34703,.T.);
#46517=ORIENTED_EDGE('',*,*,#34704,.T.);
#46518=ORIENTED_EDGE('',*,*,#34705,.F.);
#46519=ORIENTED_EDGE('',*,*,#34706,.F.);
#46520=ORIENTED_EDGE('',*,*,#34707,.T.);
#46521=ORIENTED_EDGE('',*,*,#34708,.T.);
#46522=ORIENTED_EDGE('',*,*,#34703,.F.);
#46523=ORIENTED_EDGE('',*,*,#34709,.F.);
#46524=ORIENTED_EDGE('',*,*,#34710,.T.);
#46525=ORIENTED_EDGE('',*,*,#34711,.T.);
#46526=ORIENTED_EDGE('',*,*,#34707,.F.);
#46527=ORIENTED_EDGE('',*,*,#34712,.F.);
#46528=ORIENTED_EDGE('',*,*,#34705,.T.);
#46529=ORIENTED_EDGE('',*,*,#34713,.T.);
#46530=ORIENTED_EDGE('',*,*,#34710,.F.);
#46531=ORIENTED_EDGE('',*,*,#34713,.F.);
#46532=ORIENTED_EDGE('',*,*,#34704,.F.);
#46533=ORIENTED_EDGE('',*,*,#34708,.F.);
#46534=ORIENTED_EDGE('',*,*,#34711,.F.);
#46535=ORIENTED_EDGE('',*,*,#34714,.F.);
#46536=ORIENTED_EDGE('',*,*,#34715,.T.);
#46537=ORIENTED_EDGE('',*,*,#34716,.T.);
#46538=ORIENTED_EDGE('',*,*,#34717,.F.);
#46539=ORIENTED_EDGE('',*,*,#34718,.F.);
#46540=ORIENTED_EDGE('',*,*,#34719,.T.);
#46541=ORIENTED_EDGE('',*,*,#34720,.T.);
#46542=ORIENTED_EDGE('',*,*,#34715,.F.);
#46543=ORIENTED_EDGE('',*,*,#34721,.F.);
#46544=ORIENTED_EDGE('',*,*,#34722,.T.);
#46545=ORIENTED_EDGE('',*,*,#34723,.T.);
#46546=ORIENTED_EDGE('',*,*,#34719,.F.);
#46547=ORIENTED_EDGE('',*,*,#34724,.F.);
#46548=ORIENTED_EDGE('',*,*,#34717,.T.);
#46549=ORIENTED_EDGE('',*,*,#34725,.T.);
#46550=ORIENTED_EDGE('',*,*,#34722,.F.);
#46551=ORIENTED_EDGE('',*,*,#34725,.F.);
#46552=ORIENTED_EDGE('',*,*,#34716,.F.);
#46553=ORIENTED_EDGE('',*,*,#34720,.F.);
#46554=ORIENTED_EDGE('',*,*,#34723,.F.);
#46555=ORIENTED_EDGE('',*,*,#34726,.F.);
#46556=ORIENTED_EDGE('',*,*,#34727,.T.);
#46557=ORIENTED_EDGE('',*,*,#34728,.T.);
#46558=ORIENTED_EDGE('',*,*,#34729,.F.);
#46559=ORIENTED_EDGE('',*,*,#34730,.F.);
#46560=ORIENTED_EDGE('',*,*,#34731,.T.);
#46561=ORIENTED_EDGE('',*,*,#34732,.T.);
#46562=ORIENTED_EDGE('',*,*,#34727,.F.);
#46563=ORIENTED_EDGE('',*,*,#34733,.F.);
#46564=ORIENTED_EDGE('',*,*,#34734,.T.);
#46565=ORIENTED_EDGE('',*,*,#34735,.T.);
#46566=ORIENTED_EDGE('',*,*,#34731,.F.);
#46567=ORIENTED_EDGE('',*,*,#34736,.F.);
#46568=ORIENTED_EDGE('',*,*,#34729,.T.);
#46569=ORIENTED_EDGE('',*,*,#34737,.T.);
#46570=ORIENTED_EDGE('',*,*,#34734,.F.);
#46571=ORIENTED_EDGE('',*,*,#34737,.F.);
#46572=ORIENTED_EDGE('',*,*,#34728,.F.);
#46573=ORIENTED_EDGE('',*,*,#34732,.F.);
#46574=ORIENTED_EDGE('',*,*,#34735,.F.);
#46575=ORIENTED_EDGE('',*,*,#34738,.F.);
#46576=ORIENTED_EDGE('',*,*,#34739,.T.);
#46577=ORIENTED_EDGE('',*,*,#34740,.T.);
#46578=ORIENTED_EDGE('',*,*,#34741,.F.);
#46579=ORIENTED_EDGE('',*,*,#34742,.F.);
#46580=ORIENTED_EDGE('',*,*,#34743,.T.);
#46581=ORIENTED_EDGE('',*,*,#34744,.T.);
#46582=ORIENTED_EDGE('',*,*,#34739,.F.);
#46583=ORIENTED_EDGE('',*,*,#34745,.F.);
#46584=ORIENTED_EDGE('',*,*,#34746,.T.);
#46585=ORIENTED_EDGE('',*,*,#34747,.T.);
#46586=ORIENTED_EDGE('',*,*,#34743,.F.);
#46587=ORIENTED_EDGE('',*,*,#34748,.F.);
#46588=ORIENTED_EDGE('',*,*,#34741,.T.);
#46589=ORIENTED_EDGE('',*,*,#34749,.T.);
#46590=ORIENTED_EDGE('',*,*,#34746,.F.);
#46591=ORIENTED_EDGE('',*,*,#34749,.F.);
#46592=ORIENTED_EDGE('',*,*,#34740,.F.);
#46593=ORIENTED_EDGE('',*,*,#34744,.F.);
#46594=ORIENTED_EDGE('',*,*,#34747,.F.);
#46595=ORIENTED_EDGE('',*,*,#34750,.F.);
#46596=ORIENTED_EDGE('',*,*,#34751,.T.);
#46597=ORIENTED_EDGE('',*,*,#34752,.T.);
#46598=ORIENTED_EDGE('',*,*,#34753,.F.);
#46599=ORIENTED_EDGE('',*,*,#34754,.F.);
#46600=ORIENTED_EDGE('',*,*,#34755,.T.);
#46601=ORIENTED_EDGE('',*,*,#34756,.T.);
#46602=ORIENTED_EDGE('',*,*,#34751,.F.);
#46603=ORIENTED_EDGE('',*,*,#34757,.F.);
#46604=ORIENTED_EDGE('',*,*,#34758,.T.);
#46605=ORIENTED_EDGE('',*,*,#34759,.T.);
#46606=ORIENTED_EDGE('',*,*,#34755,.F.);
#46607=ORIENTED_EDGE('',*,*,#34760,.F.);
#46608=ORIENTED_EDGE('',*,*,#34753,.T.);
#46609=ORIENTED_EDGE('',*,*,#34761,.T.);
#46610=ORIENTED_EDGE('',*,*,#34758,.F.);
#46611=ORIENTED_EDGE('',*,*,#34761,.F.);
#46612=ORIENTED_EDGE('',*,*,#34752,.F.);
#46613=ORIENTED_EDGE('',*,*,#34756,.F.);
#46614=ORIENTED_EDGE('',*,*,#34759,.F.);
#46615=ORIENTED_EDGE('',*,*,#34762,.F.);
#46616=ORIENTED_EDGE('',*,*,#34763,.T.);
#46617=ORIENTED_EDGE('',*,*,#34764,.T.);
#46618=ORIENTED_EDGE('',*,*,#34765,.F.);
#46619=ORIENTED_EDGE('',*,*,#34766,.F.);
#46620=ORIENTED_EDGE('',*,*,#34767,.T.);
#46621=ORIENTED_EDGE('',*,*,#34768,.T.);
#46622=ORIENTED_EDGE('',*,*,#34763,.F.);
#46623=ORIENTED_EDGE('',*,*,#34769,.F.);
#46624=ORIENTED_EDGE('',*,*,#34770,.T.);
#46625=ORIENTED_EDGE('',*,*,#34771,.T.);
#46626=ORIENTED_EDGE('',*,*,#34767,.F.);
#46627=ORIENTED_EDGE('',*,*,#34772,.F.);
#46628=ORIENTED_EDGE('',*,*,#34765,.T.);
#46629=ORIENTED_EDGE('',*,*,#34773,.T.);
#46630=ORIENTED_EDGE('',*,*,#34770,.F.);
#46631=ORIENTED_EDGE('',*,*,#34773,.F.);
#46632=ORIENTED_EDGE('',*,*,#34764,.F.);
#46633=ORIENTED_EDGE('',*,*,#34768,.F.);
#46634=ORIENTED_EDGE('',*,*,#34771,.F.);
#46635=ORIENTED_EDGE('',*,*,#34774,.F.);
#46636=ORIENTED_EDGE('',*,*,#34775,.T.);
#46637=ORIENTED_EDGE('',*,*,#34776,.T.);
#46638=ORIENTED_EDGE('',*,*,#34777,.F.);
#46639=ORIENTED_EDGE('',*,*,#34778,.F.);
#46640=ORIENTED_EDGE('',*,*,#34779,.T.);
#46641=ORIENTED_EDGE('',*,*,#34780,.T.);
#46642=ORIENTED_EDGE('',*,*,#34775,.F.);
#46643=ORIENTED_EDGE('',*,*,#34781,.F.);
#46644=ORIENTED_EDGE('',*,*,#34782,.T.);
#46645=ORIENTED_EDGE('',*,*,#34783,.T.);
#46646=ORIENTED_EDGE('',*,*,#34779,.F.);
#46647=ORIENTED_EDGE('',*,*,#34784,.F.);
#46648=ORIENTED_EDGE('',*,*,#34777,.T.);
#46649=ORIENTED_EDGE('',*,*,#34785,.T.);
#46650=ORIENTED_EDGE('',*,*,#34782,.F.);
#46651=ORIENTED_EDGE('',*,*,#34785,.F.);
#46652=ORIENTED_EDGE('',*,*,#34776,.F.);
#46653=ORIENTED_EDGE('',*,*,#34780,.F.);
#46654=ORIENTED_EDGE('',*,*,#34783,.F.);
#46655=ORIENTED_EDGE('',*,*,#34786,.F.);
#46656=ORIENTED_EDGE('',*,*,#34787,.T.);
#46657=ORIENTED_EDGE('',*,*,#34788,.T.);
#46658=ORIENTED_EDGE('',*,*,#34789,.F.);
#46659=ORIENTED_EDGE('',*,*,#34790,.F.);
#46660=ORIENTED_EDGE('',*,*,#34791,.T.);
#46661=ORIENTED_EDGE('',*,*,#34792,.T.);
#46662=ORIENTED_EDGE('',*,*,#34787,.F.);
#46663=ORIENTED_EDGE('',*,*,#34793,.F.);
#46664=ORIENTED_EDGE('',*,*,#34794,.T.);
#46665=ORIENTED_EDGE('',*,*,#34795,.T.);
#46666=ORIENTED_EDGE('',*,*,#34791,.F.);
#46667=ORIENTED_EDGE('',*,*,#34796,.F.);
#46668=ORIENTED_EDGE('',*,*,#34789,.T.);
#46669=ORIENTED_EDGE('',*,*,#34797,.T.);
#46670=ORIENTED_EDGE('',*,*,#34794,.F.);
#46671=ORIENTED_EDGE('',*,*,#34797,.F.);
#46672=ORIENTED_EDGE('',*,*,#34788,.F.);
#46673=ORIENTED_EDGE('',*,*,#34792,.F.);
#46674=ORIENTED_EDGE('',*,*,#34795,.F.);
#46675=ORIENTED_EDGE('',*,*,#34798,.F.);
#46676=ORIENTED_EDGE('',*,*,#34799,.T.);
#46677=ORIENTED_EDGE('',*,*,#34800,.T.);
#46678=ORIENTED_EDGE('',*,*,#34801,.F.);
#46679=ORIENTED_EDGE('',*,*,#34802,.F.);
#46680=ORIENTED_EDGE('',*,*,#34803,.T.);
#46681=ORIENTED_EDGE('',*,*,#34804,.T.);
#46682=ORIENTED_EDGE('',*,*,#34799,.F.);
#46683=ORIENTED_EDGE('',*,*,#34805,.F.);
#46684=ORIENTED_EDGE('',*,*,#34806,.T.);
#46685=ORIENTED_EDGE('',*,*,#34807,.T.);
#46686=ORIENTED_EDGE('',*,*,#34803,.F.);
#46687=ORIENTED_EDGE('',*,*,#34808,.F.);
#46688=ORIENTED_EDGE('',*,*,#34801,.T.);
#46689=ORIENTED_EDGE('',*,*,#34809,.T.);
#46690=ORIENTED_EDGE('',*,*,#34806,.F.);
#46691=ORIENTED_EDGE('',*,*,#34809,.F.);
#46692=ORIENTED_EDGE('',*,*,#34800,.F.);
#46693=ORIENTED_EDGE('',*,*,#34804,.F.);
#46694=ORIENTED_EDGE('',*,*,#34807,.F.);
#46695=ORIENTED_EDGE('',*,*,#34810,.F.);
#46696=ORIENTED_EDGE('',*,*,#34811,.T.);
#46697=ORIENTED_EDGE('',*,*,#34812,.T.);
#46698=ORIENTED_EDGE('',*,*,#34813,.F.);
#46699=ORIENTED_EDGE('',*,*,#34814,.F.);
#46700=ORIENTED_EDGE('',*,*,#34815,.T.);
#46701=ORIENTED_EDGE('',*,*,#34816,.T.);
#46702=ORIENTED_EDGE('',*,*,#34811,.F.);
#46703=ORIENTED_EDGE('',*,*,#34817,.F.);
#46704=ORIENTED_EDGE('',*,*,#34818,.T.);
#46705=ORIENTED_EDGE('',*,*,#34819,.T.);
#46706=ORIENTED_EDGE('',*,*,#34815,.F.);
#46707=ORIENTED_EDGE('',*,*,#34820,.F.);
#46708=ORIENTED_EDGE('',*,*,#34813,.T.);
#46709=ORIENTED_EDGE('',*,*,#34821,.T.);
#46710=ORIENTED_EDGE('',*,*,#34818,.F.);
#46711=ORIENTED_EDGE('',*,*,#34821,.F.);
#46712=ORIENTED_EDGE('',*,*,#34812,.F.);
#46713=ORIENTED_EDGE('',*,*,#34816,.F.);
#46714=ORIENTED_EDGE('',*,*,#34819,.F.);
#46715=ORIENTED_EDGE('',*,*,#34822,.F.);
#46716=ORIENTED_EDGE('',*,*,#34823,.T.);
#46717=ORIENTED_EDGE('',*,*,#34824,.T.);
#46718=ORIENTED_EDGE('',*,*,#34825,.F.);
#46719=ORIENTED_EDGE('',*,*,#34826,.F.);
#46720=ORIENTED_EDGE('',*,*,#34827,.T.);
#46721=ORIENTED_EDGE('',*,*,#34828,.T.);
#46722=ORIENTED_EDGE('',*,*,#34823,.F.);
#46723=ORIENTED_EDGE('',*,*,#34829,.F.);
#46724=ORIENTED_EDGE('',*,*,#34830,.T.);
#46725=ORIENTED_EDGE('',*,*,#34831,.T.);
#46726=ORIENTED_EDGE('',*,*,#34827,.F.);
#46727=ORIENTED_EDGE('',*,*,#34832,.F.);
#46728=ORIENTED_EDGE('',*,*,#34825,.T.);
#46729=ORIENTED_EDGE('',*,*,#34833,.T.);
#46730=ORIENTED_EDGE('',*,*,#34830,.F.);
#46731=ORIENTED_EDGE('',*,*,#34833,.F.);
#46732=ORIENTED_EDGE('',*,*,#34824,.F.);
#46733=ORIENTED_EDGE('',*,*,#34828,.F.);
#46734=ORIENTED_EDGE('',*,*,#34831,.F.);
#46735=ORIENTED_EDGE('',*,*,#34834,.F.);
#46736=ORIENTED_EDGE('',*,*,#34835,.T.);
#46737=ORIENTED_EDGE('',*,*,#34836,.T.);
#46738=ORIENTED_EDGE('',*,*,#34837,.F.);
#46739=ORIENTED_EDGE('',*,*,#34838,.F.);
#46740=ORIENTED_EDGE('',*,*,#34839,.T.);
#46741=ORIENTED_EDGE('',*,*,#34840,.T.);
#46742=ORIENTED_EDGE('',*,*,#34835,.F.);
#46743=ORIENTED_EDGE('',*,*,#34841,.F.);
#46744=ORIENTED_EDGE('',*,*,#34842,.T.);
#46745=ORIENTED_EDGE('',*,*,#34843,.T.);
#46746=ORIENTED_EDGE('',*,*,#34839,.F.);
#46747=ORIENTED_EDGE('',*,*,#34844,.F.);
#46748=ORIENTED_EDGE('',*,*,#34837,.T.);
#46749=ORIENTED_EDGE('',*,*,#34845,.T.);
#46750=ORIENTED_EDGE('',*,*,#34842,.F.);
#46751=ORIENTED_EDGE('',*,*,#34845,.F.);
#46752=ORIENTED_EDGE('',*,*,#34836,.F.);
#46753=ORIENTED_EDGE('',*,*,#34840,.F.);
#46754=ORIENTED_EDGE('',*,*,#34843,.F.);
#46755=ORIENTED_EDGE('',*,*,#34846,.F.);
#46756=ORIENTED_EDGE('',*,*,#34847,.T.);
#46757=ORIENTED_EDGE('',*,*,#34848,.T.);
#46758=ORIENTED_EDGE('',*,*,#34849,.F.);
#46759=ORIENTED_EDGE('',*,*,#34850,.F.);
#46760=ORIENTED_EDGE('',*,*,#34851,.T.);
#46761=ORIENTED_EDGE('',*,*,#34852,.T.);
#46762=ORIENTED_EDGE('',*,*,#34847,.F.);
#46763=ORIENTED_EDGE('',*,*,#34853,.F.);
#46764=ORIENTED_EDGE('',*,*,#34854,.T.);
#46765=ORIENTED_EDGE('',*,*,#34855,.T.);
#46766=ORIENTED_EDGE('',*,*,#34851,.F.);
#46767=ORIENTED_EDGE('',*,*,#34856,.F.);
#46768=ORIENTED_EDGE('',*,*,#34849,.T.);
#46769=ORIENTED_EDGE('',*,*,#34857,.T.);
#46770=ORIENTED_EDGE('',*,*,#34854,.F.);
#46771=ORIENTED_EDGE('',*,*,#34857,.F.);
#46772=ORIENTED_EDGE('',*,*,#34848,.F.);
#46773=ORIENTED_EDGE('',*,*,#34852,.F.);
#46774=ORIENTED_EDGE('',*,*,#34855,.F.);
#46775=ORIENTED_EDGE('',*,*,#34858,.F.);
#46776=ORIENTED_EDGE('',*,*,#34859,.F.);
#46777=ORIENTED_EDGE('',*,*,#34860,.T.);
#46778=ORIENTED_EDGE('',*,*,#34861,.F.);
#46779=ORIENTED_EDGE('',*,*,#34862,.F.);
#46780=ORIENTED_EDGE('',*,*,#34863,.F.);
#46781=ORIENTED_EDGE('',*,*,#34864,.F.);
#46782=ORIENTED_EDGE('',*,*,#34865,.F.);
#46783=ORIENTED_EDGE('',*,*,#34866,.F.);
#46784=ORIENTED_EDGE('',*,*,#34867,.F.);
#46785=ORIENTED_EDGE('',*,*,#34868,.T.);
#46786=ORIENTED_EDGE('',*,*,#34869,.F.);
#46787=ORIENTED_EDGE('',*,*,#34868,.F.);
#46788=ORIENTED_EDGE('',*,*,#34870,.F.);
#46789=ORIENTED_EDGE('',*,*,#34860,.F.);
#46790=ORIENTED_EDGE('',*,*,#34871,.F.);
#46791=ORIENTED_EDGE('',*,*,#34861,.T.);
#46792=ORIENTED_EDGE('',*,*,#34870,.T.);
#46793=ORIENTED_EDGE('',*,*,#34867,.T.);
#46794=ORIENTED_EDGE('',*,*,#34872,.F.);
#46795=ORIENTED_EDGE('',*,*,#34873,.F.);
#46796=ORIENTED_EDGE('',*,*,#34874,.F.);
#46797=ORIENTED_EDGE('',*,*,#34875,.F.);
#46798=ORIENTED_EDGE('',*,*,#34876,.F.);
#46799=ORIENTED_EDGE('',*,*,#34877,.T.);
#46800=ORIENTED_EDGE('',*,*,#34878,.F.);
#46801=ORIENTED_EDGE('',*,*,#34879,.F.);
#46802=ORIENTED_EDGE('',*,*,#34880,.F.);
#46803=ORIENTED_EDGE('',*,*,#34881,.F.);
#46804=ORIENTED_EDGE('',*,*,#34882,.F.);
#46805=ORIENTED_EDGE('',*,*,#34883,.F.);
#46806=ORIENTED_EDGE('',*,*,#34884,.F.);
#46807=ORIENTED_EDGE('',*,*,#34885,.F.);
#46808=ORIENTED_EDGE('',*,*,#34886,.F.);
#46809=ORIENTED_EDGE('',*,*,#34887,.T.);
#46810=ORIENTED_EDGE('',*,*,#34888,.F.);
#46811=ORIENTED_EDGE('',*,*,#34889,.F.);
#46812=ORIENTED_EDGE('',*,*,#34890,.F.);
#46813=ORIENTED_EDGE('',*,*,#34891,.F.);
#46814=ORIENTED_EDGE('',*,*,#34892,.F.);
#46815=ORIENTED_EDGE('',*,*,#34864,.T.);
#46816=ORIENTED_EDGE('',*,*,#34893,.T.);
#46817=ORIENTED_EDGE('',*,*,#34894,.T.);
#46818=ORIENTED_EDGE('',*,*,#34895,.T.);
#46819=ORIENTED_EDGE('',*,*,#34858,.T.);
#46820=ORIENTED_EDGE('',*,*,#34896,.T.);
#46821=ORIENTED_EDGE('',*,*,#34897,.F.);
#46822=ORIENTED_EDGE('',*,*,#34898,.T.);
#46823=ORIENTED_EDGE('',*,*,#34866,.T.);
#46824=ORIENTED_EDGE('',*,*,#34899,.T.);
#46825=ORIENTED_EDGE('',*,*,#34900,.F.);
#46826=ORIENTED_EDGE('',*,*,#34872,.T.);
#46827=ORIENTED_EDGE('',*,*,#34865,.T.);
#46828=ORIENTED_EDGE('',*,*,#34895,.F.);
#46829=ORIENTED_EDGE('',*,*,#34901,.F.);
#46830=ORIENTED_EDGE('',*,*,#34899,.F.);
#46831=ORIENTED_EDGE('',*,*,#34902,.F.);
#46832=ORIENTED_EDGE('',*,*,#34903,.F.);
#46833=ORIENTED_EDGE('',*,*,#34904,.F.);
#46834=ORIENTED_EDGE('',*,*,#34905,.F.);
#46835=ORIENTED_EDGE('',*,*,#34906,.T.);
#46836=ORIENTED_EDGE('',*,*,#34906,.F.);
#46837=ORIENTED_EDGE('',*,*,#34907,.F.);
#46838=ORIENTED_EDGE('',*,*,#34908,.T.);
#46839=ORIENTED_EDGE('',*,*,#34908,.F.);
#46840=ORIENTED_EDGE('',*,*,#34909,.F.);
#46841=ORIENTED_EDGE('',*,*,#34910,.T.);
#46842=ORIENTED_EDGE('',*,*,#34907,.T.);
#46843=ORIENTED_EDGE('',*,*,#34910,.F.);
#46844=ORIENTED_EDGE('',*,*,#34911,.F.);
#46845=ORIENTED_EDGE('',*,*,#34912,.T.);
#46846=ORIENTED_EDGE('',*,*,#34905,.T.);
#46847=ORIENTED_EDGE('',*,*,#34912,.F.);
#46848=ORIENTED_EDGE('',*,*,#34913,.T.);
#46849=ORIENTED_EDGE('',*,*,#34914,.T.);
#46850=ORIENTED_EDGE('',*,*,#34915,.T.);
#46851=ORIENTED_EDGE('',*,*,#34914,.F.);
#46852=ORIENTED_EDGE('',*,*,#34915,.F.);
#46853=ORIENTED_EDGE('',*,*,#34916,.T.);
#46854=ORIENTED_EDGE('',*,*,#34917,.T.);
#46855=ORIENTED_EDGE('',*,*,#34916,.F.);
#46856=ORIENTED_EDGE('',*,*,#34918,.F.);
#46857=ORIENTED_EDGE('',*,*,#34919,.F.);
#46858=ORIENTED_EDGE('',*,*,#34920,.F.);
#46859=ORIENTED_EDGE('',*,*,#34921,.T.);
#46860=ORIENTED_EDGE('',*,*,#34922,.F.);
#46861=ORIENTED_EDGE('',*,*,#34913,.F.);
#46862=ORIENTED_EDGE('',*,*,#34917,.F.);
#46863=ORIENTED_EDGE('',*,*,#34923,.T.);
#46864=ORIENTED_EDGE('',*,*,#34923,.F.);
#46865=ORIENTED_EDGE('',*,*,#34922,.T.);
#46866=ORIENTED_EDGE('',*,*,#34924,.T.);
#46867=ORIENTED_EDGE('',*,*,#34925,.T.);
#46868=ORIENTED_EDGE('',*,*,#34924,.F.);
#46869=ORIENTED_EDGE('',*,*,#34925,.F.);
#46870=ORIENTED_EDGE('',*,*,#34926,.T.);
#46871=ORIENTED_EDGE('',*,*,#34927,.T.);
#46872=ORIENTED_EDGE('',*,*,#34926,.F.);
#46873=ORIENTED_EDGE('',*,*,#34927,.F.);
#46874=ORIENTED_EDGE('',*,*,#34928,.T.);
#46875=ORIENTED_EDGE('',*,*,#34928,.F.);
#46876=ORIENTED_EDGE('',*,*,#34929,.F.);
#46877=ORIENTED_EDGE('',*,*,#34930,.T.);
#46878=ORIENTED_EDGE('',*,*,#34931,.T.);
#46879=ORIENTED_EDGE('',*,*,#34930,.F.);
#46880=ORIENTED_EDGE('',*,*,#34931,.F.);
#46881=ORIENTED_EDGE('',*,*,#34932,.F.);
#46882=ORIENTED_EDGE('',*,*,#34933,.F.);
#46883=ORIENTED_EDGE('',*,*,#34934,.T.);
#46884=ORIENTED_EDGE('',*,*,#34935,.T.);
#46885=ORIENTED_EDGE('',*,*,#34934,.F.);
#46886=ORIENTED_EDGE('',*,*,#34935,.F.);
#46887=ORIENTED_EDGE('',*,*,#34936,.F.);
#46888=ORIENTED_EDGE('',*,*,#34937,.F.);
#46889=ORIENTED_EDGE('',*,*,#34938,.T.);
#46890=ORIENTED_EDGE('',*,*,#34939,.T.);
#46891=ORIENTED_EDGE('',*,*,#34938,.F.);
#46892=ORIENTED_EDGE('',*,*,#34939,.F.);
#46893=ORIENTED_EDGE('',*,*,#34940,.F.);
#46894=ORIENTED_EDGE('',*,*,#34941,.F.);
#46895=ORIENTED_EDGE('',*,*,#34942,.T.);
#46896=ORIENTED_EDGE('',*,*,#34943,.T.);
#46897=ORIENTED_EDGE('',*,*,#34942,.F.);
#46898=ORIENTED_EDGE('',*,*,#34943,.F.);
#46899=ORIENTED_EDGE('',*,*,#34944,.F.);
#46900=ORIENTED_EDGE('',*,*,#34945,.F.);
#46901=ORIENTED_EDGE('',*,*,#34946,.T.);
#46902=ORIENTED_EDGE('',*,*,#34947,.T.);
#46903=ORIENTED_EDGE('',*,*,#34946,.F.);
#46904=ORIENTED_EDGE('',*,*,#34947,.F.);
#46905=ORIENTED_EDGE('',*,*,#34948,.F.);
#46906=ORIENTED_EDGE('',*,*,#34949,.F.);
#46907=ORIENTED_EDGE('',*,*,#34950,.T.);
#46908=ORIENTED_EDGE('',*,*,#34951,.T.);
#46909=ORIENTED_EDGE('',*,*,#34950,.F.);
#46910=ORIENTED_EDGE('',*,*,#34951,.F.);
#46911=ORIENTED_EDGE('',*,*,#34952,.F.);
#46912=ORIENTED_EDGE('',*,*,#34904,.T.);
#46913=ORIENTED_EDGE('',*,*,#34953,.T.);
#46914=ORIENTED_EDGE('',*,*,#34954,.T.);
#46915=ORIENTED_EDGE('',*,*,#34953,.F.);
#46916=ORIENTED_EDGE('',*,*,#34863,.T.);
#46917=ORIENTED_EDGE('',*,*,#34955,.F.);
#46918=ORIENTED_EDGE('',*,*,#34956,.F.);
#46919=ORIENTED_EDGE('',*,*,#34896,.F.);
#46920=ORIENTED_EDGE('',*,*,#34957,.F.);
#46921=ORIENTED_EDGE('',*,*,#34958,.F.);
#46922=ORIENTED_EDGE('',*,*,#34959,.F.);
#46923=ORIENTED_EDGE('',*,*,#34954,.F.);
#46924=ORIENTED_EDGE('',*,*,#34960,.T.);
#46925=ORIENTED_EDGE('',*,*,#34952,.T.);
#46926=ORIENTED_EDGE('',*,*,#34960,.F.);
#46927=ORIENTED_EDGE('',*,*,#34902,.T.);
#46928=ORIENTED_EDGE('',*,*,#34961,.T.);
#46929=ORIENTED_EDGE('',*,*,#34962,.T.);
#46930=ORIENTED_EDGE('',*,*,#34961,.F.);
#46931=ORIENTED_EDGE('',*,*,#34962,.F.);
#46932=ORIENTED_EDGE('',*,*,#34963,.T.);
#46933=ORIENTED_EDGE('',*,*,#34948,.T.);
#46934=ORIENTED_EDGE('',*,*,#34963,.F.);
#46935=ORIENTED_EDGE('',*,*,#34959,.T.);
#46936=ORIENTED_EDGE('',*,*,#34964,.T.);
#46937=ORIENTED_EDGE('',*,*,#34965,.T.);
#46938=ORIENTED_EDGE('',*,*,#34964,.F.);
#46939=ORIENTED_EDGE('',*,*,#34965,.F.);
#46940=ORIENTED_EDGE('',*,*,#34966,.T.);
#46941=ORIENTED_EDGE('',*,*,#34944,.T.);
#46942=ORIENTED_EDGE('',*,*,#34966,.F.);
#46943=ORIENTED_EDGE('',*,*,#34903,.T.);
#46944=ORIENTED_EDGE('',*,*,#34967,.T.);
#46945=ORIENTED_EDGE('',*,*,#34968,.T.);
#46946=ORIENTED_EDGE('',*,*,#34967,.F.);
#46947=ORIENTED_EDGE('',*,*,#34968,.F.);
#46948=ORIENTED_EDGE('',*,*,#34969,.T.);
#46949=ORIENTED_EDGE('',*,*,#34940,.T.);
#46950=ORIENTED_EDGE('',*,*,#34969,.F.);
#46951=ORIENTED_EDGE('',*,*,#34958,.T.);
#46952=ORIENTED_EDGE('',*,*,#34970,.T.);
#46953=ORIENTED_EDGE('',*,*,#34971,.T.);
#46954=ORIENTED_EDGE('',*,*,#34970,.F.);
#46955=ORIENTED_EDGE('',*,*,#34971,.F.);
#46956=ORIENTED_EDGE('',*,*,#34972,.T.);
#46957=ORIENTED_EDGE('',*,*,#34936,.T.);
#46958=ORIENTED_EDGE('',*,*,#34972,.F.);
#46959=ORIENTED_EDGE('',*,*,#34957,.T.);
#46960=ORIENTED_EDGE('',*,*,#34973,.T.);
#46961=ORIENTED_EDGE('',*,*,#34974,.T.);
#46962=ORIENTED_EDGE('',*,*,#34973,.F.);
#46963=ORIENTED_EDGE('',*,*,#34974,.F.);
#46964=ORIENTED_EDGE('',*,*,#34975,.T.);
#46965=ORIENTED_EDGE('',*,*,#34932,.T.);
#46966=ORIENTED_EDGE('',*,*,#34975,.F.);
#46967=ORIENTED_EDGE('',*,*,#34976,.T.);
#46968=ORIENTED_EDGE('',*,*,#34977,.T.);
#46969=ORIENTED_EDGE('',*,*,#34978,.T.);
#46970=ORIENTED_EDGE('',*,*,#34979,.T.);
#46971=ORIENTED_EDGE('',*,*,#34980,.T.);
#46972=ORIENTED_EDGE('',*,*,#34981,.T.);
#46973=ORIENTED_EDGE('',*,*,#34982,.T.);
#46974=ORIENTED_EDGE('',*,*,#34979,.F.);
#46975=ORIENTED_EDGE('',*,*,#34983,.T.);
#46976=ORIENTED_EDGE('',*,*,#34984,.T.);
#46977=ORIENTED_EDGE('',*,*,#34985,.T.);
#46978=ORIENTED_EDGE('',*,*,#34981,.F.);
#46979=ORIENTED_EDGE('',*,*,#34986,.T.);
#46980=ORIENTED_EDGE('',*,*,#34987,.T.);
#46981=ORIENTED_EDGE('',*,*,#34988,.T.);
#46982=ORIENTED_EDGE('',*,*,#34989,.T.);
#46983=ORIENTED_EDGE('',*,*,#34990,.T.);
#46984=ORIENTED_EDGE('',*,*,#34991,.T.);
#46985=ORIENTED_EDGE('',*,*,#34992,.T.);
#46986=ORIENTED_EDGE('',*,*,#34987,.F.);
#46987=ORIENTED_EDGE('',*,*,#34993,.T.);
#46988=ORIENTED_EDGE('',*,*,#34994,.T.);
#46989=ORIENTED_EDGE('',*,*,#34995,.T.);
#46990=ORIENTED_EDGE('',*,*,#34991,.F.);
#46991=ORIENTED_EDGE('',*,*,#34996,.T.);
#46992=ORIENTED_EDGE('',*,*,#34997,.T.);
#46993=ORIENTED_EDGE('',*,*,#34998,.T.);
#46994=ORIENTED_EDGE('',*,*,#34994,.F.);
#46995=ORIENTED_EDGE('',*,*,#34999,.T.);
#46996=ORIENTED_EDGE('',*,*,#34989,.F.);
#46997=ORIENTED_EDGE('',*,*,#34918,.T.);
#46998=ORIENTED_EDGE('',*,*,#35000,.T.);
#46999=ORIENTED_EDGE('',*,*,#35001,.T.);
#47000=ORIENTED_EDGE('',*,*,#35000,.F.);
#47001=ORIENTED_EDGE('',*,*,#35002,.T.);
#47002=ORIENTED_EDGE('',*,*,#34984,.F.);
#47003=ORIENTED_EDGE('',*,*,#34977,.F.);
#47004=ORIENTED_EDGE('',*,*,#35003,.F.);
#47005=ORIENTED_EDGE('',*,*,#35004,.F.);
#47006=ORIENTED_EDGE('',*,*,#34877,.F.);
#47007=ORIENTED_EDGE('',*,*,#35005,.F.);
#47008=ORIENTED_EDGE('',*,*,#35006,.F.);
#47009=ORIENTED_EDGE('',*,*,#35007,.F.);
#47010=ORIENTED_EDGE('',*,*,#35008,.F.);
#47011=ORIENTED_EDGE('',*,*,#34976,.F.);
#47012=ORIENTED_EDGE('',*,*,#35009,.F.);
#47013=ORIENTED_EDGE('',*,*,#35010,.F.);
#47014=ORIENTED_EDGE('',*,*,#35003,.T.);
#47015=ORIENTED_EDGE('',*,*,#34982,.F.);
#47016=ORIENTED_EDGE('',*,*,#35011,.T.);
#47017=ORIENTED_EDGE('',*,*,#35012,.F.);
#47018=ORIENTED_EDGE('',*,*,#35009,.T.);
#47019=ORIENTED_EDGE('',*,*,#34985,.F.);
#47020=ORIENTED_EDGE('',*,*,#35013,.T.);
#47021=ORIENTED_EDGE('',*,*,#35014,.F.);
#47022=ORIENTED_EDGE('',*,*,#35011,.F.);
#47023=ORIENTED_EDGE('',*,*,#35002,.F.);
#47024=ORIENTED_EDGE('',*,*,#34921,.F.);
#47025=ORIENTED_EDGE('',*,*,#35015,.F.);
#47026=ORIENTED_EDGE('',*,*,#35013,.F.);
#47027=ORIENTED_EDGE('',*,*,#34988,.F.);
#47028=ORIENTED_EDGE('',*,*,#35016,.F.);
#47029=ORIENTED_EDGE('',*,*,#35017,.F.);
#47030=ORIENTED_EDGE('',*,*,#34919,.T.);
#47031=ORIENTED_EDGE('',*,*,#35018,.T.);
#47032=ORIENTED_EDGE('',*,*,#35019,.T.);
#47033=ORIENTED_EDGE('',*,*,#35020,.T.);
#47034=ORIENTED_EDGE('',*,*,#35021,.T.);
#47035=ORIENTED_EDGE('',*,*,#35022,.T.);
#47036=ORIENTED_EDGE('',*,*,#35023,.T.);
#47037=ORIENTED_EDGE('',*,*,#35024,.T.);
#47038=ORIENTED_EDGE('',*,*,#35021,.F.);
#47039=ORIENTED_EDGE('',*,*,#35025,.T.);
#47040=ORIENTED_EDGE('',*,*,#35026,.T.);
#47041=ORIENTED_EDGE('',*,*,#35027,.T.);
#47042=ORIENTED_EDGE('',*,*,#35023,.F.);
#47043=ORIENTED_EDGE('',*,*,#35028,.T.);
#47044=ORIENTED_EDGE('',*,*,#34897,.T.);
#47045=ORIENTED_EDGE('',*,*,#35029,.T.);
#47046=ORIENTED_EDGE('',*,*,#35026,.F.);
#47047=ORIENTED_EDGE('',*,*,#35030,.T.);
#47048=ORIENTED_EDGE('',*,*,#35031,.T.);
#47049=ORIENTED_EDGE('',*,*,#35032,.T.);
#47050=ORIENTED_EDGE('',*,*,#34894,.F.);
#47051=ORIENTED_EDGE('',*,*,#35033,.T.);
#47052=ORIENTED_EDGE('',*,*,#35034,.T.);
#47053=ORIENTED_EDGE('',*,*,#35035,.T.);
#47054=ORIENTED_EDGE('',*,*,#35031,.F.);
#47055=ORIENTED_EDGE('',*,*,#35036,.T.);
#47056=ORIENTED_EDGE('',*,*,#35037,.T.);
#47057=ORIENTED_EDGE('',*,*,#35038,.T.);
#47058=ORIENTED_EDGE('',*,*,#35034,.F.);
#47059=ORIENTED_EDGE('',*,*,#35039,.T.);
#47060=ORIENTED_EDGE('',*,*,#35007,.T.);
#47061=ORIENTED_EDGE('',*,*,#35040,.T.);
#47062=ORIENTED_EDGE('',*,*,#35037,.F.);
#47063=ORIENTED_EDGE('',*,*,#35018,.F.);
#47064=ORIENTED_EDGE('',*,*,#35041,.F.);
#47065=ORIENTED_EDGE('',*,*,#35042,.F.);
#47066=ORIENTED_EDGE('',*,*,#35043,.T.);
#47067=ORIENTED_EDGE('',*,*,#34909,.T.);
#47068=ORIENTED_EDGE('',*,*,#34941,.T.);
#47069=ORIENTED_EDGE('',*,*,#34933,.T.);
#47070=ORIENTED_EDGE('',*,*,#34929,.T.);
#47071=ORIENTED_EDGE('',*,*,#35024,.F.);
#47072=ORIENTED_EDGE('',*,*,#35044,.T.);
#47073=ORIENTED_EDGE('',*,*,#35045,.F.);
#47074=ORIENTED_EDGE('',*,*,#35041,.T.);
#47075=ORIENTED_EDGE('',*,*,#35027,.F.);
#47076=ORIENTED_EDGE('',*,*,#35046,.F.);
#47077=ORIENTED_EDGE('',*,*,#35047,.F.);
#47078=ORIENTED_EDGE('',*,*,#35044,.F.);
#47079=ORIENTED_EDGE('',*,*,#35029,.F.);
#47080=ORIENTED_EDGE('',*,*,#34956,.T.);
#47081=ORIENTED_EDGE('',*,*,#35048,.F.);
#47082=ORIENTED_EDGE('',*,*,#35046,.T.);
#47083=ORIENTED_EDGE('',*,*,#35032,.F.);
#47084=ORIENTED_EDGE('',*,*,#35049,.T.);
#47085=ORIENTED_EDGE('',*,*,#35050,.F.);
#47086=ORIENTED_EDGE('',*,*,#34901,.T.);
#47087=ORIENTED_EDGE('',*,*,#35035,.F.);
#47088=ORIENTED_EDGE('',*,*,#35051,.F.);
#47089=ORIENTED_EDGE('',*,*,#35052,.F.);
#47090=ORIENTED_EDGE('',*,*,#35049,.F.);
#47091=ORIENTED_EDGE('',*,*,#30526,.T.);
#47092=ORIENTED_EDGE('',*,*,#30560,.T.);
#47093=ORIENTED_EDGE('',*,*,#30557,.T.);
#47094=ORIENTED_EDGE('',*,*,#30554,.T.);
#47095=ORIENTED_EDGE('',*,*,#30551,.T.);
#47096=ORIENTED_EDGE('',*,*,#30548,.T.);
#47097=ORIENTED_EDGE('',*,*,#30545,.T.);
#47098=ORIENTED_EDGE('',*,*,#30542,.T.);
#47099=ORIENTED_EDGE('',*,*,#30539,.T.);
#47100=ORIENTED_EDGE('',*,*,#30536,.T.);
#47101=ORIENTED_EDGE('',*,*,#30533,.T.);
#47102=ORIENTED_EDGE('',*,*,#30530,.T.);
#47103=ORIENTED_EDGE('',*,*,#30613,.T.);
#47104=ORIENTED_EDGE('',*,*,#30659,.T.);
#47105=ORIENTED_EDGE('',*,*,#30656,.T.);
#47106=ORIENTED_EDGE('',*,*,#30653,.T.);
#47107=ORIENTED_EDGE('',*,*,#30650,.T.);
#47108=ORIENTED_EDGE('',*,*,#30647,.T.);
#47109=ORIENTED_EDGE('',*,*,#30644,.T.);
#47110=ORIENTED_EDGE('',*,*,#30641,.T.);
#47111=ORIENTED_EDGE('',*,*,#30638,.T.);
#47112=ORIENTED_EDGE('',*,*,#30635,.T.);
#47113=ORIENTED_EDGE('',*,*,#30632,.T.);
#47114=ORIENTED_EDGE('',*,*,#30629,.T.);
#47115=ORIENTED_EDGE('',*,*,#30626,.T.);
#47116=ORIENTED_EDGE('',*,*,#30623,.T.);
#47117=ORIENTED_EDGE('',*,*,#30620,.T.);
#47118=ORIENTED_EDGE('',*,*,#30617,.T.);
#47119=ORIENTED_EDGE('',*,*,#30778,.T.);
#47120=ORIENTED_EDGE('',*,*,#30812,.T.);
#47121=ORIENTED_EDGE('',*,*,#30809,.T.);
#47122=ORIENTED_EDGE('',*,*,#30806,.T.);
#47123=ORIENTED_EDGE('',*,*,#30803,.T.);
#47124=ORIENTED_EDGE('',*,*,#30800,.T.);
#47125=ORIENTED_EDGE('',*,*,#30797,.T.);
#47126=ORIENTED_EDGE('',*,*,#30794,.T.);
#47127=ORIENTED_EDGE('',*,*,#30791,.T.);
#47128=ORIENTED_EDGE('',*,*,#30788,.T.);
#47129=ORIENTED_EDGE('',*,*,#30785,.T.);
#47130=ORIENTED_EDGE('',*,*,#30782,.T.);
#47131=ORIENTED_EDGE('',*,*,#30841,.T.);
#47132=ORIENTED_EDGE('',*,*,#30896,.T.);
#47133=ORIENTED_EDGE('',*,*,#30893,.T.);
#47134=ORIENTED_EDGE('',*,*,#30890,.T.);
#47135=ORIENTED_EDGE('',*,*,#30887,.T.);
#47136=ORIENTED_EDGE('',*,*,#30884,.T.);
#47137=ORIENTED_EDGE('',*,*,#30881,.T.);
#47138=ORIENTED_EDGE('',*,*,#30878,.T.);
#47139=ORIENTED_EDGE('',*,*,#30875,.T.);
#47140=ORIENTED_EDGE('',*,*,#30872,.T.);
#47141=ORIENTED_EDGE('',*,*,#30869,.T.);
#47142=ORIENTED_EDGE('',*,*,#30866,.T.);
#47143=ORIENTED_EDGE('',*,*,#30863,.T.);
#47144=ORIENTED_EDGE('',*,*,#30860,.T.);
#47145=ORIENTED_EDGE('',*,*,#30857,.T.);
#47146=ORIENTED_EDGE('',*,*,#30854,.T.);
#47147=ORIENTED_EDGE('',*,*,#30851,.T.);
#47148=ORIENTED_EDGE('',*,*,#30848,.T.);
#47149=ORIENTED_EDGE('',*,*,#30845,.T.);
#47150=ORIENTED_EDGE('',*,*,#31048,.T.);
#47151=ORIENTED_EDGE('',*,*,#31082,.T.);
#47152=ORIENTED_EDGE('',*,*,#31079,.T.);
#47153=ORIENTED_EDGE('',*,*,#31076,.T.);
#47154=ORIENTED_EDGE('',*,*,#31073,.T.);
#47155=ORIENTED_EDGE('',*,*,#31070,.T.);
#47156=ORIENTED_EDGE('',*,*,#31067,.T.);
#47157=ORIENTED_EDGE('',*,*,#31064,.T.);
#47158=ORIENTED_EDGE('',*,*,#31061,.T.);
#47159=ORIENTED_EDGE('',*,*,#31058,.T.);
#47160=ORIENTED_EDGE('',*,*,#31055,.T.);
#47161=ORIENTED_EDGE('',*,*,#31052,.T.);
#47162=ORIENTED_EDGE('',*,*,#31093,.T.);
#47163=ORIENTED_EDGE('',*,*,#31124,.T.);
#47164=ORIENTED_EDGE('',*,*,#31121,.T.);
#47165=ORIENTED_EDGE('',*,*,#31118,.T.);
#47166=ORIENTED_EDGE('',*,*,#31115,.T.);
#47167=ORIENTED_EDGE('',*,*,#31112,.T.);
#47168=ORIENTED_EDGE('',*,*,#31109,.T.);
#47169=ORIENTED_EDGE('',*,*,#31106,.T.);
#47170=ORIENTED_EDGE('',*,*,#31103,.T.);
#47171=ORIENTED_EDGE('',*,*,#31100,.T.);
#47172=ORIENTED_EDGE('',*,*,#31097,.T.);
#47173=ORIENTED_EDGE('',*,*,#31300,.T.);
#47174=ORIENTED_EDGE('',*,*,#31334,.T.);
#47175=ORIENTED_EDGE('',*,*,#31331,.T.);
#47176=ORIENTED_EDGE('',*,*,#31328,.T.);
#47177=ORIENTED_EDGE('',*,*,#31325,.T.);
#47178=ORIENTED_EDGE('',*,*,#31322,.T.);
#47179=ORIENTED_EDGE('',*,*,#31319,.T.);
#47180=ORIENTED_EDGE('',*,*,#31316,.T.);
#47181=ORIENTED_EDGE('',*,*,#31313,.T.);
#47182=ORIENTED_EDGE('',*,*,#31310,.T.);
#47183=ORIENTED_EDGE('',*,*,#31307,.T.);
#47184=ORIENTED_EDGE('',*,*,#31304,.T.);
#47185=ORIENTED_EDGE('',*,*,#31336,.T.);
#47186=ORIENTED_EDGE('',*,*,#31400,.T.);
#47187=ORIENTED_EDGE('',*,*,#31397,.T.);
#47188=ORIENTED_EDGE('',*,*,#31394,.T.);
#47189=ORIENTED_EDGE('',*,*,#31391,.T.);
#47190=ORIENTED_EDGE('',*,*,#31388,.T.);
#47191=ORIENTED_EDGE('',*,*,#31385,.T.);
#47192=ORIENTED_EDGE('',*,*,#31382,.T.);
#47193=ORIENTED_EDGE('',*,*,#31379,.T.);
#47194=ORIENTED_EDGE('',*,*,#31376,.T.);
#47195=ORIENTED_EDGE('',*,*,#31373,.T.);
#47196=ORIENTED_EDGE('',*,*,#31370,.T.);
#47197=ORIENTED_EDGE('',*,*,#31367,.T.);
#47198=ORIENTED_EDGE('',*,*,#31364,.T.);
#47199=ORIENTED_EDGE('',*,*,#31361,.T.);
#47200=ORIENTED_EDGE('',*,*,#31358,.T.);
#47201=ORIENTED_EDGE('',*,*,#31355,.T.);
#47202=ORIENTED_EDGE('',*,*,#31352,.T.);
#47203=ORIENTED_EDGE('',*,*,#31349,.T.);
#47204=ORIENTED_EDGE('',*,*,#31346,.T.);
#47205=ORIENTED_EDGE('',*,*,#31343,.T.);
#47206=ORIENTED_EDGE('',*,*,#31340,.T.);
#47207=ORIENTED_EDGE('',*,*,#31513,.T.);
#47208=ORIENTED_EDGE('',*,*,#31547,.T.);
#47209=ORIENTED_EDGE('',*,*,#31544,.T.);
#47210=ORIENTED_EDGE('',*,*,#31541,.T.);
#47211=ORIENTED_EDGE('',*,*,#31538,.T.);
#47212=ORIENTED_EDGE('',*,*,#31535,.T.);
#47213=ORIENTED_EDGE('',*,*,#31532,.T.);
#47214=ORIENTED_EDGE('',*,*,#31529,.T.);
#47215=ORIENTED_EDGE('',*,*,#31526,.T.);
#47216=ORIENTED_EDGE('',*,*,#31523,.T.);
#47217=ORIENTED_EDGE('',*,*,#31520,.T.);
#47218=ORIENTED_EDGE('',*,*,#31517,.T.);
#47219=ORIENTED_EDGE('',*,*,#31660,.T.);
#47220=ORIENTED_EDGE('',*,*,#31694,.T.);
#47221=ORIENTED_EDGE('',*,*,#31691,.T.);
#47222=ORIENTED_EDGE('',*,*,#31688,.T.);
#47223=ORIENTED_EDGE('',*,*,#31685,.T.);
#47224=ORIENTED_EDGE('',*,*,#31682,.T.);
#47225=ORIENTED_EDGE('',*,*,#31679,.T.);
#47226=ORIENTED_EDGE('',*,*,#31676,.T.);
#47227=ORIENTED_EDGE('',*,*,#31673,.T.);
#47228=ORIENTED_EDGE('',*,*,#31670,.T.);
#47229=ORIENTED_EDGE('',*,*,#31667,.T.);
#47230=ORIENTED_EDGE('',*,*,#31664,.T.);
#47231=ORIENTED_EDGE('',*,*,#31696,.T.);
#47232=ORIENTED_EDGE('',*,*,#31760,.T.);
#47233=ORIENTED_EDGE('',*,*,#31757,.T.);
#47234=ORIENTED_EDGE('',*,*,#31754,.T.);
#47235=ORIENTED_EDGE('',*,*,#31751,.T.);
#47236=ORIENTED_EDGE('',*,*,#31748,.T.);
#47237=ORIENTED_EDGE('',*,*,#31745,.T.);
#47238=ORIENTED_EDGE('',*,*,#31742,.T.);
#47239=ORIENTED_EDGE('',*,*,#31739,.T.);
#47240=ORIENTED_EDGE('',*,*,#31736,.T.);
#47241=ORIENTED_EDGE('',*,*,#31733,.T.);
#47242=ORIENTED_EDGE('',*,*,#31730,.T.);
#47243=ORIENTED_EDGE('',*,*,#31727,.T.);
#47244=ORIENTED_EDGE('',*,*,#31724,.T.);
#47245=ORIENTED_EDGE('',*,*,#31721,.T.);
#47246=ORIENTED_EDGE('',*,*,#31718,.T.);
#47247=ORIENTED_EDGE('',*,*,#31715,.T.);
#47248=ORIENTED_EDGE('',*,*,#31712,.T.);
#47249=ORIENTED_EDGE('',*,*,#31709,.T.);
#47250=ORIENTED_EDGE('',*,*,#31706,.T.);
#47251=ORIENTED_EDGE('',*,*,#31703,.T.);
#47252=ORIENTED_EDGE('',*,*,#31700,.T.);
#47253=ORIENTED_EDGE('',*,*,#31936,.T.);
#47254=ORIENTED_EDGE('',*,*,#31970,.T.);
#47255=ORIENTED_EDGE('',*,*,#31967,.T.);
#47256=ORIENTED_EDGE('',*,*,#31964,.T.);
#47257=ORIENTED_EDGE('',*,*,#31961,.T.);
#47258=ORIENTED_EDGE('',*,*,#31958,.T.);
#47259=ORIENTED_EDGE('',*,*,#31955,.T.);
#47260=ORIENTED_EDGE('',*,*,#31952,.T.);
#47261=ORIENTED_EDGE('',*,*,#31949,.T.);
#47262=ORIENTED_EDGE('',*,*,#31946,.T.);
#47263=ORIENTED_EDGE('',*,*,#31943,.T.);
#47264=ORIENTED_EDGE('',*,*,#31940,.T.);
#47265=ORIENTED_EDGE('',*,*,#31981,.T.);
#47266=ORIENTED_EDGE('',*,*,#32012,.T.);
#47267=ORIENTED_EDGE('',*,*,#32009,.T.);
#47268=ORIENTED_EDGE('',*,*,#32006,.T.);
#47269=ORIENTED_EDGE('',*,*,#32003,.T.);
#47270=ORIENTED_EDGE('',*,*,#32000,.T.);
#47271=ORIENTED_EDGE('',*,*,#31997,.T.);
#47272=ORIENTED_EDGE('',*,*,#31994,.T.);
#47273=ORIENTED_EDGE('',*,*,#31991,.T.);
#47274=ORIENTED_EDGE('',*,*,#31988,.T.);
#47275=ORIENTED_EDGE('',*,*,#31985,.T.);
#47276=ORIENTED_EDGE('',*,*,#32164,.T.);
#47277=ORIENTED_EDGE('',*,*,#32198,.T.);
#47278=ORIENTED_EDGE('',*,*,#32195,.T.);
#47279=ORIENTED_EDGE('',*,*,#32192,.T.);
#47280=ORIENTED_EDGE('',*,*,#32189,.T.);
#47281=ORIENTED_EDGE('',*,*,#32186,.T.);
#47282=ORIENTED_EDGE('',*,*,#32183,.T.);
#47283=ORIENTED_EDGE('',*,*,#32180,.T.);
#47284=ORIENTED_EDGE('',*,*,#32177,.T.);
#47285=ORIENTED_EDGE('',*,*,#32174,.T.);
#47286=ORIENTED_EDGE('',*,*,#32171,.T.);
#47287=ORIENTED_EDGE('',*,*,#32168,.T.);
#47288=ORIENTED_EDGE('',*,*,#32227,.T.);
#47289=ORIENTED_EDGE('',*,*,#32282,.T.);
#47290=ORIENTED_EDGE('',*,*,#32279,.T.);
#47291=ORIENTED_EDGE('',*,*,#32276,.T.);
#47292=ORIENTED_EDGE('',*,*,#32273,.T.);
#47293=ORIENTED_EDGE('',*,*,#32270,.T.);
#47294=ORIENTED_EDGE('',*,*,#32267,.T.);
#47295=ORIENTED_EDGE('',*,*,#32264,.T.);
#47296=ORIENTED_EDGE('',*,*,#32261,.T.);
#47297=ORIENTED_EDGE('',*,*,#32258,.T.);
#47298=ORIENTED_EDGE('',*,*,#32255,.T.);
#47299=ORIENTED_EDGE('',*,*,#32252,.T.);
#47300=ORIENTED_EDGE('',*,*,#32249,.T.);
#47301=ORIENTED_EDGE('',*,*,#32246,.T.);
#47302=ORIENTED_EDGE('',*,*,#32243,.T.);
#47303=ORIENTED_EDGE('',*,*,#32240,.T.);
#47304=ORIENTED_EDGE('',*,*,#32237,.T.);
#47305=ORIENTED_EDGE('',*,*,#32234,.T.);
#47306=ORIENTED_EDGE('',*,*,#32231,.T.);
#47307=ORIENTED_EDGE('',*,*,#32401,.T.);
#47308=ORIENTED_EDGE('',*,*,#32435,.T.);
#47309=ORIENTED_EDGE('',*,*,#32432,.T.);
#47310=ORIENTED_EDGE('',*,*,#32429,.T.);
#47311=ORIENTED_EDGE('',*,*,#32426,.T.);
#47312=ORIENTED_EDGE('',*,*,#32423,.T.);
#47313=ORIENTED_EDGE('',*,*,#32420,.T.);
#47314=ORIENTED_EDGE('',*,*,#32417,.T.);
#47315=ORIENTED_EDGE('',*,*,#32414,.T.);
#47316=ORIENTED_EDGE('',*,*,#32411,.T.);
#47317=ORIENTED_EDGE('',*,*,#32408,.T.);
#47318=ORIENTED_EDGE('',*,*,#32405,.T.);
#47319=ORIENTED_EDGE('',*,*,#32488,.T.);
#47320=ORIENTED_EDGE('',*,*,#32534,.T.);
#47321=ORIENTED_EDGE('',*,*,#32531,.T.);
#47322=ORIENTED_EDGE('',*,*,#32528,.T.);
#47323=ORIENTED_EDGE('',*,*,#32525,.T.);
#47324=ORIENTED_EDGE('',*,*,#32522,.T.);
#47325=ORIENTED_EDGE('',*,*,#32519,.T.);
#47326=ORIENTED_EDGE('',*,*,#32516,.T.);
#47327=ORIENTED_EDGE('',*,*,#32513,.T.);
#47328=ORIENTED_EDGE('',*,*,#32510,.T.);
#47329=ORIENTED_EDGE('',*,*,#32507,.T.);
#47330=ORIENTED_EDGE('',*,*,#32504,.T.);
#47331=ORIENTED_EDGE('',*,*,#32501,.T.);
#47332=ORIENTED_EDGE('',*,*,#32498,.T.);
#47333=ORIENTED_EDGE('',*,*,#32495,.T.);
#47334=ORIENTED_EDGE('',*,*,#32492,.T.);
#47335=ORIENTED_EDGE('',*,*,#32686,.T.);
#47336=ORIENTED_EDGE('',*,*,#32696,.T.);
#47337=ORIENTED_EDGE('',*,*,#32693,.T.);
#47338=ORIENTED_EDGE('',*,*,#32690,.T.);
#47339=ORIENTED_EDGE('',*,*,#32698,.T.);
#47340=ORIENTED_EDGE('',*,*,#32708,.T.);
#47341=ORIENTED_EDGE('',*,*,#32705,.T.);
#47342=ORIENTED_EDGE('',*,*,#32702,.T.);
#47343=ORIENTED_EDGE('',*,*,#32710,.T.);
#47344=ORIENTED_EDGE('',*,*,#32720,.T.);
#47345=ORIENTED_EDGE('',*,*,#32717,.T.);
#47346=ORIENTED_EDGE('',*,*,#32714,.T.);
#47347=ORIENTED_EDGE('',*,*,#32722,.T.);
#47348=ORIENTED_EDGE('',*,*,#32732,.T.);
#47349=ORIENTED_EDGE('',*,*,#32729,.T.);
#47350=ORIENTED_EDGE('',*,*,#32726,.T.);
#47351=ORIENTED_EDGE('',*,*,#32734,.T.);
#47352=ORIENTED_EDGE('',*,*,#32744,.T.);
#47353=ORIENTED_EDGE('',*,*,#32741,.T.);
#47354=ORIENTED_EDGE('',*,*,#32738,.T.);
#47355=ORIENTED_EDGE('',*,*,#32746,.T.);
#47356=ORIENTED_EDGE('',*,*,#32756,.T.);
#47357=ORIENTED_EDGE('',*,*,#32753,.T.);
#47358=ORIENTED_EDGE('',*,*,#32750,.T.);
#47359=ORIENTED_EDGE('',*,*,#32758,.T.);
#47360=ORIENTED_EDGE('',*,*,#32768,.T.);
#47361=ORIENTED_EDGE('',*,*,#32765,.T.);
#47362=ORIENTED_EDGE('',*,*,#32762,.T.);
#47363=ORIENTED_EDGE('',*,*,#32770,.T.);
#47364=ORIENTED_EDGE('',*,*,#32780,.T.);
#47365=ORIENTED_EDGE('',*,*,#32777,.T.);
#47366=ORIENTED_EDGE('',*,*,#32774,.T.);
#47367=ORIENTED_EDGE('',*,*,#32782,.T.);
#47368=ORIENTED_EDGE('',*,*,#32792,.T.);
#47369=ORIENTED_EDGE('',*,*,#32789,.T.);
#47370=ORIENTED_EDGE('',*,*,#32786,.T.);
#47371=ORIENTED_EDGE('',*,*,#32794,.T.);
#47372=ORIENTED_EDGE('',*,*,#32804,.T.);
#47373=ORIENTED_EDGE('',*,*,#32801,.T.);
#47374=ORIENTED_EDGE('',*,*,#32798,.T.);
#47375=ORIENTED_EDGE('',*,*,#32806,.T.);
#47376=ORIENTED_EDGE('',*,*,#32816,.T.);
#47377=ORIENTED_EDGE('',*,*,#32813,.T.);
#47378=ORIENTED_EDGE('',*,*,#32810,.T.);
#47379=ORIENTED_EDGE('',*,*,#32818,.T.);
#47380=ORIENTED_EDGE('',*,*,#32828,.T.);
#47381=ORIENTED_EDGE('',*,*,#32825,.T.);
#47382=ORIENTED_EDGE('',*,*,#32822,.T.);
#47383=ORIENTED_EDGE('',*,*,#32830,.T.);
#47384=ORIENTED_EDGE('',*,*,#32840,.T.);
#47385=ORIENTED_EDGE('',*,*,#32837,.T.);
#47386=ORIENTED_EDGE('',*,*,#32834,.T.);
#47387=ORIENTED_EDGE('',*,*,#32842,.T.);
#47388=ORIENTED_EDGE('',*,*,#32852,.T.);
#47389=ORIENTED_EDGE('',*,*,#32849,.T.);
#47390=ORIENTED_EDGE('',*,*,#32846,.T.);
#47391=ORIENTED_EDGE('',*,*,#32854,.T.);
#47392=ORIENTED_EDGE('',*,*,#32864,.T.);
#47393=ORIENTED_EDGE('',*,*,#32861,.T.);
#47394=ORIENTED_EDGE('',*,*,#32858,.T.);
#47395=ORIENTED_EDGE('',*,*,#32866,.T.);
#47396=ORIENTED_EDGE('',*,*,#32876,.T.);
#47397=ORIENTED_EDGE('',*,*,#32873,.T.);
#47398=ORIENTED_EDGE('',*,*,#32870,.T.);
#47399=ORIENTED_EDGE('',*,*,#32878,.T.);
#47400=ORIENTED_EDGE('',*,*,#32888,.T.);
#47401=ORIENTED_EDGE('',*,*,#32885,.T.);
#47402=ORIENTED_EDGE('',*,*,#32882,.T.);
#47403=ORIENTED_EDGE('',*,*,#32890,.T.);
#47404=ORIENTED_EDGE('',*,*,#32900,.T.);
#47405=ORIENTED_EDGE('',*,*,#32897,.T.);
#47406=ORIENTED_EDGE('',*,*,#32894,.T.);
#47407=ORIENTED_EDGE('',*,*,#32902,.T.);
#47408=ORIENTED_EDGE('',*,*,#32912,.T.);
#47409=ORIENTED_EDGE('',*,*,#32909,.T.);
#47410=ORIENTED_EDGE('',*,*,#32906,.T.);
#47411=ORIENTED_EDGE('',*,*,#32914,.T.);
#47412=ORIENTED_EDGE('',*,*,#32924,.T.);
#47413=ORIENTED_EDGE('',*,*,#32921,.T.);
#47414=ORIENTED_EDGE('',*,*,#32918,.T.);
#47415=ORIENTED_EDGE('',*,*,#32926,.T.);
#47416=ORIENTED_EDGE('',*,*,#32936,.T.);
#47417=ORIENTED_EDGE('',*,*,#32933,.T.);
#47418=ORIENTED_EDGE('',*,*,#32930,.T.);
#47419=ORIENTED_EDGE('',*,*,#32938,.T.);
#47420=ORIENTED_EDGE('',*,*,#32948,.T.);
#47421=ORIENTED_EDGE('',*,*,#32945,.T.);
#47422=ORIENTED_EDGE('',*,*,#32942,.T.);
#47423=ORIENTED_EDGE('',*,*,#32950,.T.);
#47424=ORIENTED_EDGE('',*,*,#32960,.T.);
#47425=ORIENTED_EDGE('',*,*,#32957,.T.);
#47426=ORIENTED_EDGE('',*,*,#32954,.T.);
#47427=ORIENTED_EDGE('',*,*,#32962,.T.);
#47428=ORIENTED_EDGE('',*,*,#32972,.T.);
#47429=ORIENTED_EDGE('',*,*,#32969,.T.);
#47430=ORIENTED_EDGE('',*,*,#32966,.T.);
#47431=ORIENTED_EDGE('',*,*,#32974,.T.);
#47432=ORIENTED_EDGE('',*,*,#32984,.T.);
#47433=ORIENTED_EDGE('',*,*,#32981,.T.);
#47434=ORIENTED_EDGE('',*,*,#32978,.T.);
#47435=ORIENTED_EDGE('',*,*,#32986,.T.);
#47436=ORIENTED_EDGE('',*,*,#32996,.T.);
#47437=ORIENTED_EDGE('',*,*,#32993,.T.);
#47438=ORIENTED_EDGE('',*,*,#32990,.T.);
#47439=ORIENTED_EDGE('',*,*,#32998,.T.);
#47440=ORIENTED_EDGE('',*,*,#33008,.T.);
#47441=ORIENTED_EDGE('',*,*,#33005,.T.);
#47442=ORIENTED_EDGE('',*,*,#33002,.T.);
#47443=ORIENTED_EDGE('',*,*,#33010,.T.);
#47444=ORIENTED_EDGE('',*,*,#33020,.T.);
#47445=ORIENTED_EDGE('',*,*,#33017,.T.);
#47446=ORIENTED_EDGE('',*,*,#33014,.T.);
#47447=ORIENTED_EDGE('',*,*,#33022,.T.);
#47448=ORIENTED_EDGE('',*,*,#33032,.T.);
#47449=ORIENTED_EDGE('',*,*,#33029,.T.);
#47450=ORIENTED_EDGE('',*,*,#33026,.T.);
#47451=ORIENTED_EDGE('',*,*,#33034,.T.);
#47452=ORIENTED_EDGE('',*,*,#33044,.T.);
#47453=ORIENTED_EDGE('',*,*,#33041,.T.);
#47454=ORIENTED_EDGE('',*,*,#33038,.T.);
#47455=ORIENTED_EDGE('',*,*,#33046,.T.);
#47456=ORIENTED_EDGE('',*,*,#33056,.T.);
#47457=ORIENTED_EDGE('',*,*,#33053,.T.);
#47458=ORIENTED_EDGE('',*,*,#33050,.T.);
#47459=ORIENTED_EDGE('',*,*,#33058,.T.);
#47460=ORIENTED_EDGE('',*,*,#33068,.T.);
#47461=ORIENTED_EDGE('',*,*,#33065,.T.);
#47462=ORIENTED_EDGE('',*,*,#33062,.T.);
#47463=ORIENTED_EDGE('',*,*,#33070,.T.);
#47464=ORIENTED_EDGE('',*,*,#33080,.T.);
#47465=ORIENTED_EDGE('',*,*,#33077,.T.);
#47466=ORIENTED_EDGE('',*,*,#33074,.T.);
#47467=ORIENTED_EDGE('',*,*,#33082,.T.);
#47468=ORIENTED_EDGE('',*,*,#33092,.T.);
#47469=ORIENTED_EDGE('',*,*,#33089,.T.);
#47470=ORIENTED_EDGE('',*,*,#33086,.T.);
#47471=ORIENTED_EDGE('',*,*,#33094,.T.);
#47472=ORIENTED_EDGE('',*,*,#33104,.T.);
#47473=ORIENTED_EDGE('',*,*,#33101,.T.);
#47474=ORIENTED_EDGE('',*,*,#33098,.T.);
#47475=ORIENTED_EDGE('',*,*,#33106,.T.);
#47476=ORIENTED_EDGE('',*,*,#33116,.T.);
#47477=ORIENTED_EDGE('',*,*,#33113,.T.);
#47478=ORIENTED_EDGE('',*,*,#33110,.T.);
#47479=ORIENTED_EDGE('',*,*,#33118,.T.);
#47480=ORIENTED_EDGE('',*,*,#33128,.T.);
#47481=ORIENTED_EDGE('',*,*,#33125,.T.);
#47482=ORIENTED_EDGE('',*,*,#33122,.T.);
#47483=ORIENTED_EDGE('',*,*,#33130,.T.);
#47484=ORIENTED_EDGE('',*,*,#33140,.T.);
#47485=ORIENTED_EDGE('',*,*,#33137,.T.);
#47486=ORIENTED_EDGE('',*,*,#33134,.T.);
#47487=ORIENTED_EDGE('',*,*,#33142,.T.);
#47488=ORIENTED_EDGE('',*,*,#33152,.T.);
#47489=ORIENTED_EDGE('',*,*,#33149,.T.);
#47490=ORIENTED_EDGE('',*,*,#33146,.T.);
#47491=ORIENTED_EDGE('',*,*,#33154,.T.);
#47492=ORIENTED_EDGE('',*,*,#33164,.T.);
#47493=ORIENTED_EDGE('',*,*,#33161,.T.);
#47494=ORIENTED_EDGE('',*,*,#33158,.T.);
#47495=ORIENTED_EDGE('',*,*,#33166,.T.);
#47496=ORIENTED_EDGE('',*,*,#33176,.T.);
#47497=ORIENTED_EDGE('',*,*,#33173,.T.);
#47498=ORIENTED_EDGE('',*,*,#33170,.T.);
#47499=ORIENTED_EDGE('',*,*,#33178,.T.);
#47500=ORIENTED_EDGE('',*,*,#33188,.T.);
#47501=ORIENTED_EDGE('',*,*,#33185,.T.);
#47502=ORIENTED_EDGE('',*,*,#33182,.T.);
#47503=ORIENTED_EDGE('',*,*,#33190,.T.);
#47504=ORIENTED_EDGE('',*,*,#33200,.T.);
#47505=ORIENTED_EDGE('',*,*,#33197,.T.);
#47506=ORIENTED_EDGE('',*,*,#33194,.T.);
#47507=ORIENTED_EDGE('',*,*,#33202,.T.);
#47508=ORIENTED_EDGE('',*,*,#33212,.T.);
#47509=ORIENTED_EDGE('',*,*,#33209,.T.);
#47510=ORIENTED_EDGE('',*,*,#33206,.T.);
#47511=ORIENTED_EDGE('',*,*,#33214,.T.);
#47512=ORIENTED_EDGE('',*,*,#33224,.T.);
#47513=ORIENTED_EDGE('',*,*,#33221,.T.);
#47514=ORIENTED_EDGE('',*,*,#33218,.T.);
#47515=ORIENTED_EDGE('',*,*,#33226,.T.);
#47516=ORIENTED_EDGE('',*,*,#33236,.T.);
#47517=ORIENTED_EDGE('',*,*,#33233,.T.);
#47518=ORIENTED_EDGE('',*,*,#33230,.T.);
#47519=ORIENTED_EDGE('',*,*,#33238,.T.);
#47520=ORIENTED_EDGE('',*,*,#33248,.T.);
#47521=ORIENTED_EDGE('',*,*,#33245,.T.);
#47522=ORIENTED_EDGE('',*,*,#33242,.T.);
#47523=ORIENTED_EDGE('',*,*,#33250,.T.);
#47524=ORIENTED_EDGE('',*,*,#33260,.T.);
#47525=ORIENTED_EDGE('',*,*,#33257,.T.);
#47526=ORIENTED_EDGE('',*,*,#33254,.T.);
#47527=ORIENTED_EDGE('',*,*,#33262,.T.);
#47528=ORIENTED_EDGE('',*,*,#33272,.T.);
#47529=ORIENTED_EDGE('',*,*,#33269,.T.);
#47530=ORIENTED_EDGE('',*,*,#33266,.T.);
#47531=ORIENTED_EDGE('',*,*,#33274,.T.);
#47532=ORIENTED_EDGE('',*,*,#33284,.T.);
#47533=ORIENTED_EDGE('',*,*,#33281,.T.);
#47534=ORIENTED_EDGE('',*,*,#33278,.T.);
#47535=ORIENTED_EDGE('',*,*,#33286,.T.);
#47536=ORIENTED_EDGE('',*,*,#33296,.T.);
#47537=ORIENTED_EDGE('',*,*,#33293,.T.);
#47538=ORIENTED_EDGE('',*,*,#33290,.T.);
#47539=ORIENTED_EDGE('',*,*,#33298,.T.);
#47540=ORIENTED_EDGE('',*,*,#33308,.T.);
#47541=ORIENTED_EDGE('',*,*,#33305,.T.);
#47542=ORIENTED_EDGE('',*,*,#33302,.T.);
#47543=ORIENTED_EDGE('',*,*,#33310,.T.);
#47544=ORIENTED_EDGE('',*,*,#33320,.T.);
#47545=ORIENTED_EDGE('',*,*,#33317,.T.);
#47546=ORIENTED_EDGE('',*,*,#33314,.T.);
#47547=ORIENTED_EDGE('',*,*,#33322,.T.);
#47548=ORIENTED_EDGE('',*,*,#33332,.T.);
#47549=ORIENTED_EDGE('',*,*,#33329,.T.);
#47550=ORIENTED_EDGE('',*,*,#33326,.T.);
#47551=ORIENTED_EDGE('',*,*,#33334,.T.);
#47552=ORIENTED_EDGE('',*,*,#33344,.T.);
#47553=ORIENTED_EDGE('',*,*,#33341,.T.);
#47554=ORIENTED_EDGE('',*,*,#33338,.T.);
#47555=ORIENTED_EDGE('',*,*,#33346,.T.);
#47556=ORIENTED_EDGE('',*,*,#33356,.T.);
#47557=ORIENTED_EDGE('',*,*,#33353,.T.);
#47558=ORIENTED_EDGE('',*,*,#33350,.T.);
#47559=ORIENTED_EDGE('',*,*,#33358,.T.);
#47560=ORIENTED_EDGE('',*,*,#33368,.T.);
#47561=ORIENTED_EDGE('',*,*,#33365,.T.);
#47562=ORIENTED_EDGE('',*,*,#33362,.T.);
#47563=ORIENTED_EDGE('',*,*,#33370,.T.);
#47564=ORIENTED_EDGE('',*,*,#33380,.T.);
#47565=ORIENTED_EDGE('',*,*,#33377,.T.);
#47566=ORIENTED_EDGE('',*,*,#33374,.T.);
#47567=ORIENTED_EDGE('',*,*,#33382,.T.);
#47568=ORIENTED_EDGE('',*,*,#33392,.T.);
#47569=ORIENTED_EDGE('',*,*,#33389,.T.);
#47570=ORIENTED_EDGE('',*,*,#33386,.T.);
#47571=ORIENTED_EDGE('',*,*,#33394,.T.);
#47572=ORIENTED_EDGE('',*,*,#33404,.T.);
#47573=ORIENTED_EDGE('',*,*,#33401,.T.);
#47574=ORIENTED_EDGE('',*,*,#33398,.T.);
#47575=ORIENTED_EDGE('',*,*,#33406,.T.);
#47576=ORIENTED_EDGE('',*,*,#33416,.T.);
#47577=ORIENTED_EDGE('',*,*,#33413,.T.);
#47578=ORIENTED_EDGE('',*,*,#33410,.T.);
#47579=ORIENTED_EDGE('',*,*,#33418,.T.);
#47580=ORIENTED_EDGE('',*,*,#33428,.T.);
#47581=ORIENTED_EDGE('',*,*,#33425,.T.);
#47582=ORIENTED_EDGE('',*,*,#33422,.T.);
#47583=ORIENTED_EDGE('',*,*,#33430,.T.);
#47584=ORIENTED_EDGE('',*,*,#33440,.T.);
#47585=ORIENTED_EDGE('',*,*,#33437,.T.);
#47586=ORIENTED_EDGE('',*,*,#33434,.T.);
#47587=ORIENTED_EDGE('',*,*,#33442,.T.);
#47588=ORIENTED_EDGE('',*,*,#33452,.T.);
#47589=ORIENTED_EDGE('',*,*,#33449,.T.);
#47590=ORIENTED_EDGE('',*,*,#33446,.T.);
#47591=ORIENTED_EDGE('',*,*,#33454,.T.);
#47592=ORIENTED_EDGE('',*,*,#33464,.T.);
#47593=ORIENTED_EDGE('',*,*,#33461,.T.);
#47594=ORIENTED_EDGE('',*,*,#33458,.T.);
#47595=ORIENTED_EDGE('',*,*,#33466,.T.);
#47596=ORIENTED_EDGE('',*,*,#33476,.T.);
#47597=ORIENTED_EDGE('',*,*,#33473,.T.);
#47598=ORIENTED_EDGE('',*,*,#33470,.T.);
#47599=ORIENTED_EDGE('',*,*,#33478,.T.);
#47600=ORIENTED_EDGE('',*,*,#33488,.T.);
#47601=ORIENTED_EDGE('',*,*,#33485,.T.);
#47602=ORIENTED_EDGE('',*,*,#33482,.T.);
#47603=ORIENTED_EDGE('',*,*,#33490,.T.);
#47604=ORIENTED_EDGE('',*,*,#33500,.T.);
#47605=ORIENTED_EDGE('',*,*,#33497,.T.);
#47606=ORIENTED_EDGE('',*,*,#33494,.T.);
#47607=ORIENTED_EDGE('',*,*,#33502,.T.);
#47608=ORIENTED_EDGE('',*,*,#33512,.T.);
#47609=ORIENTED_EDGE('',*,*,#33509,.T.);
#47610=ORIENTED_EDGE('',*,*,#33506,.T.);
#47611=ORIENTED_EDGE('',*,*,#33514,.T.);
#47612=ORIENTED_EDGE('',*,*,#33524,.T.);
#47613=ORIENTED_EDGE('',*,*,#33521,.T.);
#47614=ORIENTED_EDGE('',*,*,#33518,.T.);
#47615=ORIENTED_EDGE('',*,*,#33526,.T.);
#47616=ORIENTED_EDGE('',*,*,#33536,.T.);
#47617=ORIENTED_EDGE('',*,*,#33533,.T.);
#47618=ORIENTED_EDGE('',*,*,#33530,.T.);
#47619=ORIENTED_EDGE('',*,*,#33538,.T.);
#47620=ORIENTED_EDGE('',*,*,#33548,.T.);
#47621=ORIENTED_EDGE('',*,*,#33545,.T.);
#47622=ORIENTED_EDGE('',*,*,#33542,.T.);
#47623=ORIENTED_EDGE('',*,*,#33550,.T.);
#47624=ORIENTED_EDGE('',*,*,#33560,.T.);
#47625=ORIENTED_EDGE('',*,*,#33557,.T.);
#47626=ORIENTED_EDGE('',*,*,#33554,.T.);
#47627=ORIENTED_EDGE('',*,*,#33562,.T.);
#47628=ORIENTED_EDGE('',*,*,#33572,.T.);
#47629=ORIENTED_EDGE('',*,*,#33569,.T.);
#47630=ORIENTED_EDGE('',*,*,#33566,.T.);
#47631=ORIENTED_EDGE('',*,*,#33574,.T.);
#47632=ORIENTED_EDGE('',*,*,#33584,.T.);
#47633=ORIENTED_EDGE('',*,*,#33581,.T.);
#47634=ORIENTED_EDGE('',*,*,#33578,.T.);
#47635=ORIENTED_EDGE('',*,*,#33586,.T.);
#47636=ORIENTED_EDGE('',*,*,#33596,.T.);
#47637=ORIENTED_EDGE('',*,*,#33593,.T.);
#47638=ORIENTED_EDGE('',*,*,#33590,.T.);
#47639=ORIENTED_EDGE('',*,*,#33598,.T.);
#47640=ORIENTED_EDGE('',*,*,#33608,.T.);
#47641=ORIENTED_EDGE('',*,*,#33605,.T.);
#47642=ORIENTED_EDGE('',*,*,#33602,.T.);
#47643=ORIENTED_EDGE('',*,*,#33610,.T.);
#47644=ORIENTED_EDGE('',*,*,#33620,.T.);
#47645=ORIENTED_EDGE('',*,*,#33617,.T.);
#47646=ORIENTED_EDGE('',*,*,#33614,.T.);
#47647=ORIENTED_EDGE('',*,*,#33622,.T.);
#47648=ORIENTED_EDGE('',*,*,#33632,.T.);
#47649=ORIENTED_EDGE('',*,*,#33629,.T.);
#47650=ORIENTED_EDGE('',*,*,#33626,.T.);
#47651=ORIENTED_EDGE('',*,*,#33634,.T.);
#47652=ORIENTED_EDGE('',*,*,#33644,.T.);
#47653=ORIENTED_EDGE('',*,*,#33641,.T.);
#47654=ORIENTED_EDGE('',*,*,#33638,.T.);
#47655=ORIENTED_EDGE('',*,*,#33646,.T.);
#47656=ORIENTED_EDGE('',*,*,#33656,.T.);
#47657=ORIENTED_EDGE('',*,*,#33653,.T.);
#47658=ORIENTED_EDGE('',*,*,#33650,.T.);
#47659=ORIENTED_EDGE('',*,*,#33658,.T.);
#47660=ORIENTED_EDGE('',*,*,#33668,.T.);
#47661=ORIENTED_EDGE('',*,*,#33665,.T.);
#47662=ORIENTED_EDGE('',*,*,#33662,.T.);
#47663=ORIENTED_EDGE('',*,*,#33670,.T.);
#47664=ORIENTED_EDGE('',*,*,#33680,.T.);
#47665=ORIENTED_EDGE('',*,*,#33677,.T.);
#47666=ORIENTED_EDGE('',*,*,#33674,.T.);
#47667=ORIENTED_EDGE('',*,*,#33682,.T.);
#47668=ORIENTED_EDGE('',*,*,#33692,.T.);
#47669=ORIENTED_EDGE('',*,*,#33689,.T.);
#47670=ORIENTED_EDGE('',*,*,#33686,.T.);
#47671=ORIENTED_EDGE('',*,*,#33694,.T.);
#47672=ORIENTED_EDGE('',*,*,#33704,.T.);
#47673=ORIENTED_EDGE('',*,*,#33701,.T.);
#47674=ORIENTED_EDGE('',*,*,#33698,.T.);
#47675=ORIENTED_EDGE('',*,*,#33706,.T.);
#47676=ORIENTED_EDGE('',*,*,#33716,.T.);
#47677=ORIENTED_EDGE('',*,*,#33713,.T.);
#47678=ORIENTED_EDGE('',*,*,#33710,.T.);
#47679=ORIENTED_EDGE('',*,*,#33718,.T.);
#47680=ORIENTED_EDGE('',*,*,#33728,.T.);
#47681=ORIENTED_EDGE('',*,*,#33725,.T.);
#47682=ORIENTED_EDGE('',*,*,#33722,.T.);
#47683=ORIENTED_EDGE('',*,*,#33730,.T.);
#47684=ORIENTED_EDGE('',*,*,#33740,.T.);
#47685=ORIENTED_EDGE('',*,*,#33737,.T.);
#47686=ORIENTED_EDGE('',*,*,#33734,.T.);
#47687=ORIENTED_EDGE('',*,*,#33742,.T.);
#47688=ORIENTED_EDGE('',*,*,#33752,.T.);
#47689=ORIENTED_EDGE('',*,*,#33749,.T.);
#47690=ORIENTED_EDGE('',*,*,#33746,.T.);
#47691=ORIENTED_EDGE('',*,*,#33754,.T.);
#47692=ORIENTED_EDGE('',*,*,#33764,.T.);
#47693=ORIENTED_EDGE('',*,*,#33761,.T.);
#47694=ORIENTED_EDGE('',*,*,#33758,.T.);
#47695=ORIENTED_EDGE('',*,*,#33766,.T.);
#47696=ORIENTED_EDGE('',*,*,#33776,.T.);
#47697=ORIENTED_EDGE('',*,*,#33773,.T.);
#47698=ORIENTED_EDGE('',*,*,#33770,.T.);
#47699=ORIENTED_EDGE('',*,*,#33778,.T.);
#47700=ORIENTED_EDGE('',*,*,#33788,.T.);
#47701=ORIENTED_EDGE('',*,*,#33785,.T.);
#47702=ORIENTED_EDGE('',*,*,#33782,.T.);
#47703=ORIENTED_EDGE('',*,*,#33790,.T.);
#47704=ORIENTED_EDGE('',*,*,#33800,.T.);
#47705=ORIENTED_EDGE('',*,*,#33797,.T.);
#47706=ORIENTED_EDGE('',*,*,#33794,.T.);
#47707=ORIENTED_EDGE('',*,*,#33802,.T.);
#47708=ORIENTED_EDGE('',*,*,#33812,.T.);
#47709=ORIENTED_EDGE('',*,*,#33809,.T.);
#47710=ORIENTED_EDGE('',*,*,#33806,.T.);
#47711=ORIENTED_EDGE('',*,*,#33814,.T.);
#47712=ORIENTED_EDGE('',*,*,#33824,.T.);
#47713=ORIENTED_EDGE('',*,*,#33821,.T.);
#47714=ORIENTED_EDGE('',*,*,#33818,.T.);
#47715=ORIENTED_EDGE('',*,*,#33826,.T.);
#47716=ORIENTED_EDGE('',*,*,#33836,.T.);
#47717=ORIENTED_EDGE('',*,*,#33833,.T.);
#47718=ORIENTED_EDGE('',*,*,#33830,.T.);
#47719=ORIENTED_EDGE('',*,*,#33838,.T.);
#47720=ORIENTED_EDGE('',*,*,#33848,.T.);
#47721=ORIENTED_EDGE('',*,*,#33845,.T.);
#47722=ORIENTED_EDGE('',*,*,#33842,.T.);
#47723=ORIENTED_EDGE('',*,*,#33850,.T.);
#47724=ORIENTED_EDGE('',*,*,#33860,.T.);
#47725=ORIENTED_EDGE('',*,*,#33857,.T.);
#47726=ORIENTED_EDGE('',*,*,#33854,.T.);
#47727=ORIENTED_EDGE('',*,*,#33862,.T.);
#47728=ORIENTED_EDGE('',*,*,#33872,.T.);
#47729=ORIENTED_EDGE('',*,*,#33869,.T.);
#47730=ORIENTED_EDGE('',*,*,#33866,.T.);
#47731=ORIENTED_EDGE('',*,*,#33874,.T.);
#47732=ORIENTED_EDGE('',*,*,#33884,.T.);
#47733=ORIENTED_EDGE('',*,*,#33881,.T.);
#47734=ORIENTED_EDGE('',*,*,#33878,.T.);
#47735=ORIENTED_EDGE('',*,*,#33886,.T.);
#47736=ORIENTED_EDGE('',*,*,#33896,.T.);
#47737=ORIENTED_EDGE('',*,*,#33893,.T.);
#47738=ORIENTED_EDGE('',*,*,#33890,.T.);
#47739=ORIENTED_EDGE('',*,*,#33898,.T.);
#47740=ORIENTED_EDGE('',*,*,#33908,.T.);
#47741=ORIENTED_EDGE('',*,*,#33905,.T.);
#47742=ORIENTED_EDGE('',*,*,#33902,.T.);
#47743=ORIENTED_EDGE('',*,*,#33910,.T.);
#47744=ORIENTED_EDGE('',*,*,#33920,.T.);
#47745=ORIENTED_EDGE('',*,*,#33917,.T.);
#47746=ORIENTED_EDGE('',*,*,#33914,.T.);
#47747=ORIENTED_EDGE('',*,*,#33922,.T.);
#47748=ORIENTED_EDGE('',*,*,#33932,.T.);
#47749=ORIENTED_EDGE('',*,*,#33929,.T.);
#47750=ORIENTED_EDGE('',*,*,#33926,.T.);
#47751=ORIENTED_EDGE('',*,*,#33934,.T.);
#47752=ORIENTED_EDGE('',*,*,#33944,.T.);
#47753=ORIENTED_EDGE('',*,*,#33941,.T.);
#47754=ORIENTED_EDGE('',*,*,#33938,.T.);
#47755=ORIENTED_EDGE('',*,*,#33946,.T.);
#47756=ORIENTED_EDGE('',*,*,#33956,.T.);
#47757=ORIENTED_EDGE('',*,*,#33953,.T.);
#47758=ORIENTED_EDGE('',*,*,#33950,.T.);
#47759=ORIENTED_EDGE('',*,*,#33958,.T.);
#47760=ORIENTED_EDGE('',*,*,#33968,.T.);
#47761=ORIENTED_EDGE('',*,*,#33965,.T.);
#47762=ORIENTED_EDGE('',*,*,#33962,.T.);
#47763=ORIENTED_EDGE('',*,*,#33970,.T.);
#47764=ORIENTED_EDGE('',*,*,#33980,.T.);
#47765=ORIENTED_EDGE('',*,*,#33977,.T.);
#47766=ORIENTED_EDGE('',*,*,#33974,.T.);
#47767=ORIENTED_EDGE('',*,*,#33982,.T.);
#47768=ORIENTED_EDGE('',*,*,#33992,.T.);
#47769=ORIENTED_EDGE('',*,*,#33989,.T.);
#47770=ORIENTED_EDGE('',*,*,#33986,.T.);
#47771=ORIENTED_EDGE('',*,*,#33994,.T.);
#47772=ORIENTED_EDGE('',*,*,#34004,.T.);
#47773=ORIENTED_EDGE('',*,*,#34001,.T.);
#47774=ORIENTED_EDGE('',*,*,#33998,.T.);
#47775=ORIENTED_EDGE('',*,*,#34006,.T.);
#47776=ORIENTED_EDGE('',*,*,#34016,.T.);
#47777=ORIENTED_EDGE('',*,*,#34013,.T.);
#47778=ORIENTED_EDGE('',*,*,#34010,.T.);
#47779=ORIENTED_EDGE('',*,*,#34018,.T.);
#47780=ORIENTED_EDGE('',*,*,#34028,.T.);
#47781=ORIENTED_EDGE('',*,*,#34025,.T.);
#47782=ORIENTED_EDGE('',*,*,#34022,.T.);
#47783=ORIENTED_EDGE('',*,*,#34030,.T.);
#47784=ORIENTED_EDGE('',*,*,#34040,.T.);
#47785=ORIENTED_EDGE('',*,*,#34037,.T.);
#47786=ORIENTED_EDGE('',*,*,#34034,.T.);
#47787=ORIENTED_EDGE('',*,*,#34042,.T.);
#47788=ORIENTED_EDGE('',*,*,#34052,.T.);
#47789=ORIENTED_EDGE('',*,*,#34049,.T.);
#47790=ORIENTED_EDGE('',*,*,#34046,.T.);
#47791=ORIENTED_EDGE('',*,*,#34054,.T.);
#47792=ORIENTED_EDGE('',*,*,#34064,.T.);
#47793=ORIENTED_EDGE('',*,*,#34061,.T.);
#47794=ORIENTED_EDGE('',*,*,#34058,.T.);
#47795=ORIENTED_EDGE('',*,*,#34066,.T.);
#47796=ORIENTED_EDGE('',*,*,#34076,.T.);
#47797=ORIENTED_EDGE('',*,*,#34073,.T.);
#47798=ORIENTED_EDGE('',*,*,#34070,.T.);
#47799=ORIENTED_EDGE('',*,*,#34078,.T.);
#47800=ORIENTED_EDGE('',*,*,#34088,.T.);
#47801=ORIENTED_EDGE('',*,*,#34085,.T.);
#47802=ORIENTED_EDGE('',*,*,#34082,.T.);
#47803=ORIENTED_EDGE('',*,*,#34090,.T.);
#47804=ORIENTED_EDGE('',*,*,#34100,.T.);
#47805=ORIENTED_EDGE('',*,*,#34097,.T.);
#47806=ORIENTED_EDGE('',*,*,#34094,.T.);
#47807=ORIENTED_EDGE('',*,*,#34102,.T.);
#47808=ORIENTED_EDGE('',*,*,#34112,.T.);
#47809=ORIENTED_EDGE('',*,*,#34109,.T.);
#47810=ORIENTED_EDGE('',*,*,#34106,.T.);
#47811=ORIENTED_EDGE('',*,*,#34114,.T.);
#47812=ORIENTED_EDGE('',*,*,#34124,.T.);
#47813=ORIENTED_EDGE('',*,*,#34121,.T.);
#47814=ORIENTED_EDGE('',*,*,#34118,.T.);
#47815=ORIENTED_EDGE('',*,*,#34126,.T.);
#47816=ORIENTED_EDGE('',*,*,#34136,.T.);
#47817=ORIENTED_EDGE('',*,*,#34133,.T.);
#47818=ORIENTED_EDGE('',*,*,#34130,.T.);
#47819=ORIENTED_EDGE('',*,*,#34138,.T.);
#47820=ORIENTED_EDGE('',*,*,#34148,.T.);
#47821=ORIENTED_EDGE('',*,*,#34145,.T.);
#47822=ORIENTED_EDGE('',*,*,#34142,.T.);
#47823=ORIENTED_EDGE('',*,*,#34150,.T.);
#47824=ORIENTED_EDGE('',*,*,#34160,.T.);
#47825=ORIENTED_EDGE('',*,*,#34157,.T.);
#47826=ORIENTED_EDGE('',*,*,#34154,.T.);
#47827=ORIENTED_EDGE('',*,*,#34162,.T.);
#47828=ORIENTED_EDGE('',*,*,#34172,.T.);
#47829=ORIENTED_EDGE('',*,*,#34169,.T.);
#47830=ORIENTED_EDGE('',*,*,#34166,.T.);
#47831=ORIENTED_EDGE('',*,*,#34174,.T.);
#47832=ORIENTED_EDGE('',*,*,#34184,.T.);
#47833=ORIENTED_EDGE('',*,*,#34181,.T.);
#47834=ORIENTED_EDGE('',*,*,#34178,.T.);
#47835=ORIENTED_EDGE('',*,*,#34186,.T.);
#47836=ORIENTED_EDGE('',*,*,#34196,.T.);
#47837=ORIENTED_EDGE('',*,*,#34193,.T.);
#47838=ORIENTED_EDGE('',*,*,#34190,.T.);
#47839=ORIENTED_EDGE('',*,*,#34198,.T.);
#47840=ORIENTED_EDGE('',*,*,#34208,.T.);
#47841=ORIENTED_EDGE('',*,*,#34205,.T.);
#47842=ORIENTED_EDGE('',*,*,#34202,.T.);
#47843=ORIENTED_EDGE('',*,*,#34210,.T.);
#47844=ORIENTED_EDGE('',*,*,#34220,.T.);
#47845=ORIENTED_EDGE('',*,*,#34217,.T.);
#47846=ORIENTED_EDGE('',*,*,#34214,.T.);
#47847=ORIENTED_EDGE('',*,*,#34222,.T.);
#47848=ORIENTED_EDGE('',*,*,#34232,.T.);
#47849=ORIENTED_EDGE('',*,*,#34229,.T.);
#47850=ORIENTED_EDGE('',*,*,#34226,.T.);
#47851=ORIENTED_EDGE('',*,*,#34234,.T.);
#47852=ORIENTED_EDGE('',*,*,#34244,.T.);
#47853=ORIENTED_EDGE('',*,*,#34241,.T.);
#47854=ORIENTED_EDGE('',*,*,#34238,.T.);
#47855=ORIENTED_EDGE('',*,*,#34246,.T.);
#47856=ORIENTED_EDGE('',*,*,#34256,.T.);
#47857=ORIENTED_EDGE('',*,*,#34253,.T.);
#47858=ORIENTED_EDGE('',*,*,#34250,.T.);
#47859=ORIENTED_EDGE('',*,*,#34258,.T.);
#47860=ORIENTED_EDGE('',*,*,#34268,.T.);
#47861=ORIENTED_EDGE('',*,*,#34265,.T.);
#47862=ORIENTED_EDGE('',*,*,#34262,.T.);
#47863=ORIENTED_EDGE('',*,*,#34270,.T.);
#47864=ORIENTED_EDGE('',*,*,#34280,.T.);
#47865=ORIENTED_EDGE('',*,*,#34277,.T.);
#47866=ORIENTED_EDGE('',*,*,#34274,.T.);
#47867=ORIENTED_EDGE('',*,*,#34282,.T.);
#47868=ORIENTED_EDGE('',*,*,#34292,.T.);
#47869=ORIENTED_EDGE('',*,*,#34289,.T.);
#47870=ORIENTED_EDGE('',*,*,#34286,.T.);
#47871=ORIENTED_EDGE('',*,*,#34294,.T.);
#47872=ORIENTED_EDGE('',*,*,#34304,.T.);
#47873=ORIENTED_EDGE('',*,*,#34301,.T.);
#47874=ORIENTED_EDGE('',*,*,#34298,.T.);
#47875=ORIENTED_EDGE('',*,*,#34306,.T.);
#47876=ORIENTED_EDGE('',*,*,#34316,.T.);
#47877=ORIENTED_EDGE('',*,*,#34313,.T.);
#47878=ORIENTED_EDGE('',*,*,#34310,.T.);
#47879=ORIENTED_EDGE('',*,*,#34318,.T.);
#47880=ORIENTED_EDGE('',*,*,#34328,.T.);
#47881=ORIENTED_EDGE('',*,*,#34325,.T.);
#47882=ORIENTED_EDGE('',*,*,#34322,.T.);
#47883=ORIENTED_EDGE('',*,*,#34330,.T.);
#47884=ORIENTED_EDGE('',*,*,#34340,.T.);
#47885=ORIENTED_EDGE('',*,*,#34337,.T.);
#47886=ORIENTED_EDGE('',*,*,#34334,.T.);
#47887=ORIENTED_EDGE('',*,*,#34342,.T.);
#47888=ORIENTED_EDGE('',*,*,#34352,.T.);
#47889=ORIENTED_EDGE('',*,*,#34349,.T.);
#47890=ORIENTED_EDGE('',*,*,#34346,.T.);
#47891=ORIENTED_EDGE('',*,*,#34354,.T.);
#47892=ORIENTED_EDGE('',*,*,#34364,.T.);
#47893=ORIENTED_EDGE('',*,*,#34361,.T.);
#47894=ORIENTED_EDGE('',*,*,#34358,.T.);
#47895=ORIENTED_EDGE('',*,*,#34366,.T.);
#47896=ORIENTED_EDGE('',*,*,#34376,.T.);
#47897=ORIENTED_EDGE('',*,*,#34373,.T.);
#47898=ORIENTED_EDGE('',*,*,#34370,.T.);
#47899=ORIENTED_EDGE('',*,*,#34378,.T.);
#47900=ORIENTED_EDGE('',*,*,#34388,.T.);
#47901=ORIENTED_EDGE('',*,*,#34385,.T.);
#47902=ORIENTED_EDGE('',*,*,#34382,.T.);
#47903=ORIENTED_EDGE('',*,*,#34390,.T.);
#47904=ORIENTED_EDGE('',*,*,#34400,.T.);
#47905=ORIENTED_EDGE('',*,*,#34397,.T.);
#47906=ORIENTED_EDGE('',*,*,#34394,.T.);
#47907=ORIENTED_EDGE('',*,*,#34402,.T.);
#47908=ORIENTED_EDGE('',*,*,#34412,.T.);
#47909=ORIENTED_EDGE('',*,*,#34409,.T.);
#47910=ORIENTED_EDGE('',*,*,#34406,.T.);
#47911=ORIENTED_EDGE('',*,*,#34414,.T.);
#47912=ORIENTED_EDGE('',*,*,#34424,.T.);
#47913=ORIENTED_EDGE('',*,*,#34421,.T.);
#47914=ORIENTED_EDGE('',*,*,#34418,.T.);
#47915=ORIENTED_EDGE('',*,*,#34426,.T.);
#47916=ORIENTED_EDGE('',*,*,#34436,.T.);
#47917=ORIENTED_EDGE('',*,*,#34433,.T.);
#47918=ORIENTED_EDGE('',*,*,#34430,.T.);
#47919=ORIENTED_EDGE('',*,*,#34438,.T.);
#47920=ORIENTED_EDGE('',*,*,#34448,.T.);
#47921=ORIENTED_EDGE('',*,*,#34445,.T.);
#47922=ORIENTED_EDGE('',*,*,#34442,.T.);
#47923=ORIENTED_EDGE('',*,*,#34450,.T.);
#47924=ORIENTED_EDGE('',*,*,#34460,.T.);
#47925=ORIENTED_EDGE('',*,*,#34457,.T.);
#47926=ORIENTED_EDGE('',*,*,#34454,.T.);
#47927=ORIENTED_EDGE('',*,*,#34462,.T.);
#47928=ORIENTED_EDGE('',*,*,#34472,.T.);
#47929=ORIENTED_EDGE('',*,*,#34469,.T.);
#47930=ORIENTED_EDGE('',*,*,#34466,.T.);
#47931=ORIENTED_EDGE('',*,*,#34474,.T.);
#47932=ORIENTED_EDGE('',*,*,#34484,.T.);
#47933=ORIENTED_EDGE('',*,*,#34481,.T.);
#47934=ORIENTED_EDGE('',*,*,#34478,.T.);
#47935=ORIENTED_EDGE('',*,*,#34486,.T.);
#47936=ORIENTED_EDGE('',*,*,#34496,.T.);
#47937=ORIENTED_EDGE('',*,*,#34493,.T.);
#47938=ORIENTED_EDGE('',*,*,#34490,.T.);
#47939=ORIENTED_EDGE('',*,*,#34498,.T.);
#47940=ORIENTED_EDGE('',*,*,#34508,.T.);
#47941=ORIENTED_EDGE('',*,*,#34505,.T.);
#47942=ORIENTED_EDGE('',*,*,#34502,.T.);
#47943=ORIENTED_EDGE('',*,*,#34510,.T.);
#47944=ORIENTED_EDGE('',*,*,#34520,.T.);
#47945=ORIENTED_EDGE('',*,*,#34517,.T.);
#47946=ORIENTED_EDGE('',*,*,#34514,.T.);
#47947=ORIENTED_EDGE('',*,*,#34522,.T.);
#47948=ORIENTED_EDGE('',*,*,#34532,.T.);
#47949=ORIENTED_EDGE('',*,*,#34529,.T.);
#47950=ORIENTED_EDGE('',*,*,#34526,.T.);
#47951=ORIENTED_EDGE('',*,*,#34534,.T.);
#47952=ORIENTED_EDGE('',*,*,#34544,.T.);
#47953=ORIENTED_EDGE('',*,*,#34541,.T.);
#47954=ORIENTED_EDGE('',*,*,#34538,.T.);
#47955=ORIENTED_EDGE('',*,*,#34546,.T.);
#47956=ORIENTED_EDGE('',*,*,#34556,.T.);
#47957=ORIENTED_EDGE('',*,*,#34553,.T.);
#47958=ORIENTED_EDGE('',*,*,#34550,.T.);
#47959=ORIENTED_EDGE('',*,*,#34558,.T.);
#47960=ORIENTED_EDGE('',*,*,#34568,.T.);
#47961=ORIENTED_EDGE('',*,*,#34565,.T.);
#47962=ORIENTED_EDGE('',*,*,#34562,.T.);
#47963=ORIENTED_EDGE('',*,*,#34570,.T.);
#47964=ORIENTED_EDGE('',*,*,#34580,.T.);
#47965=ORIENTED_EDGE('',*,*,#34577,.T.);
#47966=ORIENTED_EDGE('',*,*,#34574,.T.);
#47967=ORIENTED_EDGE('',*,*,#34582,.T.);
#47968=ORIENTED_EDGE('',*,*,#34592,.T.);
#47969=ORIENTED_EDGE('',*,*,#34589,.T.);
#47970=ORIENTED_EDGE('',*,*,#34586,.T.);
#47971=ORIENTED_EDGE('',*,*,#34594,.T.);
#47972=ORIENTED_EDGE('',*,*,#34604,.T.);
#47973=ORIENTED_EDGE('',*,*,#34601,.T.);
#47974=ORIENTED_EDGE('',*,*,#34598,.T.);
#47975=ORIENTED_EDGE('',*,*,#34606,.T.);
#47976=ORIENTED_EDGE('',*,*,#34616,.T.);
#47977=ORIENTED_EDGE('',*,*,#34613,.T.);
#47978=ORIENTED_EDGE('',*,*,#34610,.T.);
#47979=ORIENTED_EDGE('',*,*,#34618,.T.);
#47980=ORIENTED_EDGE('',*,*,#34628,.T.);
#47981=ORIENTED_EDGE('',*,*,#34625,.T.);
#47982=ORIENTED_EDGE('',*,*,#34622,.T.);
#47983=ORIENTED_EDGE('',*,*,#34630,.T.);
#47984=ORIENTED_EDGE('',*,*,#34640,.T.);
#47985=ORIENTED_EDGE('',*,*,#34637,.T.);
#47986=ORIENTED_EDGE('',*,*,#34634,.T.);
#47987=ORIENTED_EDGE('',*,*,#34642,.T.);
#47988=ORIENTED_EDGE('',*,*,#34652,.T.);
#47989=ORIENTED_EDGE('',*,*,#34649,.T.);
#47990=ORIENTED_EDGE('',*,*,#34646,.T.);
#47991=ORIENTED_EDGE('',*,*,#34654,.T.);
#47992=ORIENTED_EDGE('',*,*,#34664,.T.);
#47993=ORIENTED_EDGE('',*,*,#34661,.T.);
#47994=ORIENTED_EDGE('',*,*,#34658,.T.);
#47995=ORIENTED_EDGE('',*,*,#34666,.T.);
#47996=ORIENTED_EDGE('',*,*,#34676,.T.);
#47997=ORIENTED_EDGE('',*,*,#34673,.T.);
#47998=ORIENTED_EDGE('',*,*,#34670,.T.);
#47999=ORIENTED_EDGE('',*,*,#34678,.T.);
#48000=ORIENTED_EDGE('',*,*,#34688,.T.);
#48001=ORIENTED_EDGE('',*,*,#34685,.T.);
#48002=ORIENTED_EDGE('',*,*,#34682,.T.);
#48003=ORIENTED_EDGE('',*,*,#34690,.T.);
#48004=ORIENTED_EDGE('',*,*,#34700,.T.);
#48005=ORIENTED_EDGE('',*,*,#34697,.T.);
#48006=ORIENTED_EDGE('',*,*,#34694,.T.);
#48007=ORIENTED_EDGE('',*,*,#34702,.T.);
#48008=ORIENTED_EDGE('',*,*,#34712,.T.);
#48009=ORIENTED_EDGE('',*,*,#34709,.T.);
#48010=ORIENTED_EDGE('',*,*,#34706,.T.);
#48011=ORIENTED_EDGE('',*,*,#34714,.T.);
#48012=ORIENTED_EDGE('',*,*,#34724,.T.);
#48013=ORIENTED_EDGE('',*,*,#34721,.T.);
#48014=ORIENTED_EDGE('',*,*,#34718,.T.);
#48015=ORIENTED_EDGE('',*,*,#34726,.T.);
#48016=ORIENTED_EDGE('',*,*,#34736,.T.);
#48017=ORIENTED_EDGE('',*,*,#34733,.T.);
#48018=ORIENTED_EDGE('',*,*,#34730,.T.);
#48019=ORIENTED_EDGE('',*,*,#34738,.T.);
#48020=ORIENTED_EDGE('',*,*,#34748,.T.);
#48021=ORIENTED_EDGE('',*,*,#34745,.T.);
#48022=ORIENTED_EDGE('',*,*,#34742,.T.);
#48023=ORIENTED_EDGE('',*,*,#34750,.T.);
#48024=ORIENTED_EDGE('',*,*,#34760,.T.);
#48025=ORIENTED_EDGE('',*,*,#34757,.T.);
#48026=ORIENTED_EDGE('',*,*,#34754,.T.);
#48027=ORIENTED_EDGE('',*,*,#34762,.T.);
#48028=ORIENTED_EDGE('',*,*,#34772,.T.);
#48029=ORIENTED_EDGE('',*,*,#34769,.T.);
#48030=ORIENTED_EDGE('',*,*,#34766,.T.);
#48031=ORIENTED_EDGE('',*,*,#34774,.T.);
#48032=ORIENTED_EDGE('',*,*,#34784,.T.);
#48033=ORIENTED_EDGE('',*,*,#34781,.T.);
#48034=ORIENTED_EDGE('',*,*,#34778,.T.);
#48035=ORIENTED_EDGE('',*,*,#34786,.T.);
#48036=ORIENTED_EDGE('',*,*,#34796,.T.);
#48037=ORIENTED_EDGE('',*,*,#34793,.T.);
#48038=ORIENTED_EDGE('',*,*,#34790,.T.);
#48039=ORIENTED_EDGE('',*,*,#34798,.T.);
#48040=ORIENTED_EDGE('',*,*,#34808,.T.);
#48041=ORIENTED_EDGE('',*,*,#34805,.T.);
#48042=ORIENTED_EDGE('',*,*,#34802,.T.);
#48043=ORIENTED_EDGE('',*,*,#34810,.T.);
#48044=ORIENTED_EDGE('',*,*,#34820,.T.);
#48045=ORIENTED_EDGE('',*,*,#34817,.T.);
#48046=ORIENTED_EDGE('',*,*,#34814,.T.);
#48047=ORIENTED_EDGE('',*,*,#34822,.T.);
#48048=ORIENTED_EDGE('',*,*,#34832,.T.);
#48049=ORIENTED_EDGE('',*,*,#34829,.T.);
#48050=ORIENTED_EDGE('',*,*,#34826,.T.);
#48051=ORIENTED_EDGE('',*,*,#34834,.T.);
#48052=ORIENTED_EDGE('',*,*,#34844,.T.);
#48053=ORIENTED_EDGE('',*,*,#34841,.T.);
#48054=ORIENTED_EDGE('',*,*,#34838,.T.);
#48055=ORIENTED_EDGE('',*,*,#34846,.T.);
#48056=ORIENTED_EDGE('',*,*,#34856,.T.);
#48057=ORIENTED_EDGE('',*,*,#34853,.T.);
#48058=ORIENTED_EDGE('',*,*,#34850,.T.);
#48059=ORIENTED_EDGE('',*,*,#32620,.T.);
#48060=ORIENTED_EDGE('',*,*,#32684,.T.);
#48061=ORIENTED_EDGE('',*,*,#32681,.T.);
#48062=ORIENTED_EDGE('',*,*,#32678,.T.);
#48063=ORIENTED_EDGE('',*,*,#32675,.T.);
#48064=ORIENTED_EDGE('',*,*,#32672,.T.);
#48065=ORIENTED_EDGE('',*,*,#32669,.T.);
#48066=ORIENTED_EDGE('',*,*,#32666,.T.);
#48067=ORIENTED_EDGE('',*,*,#32663,.T.);
#48068=ORIENTED_EDGE('',*,*,#32660,.T.);
#48069=ORIENTED_EDGE('',*,*,#32657,.T.);
#48070=ORIENTED_EDGE('',*,*,#32654,.T.);
#48071=ORIENTED_EDGE('',*,*,#32651,.T.);
#48072=ORIENTED_EDGE('',*,*,#32648,.T.);
#48073=ORIENTED_EDGE('',*,*,#32645,.T.);
#48074=ORIENTED_EDGE('',*,*,#32642,.T.);
#48075=ORIENTED_EDGE('',*,*,#32639,.T.);
#48076=ORIENTED_EDGE('',*,*,#32636,.T.);
#48077=ORIENTED_EDGE('',*,*,#32633,.T.);
#48078=ORIENTED_EDGE('',*,*,#32630,.T.);
#48079=ORIENTED_EDGE('',*,*,#32627,.T.);
#48080=ORIENTED_EDGE('',*,*,#32624,.T.);
#48081=ORIENTED_EDGE('',*,*,#32560,.T.);
#48082=ORIENTED_EDGE('',*,*,#32594,.T.);
#48083=ORIENTED_EDGE('',*,*,#32591,.T.);
#48084=ORIENTED_EDGE('',*,*,#32588,.T.);
#48085=ORIENTED_EDGE('',*,*,#32585,.T.);
#48086=ORIENTED_EDGE('',*,*,#32582,.T.);
#48087=ORIENTED_EDGE('',*,*,#32579,.T.);
#48088=ORIENTED_EDGE('',*,*,#32576,.T.);
#48089=ORIENTED_EDGE('',*,*,#32573,.T.);
#48090=ORIENTED_EDGE('',*,*,#32570,.T.);
#48091=ORIENTED_EDGE('',*,*,#32567,.T.);
#48092=ORIENTED_EDGE('',*,*,#32564,.T.);
#48093=ORIENTED_EDGE('',*,*,#32344,.T.);
#48094=ORIENTED_EDGE('',*,*,#32375,.T.);
#48095=ORIENTED_EDGE('',*,*,#32372,.T.);
#48096=ORIENTED_EDGE('',*,*,#32369,.T.);
#48097=ORIENTED_EDGE('',*,*,#32366,.T.);
#48098=ORIENTED_EDGE('',*,*,#32363,.T.);
#48099=ORIENTED_EDGE('',*,*,#32360,.T.);
#48100=ORIENTED_EDGE('',*,*,#32357,.T.);
#48101=ORIENTED_EDGE('',*,*,#32354,.T.);
#48102=ORIENTED_EDGE('',*,*,#32351,.T.);
#48103=ORIENTED_EDGE('',*,*,#32348,.T.);
#48104=ORIENTED_EDGE('',*,*,#32308,.T.);
#48105=ORIENTED_EDGE('',*,*,#32342,.T.);
#48106=ORIENTED_EDGE('',*,*,#32339,.T.);
#48107=ORIENTED_EDGE('',*,*,#32336,.T.);
#48108=ORIENTED_EDGE('',*,*,#32333,.T.);
#48109=ORIENTED_EDGE('',*,*,#32330,.T.);
#48110=ORIENTED_EDGE('',*,*,#32327,.T.);
#48111=ORIENTED_EDGE('',*,*,#32324,.T.);
#48112=ORIENTED_EDGE('',*,*,#32321,.T.);
#48113=ORIENTED_EDGE('',*,*,#32318,.T.);
#48114=ORIENTED_EDGE('',*,*,#32315,.T.);
#48115=ORIENTED_EDGE('',*,*,#32312,.T.);
#48116=ORIENTED_EDGE('',*,*,#32074,.T.);
#48117=ORIENTED_EDGE('',*,*,#32138,.T.);
#48118=ORIENTED_EDGE('',*,*,#32135,.T.);
#48119=ORIENTED_EDGE('',*,*,#32132,.T.);
#48120=ORIENTED_EDGE('',*,*,#32129,.T.);
#48121=ORIENTED_EDGE('',*,*,#32126,.T.);
#48122=ORIENTED_EDGE('',*,*,#32123,.T.);
#48123=ORIENTED_EDGE('',*,*,#32120,.T.);
#48124=ORIENTED_EDGE('',*,*,#32117,.T.);
#48125=ORIENTED_EDGE('',*,*,#32114,.T.);
#48126=ORIENTED_EDGE('',*,*,#32111,.T.);
#48127=ORIENTED_EDGE('',*,*,#32108,.T.);
#48128=ORIENTED_EDGE('',*,*,#32105,.T.);
#48129=ORIENTED_EDGE('',*,*,#32102,.T.);
#48130=ORIENTED_EDGE('',*,*,#32099,.T.);
#48131=ORIENTED_EDGE('',*,*,#32096,.T.);
#48132=ORIENTED_EDGE('',*,*,#32093,.T.);
#48133=ORIENTED_EDGE('',*,*,#32090,.T.);
#48134=ORIENTED_EDGE('',*,*,#32087,.T.);
#48135=ORIENTED_EDGE('',*,*,#32084,.T.);
#48136=ORIENTED_EDGE('',*,*,#32081,.T.);
#48137=ORIENTED_EDGE('',*,*,#32078,.T.);
#48138=ORIENTED_EDGE('',*,*,#32038,.T.);
#48139=ORIENTED_EDGE('',*,*,#32072,.T.);
#48140=ORIENTED_EDGE('',*,*,#32069,.T.);
#48141=ORIENTED_EDGE('',*,*,#32066,.T.);
#48142=ORIENTED_EDGE('',*,*,#32063,.T.);
#48143=ORIENTED_EDGE('',*,*,#32060,.T.);
#48144=ORIENTED_EDGE('',*,*,#32057,.T.);
#48145=ORIENTED_EDGE('',*,*,#32054,.T.);
#48146=ORIENTED_EDGE('',*,*,#32051,.T.);
#48147=ORIENTED_EDGE('',*,*,#32048,.T.);
#48148=ORIENTED_EDGE('',*,*,#32045,.T.);
#48149=ORIENTED_EDGE('',*,*,#32042,.T.);
#48150=ORIENTED_EDGE('',*,*,#31822,.T.);
#48151=ORIENTED_EDGE('',*,*,#31910,.T.);
#48152=ORIENTED_EDGE('',*,*,#31907,.T.);
#48153=ORIENTED_EDGE('',*,*,#31904,.T.);
#48154=ORIENTED_EDGE('',*,*,#31901,.T.);
#48155=ORIENTED_EDGE('',*,*,#31898,.T.);
#48156=ORIENTED_EDGE('',*,*,#31895,.T.);
#48157=ORIENTED_EDGE('',*,*,#31892,.T.);
#48158=ORIENTED_EDGE('',*,*,#31889,.T.);
#48159=ORIENTED_EDGE('',*,*,#31886,.T.);
#48160=ORIENTED_EDGE('',*,*,#31883,.T.);
#48161=ORIENTED_EDGE('',*,*,#31880,.T.);
#48162=ORIENTED_EDGE('',*,*,#31877,.T.);
#48163=ORIENTED_EDGE('',*,*,#31874,.T.);
#48164=ORIENTED_EDGE('',*,*,#31871,.T.);
#48165=ORIENTED_EDGE('',*,*,#31868,.T.);
#48166=ORIENTED_EDGE('',*,*,#31865,.T.);
#48167=ORIENTED_EDGE('',*,*,#31862,.T.);
#48168=ORIENTED_EDGE('',*,*,#31859,.T.);
#48169=ORIENTED_EDGE('',*,*,#31856,.T.);
#48170=ORIENTED_EDGE('',*,*,#31853,.T.);
#48171=ORIENTED_EDGE('',*,*,#31850,.T.);
#48172=ORIENTED_EDGE('',*,*,#31847,.T.);
#48173=ORIENTED_EDGE('',*,*,#31844,.T.);
#48174=ORIENTED_EDGE('',*,*,#31841,.T.);
#48175=ORIENTED_EDGE('',*,*,#31838,.T.);
#48176=ORIENTED_EDGE('',*,*,#31835,.T.);
#48177=ORIENTED_EDGE('',*,*,#31832,.T.);
#48178=ORIENTED_EDGE('',*,*,#31829,.T.);
#48179=ORIENTED_EDGE('',*,*,#31826,.T.);
#48180=ORIENTED_EDGE('',*,*,#31786,.T.);
#48181=ORIENTED_EDGE('',*,*,#31820,.T.);
#48182=ORIENTED_EDGE('',*,*,#31817,.T.);
#48183=ORIENTED_EDGE('',*,*,#31814,.T.);
#48184=ORIENTED_EDGE('',*,*,#31811,.T.);
#48185=ORIENTED_EDGE('',*,*,#31808,.T.);
#48186=ORIENTED_EDGE('',*,*,#31805,.T.);
#48187=ORIENTED_EDGE('',*,*,#31802,.T.);
#48188=ORIENTED_EDGE('',*,*,#31799,.T.);
#48189=ORIENTED_EDGE('',*,*,#31796,.T.);
#48190=ORIENTED_EDGE('',*,*,#31793,.T.);
#48191=ORIENTED_EDGE('',*,*,#31790,.T.);
#48192=ORIENTED_EDGE('',*,*,#31609,.T.);
#48193=ORIENTED_EDGE('',*,*,#31634,.T.);
#48194=ORIENTED_EDGE('',*,*,#31631,.T.);
#48195=ORIENTED_EDGE('',*,*,#31628,.T.);
#48196=ORIENTED_EDGE('',*,*,#31625,.T.);
#48197=ORIENTED_EDGE('',*,*,#31622,.T.);
#48198=ORIENTED_EDGE('',*,*,#31619,.T.);
#48199=ORIENTED_EDGE('',*,*,#31616,.T.);
#48200=ORIENTED_EDGE('',*,*,#31613,.T.);
#48201=ORIENTED_EDGE('',*,*,#31573,.T.);
#48202=ORIENTED_EDGE('',*,*,#31607,.T.);
#48203=ORIENTED_EDGE('',*,*,#31604,.T.);
#48204=ORIENTED_EDGE('',*,*,#31601,.T.);
#48205=ORIENTED_EDGE('',*,*,#31598,.T.);
#48206=ORIENTED_EDGE('',*,*,#31595,.T.);
#48207=ORIENTED_EDGE('',*,*,#31592,.T.);
#48208=ORIENTED_EDGE('',*,*,#31589,.T.);
#48209=ORIENTED_EDGE('',*,*,#31586,.T.);
#48210=ORIENTED_EDGE('',*,*,#31583,.T.);
#48211=ORIENTED_EDGE('',*,*,#31580,.T.);
#48212=ORIENTED_EDGE('',*,*,#31577,.T.);
#48213=ORIENTED_EDGE('',*,*,#31462,.T.);
#48214=ORIENTED_EDGE('',*,*,#31487,.T.);
#48215=ORIENTED_EDGE('',*,*,#31484,.T.);
#48216=ORIENTED_EDGE('',*,*,#31481,.T.);
#48217=ORIENTED_EDGE('',*,*,#31478,.T.);
#48218=ORIENTED_EDGE('',*,*,#31475,.T.);
#48219=ORIENTED_EDGE('',*,*,#31472,.T.);
#48220=ORIENTED_EDGE('',*,*,#31469,.T.);
#48221=ORIENTED_EDGE('',*,*,#31466,.T.);
#48222=ORIENTED_EDGE('',*,*,#31426,.T.);
#48223=ORIENTED_EDGE('',*,*,#31460,.T.);
#48224=ORIENTED_EDGE('',*,*,#31457,.T.);
#48225=ORIENTED_EDGE('',*,*,#31454,.T.);
#48226=ORIENTED_EDGE('',*,*,#31451,.T.);
#48227=ORIENTED_EDGE('',*,*,#31448,.T.);
#48228=ORIENTED_EDGE('',*,*,#31445,.T.);
#48229=ORIENTED_EDGE('',*,*,#31442,.T.);
#48230=ORIENTED_EDGE('',*,*,#31439,.T.);
#48231=ORIENTED_EDGE('',*,*,#31436,.T.);
#48232=ORIENTED_EDGE('',*,*,#31433,.T.);
#48233=ORIENTED_EDGE('',*,*,#31430,.T.);
#48234=ORIENTED_EDGE('',*,*,#31186,.T.);
#48235=ORIENTED_EDGE('',*,*,#31274,.T.);
#48236=ORIENTED_EDGE('',*,*,#31271,.T.);
#48237=ORIENTED_EDGE('',*,*,#31268,.T.);
#48238=ORIENTED_EDGE('',*,*,#31265,.T.);
#48239=ORIENTED_EDGE('',*,*,#31262,.T.);
#48240=ORIENTED_EDGE('',*,*,#31259,.T.);
#48241=ORIENTED_EDGE('',*,*,#31256,.T.);
#48242=ORIENTED_EDGE('',*,*,#31253,.T.);
#48243=ORIENTED_EDGE('',*,*,#31250,.T.);
#48244=ORIENTED_EDGE('',*,*,#31247,.T.);
#48245=ORIENTED_EDGE('',*,*,#31244,.T.);
#48246=ORIENTED_EDGE('',*,*,#31241,.T.);
#48247=ORIENTED_EDGE('',*,*,#31238,.T.);
#48248=ORIENTED_EDGE('',*,*,#31235,.T.);
#48249=ORIENTED_EDGE('',*,*,#31232,.T.);
#48250=ORIENTED_EDGE('',*,*,#31229,.T.);
#48251=ORIENTED_EDGE('',*,*,#31226,.T.);
#48252=ORIENTED_EDGE('',*,*,#31223,.T.);
#48253=ORIENTED_EDGE('',*,*,#31220,.T.);
#48254=ORIENTED_EDGE('',*,*,#31217,.T.);
#48255=ORIENTED_EDGE('',*,*,#31214,.T.);
#48256=ORIENTED_EDGE('',*,*,#31211,.T.);
#48257=ORIENTED_EDGE('',*,*,#31208,.T.);
#48258=ORIENTED_EDGE('',*,*,#31205,.T.);
#48259=ORIENTED_EDGE('',*,*,#31202,.T.);
#48260=ORIENTED_EDGE('',*,*,#31199,.T.);
#48261=ORIENTED_EDGE('',*,*,#31196,.T.);
#48262=ORIENTED_EDGE('',*,*,#31193,.T.);
#48263=ORIENTED_EDGE('',*,*,#31190,.T.);
#48264=ORIENTED_EDGE('',*,*,#31150,.T.);
#48265=ORIENTED_EDGE('',*,*,#31184,.T.);
#48266=ORIENTED_EDGE('',*,*,#31181,.T.);
#48267=ORIENTED_EDGE('',*,*,#31178,.T.);
#48268=ORIENTED_EDGE('',*,*,#31175,.T.);
#48269=ORIENTED_EDGE('',*,*,#31172,.T.);
#48270=ORIENTED_EDGE('',*,*,#31169,.T.);
#48271=ORIENTED_EDGE('',*,*,#31166,.T.);
#48272=ORIENTED_EDGE('',*,*,#31163,.T.);
#48273=ORIENTED_EDGE('',*,*,#31160,.T.);
#48274=ORIENTED_EDGE('',*,*,#31157,.T.);
#48275=ORIENTED_EDGE('',*,*,#31154,.T.);
#48276=ORIENTED_EDGE('',*,*,#30958,.T.);
#48277=ORIENTED_EDGE('',*,*,#31022,.T.);
#48278=ORIENTED_EDGE('',*,*,#31019,.T.);
#48279=ORIENTED_EDGE('',*,*,#31016,.T.);
#48280=ORIENTED_EDGE('',*,*,#31013,.T.);
#48281=ORIENTED_EDGE('',*,*,#31010,.T.);
#48282=ORIENTED_EDGE('',*,*,#31007,.T.);
#48283=ORIENTED_EDGE('',*,*,#31004,.T.);
#48284=ORIENTED_EDGE('',*,*,#31001,.T.);
#48285=ORIENTED_EDGE('',*,*,#30998,.T.);
#48286=ORIENTED_EDGE('',*,*,#30995,.T.);
#48287=ORIENTED_EDGE('',*,*,#30992,.T.);
#48288=ORIENTED_EDGE('',*,*,#30989,.T.);
#48289=ORIENTED_EDGE('',*,*,#30986,.T.);
#48290=ORIENTED_EDGE('',*,*,#30983,.T.);
#48291=ORIENTED_EDGE('',*,*,#30980,.T.);
#48292=ORIENTED_EDGE('',*,*,#30977,.T.);
#48293=ORIENTED_EDGE('',*,*,#30974,.T.);
#48294=ORIENTED_EDGE('',*,*,#30971,.T.);
#48295=ORIENTED_EDGE('',*,*,#30968,.T.);
#48296=ORIENTED_EDGE('',*,*,#30965,.T.);
#48297=ORIENTED_EDGE('',*,*,#30962,.T.);
#48298=ORIENTED_EDGE('',*,*,#30922,.T.);
#48299=ORIENTED_EDGE('',*,*,#30956,.T.);
#48300=ORIENTED_EDGE('',*,*,#30953,.T.);
#48301=ORIENTED_EDGE('',*,*,#30950,.T.);
#48302=ORIENTED_EDGE('',*,*,#30947,.T.);
#48303=ORIENTED_EDGE('',*,*,#30944,.T.);
#48304=ORIENTED_EDGE('',*,*,#30941,.T.);
#48305=ORIENTED_EDGE('',*,*,#30938,.T.);
#48306=ORIENTED_EDGE('',*,*,#30935,.T.);
#48307=ORIENTED_EDGE('',*,*,#30932,.T.);
#48308=ORIENTED_EDGE('',*,*,#30929,.T.);
#48309=ORIENTED_EDGE('',*,*,#30926,.T.);
#48310=ORIENTED_EDGE('',*,*,#30721,.T.);
#48311=ORIENTED_EDGE('',*,*,#30752,.T.);
#48312=ORIENTED_EDGE('',*,*,#30749,.T.);
#48313=ORIENTED_EDGE('',*,*,#30746,.T.);
#48314=ORIENTED_EDGE('',*,*,#30743,.T.);
#48315=ORIENTED_EDGE('',*,*,#30740,.T.);
#48316=ORIENTED_EDGE('',*,*,#30737,.T.);
#48317=ORIENTED_EDGE('',*,*,#30734,.T.);
#48318=ORIENTED_EDGE('',*,*,#30731,.T.);
#48319=ORIENTED_EDGE('',*,*,#30728,.T.);
#48320=ORIENTED_EDGE('',*,*,#30725,.T.);
#48321=ORIENTED_EDGE('',*,*,#30685,.T.);
#48322=ORIENTED_EDGE('',*,*,#30719,.T.);
#48323=ORIENTED_EDGE('',*,*,#30716,.T.);
#48324=ORIENTED_EDGE('',*,*,#30713,.T.);
#48325=ORIENTED_EDGE('',*,*,#30710,.T.);
#48326=ORIENTED_EDGE('',*,*,#30707,.T.);
#48327=ORIENTED_EDGE('',*,*,#30704,.T.);
#48328=ORIENTED_EDGE('',*,*,#30701,.T.);
#48329=ORIENTED_EDGE('',*,*,#30698,.T.);
#48330=ORIENTED_EDGE('',*,*,#30695,.T.);
#48331=ORIENTED_EDGE('',*,*,#30692,.T.);
#48332=ORIENTED_EDGE('',*,*,#30689,.T.);
#48333=ORIENTED_EDGE('',*,*,#30436,.T.);
#48334=ORIENTED_EDGE('',*,*,#30500,.T.);
#48335=ORIENTED_EDGE('',*,*,#30497,.T.);
#48336=ORIENTED_EDGE('',*,*,#30494,.T.);
#48337=ORIENTED_EDGE('',*,*,#30491,.T.);
#48338=ORIENTED_EDGE('',*,*,#30488,.T.);
#48339=ORIENTED_EDGE('',*,*,#30485,.T.);
#48340=ORIENTED_EDGE('',*,*,#30482,.T.);
#48341=ORIENTED_EDGE('',*,*,#30479,.T.);
#48342=ORIENTED_EDGE('',*,*,#30476,.T.);
#48343=ORIENTED_EDGE('',*,*,#30473,.T.);
#48344=ORIENTED_EDGE('',*,*,#30470,.T.);
#48345=ORIENTED_EDGE('',*,*,#30467,.T.);
#48346=ORIENTED_EDGE('',*,*,#30464,.T.);
#48347=ORIENTED_EDGE('',*,*,#30461,.T.);
#48348=ORIENTED_EDGE('',*,*,#30458,.T.);
#48349=ORIENTED_EDGE('',*,*,#30455,.T.);
#48350=ORIENTED_EDGE('',*,*,#30452,.T.);
#48351=ORIENTED_EDGE('',*,*,#30449,.T.);
#48352=ORIENTED_EDGE('',*,*,#30446,.T.);
#48353=ORIENTED_EDGE('',*,*,#30443,.T.);
#48354=ORIENTED_EDGE('',*,*,#30440,.T.);
#48355=ORIENTED_EDGE('',*,*,#30376,.T.);
#48356=ORIENTED_EDGE('',*,*,#30410,.T.);
#48357=ORIENTED_EDGE('',*,*,#30407,.T.);
#48358=ORIENTED_EDGE('',*,*,#30404,.T.);
#48359=ORIENTED_EDGE('',*,*,#30401,.T.);
#48360=ORIENTED_EDGE('',*,*,#30398,.T.);
#48361=ORIENTED_EDGE('',*,*,#30395,.T.);
#48362=ORIENTED_EDGE('',*,*,#30392,.T.);
#48363=ORIENTED_EDGE('',*,*,#30389,.T.);
#48364=ORIENTED_EDGE('',*,*,#30386,.T.);
#48365=ORIENTED_EDGE('',*,*,#30383,.T.);
#48366=ORIENTED_EDGE('',*,*,#30380,.T.);
#48367=ORIENTED_EDGE('',*,*,#35038,.F.);
#48368=ORIENTED_EDGE('',*,*,#35053,.T.);
#48369=ORIENTED_EDGE('',*,*,#35054,.F.);
#48370=ORIENTED_EDGE('',*,*,#35051,.T.);
#48371=ORIENTED_EDGE('',*,*,#35040,.F.);
#48372=ORIENTED_EDGE('',*,*,#35006,.T.);
#48373=ORIENTED_EDGE('',*,*,#35055,.F.);
#48374=ORIENTED_EDGE('',*,*,#35053,.F.);
#48375=ORIENTED_EDGE('',*,*,#34911,.T.);
#48376=ORIENTED_EDGE('',*,*,#34949,.T.);
#48377=ORIENTED_EDGE('',*,*,#34945,.T.);
#48378=ORIENTED_EDGE('',*,*,#34937,.T.);
#48379=ORIENTED_EDGE('',*,*,#35056,.T.);
#48380=ORIENTED_EDGE('',*,*,#35057,.T.);
#48381=ORIENTED_EDGE('',*,*,#34886,.T.);
#48382=ORIENTED_EDGE('',*,*,#35058,.T.);
#48383=ORIENTED_EDGE('',*,*,#34885,.T.);
#48384=ORIENTED_EDGE('',*,*,#35059,.T.);
#48385=ORIENTED_EDGE('',*,*,#35060,.T.);
#48386=ORIENTED_EDGE('',*,*,#35058,.F.);
#48387=ORIENTED_EDGE('',*,*,#34884,.T.);
#48388=ORIENTED_EDGE('',*,*,#35061,.T.);
#48389=ORIENTED_EDGE('',*,*,#35062,.T.);
#48390=ORIENTED_EDGE('',*,*,#35059,.F.);
#48391=ORIENTED_EDGE('',*,*,#34883,.T.);
#48392=ORIENTED_EDGE('',*,*,#35063,.T.);
#48393=ORIENTED_EDGE('',*,*,#35017,.T.);
#48394=ORIENTED_EDGE('',*,*,#35061,.F.);
#48395=ORIENTED_EDGE('',*,*,#34882,.T.);
#48396=ORIENTED_EDGE('',*,*,#35064,.T.);
#48397=ORIENTED_EDGE('',*,*,#34920,.T.);
#48398=ORIENTED_EDGE('',*,*,#35063,.F.);
#48399=ORIENTED_EDGE('',*,*,#34881,.T.);
#48400=ORIENTED_EDGE('',*,*,#35065,.T.);
#48401=ORIENTED_EDGE('',*,*,#35015,.T.);
#48402=ORIENTED_EDGE('',*,*,#35064,.F.);
#48403=ORIENTED_EDGE('',*,*,#34880,.T.);
#48404=ORIENTED_EDGE('',*,*,#35066,.T.);
#48405=ORIENTED_EDGE('',*,*,#35014,.T.);
#48406=ORIENTED_EDGE('',*,*,#35065,.F.);
#48407=ORIENTED_EDGE('',*,*,#34879,.T.);
#48408=ORIENTED_EDGE('',*,*,#35067,.T.);
#48409=ORIENTED_EDGE('',*,*,#35012,.T.);
#48410=ORIENTED_EDGE('',*,*,#35066,.F.);
#48411=ORIENTED_EDGE('',*,*,#34878,.T.);
#48412=ORIENTED_EDGE('',*,*,#35004,.T.);
#48413=ORIENTED_EDGE('',*,*,#35010,.T.);
#48414=ORIENTED_EDGE('',*,*,#35067,.F.);
#48415=ORIENTED_EDGE('',*,*,#35055,.T.);
#48416=ORIENTED_EDGE('',*,*,#35005,.T.);
#48417=ORIENTED_EDGE('',*,*,#34876,.T.);
#48418=ORIENTED_EDGE('',*,*,#35068,.T.);
#48419=ORIENTED_EDGE('',*,*,#34875,.T.);
#48420=ORIENTED_EDGE('',*,*,#35069,.T.);
#48421=ORIENTED_EDGE('',*,*,#35054,.T.);
#48422=ORIENTED_EDGE('',*,*,#35068,.F.);
#48423=ORIENTED_EDGE('',*,*,#34874,.T.);
#48424=ORIENTED_EDGE('',*,*,#35070,.T.);
#48425=ORIENTED_EDGE('',*,*,#35052,.T.);
#48426=ORIENTED_EDGE('',*,*,#35069,.F.);
#48427=ORIENTED_EDGE('',*,*,#35050,.T.);
#48428=ORIENTED_EDGE('',*,*,#35070,.F.);
#48429=ORIENTED_EDGE('',*,*,#34873,.T.);
#48430=ORIENTED_EDGE('',*,*,#34900,.T.);
#48431=ORIENTED_EDGE('',*,*,#34862,.T.);
#48432=ORIENTED_EDGE('',*,*,#34892,.T.);
#48433=ORIENTED_EDGE('',*,*,#35071,.T.);
#48434=ORIENTED_EDGE('',*,*,#34955,.T.);
#48435=ORIENTED_EDGE('',*,*,#35048,.T.);
#48436=ORIENTED_EDGE('',*,*,#35071,.F.);
#48437=ORIENTED_EDGE('',*,*,#34891,.T.);
#48438=ORIENTED_EDGE('',*,*,#35072,.T.);
#48439=ORIENTED_EDGE('',*,*,#35047,.T.);
#48440=ORIENTED_EDGE('',*,*,#35072,.F.);
#48441=ORIENTED_EDGE('',*,*,#34890,.T.);
#48442=ORIENTED_EDGE('',*,*,#35073,.T.);
#48443=ORIENTED_EDGE('',*,*,#35045,.T.);
#48444=ORIENTED_EDGE('',*,*,#35073,.F.);
#48445=ORIENTED_EDGE('',*,*,#34889,.T.);
#48446=ORIENTED_EDGE('',*,*,#35074,.T.);
#48447=ORIENTED_EDGE('',*,*,#34888,.T.);
#48448=ORIENTED_EDGE('',*,*,#35075,.T.);
#48449=ORIENTED_EDGE('',*,*,#35042,.T.);
#48450=ORIENTED_EDGE('',*,*,#35074,.F.);
#48451=ORIENTED_EDGE('',*,*,#34859,.T.);
#48452=ORIENTED_EDGE('',*,*,#34898,.F.);
#48453=ORIENTED_EDGE('',*,*,#35028,.F.);
#48454=ORIENTED_EDGE('',*,*,#35025,.F.);
#48455=ORIENTED_EDGE('',*,*,#35022,.F.);
#48456=ORIENTED_EDGE('',*,*,#35020,.F.);
#48457=ORIENTED_EDGE('',*,*,#35076,.T.);
#48458=ORIENTED_EDGE('',*,*,#34996,.F.);
#48459=ORIENTED_EDGE('',*,*,#34993,.F.);
#48460=ORIENTED_EDGE('',*,*,#34990,.F.);
#48461=ORIENTED_EDGE('',*,*,#34986,.F.);
#48462=ORIENTED_EDGE('',*,*,#34999,.F.);
#48463=ORIENTED_EDGE('',*,*,#35001,.F.);
#48464=ORIENTED_EDGE('',*,*,#34983,.F.);
#48465=ORIENTED_EDGE('',*,*,#34980,.F.);
#48466=ORIENTED_EDGE('',*,*,#34978,.F.);
#48467=ORIENTED_EDGE('',*,*,#35008,.T.);
#48468=ORIENTED_EDGE('',*,*,#35039,.F.);
#48469=ORIENTED_EDGE('',*,*,#35036,.F.);
#48470=ORIENTED_EDGE('',*,*,#35033,.F.);
#48471=ORIENTED_EDGE('',*,*,#35030,.F.);
#48472=ORIENTED_EDGE('',*,*,#34893,.F.);
#48473=ORIENTED_EDGE('',*,*,#34869,.T.);
#48474=ORIENTED_EDGE('',*,*,#34871,.T.);
#48475=ORIENTED_EDGE('',*,*,#34992,.F.);
#48476=ORIENTED_EDGE('',*,*,#35077,.F.);
#48477=ORIENTED_EDGE('',*,*,#35062,.F.);
#48478=ORIENTED_EDGE('',*,*,#35016,.T.);
#48479=ORIENTED_EDGE('',*,*,#34997,.F.);
#48480=ORIENTED_EDGE('',*,*,#35076,.F.);
#48481=ORIENTED_EDGE('',*,*,#35019,.F.);
#48482=ORIENTED_EDGE('',*,*,#35043,.F.);
#48483=ORIENTED_EDGE('',*,*,#35075,.F.);
#48484=ORIENTED_EDGE('',*,*,#34887,.F.);
#48485=ORIENTED_EDGE('',*,*,#35057,.F.);
#48486=ORIENTED_EDGE('',*,*,#35078,.F.);
#48487=ORIENTED_EDGE('',*,*,#34995,.F.);
#48488=ORIENTED_EDGE('',*,*,#35079,.T.);
#48489=ORIENTED_EDGE('',*,*,#35060,.F.);
#48490=ORIENTED_EDGE('',*,*,#35077,.T.);
#48491=ORIENTED_EDGE('',*,*,#34998,.F.);
#48492=ORIENTED_EDGE('',*,*,#35078,.T.);
#48493=ORIENTED_EDGE('',*,*,#35056,.F.);
#48494=ORIENTED_EDGE('',*,*,#35079,.F.);
#56413=B_SPLINE_SURFACE_WITH_KNOTS('',2,1,((#76146,#76147),(#76148,#76149),
(#76150,#76151)),.UNSPECIFIED.,.F.,.F.,.F.,(3,3),(2,2),(0.,1.),(0.,0.0149999999999997),
 .UNSPECIFIED.);
#56414=B_SPLINE_SURFACE_WITH_KNOTS('',2,1,((#76164,#76165),(#76166,#76167),
(#76168,#76169)),.UNSPECIFIED.,.F.,.F.,.F.,(3,3),(2,2),(0.,1.),(0.,0.0149999999999997),
 .UNSPECIFIED.);
#56415=B_SPLINE_SURFACE_WITH_KNOTS('',2,1,((#76179,#76180),(#76181,#76182),
(#76183,#76184)),.UNSPECIFIED.,.F.,.F.,.F.,(3,3),(2,2),(0.,1.),(0.,0.0149999999999997),
 .UNSPECIFIED.);
#56416=B_SPLINE_SURFACE_WITH_KNOTS('',2,1,((#76194,#76195),(#76196,#76197),
(#76198,#76199)),.UNSPECIFIED.,.F.,.F.,.F.,(3,3),(2,2),(0.,1.),(0.,0.0149999999999997),
 .UNSPECIFIED.);
#56417=B_SPLINE_SURFACE_WITH_KNOTS('',2,1,((#76209,#76210),(#76211,#76212),
(#76213,#76214)),.UNSPECIFIED.,.F.,.F.,.F.,(3,3),(2,2),(0.,1.),(0.,0.0149999999999997),
 .UNSPECIFIED.);
#56418=B_SPLINE_SURFACE_WITH_KNOTS('',2,1,((#76224,#76225),(#76226,#76227),
(#76228,#76229)),.UNSPECIFIED.,.F.,.F.,.F.,(3,3),(2,2),(0.,1.),(0.,0.0149999999999997),
 .UNSPECIFIED.);
#56419=B_SPLINE_SURFACE_WITH_KNOTS('',2,1,((#76239,#76240),(#76241,#76242),
(#76243,#76244)),.UNSPECIFIED.,.F.,.F.,.F.,(3,3),(2,2),(0.,1.),(0.,0.0149999999999997),
 .UNSPECIFIED.);
#56420=B_SPLINE_SURFACE_WITH_KNOTS('',2,1,((#76254,#76255),(#76256,#76257),
(#76258,#76259)),.UNSPECIFIED.,.F.,.F.,.F.,(3,3),(2,2),(0.,1.),(0.,0.0149999999999997),
 .UNSPECIFIED.);
#56421=B_SPLINE_SURFACE_WITH_KNOTS('',2,1,((#76266,#76267),(#76268,#76269),
(#76270,#76271)),.UNSPECIFIED.,.F.,.F.,.F.,(3,3),(2,2),(0.,1.),(0.,0.0149999999999997),
 .UNSPECIFIED.);
#56422=B_SPLINE_SURFACE_WITH_KNOTS('',2,1,((#76284,#76285),(#76286,#76287),
(#76288,#76289)),.UNSPECIFIED.,.F.,.F.,.F.,(3,3),(2,2),(0.,1.),(0.,0.0149999999999997),
 .UNSPECIFIED.);
#56423=B_SPLINE_SURFACE_WITH_KNOTS('',2,1,((#76299,#76300),(#76301,#76302),
(#76303,#76304)),.UNSPECIFIED.,.F.,.F.,.F.,(3,3),(2,2),(0.,1.),(0.,0.0149999999999997),
 .UNSPECIFIED.);
#56424=B_SPLINE_SURFACE_WITH_KNOTS('',2,1,((#76314,#76315),(#76316,#76317),
(#76318,#76319)),.UNSPECIFIED.,.F.,.F.,.F.,(3,3),(2,2),(0.,1.),(0.,0.0149999999999997),
 .UNSPECIFIED.);
#56425=B_SPLINE_SURFACE_WITH_KNOTS('',2,1,((#76329,#76330),(#76331,#76332),
(#76333,#76334)),.UNSPECIFIED.,.F.,.F.,.F.,(3,3),(2,2),(0.,1.),(0.,0.0149999999999997),
 .UNSPECIFIED.);
#56426=B_SPLINE_SURFACE_WITH_KNOTS('',2,1,((#76344,#76345),(#76346,#76347),
(#76348,#76349)),.UNSPECIFIED.,.F.,.F.,.F.,(3,3),(2,2),(0.,1.),(0.,0.0149999999999997),
 .UNSPECIFIED.);
#56427=B_SPLINE_SURFACE_WITH_KNOTS('',2,1,((#76359,#76360),(#76361,#76362),
(#76363,#76364)),.UNSPECIFIED.,.F.,.F.,.F.,(3,3),(2,2),(0.,1.),(0.,0.0149999999999997),
 .UNSPECIFIED.);
#56428=B_SPLINE_SURFACE_WITH_KNOTS('',2,1,((#76374,#76375),(#76376,#76377),
(#76378,#76379)),.UNSPECIFIED.,.F.,.F.,.F.,(3,3),(2,2),(0.,1.),(0.,0.0149999999999997),
 .UNSPECIFIED.);
#56429=B_SPLINE_SURFACE_WITH_KNOTS('',2,1,((#76389,#76390),(#76391,#76392),
(#76393,#76394)),.UNSPECIFIED.,.F.,.F.,.F.,(3,3),(2,2),(0.,1.),(0.,0.0149999999999997),
 .UNSPECIFIED.);
#56430=B_SPLINE_SURFACE_WITH_KNOTS('',2,1,((#76404,#76405),(#76406,#76407),
(#76408,#76409)),.UNSPECIFIED.,.F.,.F.,.F.,(3,3),(2,2),(0.,1.),(0.,0.0149999999999997),
 .UNSPECIFIED.);
#56431=B_SPLINE_SURFACE_WITH_KNOTS('',2,1,((#76419,#76420),(#76421,#76422),
(#76423,#76424)),.UNSPECIFIED.,.F.,.F.,.F.,(3,3),(2,2),(0.,1.),(0.,0.0149999999999997),
 .UNSPECIFIED.);
#56432=B_SPLINE_SURFACE_WITH_KNOTS('',2,1,((#76434,#76435),(#76436,#76437),
(#76438,#76439)),.UNSPECIFIED.,.F.,.F.,.F.,(3,3),(2,2),(0.,1.),(0.,0.0149999999999997),
 .UNSPECIFIED.);
#56433=B_SPLINE_SURFACE_WITH_KNOTS('',2,1,((#76447,#76448),(#76449,#76450),
(#76451,#76452)),.UNSPECIFIED.,.F.,.F.,.F.,(3,3),(2,2),(0.,1.),(0.,0.0149999999999997),
 .UNSPECIFIED.);
#56434=B_SPLINE_SURFACE_WITH_KNOTS('',2,1,((#76465,#76466),(#76467,#76468),
(#76469,#76470)),.UNSPECIFIED.,.F.,.F.,.F.,(3,3),(2,2),(0.,1.),(0.,0.0149999999999997),
 .UNSPECIFIED.);
#56435=B_SPLINE_SURFACE_WITH_KNOTS('',2,1,((#76480,#76481),(#76482,#76483),
(#76484,#76485)),.UNSPECIFIED.,.F.,.F.,.F.,(3,3),(2,2),(0.,1.),(0.,0.0149999999999997),
 .UNSPECIFIED.);
#56436=B_SPLINE_SURFACE_WITH_KNOTS('',2,1,((#76495,#76496),(#76497,#76498),
(#76499,#76500)),.UNSPECIFIED.,.F.,.F.,.F.,(3,3),(2,2),(0.,1.),(0.,0.0149999999999997),
 .UNSPECIFIED.);
#56437=B_SPLINE_SURFACE_WITH_KNOTS('',2,1,((#76510,#76511),(#76512,#76513),
(#76514,#76515)),.UNSPECIFIED.,.F.,.F.,.F.,(3,3),(2,2),(0.,1.),(0.,0.0149999999999997),
 .UNSPECIFIED.);
#56438=B_SPLINE_SURFACE_WITH_KNOTS('',2,1,((#76525,#76526),(#76527,#76528),
(#76529,#76530)),.UNSPECIFIED.,.F.,.F.,.F.,(3,3),(2,2),(0.,1.),(0.,0.0149999999999997),
 .UNSPECIFIED.);
#56439=B_SPLINE_SURFACE_WITH_KNOTS('',2,1,((#76540,#76541),(#76542,#76543),
(#76544,#76545)),.UNSPECIFIED.,.F.,.F.,.F.,(3,3),(2,2),(0.,1.),(0.,0.0149999999999997),
 .UNSPECIFIED.);
#56440=B_SPLINE_SURFACE_WITH_KNOTS('',2,1,((#76555,#76556),(#76557,#76558),
(#76559,#76560)),.UNSPECIFIED.,.F.,.F.,.F.,(3,3),(2,2),(0.,1.),(0.,0.0149999999999997),
 .UNSPECIFIED.);
#56441=B_SPLINE_SURFACE_WITH_KNOTS('',2,1,((#76567,#76568),(#76569,#76570),
(#76571,#76572)),.UNSPECIFIED.,.F.,.F.,.F.,(3,3),(2,2),(0.,1.),(0.,0.0149999999999997),
 .UNSPECIFIED.);
#56442=B_SPLINE_SURFACE_WITH_KNOTS('',2,1,((#76585,#76586),(#76587,#76588),
(#76589,#76590)),.UNSPECIFIED.,.F.,.F.,.F.,(3,3),(2,2),(0.,1.),(0.,0.0149999999999997),
 .UNSPECIFIED.);
#56443=B_SPLINE_SURFACE_WITH_KNOTS('',2,1,((#76600,#76601),(#76602,#76603),
(#76604,#76605)),.UNSPECIFIED.,.F.,.F.,.F.,(3,3),(2,2),(0.,1.),(0.,0.0149999999999997),
 .UNSPECIFIED.);
#56444=B_SPLINE_SURFACE_WITH_KNOTS('',2,1,((#76615,#76616),(#76617,#76618),
(#76619,#76620)),.UNSPECIFIED.,.F.,.F.,.F.,(3,3),(2,2),(0.,1.),(0.,0.0149999999999997),
 .UNSPECIFIED.);
#56445=B_SPLINE_SURFACE_WITH_KNOTS('',2,1,((#76630,#76631),(#76632,#76633),
(#76634,#76635)),.UNSPECIFIED.,.F.,.F.,.F.,(3,3),(2,2),(0.,1.),(0.,0.0149999999999997),
 .UNSPECIFIED.);
#56446=B_SPLINE_SURFACE_WITH_KNOTS('',2,1,((#76645,#76646),(#76647,#76648),
(#76649,#76650)),.UNSPECIFIED.,.F.,.F.,.F.,(3,3),(2,2),(0.,1.),(0.,0.0149999999999997),
 .UNSPECIFIED.);
#56447=B_SPLINE_SURFACE_WITH_KNOTS('',2,1,((#76660,#76661),(#76662,#76663),
(#76664,#76665)),.UNSPECIFIED.,.F.,.F.,.F.,(3,3),(2,2),(0.,1.),(0.,0.0149999999999997),
 .UNSPECIFIED.);
#56448=B_SPLINE_SURFACE_WITH_KNOTS('',2,1,((#76675,#76676),(#76677,#76678),
(#76679,#76680)),.UNSPECIFIED.,.F.,.F.,.F.,(3,3),(2,2),(0.,1.),(0.,0.0149999999999997),
 .UNSPECIFIED.);
#56449=B_SPLINE_SURFACE_WITH_KNOTS('',2,1,((#76690,#76691),(#76692,#76693),
(#76694,#76695)),.UNSPECIFIED.,.F.,.F.,.F.,(3,3),(2,2),(0.,1.),(0.,0.0149999999999997),
 .UNSPECIFIED.);
#56450=B_SPLINE_SURFACE_WITH_KNOTS('',2,1,((#76705,#76706),(#76707,#76708),
(#76709,#76710)),.UNSPECIFIED.,.F.,.F.,.F.,(3,3),(2,2),(0.,1.),(0.,0.0149999999999997),
 .UNSPECIFIED.);
#56451=B_SPLINE_SURFACE_WITH_KNOTS('',2,1,((#76720,#76721),(#76722,#76723),
(#76724,#76725)),.UNSPECIFIED.,.F.,.F.,.F.,(3,3),(2,2),(0.,1.),(0.,0.0149999999999997),
 .UNSPECIFIED.);
#56452=B_SPLINE_SURFACE_WITH_KNOTS('',2,1,((#76735,#76736),(#76737,#76738),
(#76739,#76740)),.UNSPECIFIED.,.F.,.F.,.F.,(3,3),(2,2),(0.,1.),(0.,0.0149999999999997),
 .UNSPECIFIED.);
#56453=B_SPLINE_SURFACE_WITH_KNOTS('',2,1,((#76750,#76751),(#76752,#76753),
(#76754,#76755)),.UNSPECIFIED.,.F.,.F.,.F.,(3,3),(2,2),(0.,1.),(0.,0.0149999999999997),
 .UNSPECIFIED.);
#56454=B_SPLINE_SURFACE_WITH_KNOTS('',2,1,((#76765,#76766),(#76767,#76768),
(#76769,#76770)),.UNSPECIFIED.,.F.,.F.,.F.,(3,3),(2,2),(0.,1.),(0.,0.0149999999999997),
 .UNSPECIFIED.);
#56455=B_SPLINE_SURFACE_WITH_KNOTS('',2,1,((#76780,#76781),(#76782,#76783),
(#76784,#76785)),.UNSPECIFIED.,.F.,.F.,.F.,(3,3),(2,2),(0.,1.),(0.,0.0149999999999997),
 .UNSPECIFIED.);
#56456=B_SPLINE_SURFACE_WITH_KNOTS('',2,1,((#76795,#76796),(#76797,#76798),
(#76799,#76800)),.UNSPECIFIED.,.F.,.F.,.F.,(3,3),(2,2),(0.,1.),(0.,0.0149999999999997),
 .UNSPECIFIED.);
#56457=B_SPLINE_SURFACE_WITH_KNOTS('',2,1,((#76810,#76811),(#76812,#76813),
(#76814,#76815)),.UNSPECIFIED.,.F.,.F.,.F.,(3,3),(2,2),(0.,1.),(0.,0.0149999999999997),
 .UNSPECIFIED.);
#56458=B_SPLINE_SURFACE_WITH_KNOTS('',2,1,((#76825,#76826),(#76827,#76828),
(#76829,#76830)),.UNSPECIFIED.,.F.,.F.,.F.,(3,3),(2,2),(0.,1.),(0.,0.0149999999999997),
 .UNSPECIFIED.);
#56459=B_SPLINE_SURFACE_WITH_KNOTS('',2,1,((#76840,#76841),(#76842,#76843),
(#76844,#76845)),.UNSPECIFIED.,.F.,.F.,.F.,(3,3),(2,2),(0.,1.),(0.,0.0149999999999997),
 .UNSPECIFIED.);
#56460=B_SPLINE_SURFACE_WITH_KNOTS('',2,1,((#76855,#76856),(#76857,#76858),
(#76859,#76860)),.UNSPECIFIED.,.F.,.F.,.F.,(3,3),(2,2),(0.,1.),(0.,0.0149999999999997),
 .UNSPECIFIED.);
#56461=B_SPLINE_SURFACE_WITH_KNOTS('',2,1,((#76876,#76877),(#76878,#76879),
(#76880,#76881)),.UNSPECIFIED.,.F.,.F.,.F.,(3,3),(2,2),(0.,1.),(0.,0.0149999999999997),
 .UNSPECIFIED.);
#56462=B_SPLINE_SURFACE_WITH_KNOTS('',2,1,((#76891,#76892),(#76893,#76894),
(#76895,#76896)),.UNSPECIFIED.,.F.,.F.,.F.,(3,3),(2,2),(0.,1.),(0.,0.0149999999999997),
 .UNSPECIFIED.);
#56463=B_SPLINE_SURFACE_WITH_KNOTS('',2,1,((#76909,#76910),(#76911,#76912),
(#76913,#76914)),.UNSPECIFIED.,.F.,.F.,.F.,(3,3),(2,2),(0.,1.),(0.,0.0149999999999997),
 .UNSPECIFIED.);
#56464=B_SPLINE_SURFACE_WITH_KNOTS('',2,1,((#76924,#76925),(#76926,#76927),
(#76928,#76929)),.UNSPECIFIED.,.F.,.F.,.F.,(3,3),(2,2),(0.,1.),(0.,0.0149999999999997),
 .UNSPECIFIED.);
#56465=B_SPLINE_SURFACE_WITH_KNOTS('',2,1,((#76939,#76940),(#76941,#76942),
(#76943,#76944)),.UNSPECIFIED.,.F.,.F.,.F.,(3,3),(2,2),(0.,1.),(0.,0.0149999999999997),
 .UNSPECIFIED.);
#56466=B_SPLINE_SURFACE_WITH_KNOTS('',2,1,((#76954,#76955),(#76956,#76957),
(#76958,#76959)),.UNSPECIFIED.,.F.,.F.,.F.,(3,3),(2,2),(0.,1.),(0.,0.0149999999999997),
 .UNSPECIFIED.);
#56467=B_SPLINE_SURFACE_WITH_KNOTS('',2,1,((#76969,#76970),(#76971,#76972),
(#76973,#76974)),.UNSPECIFIED.,.F.,.F.,.F.,(3,3),(2,2),(0.,1.),(0.,0.0149999999999997),
 .UNSPECIFIED.);
#56468=B_SPLINE_SURFACE_WITH_KNOTS('',2,1,((#76984,#76985),(#76986,#76987),
(#76988,#76989)),.UNSPECIFIED.,.F.,.F.,.F.,(3,3),(2,2),(0.,1.),(0.,0.0149999999999997),
 .UNSPECIFIED.);
#56469=B_SPLINE_SURFACE_WITH_KNOTS('',2,1,((#76999,#77000),(#77001,#77002),
(#77003,#77004)),.UNSPECIFIED.,.F.,.F.,.F.,(3,3),(2,2),(0.,1.),(0.,0.0149999999999997),
 .UNSPECIFIED.);
#56470=B_SPLINE_SURFACE_WITH_KNOTS('',2,1,((#77011,#77012),(#77013,#77014),
(#77015,#77016)),.UNSPECIFIED.,.F.,.F.,.F.,(3,3),(2,2),(0.,1.),(0.,0.0149999999999997),
 .UNSPECIFIED.);
#56471=B_SPLINE_SURFACE_WITH_KNOTS('',2,1,((#77029,#77030),(#77031,#77032),
(#77033,#77034)),.UNSPECIFIED.,.F.,.F.,.F.,(3,3),(2,2),(0.,1.),(0.,0.0149999999999997),
 .UNSPECIFIED.);
#56472=B_SPLINE_SURFACE_WITH_KNOTS('',2,1,((#77044,#77045),(#77046,#77047),
(#77048,#77049)),.UNSPECIFIED.,.F.,.F.,.F.,(3,3),(2,2),(0.,1.),(0.,0.0149999999999997),
 .UNSPECIFIED.);
#56473=B_SPLINE_SURFACE_WITH_KNOTS('',2,1,((#77059,#77060),(#77061,#77062),
(#77063,#77064)),.UNSPECIFIED.,.F.,.F.,.F.,(3,3),(2,2),(0.,1.),(0.,0.0149999999999997),
 .UNSPECIFIED.);
#56474=B_SPLINE_SURFACE_WITH_KNOTS('',2,1,((#77074,#77075),(#77076,#77077),
(#77078,#77079)),.UNSPECIFIED.,.F.,.F.,.F.,(3,3),(2,2),(0.,1.),(0.,0.0149999999999997),
 .UNSPECIFIED.);
#56475=B_SPLINE_SURFACE_WITH_KNOTS('',2,1,((#77089,#77090),(#77091,#77092),
(#77093,#77094)),.UNSPECIFIED.,.F.,.F.,.F.,(3,3),(2,2),(0.,1.),(0.,0.0149999999999997),
 .UNSPECIFIED.);
#56476=B_SPLINE_SURFACE_WITH_KNOTS('',2,1,((#77104,#77105),(#77106,#77107),
(#77108,#77109)),.UNSPECIFIED.,.F.,.F.,.F.,(3,3),(2,2),(0.,1.),(0.,0.0149999999999997),
 .UNSPECIFIED.);
#56477=B_SPLINE_SURFACE_WITH_KNOTS('',2,1,((#77119,#77120),(#77121,#77122),
(#77123,#77124)),.UNSPECIFIED.,.F.,.F.,.F.,(3,3),(2,2),(0.,1.),(0.,0.0149999999999997),
 .UNSPECIFIED.);
#56478=B_SPLINE_SURFACE_WITH_KNOTS('',2,1,((#77134,#77135),(#77136,#77137),
(#77138,#77139)),.UNSPECIFIED.,.F.,.F.,.F.,(3,3),(2,2),(0.,1.),(0.,0.0149999999999997),
 .UNSPECIFIED.);
#56479=B_SPLINE_SURFACE_WITH_KNOTS('',2,1,((#77149,#77150),(#77151,#77152),
(#77153,#77154)),.UNSPECIFIED.,.F.,.F.,.F.,(3,3),(2,2),(0.,1.),(0.,0.0149999999999997),
 .UNSPECIFIED.);
#56480=B_SPLINE_SURFACE_WITH_KNOTS('',2,1,((#77164,#77165),(#77166,#77167),
(#77168,#77169)),.UNSPECIFIED.,.F.,.F.,.F.,(3,3),(2,2),(0.,1.),(0.,0.0149999999999997),
 .UNSPECIFIED.);
#56481=B_SPLINE_SURFACE_WITH_KNOTS('',2,1,((#77179,#77180),(#77181,#77182),
(#77183,#77184)),.UNSPECIFIED.,.F.,.F.,.F.,(3,3),(2,2),(0.,1.),(0.,0.0149999999999997),
 .UNSPECIFIED.);
#56482=B_SPLINE_SURFACE_WITH_KNOTS('',2,1,((#77192,#77193),(#77194,#77195),
(#77196,#77197)),.UNSPECIFIED.,.F.,.F.,.F.,(3,3),(2,2),(0.,1.),(0.,0.0149999999999997),
 .UNSPECIFIED.);
#56483=B_SPLINE_SURFACE_WITH_KNOTS('',2,1,((#77210,#77211),(#77212,#77213),
(#77214,#77215)),.UNSPECIFIED.,.F.,.F.,.F.,(3,3),(2,2),(0.,1.),(0.,0.0149999999999997),
 .UNSPECIFIED.);
#56484=B_SPLINE_SURFACE_WITH_KNOTS('',2,1,((#77225,#77226),(#77227,#77228),
(#77229,#77230)),.UNSPECIFIED.,.F.,.F.,.F.,(3,3),(2,2),(0.,1.),(0.,0.0149999999999997),
 .UNSPECIFIED.);
#56485=B_SPLINE_SURFACE_WITH_KNOTS('',2,1,((#77240,#77241),(#77242,#77243),
(#77244,#77245)),.UNSPECIFIED.,.F.,.F.,.F.,(3,3),(2,2),(0.,1.),(0.,0.0149999999999997),
 .UNSPECIFIED.);
#56486=B_SPLINE_SURFACE_WITH_KNOTS('',2,1,((#77255,#77256),(#77257,#77258),
(#77259,#77260)),.UNSPECIFIED.,.F.,.F.,.F.,(3,3),(2,2),(0.,1.),(0.,0.0149999999999997),
 .UNSPECIFIED.);
#56487=B_SPLINE_SURFACE_WITH_KNOTS('',2,1,((#77270,#77271),(#77272,#77273),
(#77274,#77275)),.UNSPECIFIED.,.F.,.F.,.F.,(3,3),(2,2),(0.,1.),(0.,0.0149999999999997),
 .UNSPECIFIED.);
#56488=B_SPLINE_SURFACE_WITH_KNOTS('',2,1,((#77285,#77286),(#77287,#77288),
(#77289,#77290)),.UNSPECIFIED.,.F.,.F.,.F.,(3,3),(2,2),(0.,1.),(0.,0.0149999999999997),
 .UNSPECIFIED.);
#56489=B_SPLINE_SURFACE_WITH_KNOTS('',2,1,((#77300,#77301),(#77302,#77303),
(#77304,#77305)),.UNSPECIFIED.,.F.,.F.,.F.,(3,3),(2,2),(0.,1.),(0.,0.0149999999999997),
 .UNSPECIFIED.);
#56490=B_SPLINE_SURFACE_WITH_KNOTS('',2,1,((#77312,#77313),(#77314,#77315),
(#77316,#77317)),.UNSPECIFIED.,.F.,.F.,.F.,(3,3),(2,2),(0.,1.),(0.,0.0149999999999997),
 .UNSPECIFIED.);
#56491=B_SPLINE_SURFACE_WITH_KNOTS('',2,1,((#77330,#77331),(#77332,#77333),
(#77334,#77335)),.UNSPECIFIED.,.F.,.F.,.F.,(3,3),(2,2),(0.,1.),(0.,0.0149999999999997),
 .UNSPECIFIED.);
#56492=B_SPLINE_SURFACE_WITH_KNOTS('',2,1,((#77345,#77346),(#77347,#77348),
(#77349,#77350)),.UNSPECIFIED.,.F.,.F.,.F.,(3,3),(2,2),(0.,1.),(0.,0.0149999999999997),
 .UNSPECIFIED.);
#56493=B_SPLINE_SURFACE_WITH_KNOTS('',2,1,((#77360,#77361),(#77362,#77363),
(#77364,#77365)),.UNSPECIFIED.,.F.,.F.,.F.,(3,3),(2,2),(0.,1.),(0.,0.0149999999999997),
 .UNSPECIFIED.);
#56494=B_SPLINE_SURFACE_WITH_KNOTS('',2,1,((#77375,#77376),(#77377,#77378),
(#77379,#77380)),.UNSPECIFIED.,.F.,.F.,.F.,(3,3),(2,2),(0.,1.),(0.,0.0149999999999997),
 .UNSPECIFIED.);
#56495=B_SPLINE_SURFACE_WITH_KNOTS('',2,1,((#77390,#77391),(#77392,#77393),
(#77394,#77395)),.UNSPECIFIED.,.F.,.F.,.F.,(3,3),(2,2),(0.,1.),(0.,0.0149999999999997),
 .UNSPECIFIED.);
#56496=B_SPLINE_SURFACE_WITH_KNOTS('',2,1,((#77405,#77406),(#77407,#77408),
(#77409,#77410)),.UNSPECIFIED.,.F.,.F.,.F.,(3,3),(2,2),(0.,1.),(0.,0.0149999999999997),
 .UNSPECIFIED.);
#56497=B_SPLINE_SURFACE_WITH_KNOTS('',2,1,((#77420,#77421),(#77422,#77423),
(#77424,#77425)),.UNSPECIFIED.,.F.,.F.,.F.,(3,3),(2,2),(0.,1.),(0.,0.0149999999999997),
 .UNSPECIFIED.);
#56498=B_SPLINE_SURFACE_WITH_KNOTS('',2,1,((#77435,#77436),(#77437,#77438),
(#77439,#77440)),.UNSPECIFIED.,.F.,.F.,.F.,(3,3),(2,2),(0.,1.),(0.,0.0149999999999997),
 .UNSPECIFIED.);
#56499=B_SPLINE_SURFACE_WITH_KNOTS('',2,1,((#77447,#77448),(#77449,#77450),
(#77451,#77452)),.UNSPECIFIED.,.F.,.F.,.F.,(3,3),(2,2),(0.,1.),(0.,0.0149999999999997),
 .UNSPECIFIED.);
#56500=B_SPLINE_SURFACE_WITH_KNOTS('',2,1,((#77465,#77466),(#77467,#77468),
(#77469,#77470)),.UNSPECIFIED.,.F.,.F.,.F.,(3,3),(2,2),(0.,1.),(0.,0.0149999999999997),
 .UNSPECIFIED.);
#56501=B_SPLINE_SURFACE_WITH_KNOTS('',2,1,((#77480,#77481),(#77482,#77483),
(#77484,#77485)),.UNSPECIFIED.,.F.,.F.,.F.,(3,3),(2,2),(0.,1.),(0.,0.0149999999999997),
 .UNSPECIFIED.);
#56502=B_SPLINE_SURFACE_WITH_KNOTS('',2,1,((#77495,#77496),(#77497,#77498),
(#77499,#77500)),.UNSPECIFIED.,.F.,.F.,.F.,(3,3),(2,2),(0.,1.),(0.,0.0149999999999997),
 .UNSPECIFIED.);
#56503=B_SPLINE_SURFACE_WITH_KNOTS('',2,1,((#77510,#77511),(#77512,#77513),
(#77514,#77515)),.UNSPECIFIED.,.F.,.F.,.F.,(3,3),(2,2),(0.,1.),(0.,0.0149999999999997),
 .UNSPECIFIED.);
#56504=B_SPLINE_SURFACE_WITH_KNOTS('',2,1,((#77525,#77526),(#77527,#77528),
(#77529,#77530)),.UNSPECIFIED.,.F.,.F.,.F.,(3,3),(2,2),(0.,1.),(0.,0.0149999999999997),
 .UNSPECIFIED.);
#56505=B_SPLINE_SURFACE_WITH_KNOTS('',2,1,((#77540,#77541),(#77542,#77543),
(#77544,#77545)),.UNSPECIFIED.,.F.,.F.,.F.,(3,3),(2,2),(0.,1.),(0.,0.0149999999999997),
 .UNSPECIFIED.);
#56506=B_SPLINE_SURFACE_WITH_KNOTS('',2,1,((#77555,#77556),(#77557,#77558),
(#77559,#77560)),.UNSPECIFIED.,.F.,.F.,.F.,(3,3),(2,2),(0.,1.),(0.,0.0149999999999997),
 .UNSPECIFIED.);
#56507=B_SPLINE_SURFACE_WITH_KNOTS('',2,1,((#77570,#77571),(#77572,#77573),
(#77574,#77575)),.UNSPECIFIED.,.F.,.F.,.F.,(3,3),(2,2),(0.,1.),(0.,0.0149999999999997),
 .UNSPECIFIED.);
#56508=B_SPLINE_SURFACE_WITH_KNOTS('',2,1,((#77585,#77586),(#77587,#77588),
(#77589,#77590)),.UNSPECIFIED.,.F.,.F.,.F.,(3,3),(2,2),(0.,1.),(0.,0.0149999999999997),
 .UNSPECIFIED.);
#56509=B_SPLINE_SURFACE_WITH_KNOTS('',2,1,((#77600,#77601),(#77602,#77603),
(#77604,#77605)),.UNSPECIFIED.,.F.,.F.,.F.,(3,3),(2,2),(0.,1.),(0.,0.0149999999999997),
 .UNSPECIFIED.);
#56510=B_SPLINE_SURFACE_WITH_KNOTS('',2,1,((#77615,#77616),(#77617,#77618),
(#77619,#77620)),.UNSPECIFIED.,.F.,.F.,.F.,(3,3),(2,2),(0.,1.),(0.,0.0149999999999997),
 .UNSPECIFIED.);
#56511=B_SPLINE_SURFACE_WITH_KNOTS('',2,1,((#77630,#77631),(#77632,#77633),
(#77634,#77635)),.UNSPECIFIED.,.F.,.F.,.F.,(3,3),(2,2),(0.,1.),(0.,0.0149999999999997),
 .UNSPECIFIED.);
#56512=B_SPLINE_SURFACE_WITH_KNOTS('',2,1,((#77645,#77646),(#77647,#77648),
(#77649,#77650)),.UNSPECIFIED.,.F.,.F.,.F.,(3,3),(2,2),(0.,1.),(0.,0.0149999999999997),
 .UNSPECIFIED.);
#56513=B_SPLINE_SURFACE_WITH_KNOTS('',2,1,((#77660,#77661),(#77662,#77663),
(#77664,#77665)),.UNSPECIFIED.,.F.,.F.,.F.,(3,3),(2,2),(0.,1.),(0.,0.0149999999999997),
 .UNSPECIFIED.);
#56514=B_SPLINE_SURFACE_WITH_KNOTS('',2,1,((#77675,#77676),(#77677,#77678),
(#77679,#77680)),.UNSPECIFIED.,.F.,.F.,.F.,(3,3),(2,2),(0.,1.),(0.,0.0149999999999997),
 .UNSPECIFIED.);
#56515=B_SPLINE_SURFACE_WITH_KNOTS('',2,1,((#77691,#77692),(#77693,#77694),
(#77695,#77696)),.UNSPECIFIED.,.F.,.F.,.F.,(3,3),(2,2),(0.,1.),(0.,0.0149999999999997),
 .UNSPECIFIED.);
#56516=B_SPLINE_SURFACE_WITH_KNOTS('',2,1,((#77709,#77710),(#77711,#77712),
(#77713,#77714)),.UNSPECIFIED.,.F.,.F.,.F.,(3,3),(2,2),(0.,1.),(0.,0.0149999999999997),
 .UNSPECIFIED.);
#56517=B_SPLINE_SURFACE_WITH_KNOTS('',2,1,((#77724,#77725),(#77726,#77727),
(#77728,#77729)),.UNSPECIFIED.,.F.,.F.,.F.,(3,3),(2,2),(0.,1.),(0.,0.0149999999999997),
 .UNSPECIFIED.);
#56518=B_SPLINE_SURFACE_WITH_KNOTS('',2,1,((#77739,#77740),(#77741,#77742),
(#77743,#77744)),.UNSPECIFIED.,.F.,.F.,.F.,(3,3),(2,2),(0.,1.),(0.,0.0149999999999997),
 .UNSPECIFIED.);
#56519=B_SPLINE_SURFACE_WITH_KNOTS('',2,1,((#77754,#77755),(#77756,#77757),
(#77758,#77759)),.UNSPECIFIED.,.F.,.F.,.F.,(3,3),(2,2),(0.,1.),(0.,0.0149999999999997),
 .UNSPECIFIED.);
#56520=B_SPLINE_SURFACE_WITH_KNOTS('',2,1,((#77769,#77770),(#77771,#77772),
(#77773,#77774)),.UNSPECIFIED.,.F.,.F.,.F.,(3,3),(2,2),(0.,1.),(0.,0.0149999999999997),
 .UNSPECIFIED.);
#56521=B_SPLINE_SURFACE_WITH_KNOTS('',2,1,((#77784,#77785),(#77786,#77787),
(#77788,#77789)),.UNSPECIFIED.,.F.,.F.,.F.,(3,3),(2,2),(0.,1.),(0.,0.0149999999999997),
 .UNSPECIFIED.);
#56522=B_SPLINE_SURFACE_WITH_KNOTS('',2,1,((#77799,#77800),(#77801,#77802),
(#77803,#77804)),.UNSPECIFIED.,.F.,.F.,.F.,(3,3),(2,2),(0.,1.),(0.,0.0149999999999997),
 .UNSPECIFIED.);
#56523=B_SPLINE_SURFACE_WITH_KNOTS('',2,1,((#77811,#77812),(#77813,#77814),
(#77815,#77816)),.UNSPECIFIED.,.F.,.F.,.F.,(3,3),(2,2),(0.,1.),(0.,0.0149999999999997),
 .UNSPECIFIED.);
#56524=B_SPLINE_SURFACE_WITH_KNOTS('',2,1,((#77829,#77830),(#77831,#77832),
(#77833,#77834)),.UNSPECIFIED.,.F.,.F.,.F.,(3,3),(2,2),(0.,1.),(0.,0.0149999999999997),
 .UNSPECIFIED.);
#56525=B_SPLINE_SURFACE_WITH_KNOTS('',2,1,((#77844,#77845),(#77846,#77847),
(#77848,#77849)),.UNSPECIFIED.,.F.,.F.,.F.,(3,3),(2,2),(0.,1.),(0.,0.0149999999999997),
 .UNSPECIFIED.);
#56526=B_SPLINE_SURFACE_WITH_KNOTS('',2,1,((#77859,#77860),(#77861,#77862),
(#77863,#77864)),.UNSPECIFIED.,.F.,.F.,.F.,(3,3),(2,2),(0.,1.),(0.,0.0149999999999997),
 .UNSPECIFIED.);
#56527=B_SPLINE_SURFACE_WITH_KNOTS('',2,1,((#77874,#77875),(#77876,#77877),
(#77878,#77879)),.UNSPECIFIED.,.F.,.F.,.F.,(3,3),(2,2),(0.,1.),(0.,0.0149999999999997),
 .UNSPECIFIED.);
#56528=B_SPLINE_SURFACE_WITH_KNOTS('',2,1,((#77889,#77890),(#77891,#77892),
(#77893,#77894)),.UNSPECIFIED.,.F.,.F.,.F.,(3,3),(2,2),(0.,1.),(0.,0.0149999999999997),
 .UNSPECIFIED.);
#56529=B_SPLINE_SURFACE_WITH_KNOTS('',2,1,((#77904,#77905),(#77906,#77907),
(#77908,#77909)),.UNSPECIFIED.,.F.,.F.,.F.,(3,3),(2,2),(0.,1.),(0.,0.0149999999999997),
 .UNSPECIFIED.);
#56530=B_SPLINE_SURFACE_WITH_KNOTS('',2,1,((#77919,#77920),(#77921,#77922),
(#77923,#77924)),.UNSPECIFIED.,.F.,.F.,.F.,(3,3),(2,2),(0.,1.),(0.,0.0149999999999997),
 .UNSPECIFIED.);
#56531=B_SPLINE_SURFACE_WITH_KNOTS('',2,1,((#77934,#77935),(#77936,#77937),
(#77938,#77939)),.UNSPECIFIED.,.F.,.F.,.F.,(3,3),(2,2),(0.,1.),(0.,0.0149999999999997),
 .UNSPECIFIED.);
#56532=B_SPLINE_SURFACE_WITH_KNOTS('',2,1,((#77949,#77950),(#77951,#77952),
(#77953,#77954)),.UNSPECIFIED.,.F.,.F.,.F.,(3,3),(2,2),(0.,1.),(0.,0.0149999999999997),
 .UNSPECIFIED.);
#56533=B_SPLINE_SURFACE_WITH_KNOTS('',2,1,((#77964,#77965),(#77966,#77967),
(#77968,#77969)),.UNSPECIFIED.,.F.,.F.,.F.,(3,3),(2,2),(0.,1.),(0.,0.0149999999999997),
 .UNSPECIFIED.);
#56534=B_SPLINE_SURFACE_WITH_KNOTS('',2,1,((#77979,#77980),(#77981,#77982),
(#77983,#77984)),.UNSPECIFIED.,.F.,.F.,.F.,(3,3),(2,2),(0.,1.),(0.,0.0149999999999997),
 .UNSPECIFIED.);
#56535=B_SPLINE_SURFACE_WITH_KNOTS('',2,1,((#77992,#77993),(#77994,#77995),
(#77996,#77997)),.UNSPECIFIED.,.F.,.F.,.F.,(3,3),(2,2),(0.,1.),(0.,0.0149999999999997),
 .UNSPECIFIED.);
#56536=B_SPLINE_SURFACE_WITH_KNOTS('',2,1,((#78010,#78011),(#78012,#78013),
(#78014,#78015)),.UNSPECIFIED.,.F.,.F.,.F.,(3,3),(2,2),(0.,1.),(0.,0.0149999999999997),
 .UNSPECIFIED.);
#56537=B_SPLINE_SURFACE_WITH_KNOTS('',2,1,((#78025,#78026),(#78027,#78028),
(#78029,#78030)),.UNSPECIFIED.,.F.,.F.,.F.,(3,3),(2,2),(0.,1.),(0.,0.0149999999999997),
 .UNSPECIFIED.);
#56538=B_SPLINE_SURFACE_WITH_KNOTS('',2,1,((#78046,#78047),(#78048,#78049),
(#78050,#78051)),.UNSPECIFIED.,.F.,.F.,.F.,(3,3),(2,2),(0.,1.),(0.,0.0149999999999997),
 .UNSPECIFIED.);
#56539=B_SPLINE_SURFACE_WITH_KNOTS('',2,1,((#78061,#78062),(#78063,#78064),
(#78065,#78066)),.UNSPECIFIED.,.F.,.F.,.F.,(3,3),(2,2),(0.,1.),(0.,0.0149999999999997),
 .UNSPECIFIED.);
#56540=B_SPLINE_SURFACE_WITH_KNOTS('',2,1,((#78076,#78077),(#78078,#78079),
(#78080,#78081)),.UNSPECIFIED.,.F.,.F.,.F.,(3,3),(2,2),(0.,1.),(0.,0.0149999999999997),
 .UNSPECIFIED.);
#56541=B_SPLINE_SURFACE_WITH_KNOTS('',2,1,((#78114,#78115),(#78116,#78117),
(#78118,#78119)),.UNSPECIFIED.,.F.,.F.,.F.,(3,3),(2,2),(0.,1.),(0.,0.0149999999999997),
 .UNSPECIFIED.);
#56542=B_SPLINE_SURFACE_WITH_KNOTS('',2,1,((#78132,#78133),(#78134,#78135),
(#78136,#78137)),.UNSPECIFIED.,.F.,.F.,.F.,(3,3),(2,2),(0.,1.),(0.,0.0149999999999997),
 .UNSPECIFIED.);
#56543=B_SPLINE_SURFACE_WITH_KNOTS('',2,1,((#78147,#78148),(#78149,#78150),
(#78151,#78152)),.UNSPECIFIED.,.F.,.F.,.F.,(3,3),(2,2),(0.,1.),(0.,0.0149999999999997),
 .UNSPECIFIED.);
#56544=B_SPLINE_SURFACE_WITH_KNOTS('',2,1,((#78162,#78163),(#78164,#78165),
(#78166,#78167)),.UNSPECIFIED.,.F.,.F.,.F.,(3,3),(2,2),(0.,1.),(0.,0.0149999999999997),
 .UNSPECIFIED.);
#56545=B_SPLINE_SURFACE_WITH_KNOTS('',2,1,((#78177,#78178),(#78179,#78180),
(#78181,#78182)),.UNSPECIFIED.,.F.,.F.,.F.,(3,3),(2,2),(0.,1.),(0.,0.0149999999999997),
 .UNSPECIFIED.);
#56546=B_SPLINE_SURFACE_WITH_KNOTS('',2,1,((#78192,#78193),(#78194,#78195),
(#78196,#78197)),.UNSPECIFIED.,.F.,.F.,.F.,(3,3),(2,2),(0.,1.),(0.,0.0149999999999997),
 .UNSPECIFIED.);
#56547=B_SPLINE_SURFACE_WITH_KNOTS('',2,1,((#78207,#78208),(#78209,#78210),
(#78211,#78212)),.UNSPECIFIED.,.F.,.F.,.F.,(3,3),(2,2),(0.,1.),(0.,0.0149999999999997),
 .UNSPECIFIED.);
#56548=B_SPLINE_SURFACE_WITH_KNOTS('',2,1,((#78222,#78223),(#78224,#78225),
(#78226,#78227)),.UNSPECIFIED.,.F.,.F.,.F.,(3,3),(2,2),(0.,1.),(0.,0.0149999999999997),
 .UNSPECIFIED.);
#56549=B_SPLINE_SURFACE_WITH_KNOTS('',2,1,((#78234,#78235),(#78236,#78237),
(#78238,#78239)),.UNSPECIFIED.,.F.,.F.,.F.,(3,3),(2,2),(0.,1.),(0.,0.0149999999999997),
 .UNSPECIFIED.);
#56550=B_SPLINE_SURFACE_WITH_KNOTS('',2,1,((#78252,#78253),(#78254,#78255),
(#78256,#78257)),.UNSPECIFIED.,.F.,.F.,.F.,(3,3),(2,2),(0.,1.),(0.,0.0149999999999997),
 .UNSPECIFIED.);
#56551=B_SPLINE_SURFACE_WITH_KNOTS('',2,1,((#78267,#78268),(#78269,#78270),
(#78271,#78272)),.UNSPECIFIED.,.F.,.F.,.F.,(3,3),(2,2),(0.,1.),(0.,0.0149999999999997),
 .UNSPECIFIED.);
#56552=B_SPLINE_SURFACE_WITH_KNOTS('',2,1,((#78282,#78283),(#78284,#78285),
(#78286,#78287)),.UNSPECIFIED.,.F.,.F.,.F.,(3,3),(2,2),(0.,1.),(0.,0.0149999999999997),
 .UNSPECIFIED.);
#56553=B_SPLINE_SURFACE_WITH_KNOTS('',2,1,((#78297,#78298),(#78299,#78300),
(#78301,#78302)),.UNSPECIFIED.,.F.,.F.,.F.,(3,3),(2,2),(0.,1.),(0.,0.0149999999999997),
 .UNSPECIFIED.);
#56554=B_SPLINE_SURFACE_WITH_KNOTS('',2,1,((#78312,#78313),(#78314,#78315),
(#78316,#78317)),.UNSPECIFIED.,.F.,.F.,.F.,(3,3),(2,2),(0.,1.),(0.,0.0149999999999997),
 .UNSPECIFIED.);
#56555=B_SPLINE_SURFACE_WITH_KNOTS('',2,1,((#78327,#78328),(#78329,#78330),
(#78331,#78332)),.UNSPECIFIED.,.F.,.F.,.F.,(3,3),(2,2),(0.,1.),(0.,0.0149999999999997),
 .UNSPECIFIED.);
#56556=B_SPLINE_SURFACE_WITH_KNOTS('',2,1,((#78342,#78343),(#78344,#78345),
(#78346,#78347)),.UNSPECIFIED.,.F.,.F.,.F.,(3,3),(2,2),(0.,1.),(0.,0.0149999999999997),
 .UNSPECIFIED.);
#56557=B_SPLINE_SURFACE_WITH_KNOTS('',2,1,((#78357,#78358),(#78359,#78360),
(#78361,#78362)),.UNSPECIFIED.,.F.,.F.,.F.,(3,3),(2,2),(0.,1.),(0.,0.0149999999999997),
 .UNSPECIFIED.);
#56558=B_SPLINE_SURFACE_WITH_KNOTS('',2,1,((#78372,#78373),(#78374,#78375),
(#78376,#78377)),.UNSPECIFIED.,.F.,.F.,.F.,(3,3),(2,2),(0.,1.),(0.,0.0149999999999997),
 .UNSPECIFIED.);
#56559=B_SPLINE_SURFACE_WITH_KNOTS('',2,1,((#78387,#78388),(#78389,#78390),
(#78391,#78392)),.UNSPECIFIED.,.F.,.F.,.F.,(3,3),(2,2),(0.,1.),(0.,0.0149999999999997),
 .UNSPECIFIED.);
#56560=B_SPLINE_SURFACE_WITH_KNOTS('',2,1,((#78402,#78403),(#78404,#78405),
(#78406,#78407)),.UNSPECIFIED.,.F.,.F.,.F.,(3,3),(2,2),(0.,1.),(0.,0.0149999999999997),
 .UNSPECIFIED.);
#56561=B_SPLINE_SURFACE_WITH_KNOTS('',2,1,((#78415,#78416),(#78417,#78418),
(#78419,#78420)),.UNSPECIFIED.,.F.,.F.,.F.,(3,3),(2,2),(0.,1.),(0.,0.0149999999999997),
 .UNSPECIFIED.);
#56562=B_SPLINE_SURFACE_WITH_KNOTS('',2,1,((#78433,#78434),(#78435,#78436),
(#78437,#78438)),.UNSPECIFIED.,.F.,.F.,.F.,(3,3),(2,2),(0.,1.),(0.,0.0149999999999997),
 .UNSPECIFIED.);
#56563=B_SPLINE_SURFACE_WITH_KNOTS('',2,1,((#78448,#78449),(#78450,#78451),
(#78452,#78453)),.UNSPECIFIED.,.F.,.F.,.F.,(3,3),(2,2),(0.,1.),(0.,0.0149999999999997),
 .UNSPECIFIED.);
#56564=B_SPLINE_SURFACE_WITH_KNOTS('',2,1,((#78463,#78464),(#78465,#78466),
(#78467,#78468)),.UNSPECIFIED.,.F.,.F.,.F.,(3,3),(2,2),(0.,1.),(0.,0.0149999999999997),
 .UNSPECIFIED.);
#56565=B_SPLINE_SURFACE_WITH_KNOTS('',2,1,((#78478,#78479),(#78480,#78481),
(#78482,#78483)),.UNSPECIFIED.,.F.,.F.,.F.,(3,3),(2,2),(0.,1.),(0.,0.0149999999999997),
 .UNSPECIFIED.);
#56566=B_SPLINE_SURFACE_WITH_KNOTS('',2,1,((#78493,#78494),(#78495,#78496),
(#78497,#78498)),.UNSPECIFIED.,.F.,.F.,.F.,(3,3),(2,2),(0.,1.),(0.,0.0149999999999997),
 .UNSPECIFIED.);
#56567=B_SPLINE_SURFACE_WITH_KNOTS('',2,1,((#78508,#78509),(#78510,#78511),
(#78512,#78513)),.UNSPECIFIED.,.F.,.F.,.F.,(3,3),(2,2),(0.,1.),(0.,0.0149999999999997),
 .UNSPECIFIED.);
#56568=B_SPLINE_SURFACE_WITH_KNOTS('',2,1,((#78523,#78524),(#78525,#78526),
(#78527,#78528)),.UNSPECIFIED.,.F.,.F.,.F.,(3,3),(2,2),(0.,1.),(0.,0.0149999999999997),
 .UNSPECIFIED.);
#56569=B_SPLINE_SURFACE_WITH_KNOTS('',2,1,((#78538,#78539),(#78540,#78541),
(#78542,#78543)),.UNSPECIFIED.,.F.,.F.,.F.,(3,3),(2,2),(0.,1.),(0.,0.0149999999999997),
 .UNSPECIFIED.);
#56570=B_SPLINE_SURFACE_WITH_KNOTS('',2,1,((#78550,#78551),(#78552,#78553),
(#78554,#78555)),.UNSPECIFIED.,.F.,.F.,.F.,(3,3),(2,2),(0.,1.),(0.,0.0149999999999997),
 .UNSPECIFIED.);
#56571=B_SPLINE_SURFACE_WITH_KNOTS('',2,1,((#78568,#78569),(#78570,#78571),
(#78572,#78573)),.UNSPECIFIED.,.F.,.F.,.F.,(3,3),(2,2),(0.,1.),(0.,0.0149999999999997),
 .UNSPECIFIED.);
#56572=B_SPLINE_SURFACE_WITH_KNOTS('',2,1,((#78583,#78584),(#78585,#78586),
(#78587,#78588)),.UNSPECIFIED.,.F.,.F.,.F.,(3,3),(2,2),(0.,1.),(0.,0.0149999999999997),
 .UNSPECIFIED.);
#56573=B_SPLINE_SURFACE_WITH_KNOTS('',2,1,((#78598,#78599),(#78600,#78601),
(#78602,#78603)),.UNSPECIFIED.,.F.,.F.,.F.,(3,3),(2,2),(0.,1.),(0.,0.0149999999999997),
 .UNSPECIFIED.);
#56574=B_SPLINE_SURFACE_WITH_KNOTS('',2,1,((#78613,#78614),(#78615,#78616),
(#78617,#78618)),.UNSPECIFIED.,.F.,.F.,.F.,(3,3),(2,2),(0.,1.),(0.,0.0149999999999997),
 .UNSPECIFIED.);
#56575=B_SPLINE_SURFACE_WITH_KNOTS('',2,1,((#78628,#78629),(#78630,#78631),
(#78632,#78633)),.UNSPECIFIED.,.F.,.F.,.F.,(3,3),(2,2),(0.,1.),(0.,0.0149999999999997),
 .UNSPECIFIED.);
#56576=B_SPLINE_SURFACE_WITH_KNOTS('',2,1,((#78643,#78644),(#78645,#78646),
(#78647,#78648)),.UNSPECIFIED.,.F.,.F.,.F.,(3,3),(2,2),(0.,1.),(0.,0.0149999999999997),
 .UNSPECIFIED.);
#56577=B_SPLINE_SURFACE_WITH_KNOTS('',2,1,((#78658,#78659),(#78660,#78661),
(#78662,#78663)),.UNSPECIFIED.,.F.,.F.,.F.,(3,3),(2,2),(0.,1.),(0.,0.0149999999999997),
 .UNSPECIFIED.);
#56578=B_SPLINE_SURFACE_WITH_KNOTS('',2,1,((#78673,#78674),(#78675,#78676),
(#78677,#78678)),.UNSPECIFIED.,.F.,.F.,.F.,(3,3),(2,2),(0.,1.),(0.,0.0149999999999997),
 .UNSPECIFIED.);
#56579=B_SPLINE_SURFACE_WITH_KNOTS('',2,1,((#78688,#78689),(#78690,#78691),
(#78692,#78693)),.UNSPECIFIED.,.F.,.F.,.F.,(3,3),(2,2),(0.,1.),(0.,0.0149999999999997),
 .UNSPECIFIED.);
#56580=B_SPLINE_SURFACE_WITH_KNOTS('',2,1,((#78703,#78704),(#78705,#78706),
(#78707,#78708)),.UNSPECIFIED.,.F.,.F.,.F.,(3,3),(2,2),(0.,1.),(0.,0.0149999999999997),
 .UNSPECIFIED.);
#56581=B_SPLINE_SURFACE_WITH_KNOTS('',2,1,((#78718,#78719),(#78720,#78721),
(#78722,#78723)),.UNSPECIFIED.,.F.,.F.,.F.,(3,3),(2,2),(0.,1.),(0.,0.0149999999999997),
 .UNSPECIFIED.);
#56582=B_SPLINE_SURFACE_WITH_KNOTS('',2,1,((#78733,#78734),(#78735,#78736),
(#78737,#78738)),.UNSPECIFIED.,.F.,.F.,.F.,(3,3),(2,2),(0.,1.),(0.,0.0149999999999997),
 .UNSPECIFIED.);
#56583=B_SPLINE_SURFACE_WITH_KNOTS('',2,1,((#78748,#78749),(#78750,#78751),
(#78752,#78753)),.UNSPECIFIED.,.F.,.F.,.F.,(3,3),(2,2),(0.,1.),(0.,0.0149999999999997),
 .UNSPECIFIED.);
#56584=B_SPLINE_SURFACE_WITH_KNOTS('',2,1,((#78763,#78764),(#78765,#78766),
(#78767,#78768)),.UNSPECIFIED.,.F.,.F.,.F.,(3,3),(2,2),(0.,1.),(0.,0.0149999999999997),
 .UNSPECIFIED.);
#56585=B_SPLINE_SURFACE_WITH_KNOTS('',2,1,((#78778,#78779),(#78780,#78781),
(#78782,#78783)),.UNSPECIFIED.,.F.,.F.,.F.,(3,3),(2,2),(0.,1.),(0.,0.0149999999999997),
 .UNSPECIFIED.);
#56586=B_SPLINE_SURFACE_WITH_KNOTS('',2,1,((#78793,#78794),(#78795,#78796),
(#78797,#78798)),.UNSPECIFIED.,.F.,.F.,.F.,(3,3),(2,2),(0.,1.),(0.,0.0149999999999997),
 .UNSPECIFIED.);
#56587=B_SPLINE_SURFACE_WITH_KNOTS('',2,1,((#78814,#78815),(#78816,#78817),
(#78818,#78819)),.UNSPECIFIED.,.F.,.F.,.F.,(3,3),(2,2),(0.,1.),(0.,0.0149999999999997),
 .UNSPECIFIED.);
#56588=B_SPLINE_SURFACE_WITH_KNOTS('',2,1,((#78829,#78830),(#78831,#78832),
(#78833,#78834)),.UNSPECIFIED.,.F.,.F.,.F.,(3,3),(2,2),(0.,1.),(0.,0.0149999999999997),
 .UNSPECIFIED.);
#56589=B_SPLINE_SURFACE_WITH_KNOTS('',2,1,((#78847,#78848),(#78849,#78850),
(#78851,#78852)),.UNSPECIFIED.,.F.,.F.,.F.,(3,3),(2,2),(0.,1.),(0.,0.0149999999999997),
 .UNSPECIFIED.);
#56590=B_SPLINE_SURFACE_WITH_KNOTS('',2,1,((#78862,#78863),(#78864,#78865),
(#78866,#78867)),.UNSPECIFIED.,.F.,.F.,.F.,(3,3),(2,2),(0.,1.),(0.,0.0149999999999997),
 .UNSPECIFIED.);
#56591=B_SPLINE_SURFACE_WITH_KNOTS('',2,1,((#78877,#78878),(#78879,#78880),
(#78881,#78882)),.UNSPECIFIED.,.F.,.F.,.F.,(3,3),(2,2),(0.,1.),(0.,0.0149999999999997),
 .UNSPECIFIED.);
#56592=B_SPLINE_SURFACE_WITH_KNOTS('',2,1,((#78892,#78893),(#78894,#78895),
(#78896,#78897)),.UNSPECIFIED.,.F.,.F.,.F.,(3,3),(2,2),(0.,1.),(0.,0.0149999999999997),
 .UNSPECIFIED.);
#56593=B_SPLINE_SURFACE_WITH_KNOTS('',2,1,((#78907,#78908),(#78909,#78910),
(#78911,#78912)),.UNSPECIFIED.,.F.,.F.,.F.,(3,3),(2,2),(0.,1.),(0.,0.0149999999999997),
 .UNSPECIFIED.);
#56594=B_SPLINE_SURFACE_WITH_KNOTS('',2,1,((#78922,#78923),(#78924,#78925),
(#78926,#78927)),.UNSPECIFIED.,.F.,.F.,.F.,(3,3),(2,2),(0.,1.),(0.,0.0149999999999997),
 .UNSPECIFIED.);
#56595=B_SPLINE_SURFACE_WITH_KNOTS('',2,1,((#78937,#78938),(#78939,#78940),
(#78941,#78942)),.UNSPECIFIED.,.F.,.F.,.F.,(3,3),(2,2),(0.,1.),(0.,0.0149999999999997),
 .UNSPECIFIED.);
#56596=B_SPLINE_SURFACE_WITH_KNOTS('',2,1,((#78949,#78950),(#78951,#78952),
(#78953,#78954)),.UNSPECIFIED.,.F.,.F.,.F.,(3,3),(2,2),(0.,1.),(0.,0.0149999999999997),
 .UNSPECIFIED.);
#56597=B_SPLINE_SURFACE_WITH_KNOTS('',2,1,((#78967,#78968),(#78969,#78970),
(#78971,#78972)),.UNSPECIFIED.,.F.,.F.,.F.,(3,3),(2,2),(0.,1.),(0.,0.0149999999999997),
 .UNSPECIFIED.);
#56598=B_SPLINE_SURFACE_WITH_KNOTS('',2,1,((#78982,#78983),(#78984,#78985),
(#78986,#78987)),.UNSPECIFIED.,.F.,.F.,.F.,(3,3),(2,2),(0.,1.),(0.,0.0149999999999997),
 .UNSPECIFIED.);
#56599=B_SPLINE_SURFACE_WITH_KNOTS('',2,1,((#78997,#78998),(#78999,#79000),
(#79001,#79002)),.UNSPECIFIED.,.F.,.F.,.F.,(3,3),(2,2),(0.,1.),(0.,0.0149999999999997),
 .UNSPECIFIED.);
#56600=B_SPLINE_SURFACE_WITH_KNOTS('',2,1,((#79012,#79013),(#79014,#79015),
(#79016,#79017)),.UNSPECIFIED.,.F.,.F.,.F.,(3,3),(2,2),(0.,1.),(0.,0.0149999999999997),
 .UNSPECIFIED.);
#56601=B_SPLINE_SURFACE_WITH_KNOTS('',2,1,((#79027,#79028),(#79029,#79030),
(#79031,#79032)),.UNSPECIFIED.,.F.,.F.,.F.,(3,3),(2,2),(0.,1.),(0.,0.0149999999999997),
 .UNSPECIFIED.);
#56602=B_SPLINE_SURFACE_WITH_KNOTS('',2,1,((#79042,#79043),(#79044,#79045),
(#79046,#79047)),.UNSPECIFIED.,.F.,.F.,.F.,(3,3),(2,2),(0.,1.),(0.,0.0149999999999997),
 .UNSPECIFIED.);
#56603=B_SPLINE_SURFACE_WITH_KNOTS('',2,1,((#79057,#79058),(#79059,#79060),
(#79061,#79062)),.UNSPECIFIED.,.F.,.F.,.F.,(3,3),(2,2),(0.,1.),(0.,0.0149999999999997),
 .UNSPECIFIED.);
#56604=B_SPLINE_SURFACE_WITH_KNOTS('',2,1,((#79072,#79073),(#79074,#79075),
(#79076,#79077)),.UNSPECIFIED.,.F.,.F.,.F.,(3,3),(2,2),(0.,1.),(0.,0.0149999999999997),
 .UNSPECIFIED.);
#56605=B_SPLINE_SURFACE_WITH_KNOTS('',2,1,((#79087,#79088),(#79089,#79090),
(#79091,#79092)),.UNSPECIFIED.,.F.,.F.,.F.,(3,3),(2,2),(0.,1.),(0.,0.0149999999999997),
 .UNSPECIFIED.);
#56606=B_SPLINE_SURFACE_WITH_KNOTS('',2,1,((#79102,#79103),(#79104,#79105),
(#79106,#79107)),.UNSPECIFIED.,.F.,.F.,.F.,(3,3),(2,2),(0.,1.),(0.,0.0149999999999997),
 .UNSPECIFIED.);
#56607=B_SPLINE_SURFACE_WITH_KNOTS('',2,1,((#79117,#79118),(#79119,#79120),
(#79121,#79122)),.UNSPECIFIED.,.F.,.F.,.F.,(3,3),(2,2),(0.,1.),(0.,0.0149999999999997),
 .UNSPECIFIED.);
#56608=B_SPLINE_SURFACE_WITH_KNOTS('',2,1,((#79130,#79131),(#79132,#79133),
(#79134,#79135)),.UNSPECIFIED.,.F.,.F.,.F.,(3,3),(2,2),(0.,1.),(0.,0.0149999999999997),
 .UNSPECIFIED.);
#56609=B_SPLINE_SURFACE_WITH_KNOTS('',2,1,((#79148,#79149),(#79150,#79151),
(#79152,#79153)),.UNSPECIFIED.,.F.,.F.,.F.,(3,3),(2,2),(0.,1.),(0.,0.0149999999999997),
 .UNSPECIFIED.);
#56610=B_SPLINE_SURFACE_WITH_KNOTS('',2,1,((#79163,#79164),(#79165,#79166),
(#79167,#79168)),.UNSPECIFIED.,.F.,.F.,.F.,(3,3),(2,2),(0.,1.),(0.,0.0149999999999997),
 .UNSPECIFIED.);
#56611=B_SPLINE_SURFACE_WITH_KNOTS('',2,1,((#79178,#79179),(#79180,#79181),
(#79182,#79183)),.UNSPECIFIED.,.F.,.F.,.F.,(3,3),(2,2),(0.,1.),(0.,0.0149999999999997),
 .UNSPECIFIED.);
#56612=B_SPLINE_SURFACE_WITH_KNOTS('',2,1,((#79193,#79194),(#79195,#79196),
(#79197,#79198)),.UNSPECIFIED.,.F.,.F.,.F.,(3,3),(2,2),(0.,1.),(0.,0.0149999999999997),
 .UNSPECIFIED.);
#56613=B_SPLINE_SURFACE_WITH_KNOTS('',2,1,((#79208,#79209),(#79210,#79211),
(#79212,#79213)),.UNSPECIFIED.,.F.,.F.,.F.,(3,3),(2,2),(0.,1.),(0.,0.0149999999999997),
 .UNSPECIFIED.);
#56614=B_SPLINE_SURFACE_WITH_KNOTS('',2,1,((#79259,#79260),(#79261,#79262),
(#79263,#79264)),.UNSPECIFIED.,.F.,.F.,.F.,(3,3),(2,2),(0.,1.),(0.,0.0149999999999997),
 .UNSPECIFIED.);
#56615=B_SPLINE_SURFACE_WITH_KNOTS('',2,1,((#79274,#79275),(#79276,#79277),
(#79278,#79279)),.UNSPECIFIED.,.F.,.F.,.F.,(3,3),(2,2),(0.,1.),(0.,0.0149999999999997),
 .UNSPECIFIED.);
#56616=B_SPLINE_SURFACE_WITH_KNOTS('',2,1,((#79289,#79290),(#79291,#79292),
(#79293,#79294)),.UNSPECIFIED.,.F.,.F.,.F.,(3,3),(2,2),(0.,1.),(0.,0.0149999999999997),
 .UNSPECIFIED.);
#56617=B_SPLINE_SURFACE_WITH_KNOTS('',2,1,((#79304,#79305),(#79306,#79307),
(#79308,#79309)),.UNSPECIFIED.,.F.,.F.,.F.,(3,3),(2,2),(0.,1.),(0.,0.0149999999999997),
 .UNSPECIFIED.);
#56618=B_SPLINE_SURFACE_WITH_KNOTS('',2,1,((#79319,#79320),(#79321,#79322),
(#79323,#79324)),.UNSPECIFIED.,.F.,.F.,.F.,(3,3),(2,2),(0.,1.),(0.,0.0149999999999997),
 .UNSPECIFIED.);
#56619=B_SPLINE_SURFACE_WITH_KNOTS('',2,1,((#79334,#79335),(#79336,#79337),
(#79338,#79339)),.UNSPECIFIED.,.F.,.F.,.F.,(3,3),(2,2),(0.,1.),(0.,0.0149999999999997),
 .UNSPECIFIED.);
#56620=B_SPLINE_SURFACE_WITH_KNOTS('',2,1,((#79349,#79350),(#79351,#79352),
(#79353,#79354)),.UNSPECIFIED.,.F.,.F.,.F.,(3,3),(2,2),(0.,1.),(0.,0.0149999999999997),
 .UNSPECIFIED.);
#56621=B_SPLINE_SURFACE_WITH_KNOTS('',2,1,((#79364,#79365),(#79366,#79367),
(#79368,#79369)),.UNSPECIFIED.,.F.,.F.,.F.,(3,3),(2,2),(0.,1.),(0.,0.0149999999999997),
 .UNSPECIFIED.);
#56622=B_SPLINE_SURFACE_WITH_KNOTS('',2,1,((#79385,#79386),(#79387,#79388),
(#79389,#79390)),.UNSPECIFIED.,.F.,.F.,.F.,(3,3),(2,2),(0.,1.),(0.,0.0149999999999997),
 .UNSPECIFIED.);
#56623=B_SPLINE_SURFACE_WITH_KNOTS('',2,1,((#79399,#79400),(#79401,#79402),
(#79403,#79404)),.UNSPECIFIED.,.F.,.F.,.F.,(3,3),(2,2),(0.,1.),(0.,0.0149999999999997),
 .UNSPECIFIED.);
#56624=B_SPLINE_SURFACE_WITH_KNOTS('',2,1,((#79417,#79418),(#79419,#79420),
(#79421,#79422)),.UNSPECIFIED.,.F.,.F.,.F.,(3,3),(2,2),(0.,1.),(0.,0.0149999999999997),
 .UNSPECIFIED.);
#56625=B_SPLINE_SURFACE_WITH_KNOTS('',2,1,((#79432,#79433),(#79434,#79435),
(#79436,#79437)),.UNSPECIFIED.,.F.,.F.,.F.,(3,3),(2,2),(0.,1.),(0.,0.0149999999999997),
 .UNSPECIFIED.);
#56626=B_SPLINE_SURFACE_WITH_KNOTS('',2,1,((#79447,#79448),(#79449,#79450),
(#79451,#79452)),.UNSPECIFIED.,.F.,.F.,.F.,(3,3),(2,2),(0.,1.),(0.,0.0149999999999997),
 .UNSPECIFIED.);
#56627=B_SPLINE_SURFACE_WITH_KNOTS('',2,1,((#79462,#79463),(#79464,#79465),
(#79466,#79467)),.UNSPECIFIED.,.F.,.F.,.F.,(3,3),(2,2),(0.,1.),(0.,0.0149999999999997),
 .UNSPECIFIED.);
#56628=B_SPLINE_SURFACE_WITH_KNOTS('',2,1,((#79477,#79478),(#79479,#79480),
(#79481,#79482)),.UNSPECIFIED.,.F.,.F.,.F.,(3,3),(2,2),(0.,1.),(0.,0.0149999999999997),
 .UNSPECIFIED.);
#56629=B_SPLINE_SURFACE_WITH_KNOTS('',2,1,((#79492,#79493),(#79494,#79495),
(#79496,#79497)),.UNSPECIFIED.,.F.,.F.,.F.,(3,3),(2,2),(0.,1.),(0.,0.0149999999999997),
 .UNSPECIFIED.);
#56630=B_SPLINE_SURFACE_WITH_KNOTS('',2,1,((#79507,#79508),(#79509,#79510),
(#79511,#79512)),.UNSPECIFIED.,.F.,.F.,.F.,(3,3),(2,2),(0.,1.),(0.,0.0149999999999997),
 .UNSPECIFIED.);
#56631=B_SPLINE_SURFACE_WITH_KNOTS('',2,1,((#79519,#79520),(#79521,#79522),
(#79523,#79524)),.UNSPECIFIED.,.F.,.F.,.F.,(3,3),(2,2),(0.,1.),(0.,0.0149999999999997),
 .UNSPECIFIED.);
#56632=B_SPLINE_SURFACE_WITH_KNOTS('',2,1,((#79537,#79538),(#79539,#79540),
(#79541,#79542)),.UNSPECIFIED.,.F.,.F.,.F.,(3,3),(2,2),(0.,1.),(0.,0.0149999999999997),
 .UNSPECIFIED.);
#56633=B_SPLINE_SURFACE_WITH_KNOTS('',2,1,((#79552,#79553),(#79554,#79555),
(#79556,#79557)),.UNSPECIFIED.,.F.,.F.,.F.,(3,3),(2,2),(0.,1.),(0.,0.0149999999999997),
 .UNSPECIFIED.);
#56634=B_SPLINE_SURFACE_WITH_KNOTS('',2,1,((#79567,#79568),(#79569,#79570),
(#79571,#79572)),.UNSPECIFIED.,.F.,.F.,.F.,(3,3),(2,2),(0.,1.),(0.,0.0149999999999997),
 .UNSPECIFIED.);
#56635=B_SPLINE_SURFACE_WITH_KNOTS('',2,1,((#79582,#79583),(#79584,#79585),
(#79586,#79587)),.UNSPECIFIED.,.F.,.F.,.F.,(3,3),(2,2),(0.,1.),(0.,0.0149999999999997),
 .UNSPECIFIED.);
#56636=B_SPLINE_SURFACE_WITH_KNOTS('',2,1,((#79597,#79598),(#79599,#79600),
(#79601,#79602)),.UNSPECIFIED.,.F.,.F.,.F.,(3,3),(2,2),(0.,1.),(0.,0.0149999999999997),
 .UNSPECIFIED.);
#56637=B_SPLINE_SURFACE_WITH_KNOTS('',2,1,((#79612,#79613),(#79614,#79615),
(#79616,#79617)),.UNSPECIFIED.,.F.,.F.,.F.,(3,3),(2,2),(0.,1.),(0.,0.0149999999999997),
 .UNSPECIFIED.);
#56638=B_SPLINE_SURFACE_WITH_KNOTS('',2,1,((#79627,#79628),(#79629,#79630),
(#79631,#79632)),.UNSPECIFIED.,.F.,.F.,.F.,(3,3),(2,2),(0.,1.),(0.,0.0149999999999997),
 .UNSPECIFIED.);
#56639=B_SPLINE_SURFACE_WITH_KNOTS('',2,1,((#79642,#79643),(#79644,#79645),
(#79646,#79647)),.UNSPECIFIED.,.F.,.F.,.F.,(3,3),(2,2),(0.,1.),(0.,0.0149999999999997),
 .UNSPECIFIED.);
#56640=B_SPLINE_SURFACE_WITH_KNOTS('',2,1,((#79657,#79658),(#79659,#79660),
(#79661,#79662)),.UNSPECIFIED.,.F.,.F.,.F.,(3,3),(2,2),(0.,1.),(0.,0.0149999999999997),
 .UNSPECIFIED.);
#56641=B_SPLINE_SURFACE_WITH_KNOTS('',2,1,((#79672,#79673),(#79674,#79675),
(#79676,#79677)),.UNSPECIFIED.,.F.,.F.,.F.,(3,3),(2,2),(0.,1.),(0.,0.0149999999999997),
 .UNSPECIFIED.);
#56642=B_SPLINE_SURFACE_WITH_KNOTS('',2,1,((#79687,#79688),(#79689,#79690),
(#79691,#79692)),.UNSPECIFIED.,.F.,.F.,.F.,(3,3),(2,2),(0.,1.),(0.,0.0149999999999997),
 .UNSPECIFIED.);
#56643=B_SPLINE_SURFACE_WITH_KNOTS('',2,1,((#79787,#79788),(#79789,#79790),
(#79791,#79792)),.UNSPECIFIED.,.F.,.F.,.F.,(3,3),(2,2),(0.,1.),(0.,0.0149999999999997),
 .UNSPECIFIED.);
#56644=B_SPLINE_SURFACE_WITH_KNOTS('',2,1,((#79805,#79806),(#79807,#79808),
(#79809,#79810)),.UNSPECIFIED.,.F.,.F.,.F.,(3,3),(2,2),(0.,1.),(0.,0.0149999999999997),
 .UNSPECIFIED.);
#56645=B_SPLINE_SURFACE_WITH_KNOTS('',2,1,((#79820,#79821),(#79822,#79823),
(#79824,#79825)),.UNSPECIFIED.,.F.,.F.,.F.,(3,3),(2,2),(0.,1.),(0.,0.0149999999999997),
 .UNSPECIFIED.);
#56646=B_SPLINE_SURFACE_WITH_KNOTS('',2,1,((#79835,#79836),(#79837,#79838),
(#79839,#79840)),.UNSPECIFIED.,.F.,.F.,.F.,(3,3),(2,2),(0.,1.),(0.,0.0149999999999997),
 .UNSPECIFIED.);
#56647=B_SPLINE_SURFACE_WITH_KNOTS('',2,1,((#79850,#79851),(#79852,#79853),
(#79854,#79855)),.UNSPECIFIED.,.F.,.F.,.F.,(3,3),(2,2),(0.,1.),(0.,0.0149999999999997),
 .UNSPECIFIED.);
#56648=B_SPLINE_SURFACE_WITH_KNOTS('',2,1,((#79865,#79866),(#79867,#79868),
(#79869,#79870)),.UNSPECIFIED.,.F.,.F.,.F.,(3,3),(2,2),(0.,1.),(0.,0.0149999999999997),
 .UNSPECIFIED.);
#56649=B_SPLINE_SURFACE_WITH_KNOTS('',2,1,((#79880,#79881),(#79882,#79883),
(#79884,#79885)),.UNSPECIFIED.,.F.,.F.,.F.,(3,3),(2,2),(0.,1.),(0.,0.0149999999999997),
 .UNSPECIFIED.);
#56650=B_SPLINE_SURFACE_WITH_KNOTS('',2,1,((#79895,#79896),(#79897,#79898),
(#79899,#79900)),.UNSPECIFIED.,.F.,.F.,.F.,(3,3),(2,2),(0.,1.),(0.,0.0149999999999997),
 .UNSPECIFIED.);
#56651=B_SPLINE_SURFACE_WITH_KNOTS('',2,1,((#79907,#79908),(#79909,#79910),
(#79911,#79912)),.UNSPECIFIED.,.F.,.F.,.F.,(3,3),(2,2),(0.,1.),(0.,0.0149999999999997),
 .UNSPECIFIED.);
#56652=B_SPLINE_SURFACE_WITH_KNOTS('',2,1,((#79925,#79926),(#79927,#79928),
(#79929,#79930)),.UNSPECIFIED.,.F.,.F.,.F.,(3,3),(2,2),(0.,1.),(0.,0.0149999999999997),
 .UNSPECIFIED.);
#56653=B_SPLINE_SURFACE_WITH_KNOTS('',2,1,((#79940,#79941),(#79942,#79943),
(#79944,#79945)),.UNSPECIFIED.,.F.,.F.,.F.,(3,3),(2,2),(0.,1.),(0.,0.0149999999999997),
 .UNSPECIFIED.);
#56654=B_SPLINE_SURFACE_WITH_KNOTS('',2,1,((#79955,#79956),(#79957,#79958),
(#79959,#79960)),.UNSPECIFIED.,.F.,.F.,.F.,(3,3),(2,2),(0.,1.),(0.,0.0149999999999997),
 .UNSPECIFIED.);
#56655=B_SPLINE_SURFACE_WITH_KNOTS('',2,1,((#79970,#79971),(#79972,#79973),
(#79974,#79975)),.UNSPECIFIED.,.F.,.F.,.F.,(3,3),(2,2),(0.,1.),(0.,0.0149999999999997),
 .UNSPECIFIED.);
#56656=B_SPLINE_SURFACE_WITH_KNOTS('',2,1,((#79985,#79986),(#79987,#79988),
(#79989,#79990)),.UNSPECIFIED.,.F.,.F.,.F.,(3,3),(2,2),(0.,1.),(0.,0.0149999999999997),
 .UNSPECIFIED.);
#56657=B_SPLINE_SURFACE_WITH_KNOTS('',2,1,((#80000,#80001),(#80002,#80003),
(#80004,#80005)),.UNSPECIFIED.,.F.,.F.,.F.,(3,3),(2,2),(0.,1.),(0.,0.0149999999999997),
 .UNSPECIFIED.);
#56658=B_SPLINE_SURFACE_WITH_KNOTS('',2,1,((#80015,#80016),(#80017,#80018),
(#80019,#80020)),.UNSPECIFIED.,.F.,.F.,.F.,(3,3),(2,2),(0.,1.),(0.,0.0149999999999997),
 .UNSPECIFIED.);
#56659=B_SPLINE_SURFACE_WITH_KNOTS('',2,1,((#80030,#80031),(#80032,#80033),
(#80034,#80035)),.UNSPECIFIED.,.F.,.F.,.F.,(3,3),(2,2),(0.,1.),(0.,0.0149999999999997),
 .UNSPECIFIED.);
#56660=B_SPLINE_SURFACE_WITH_KNOTS('',2,1,((#80045,#80046),(#80047,#80048),
(#80049,#80050)),.UNSPECIFIED.,.F.,.F.,.F.,(3,3),(2,2),(0.,1.),(0.,0.0149999999999997),
 .UNSPECIFIED.);
#56661=B_SPLINE_SURFACE_WITH_KNOTS('',2,1,((#80060,#80061),(#80062,#80063),
(#80064,#80065)),.UNSPECIFIED.,.F.,.F.,.F.,(3,3),(2,2),(0.,1.),(0.,0.0149999999999997),
 .UNSPECIFIED.);
#56662=B_SPLINE_SURFACE_WITH_KNOTS('',2,1,((#80075,#80076),(#80077,#80078),
(#80079,#80080)),.UNSPECIFIED.,.F.,.F.,.F.,(3,3),(2,2),(0.,1.),(0.,0.0149999999999997),
 .UNSPECIFIED.);
#56663=B_SPLINE_SURFACE_WITH_KNOTS('',2,1,((#80088,#80089),(#80090,#80091),
(#80092,#80093)),.UNSPECIFIED.,.F.,.F.,.F.,(3,3),(2,2),(0.,1.),(0.,0.0149999999999997),
 .UNSPECIFIED.);
#56664=B_SPLINE_SURFACE_WITH_KNOTS('',2,1,((#80106,#80107),(#80108,#80109),
(#80110,#80111)),.UNSPECIFIED.,.F.,.F.,.F.,(3,3),(2,2),(0.,1.),(0.,0.0149999999999997),
 .UNSPECIFIED.);
#56665=B_SPLINE_SURFACE_WITH_KNOTS('',2,1,((#80121,#80122),(#80123,#80124),
(#80125,#80126)),.UNSPECIFIED.,.F.,.F.,.F.,(3,3),(2,2),(0.,1.),(0.,0.0149999999999997),
 .UNSPECIFIED.);
#56666=B_SPLINE_SURFACE_WITH_KNOTS('',2,1,((#80136,#80137),(#80138,#80139),
(#80140,#80141)),.UNSPECIFIED.,.F.,.F.,.F.,(3,3),(2,2),(0.,1.),(0.,0.0149999999999997),
 .UNSPECIFIED.);
#56667=B_SPLINE_SURFACE_WITH_KNOTS('',2,1,((#80151,#80152),(#80153,#80154),
(#80155,#80156)),.UNSPECIFIED.,.F.,.F.,.F.,(3,3),(2,2),(0.,1.),(0.,0.0149999999999997),
 .UNSPECIFIED.);
#56668=B_SPLINE_SURFACE_WITH_KNOTS('',2,1,((#80166,#80167),(#80168,#80169),
(#80170,#80171)),.UNSPECIFIED.,.F.,.F.,.F.,(3,3),(2,2),(0.,1.),(0.,0.0149999999999997),
 .UNSPECIFIED.);
#56669=B_SPLINE_SURFACE_WITH_KNOTS('',2,1,((#80181,#80182),(#80183,#80184),
(#80185,#80186)),.UNSPECIFIED.,.F.,.F.,.F.,(3,3),(2,2),(0.,1.),(0.,0.0149999999999997),
 .UNSPECIFIED.);
#56670=B_SPLINE_SURFACE_WITH_KNOTS('',2,1,((#80196,#80197),(#80198,#80199),
(#80200,#80201)),.UNSPECIFIED.,.F.,.F.,.F.,(3,3),(2,2),(0.,1.),(0.,0.0149999999999997),
 .UNSPECIFIED.);
#56671=B_SPLINE_SURFACE_WITH_KNOTS('',2,1,((#80211,#80212),(#80213,#80214),
(#80215,#80216)),.UNSPECIFIED.,.F.,.F.,.F.,(3,3),(2,2),(0.,1.),(0.,0.0149999999999997),
 .UNSPECIFIED.);
#56672=B_SPLINE_SURFACE_WITH_KNOTS('',2,1,((#80226,#80227),(#80228,#80229),
(#80230,#80231)),.UNSPECIFIED.,.F.,.F.,.F.,(3,3),(2,2),(0.,1.),(0.,0.0149999999999997),
 .UNSPECIFIED.);
#56673=B_SPLINE_SURFACE_WITH_KNOTS('',2,1,((#80241,#80242),(#80243,#80244),
(#80245,#80246)),.UNSPECIFIED.,.F.,.F.,.F.,(3,3),(2,2),(0.,1.),(0.,0.0149999999999997),
 .UNSPECIFIED.);
#56674=B_SPLINE_SURFACE_WITH_KNOTS('',2,1,((#80256,#80257),(#80258,#80259),
(#80260,#80261)),.UNSPECIFIED.,.F.,.F.,.F.,(3,3),(2,2),(0.,1.),(0.,0.0149999999999997),
 .UNSPECIFIED.);
#56675=B_SPLINE_SURFACE_WITH_KNOTS('',2,1,((#80277,#80278),(#80279,#80280),
(#80281,#80282)),.UNSPECIFIED.,.F.,.F.,.F.,(3,3),(2,2),(0.,1.),(0.,0.0149999999999997),
 .UNSPECIFIED.);
#56676=B_SPLINE_SURFACE_WITH_KNOTS('',2,1,((#80292,#80293),(#80294,#80295),
(#80296,#80297)),.UNSPECIFIED.,.F.,.F.,.F.,(3,3),(2,2),(0.,1.),(0.,0.0149999999999997),
 .UNSPECIFIED.);
#56677=B_SPLINE_SURFACE_WITH_KNOTS('',2,1,((#80307,#80308),(#80309,#80310),
(#80311,#80312)),.UNSPECIFIED.,.F.,.F.,.F.,(3,3),(2,2),(0.,1.),(0.,0.0149999999999997),
 .UNSPECIFIED.);
#56678=B_SPLINE_SURFACE_WITH_KNOTS('',2,1,((#80322,#80323),(#80324,#80325),
(#80326,#80327)),.UNSPECIFIED.,.F.,.F.,.F.,(3,3),(2,2),(0.,1.),(0.,0.0149999999999997),
 .UNSPECIFIED.);
#56679=B_SPLINE_SURFACE_WITH_KNOTS('',2,1,((#80337,#80338),(#80339,#80340),
(#80341,#80342)),.UNSPECIFIED.,.F.,.F.,.F.,(3,3),(2,2),(0.,1.),(0.,0.0149999999999997),
 .UNSPECIFIED.);
#56680=B_SPLINE_SURFACE_WITH_KNOTS('',2,1,((#80352,#80353),(#80354,#80355),
(#80356,#80357)),.UNSPECIFIED.,.F.,.F.,.F.,(3,3),(2,2),(0.,1.),(0.,0.0149999999999997),
 .UNSPECIFIED.);
#56681=B_SPLINE_SURFACE_WITH_KNOTS('',2,1,((#80367,#80368),(#80369,#80370),
(#80371,#80372)),.UNSPECIFIED.,.F.,.F.,.F.,(3,3),(2,2),(0.,1.),(0.,0.0149999999999997),
 .UNSPECIFIED.);
#56682=B_SPLINE_SURFACE_WITH_KNOTS('',2,1,((#80388,#80389),(#80390,#80391),
(#80392,#80393)),.UNSPECIFIED.,.F.,.F.,.F.,(3,3),(2,2),(0.,1.),(0.,0.0149999999999997),
 .UNSPECIFIED.);
#56683=B_SPLINE_SURFACE_WITH_KNOTS('',2,1,((#80403,#80404),(#80405,#80406),
(#80407,#80408)),.UNSPECIFIED.,.F.,.F.,.F.,(3,3),(2,2),(0.,1.),(0.,0.0149999999999997),
 .UNSPECIFIED.);
#56684=B_SPLINE_SURFACE_WITH_KNOTS('',2,1,((#80418,#80419),(#80420,#80421),
(#80422,#80423)),.UNSPECIFIED.,.F.,.F.,.F.,(3,3),(2,2),(0.,1.),(0.,0.0149999999999997),
 .UNSPECIFIED.);
#56685=B_SPLINE_SURFACE_WITH_KNOTS('',2,1,((#80433,#80434),(#80435,#80436),
(#80437,#80438)),.UNSPECIFIED.,.F.,.F.,.F.,(3,3),(2,2),(0.,1.),(0.,0.0149999999999997),
 .UNSPECIFIED.);
#56686=B_SPLINE_SURFACE_WITH_KNOTS('',2,1,((#80448,#80449),(#80450,#80451),
(#80452,#80453)),.UNSPECIFIED.,.F.,.F.,.F.,(3,3),(2,2),(0.,1.),(0.,0.0149999999999997),
 .UNSPECIFIED.);
#56687=B_SPLINE_SURFACE_WITH_KNOTS('',2,1,((#80463,#80464),(#80465,#80466),
(#80467,#80468)),.UNSPECIFIED.,.F.,.F.,.F.,(3,3),(2,2),(0.,1.),(0.,0.0149999999999997),
 .UNSPECIFIED.);
#56688=B_SPLINE_SURFACE_WITH_KNOTS('',2,1,((#80478,#80479),(#80480,#80481),
(#80482,#80483)),.UNSPECIFIED.,.F.,.F.,.F.,(3,3),(2,2),(0.,1.),(0.,0.0149999999999997),
 .UNSPECIFIED.);
#56689=B_SPLINE_SURFACE_WITH_KNOTS('',2,1,((#80499,#80500),(#80501,#80502),
(#80503,#80504)),.UNSPECIFIED.,.F.,.F.,.F.,(3,3),(2,2),(0.,1.),(0.,0.0149999999999997),
 .UNSPECIFIED.);
#56690=B_SPLINE_SURFACE_WITH_KNOTS('',2,1,((#80513,#80514),(#80515,#80516),
(#80517,#80518)),.UNSPECIFIED.,.F.,.F.,.F.,(3,3),(2,2),(0.,1.),(0.,0.0149999999999997),
 .UNSPECIFIED.);
#56691=B_SPLINE_SURFACE_WITH_KNOTS('',2,1,((#80531,#80532),(#80533,#80534),
(#80535,#80536)),.UNSPECIFIED.,.F.,.F.,.F.,(3,3),(2,2),(0.,1.),(0.,0.0149999999999997),
 .UNSPECIFIED.);
#56692=B_SPLINE_SURFACE_WITH_KNOTS('',2,1,((#80546,#80547),(#80548,#80549),
(#80550,#80551)),.UNSPECIFIED.,.F.,.F.,.F.,(3,3),(2,2),(0.,1.),(0.,0.0149999999999997),
 .UNSPECIFIED.);
#56693=B_SPLINE_SURFACE_WITH_KNOTS('',2,1,((#80561,#80562),(#80563,#80564),
(#80565,#80566)),.UNSPECIFIED.,.F.,.F.,.F.,(3,3),(2,2),(0.,1.),(0.,0.0149999999999997),
 .UNSPECIFIED.);
#56694=B_SPLINE_SURFACE_WITH_KNOTS('',2,1,((#80576,#80577),(#80578,#80579),
(#80580,#80581)),.UNSPECIFIED.,.F.,.F.,.F.,(3,3),(2,2),(0.,1.),(0.,0.0149999999999997),
 .UNSPECIFIED.);
#56695=B_SPLINE_SURFACE_WITH_KNOTS('',2,1,((#80591,#80592),(#80593,#80594),
(#80595,#80596)),.UNSPECIFIED.,.F.,.F.,.F.,(3,3),(2,2),(0.,1.),(0.,0.0149999999999997),
 .UNSPECIFIED.);
#56696=B_SPLINE_SURFACE_WITH_KNOTS('',2,1,((#80606,#80607),(#80608,#80609),
(#80610,#80611)),.UNSPECIFIED.,.F.,.F.,.F.,(3,3),(2,2),(0.,1.),(0.,0.0149999999999997),
 .UNSPECIFIED.);
#56697=B_SPLINE_SURFACE_WITH_KNOTS('',2,1,((#80621,#80622),(#80623,#80624),
(#80625,#80626)),.UNSPECIFIED.,.F.,.F.,.F.,(3,3),(2,2),(0.,1.),(0.,0.0149999999999997),
 .UNSPECIFIED.);
#56698=B_SPLINE_SURFACE_WITH_KNOTS('',2,1,((#80633,#80634),(#80635,#80636),
(#80637,#80638)),.UNSPECIFIED.,.F.,.F.,.F.,(3,3),(2,2),(0.,1.),(0.,0.0149999999999997),
 .UNSPECIFIED.);
#56699=B_SPLINE_SURFACE_WITH_KNOTS('',2,1,((#80651,#80652),(#80653,#80654),
(#80655,#80656)),.UNSPECIFIED.,.F.,.F.,.F.,(3,3),(2,2),(0.,1.),(0.,0.0149999999999997),
 .UNSPECIFIED.);
#56700=B_SPLINE_SURFACE_WITH_KNOTS('',2,1,((#80666,#80667),(#80668,#80669),
(#80670,#80671)),.UNSPECIFIED.,.F.,.F.,.F.,(3,3),(2,2),(0.,1.),(0.,0.0149999999999997),
 .UNSPECIFIED.);
#56701=B_SPLINE_SURFACE_WITH_KNOTS('',2,1,((#80681,#80682),(#80683,#80684),
(#80685,#80686)),.UNSPECIFIED.,.F.,.F.,.F.,(3,3),(2,2),(0.,1.),(0.,0.0149999999999997),
 .UNSPECIFIED.);
#56702=B_SPLINE_SURFACE_WITH_KNOTS('',2,1,((#80696,#80697),(#80698,#80699),
(#80700,#80701)),.UNSPECIFIED.,.F.,.F.,.F.,(3,3),(2,2),(0.,1.),(0.,0.0149999999999997),
 .UNSPECIFIED.);
#56703=B_SPLINE_SURFACE_WITH_KNOTS('',2,1,((#80711,#80712),(#80713,#80714),
(#80715,#80716)),.UNSPECIFIED.,.F.,.F.,.F.,(3,3),(2,2),(0.,1.),(0.,0.0149999999999997),
 .UNSPECIFIED.);
#56704=B_SPLINE_SURFACE_WITH_KNOTS('',2,1,((#80726,#80727),(#80728,#80729),
(#80730,#80731)),.UNSPECIFIED.,.F.,.F.,.F.,(3,3),(2,2),(0.,1.),(0.,0.0149999999999997),
 .UNSPECIFIED.);
#56705=B_SPLINE_SURFACE_WITH_KNOTS('',2,1,((#80741,#80742),(#80743,#80744),
(#80745,#80746)),.UNSPECIFIED.,.F.,.F.,.F.,(3,3),(2,2),(0.,1.),(0.,0.0149999999999997),
 .UNSPECIFIED.);
#56706=B_SPLINE_SURFACE_WITH_KNOTS('',2,1,((#80756,#80757),(#80758,#80759),
(#80760,#80761)),.UNSPECIFIED.,.F.,.F.,.F.,(3,3),(2,2),(0.,1.),(0.,0.0149999999999997),
 .UNSPECIFIED.);
#56707=B_SPLINE_SURFACE_WITH_KNOTS('',2,1,((#80771,#80772),(#80773,#80774),
(#80775,#80776)),.UNSPECIFIED.,.F.,.F.,.F.,(3,3),(2,2),(0.,1.),(0.,0.0149999999999997),
 .UNSPECIFIED.);
#56708=B_SPLINE_SURFACE_WITH_KNOTS('',2,1,((#80786,#80787),(#80788,#80789),
(#80790,#80791)),.UNSPECIFIED.,.F.,.F.,.F.,(3,3),(2,2),(0.,1.),(0.,0.0149999999999997),
 .UNSPECIFIED.);
#56709=B_SPLINE_SURFACE_WITH_KNOTS('',2,1,((#80801,#80802),(#80803,#80804),
(#80805,#80806)),.UNSPECIFIED.,.F.,.F.,.F.,(3,3),(2,2),(0.,1.),(0.,0.0149999999999997),
 .UNSPECIFIED.);
#56710=B_SPLINE_SURFACE_WITH_KNOTS('',2,1,((#80814,#80815),(#80816,#80817),
(#80818,#80819)),.UNSPECIFIED.,.F.,.F.,.F.,(3,3),(2,2),(0.,1.),(0.,0.0149999999999997),
 .UNSPECIFIED.);
#56711=B_SPLINE_SURFACE_WITH_KNOTS('',2,1,((#80832,#80833),(#80834,#80835),
(#80836,#80837)),.UNSPECIFIED.,.F.,.F.,.F.,(3,3),(2,2),(0.,1.),(0.,0.0149999999999997),
 .UNSPECIFIED.);
#56712=B_SPLINE_SURFACE_WITH_KNOTS('',2,1,((#80847,#80848),(#80849,#80850),
(#80851,#80852)),.UNSPECIFIED.,.F.,.F.,.F.,(3,3),(2,2),(0.,1.),(0.,0.0149999999999997),
 .UNSPECIFIED.);
#56713=B_SPLINE_SURFACE_WITH_KNOTS('',2,1,((#80862,#80863),(#80864,#80865),
(#80866,#80867)),.UNSPECIFIED.,.F.,.F.,.F.,(3,3),(2,2),(0.,1.),(0.,0.0149999999999997),
 .UNSPECIFIED.);
#56714=B_SPLINE_SURFACE_WITH_KNOTS('',2,1,((#80877,#80878),(#80879,#80880),
(#80881,#80882)),.UNSPECIFIED.,.F.,.F.,.F.,(3,3),(2,2),(0.,1.),(0.,0.0149999999999997),
 .UNSPECIFIED.);
#56715=B_SPLINE_SURFACE_WITH_KNOTS('',2,1,((#80892,#80893),(#80894,#80895),
(#80896,#80897)),.UNSPECIFIED.,.F.,.F.,.F.,(3,3),(2,2),(0.,1.),(0.,0.0149999999999997),
 .UNSPECIFIED.);
#56716=B_SPLINE_SURFACE_WITH_KNOTS('',2,1,((#80907,#80908),(#80909,#80910),
(#80911,#80912)),.UNSPECIFIED.,.F.,.F.,.F.,(3,3),(2,2),(0.,1.),(0.,0.0149999999999997),
 .UNSPECIFIED.);
#56717=B_SPLINE_SURFACE_WITH_KNOTS('',2,1,((#80922,#80923),(#80924,#80925),
(#80926,#80927)),.UNSPECIFIED.,.F.,.F.,.F.,(3,3),(2,2),(0.,1.),(0.,0.0149999999999997),
 .UNSPECIFIED.);
#56718=B_SPLINE_SURFACE_WITH_KNOTS('',2,1,((#80937,#80938),(#80939,#80940),
(#80941,#80942)),.UNSPECIFIED.,.F.,.F.,.F.,(3,3),(2,2),(0.,1.),(0.,0.0149999999999997),
 .UNSPECIFIED.);
#56719=B_SPLINE_SURFACE_WITH_KNOTS('',2,1,((#80958,#80959),(#80960,#80961),
(#80962,#80963)),.UNSPECIFIED.,.F.,.F.,.F.,(3,3),(2,2),(0.,1.),(0.,0.0149999999999997),
 .UNSPECIFIED.);
#56720=B_SPLINE_SURFACE_WITH_KNOTS('',2,1,((#80973,#80974),(#80975,#80976),
(#80977,#80978)),.UNSPECIFIED.,.F.,.F.,.F.,(3,3),(2,2),(0.,1.),(0.,0.0149999999999997),
 .UNSPECIFIED.);
#56721=B_SPLINE_SURFACE_WITH_KNOTS('',2,1,((#80988,#80989),(#80990,#80991),
(#80992,#80993)),.UNSPECIFIED.,.F.,.F.,.F.,(3,3),(2,2),(0.,1.),(0.,0.0149999999999997),
 .UNSPECIFIED.);
#56722=B_SPLINE_SURFACE_WITH_KNOTS('',2,1,((#81003,#81004),(#81005,#81006),
(#81007,#81008)),.UNSPECIFIED.,.F.,.F.,.F.,(3,3),(2,2),(0.,1.),(0.,0.0149999999999997),
 .UNSPECIFIED.);
#56723=B_SPLINE_SURFACE_WITH_KNOTS('',2,1,((#81018,#81019),(#81020,#81021),
(#81022,#81023)),.UNSPECIFIED.,.F.,.F.,.F.,(3,3),(2,2),(0.,1.),(0.,0.0149999999999997),
 .UNSPECIFIED.);
#56724=B_SPLINE_SURFACE_WITH_KNOTS('',2,1,((#81033,#81034),(#81035,#81036),
(#81037,#81038)),.UNSPECIFIED.,.F.,.F.,.F.,(3,3),(2,2),(0.,1.),(0.,0.0149999999999997),
 .UNSPECIFIED.);
#56725=B_SPLINE_SURFACE_WITH_KNOTS('',2,1,((#81048,#81049),(#81050,#81051),
(#81052,#81053)),.UNSPECIFIED.,.F.,.F.,.F.,(3,3),(2,2),(0.,1.),(0.,0.0149999999999997),
 .UNSPECIFIED.);
#56726=B_SPLINE_SURFACE_WITH_KNOTS('',2,1,((#81063,#81064),(#81065,#81066),
(#81067,#81068)),.UNSPECIFIED.,.F.,.F.,.F.,(3,3),(2,2),(0.,1.),(0.,0.0149999999999997),
 .UNSPECIFIED.);
#56727=B_SPLINE_SURFACE_WITH_KNOTS('',2,1,((#81078,#81079),(#81080,#81081),
(#81082,#81083)),.UNSPECIFIED.,.F.,.F.,.F.,(3,3),(2,2),(0.,1.),(0.,0.0149999999999997),
 .UNSPECIFIED.);
#56728=B_SPLINE_SURFACE_WITH_KNOTS('',2,1,((#81110,#81111),(#81112,#81113),
(#81114,#81115)),.UNSPECIFIED.,.F.,.F.,.F.,(3,3),(2,2),(0.,1.),(0.,0.0149999999999997),
 .UNSPECIFIED.);
#56729=B_SPLINE_SURFACE_WITH_KNOTS('',2,1,((#81128,#81129),(#81130,#81131),
(#81132,#81133)),.UNSPECIFIED.,.F.,.F.,.F.,(3,3),(2,2),(0.,1.),(0.,0.0149999999999997),
 .UNSPECIFIED.);
#56730=B_SPLINE_SURFACE_WITH_KNOTS('',2,1,((#81143,#81144),(#81145,#81146),
(#81147,#81148)),.UNSPECIFIED.,.F.,.F.,.F.,(3,3),(2,2),(0.,1.),(0.,0.0149999999999997),
 .UNSPECIFIED.);
#56731=B_SPLINE_SURFACE_WITH_KNOTS('',2,1,((#81158,#81159),(#81160,#81161),
(#81162,#81163)),.UNSPECIFIED.,.F.,.F.,.F.,(3,3),(2,2),(0.,1.),(0.,0.0149999999999997),
 .UNSPECIFIED.);
#56732=B_SPLINE_SURFACE_WITH_KNOTS('',2,1,((#81173,#81174),(#81175,#81176),
(#81177,#81178)),.UNSPECIFIED.,.F.,.F.,.F.,(3,3),(2,2),(0.,1.),(0.,0.0149999999999997),
 .UNSPECIFIED.);
#56733=B_SPLINE_SURFACE_WITH_KNOTS('',2,1,((#81188,#81189),(#81190,#81191),
(#81192,#81193)),.UNSPECIFIED.,.F.,.F.,.F.,(3,3),(2,2),(0.,1.),(0.,0.0149999999999997),
 .UNSPECIFIED.);
#56734=B_SPLINE_SURFACE_WITH_KNOTS('',2,1,((#81203,#81204),(#81205,#81206),
(#81207,#81208)),.UNSPECIFIED.,.F.,.F.,.F.,(3,3),(2,2),(0.,1.),(0.,0.0149999999999997),
 .UNSPECIFIED.);
#56735=B_SPLINE_SURFACE_WITH_KNOTS('',2,1,((#81218,#81219),(#81220,#81221),
(#81222,#81223)),.UNSPECIFIED.,.F.,.F.,.F.,(3,3),(2,2),(0.,1.),(0.,0.0149999999999997),
 .UNSPECIFIED.);
#56736=B_SPLINE_SURFACE_WITH_KNOTS('',2,1,((#81230,#81231),(#81232,#81233),
(#81234,#81235)),.UNSPECIFIED.,.F.,.F.,.F.,(3,3),(2,2),(0.,1.),(0.,0.0149999999999997),
 .UNSPECIFIED.);
#56737=B_SPLINE_SURFACE_WITH_KNOTS('',2,1,((#81248,#81249),(#81250,#81251),
(#81252,#81253)),.UNSPECIFIED.,.F.,.F.,.F.,(3,3),(2,2),(0.,1.),(0.,0.0149999999999997),
 .UNSPECIFIED.);
#56738=B_SPLINE_SURFACE_WITH_KNOTS('',2,1,((#81263,#81264),(#81265,#81266),
(#81267,#81268)),.UNSPECIFIED.,.F.,.F.,.F.,(3,3),(2,2),(0.,1.),(0.,0.0149999999999997),
 .UNSPECIFIED.);
#56739=B_SPLINE_SURFACE_WITH_KNOTS('',2,1,((#81278,#81279),(#81280,#81281),
(#81282,#81283)),.UNSPECIFIED.,.F.,.F.,.F.,(3,3),(2,2),(0.,1.),(0.,0.0149999999999997),
 .UNSPECIFIED.);
#56740=B_SPLINE_SURFACE_WITH_KNOTS('',2,1,((#81293,#81294),(#81295,#81296),
(#81297,#81298)),.UNSPECIFIED.,.F.,.F.,.F.,(3,3),(2,2),(0.,1.),(0.,0.0149999999999997),
 .UNSPECIFIED.);
#56741=B_SPLINE_SURFACE_WITH_KNOTS('',2,1,((#81308,#81309),(#81310,#81311),
(#81312,#81313)),.UNSPECIFIED.,.F.,.F.,.F.,(3,3),(2,2),(0.,1.),(0.,0.0149999999999997),
 .UNSPECIFIED.);
#56742=B_SPLINE_SURFACE_WITH_KNOTS('',2,1,((#81323,#81324),(#81325,#81326),
(#81327,#81328)),.UNSPECIFIED.,.F.,.F.,.F.,(3,3),(2,2),(0.,1.),(0.,0.0149999999999997),
 .UNSPECIFIED.);
#56743=B_SPLINE_SURFACE_WITH_KNOTS('',2,1,((#81338,#81339),(#81340,#81341),
(#81342,#81343)),.UNSPECIFIED.,.F.,.F.,.F.,(3,3),(2,2),(0.,1.),(0.,0.0149999999999997),
 .UNSPECIFIED.);
#56744=B_SPLINE_SURFACE_WITH_KNOTS('',2,1,((#81353,#81354),(#81355,#81356),
(#81357,#81358)),.UNSPECIFIED.,.F.,.F.,.F.,(3,3),(2,2),(0.,1.),(0.,0.0149999999999997),
 .UNSPECIFIED.);
#56745=B_SPLINE_SURFACE_WITH_KNOTS('',2,1,((#81368,#81369),(#81370,#81371),
(#81372,#81373)),.UNSPECIFIED.,.F.,.F.,.F.,(3,3),(2,2),(0.,1.),(0.,0.0149999999999997),
 .UNSPECIFIED.);
#56746=B_SPLINE_SURFACE_WITH_KNOTS('',2,1,((#81383,#81384),(#81385,#81386),
(#81387,#81388)),.UNSPECIFIED.,.F.,.F.,.F.,(3,3),(2,2),(0.,1.),(0.,0.0149999999999997),
 .UNSPECIFIED.);
#56747=B_SPLINE_SURFACE_WITH_KNOTS('',2,1,((#81398,#81399),(#81400,#81401),
(#81402,#81403)),.UNSPECIFIED.,.F.,.F.,.F.,(3,3),(2,2),(0.,1.),(0.,0.0149999999999997),
 .UNSPECIFIED.);
#56748=B_SPLINE_SURFACE_WITH_KNOTS('',2,1,((#81420,#81421),(#81422,#81423),
(#81424,#81425)),.UNSPECIFIED.,.F.,.F.,.F.,(3,3),(2,2),(0.,1.),(0.,0.0149999999999997),
 .UNSPECIFIED.);
#56749=B_SPLINE_SURFACE_WITH_KNOTS('',2,1,((#81435,#81436),(#81437,#81438),
(#81439,#81440)),.UNSPECIFIED.,.F.,.F.,.F.,(3,3),(2,2),(0.,1.),(0.,0.0149999999999997),
 .UNSPECIFIED.);
#56750=B_SPLINE_SURFACE_WITH_KNOTS('',2,1,((#81456,#81457),(#81458,#81459),
(#81460,#81461)),.UNSPECIFIED.,.F.,.F.,.F.,(3,3),(2,2),(0.,1.),(0.,0.0149999999999997),
 .UNSPECIFIED.);
#56751=B_SPLINE_SURFACE_WITH_KNOTS('',2,1,((#81471,#81472),(#81473,#81474),
(#81475,#81476)),.UNSPECIFIED.,.F.,.F.,.F.,(3,3),(2,2),(0.,1.),(0.,0.0149999999999997),
 .UNSPECIFIED.);
#56752=B_SPLINE_SURFACE_WITH_KNOTS('',2,1,((#81503,#81504),(#81505,#81506),
(#81507,#81508)),.UNSPECIFIED.,.F.,.F.,.F.,(3,3),(2,2),(0.,1.),(0.,0.0149999999999997),
 .UNSPECIFIED.);
#56753=B_SPLINE_SURFACE_WITH_KNOTS('',2,1,((#81521,#81522),(#81523,#81524),
(#81525,#81526)),.UNSPECIFIED.,.F.,.F.,.F.,(3,3),(2,2),(0.,1.),(0.,0.0149999999999997),
 .UNSPECIFIED.);
#56754=B_SPLINE_SURFACE_WITH_KNOTS('',2,1,((#81536,#81537),(#81538,#81539),
(#81540,#81541)),.UNSPECIFIED.,.F.,.F.,.F.,(3,3),(2,2),(0.,1.),(0.,0.0149999999999997),
 .UNSPECIFIED.);
#56755=B_SPLINE_SURFACE_WITH_KNOTS('',2,1,((#81551,#81552),(#81553,#81554),
(#81555,#81556)),.UNSPECIFIED.,.F.,.F.,.F.,(3,3),(2,2),(0.,1.),(0.,0.0149999999999997),
 .UNSPECIFIED.);
#56756=B_SPLINE_SURFACE_WITH_KNOTS('',2,1,((#81566,#81567),(#81568,#81569),
(#81570,#81571)),.UNSPECIFIED.,.F.,.F.,.F.,(3,3),(2,2),(0.,1.),(0.,0.0149999999999997),
 .UNSPECIFIED.);
#56757=B_SPLINE_SURFACE_WITH_KNOTS('',2,1,((#81581,#81582),(#81583,#81584),
(#81585,#81586)),.UNSPECIFIED.,.F.,.F.,.F.,(3,3),(2,2),(0.,1.),(0.,0.0149999999999997),
 .UNSPECIFIED.);
#56758=B_SPLINE_SURFACE_WITH_KNOTS('',2,1,((#81596,#81597),(#81598,#81599),
(#81600,#81601)),.UNSPECIFIED.,.F.,.F.,.F.,(3,3),(2,2),(0.,1.),(0.,0.0149999999999997),
 .UNSPECIFIED.);
#56759=B_SPLINE_SURFACE_WITH_KNOTS('',2,1,((#81611,#81612),(#81613,#81614),
(#81615,#81616)),.UNSPECIFIED.,.F.,.F.,.F.,(3,3),(2,2),(0.,1.),(0.,0.0149999999999997),
 .UNSPECIFIED.);
#56760=B_SPLINE_SURFACE_WITH_KNOTS('',2,1,((#81623,#81624),(#81625,#81626),
(#81627,#81628)),.UNSPECIFIED.,.F.,.F.,.F.,(3,3),(2,2),(0.,1.),(0.,0.0149999999999997),
 .UNSPECIFIED.);
#56761=B_SPLINE_SURFACE_WITH_KNOTS('',2,1,((#81641,#81642),(#81643,#81644),
(#81645,#81646)),.UNSPECIFIED.,.F.,.F.,.F.,(3,3),(2,2),(0.,1.),(0.,0.0149999999999997),
 .UNSPECIFIED.);
#56762=B_SPLINE_SURFACE_WITH_KNOTS('',2,1,((#81656,#81657),(#81658,#81659),
(#81660,#81661)),.UNSPECIFIED.,.F.,.F.,.F.,(3,3),(2,2),(0.,1.),(0.,0.0149999999999997),
 .UNSPECIFIED.);
#56763=B_SPLINE_SURFACE_WITH_KNOTS('',2,1,((#81671,#81672),(#81673,#81674),
(#81675,#81676)),.UNSPECIFIED.,.F.,.F.,.F.,(3,3),(2,2),(0.,1.),(0.,0.0149999999999997),
 .UNSPECIFIED.);
#56764=B_SPLINE_SURFACE_WITH_KNOTS('',2,1,((#81686,#81687),(#81688,#81689),
(#81690,#81691)),.UNSPECIFIED.,.F.,.F.,.F.,(3,3),(2,2),(0.,1.),(0.,0.0149999999999997),
 .UNSPECIFIED.);
#56765=B_SPLINE_SURFACE_WITH_KNOTS('',2,1,((#81701,#81702),(#81703,#81704),
(#81705,#81706)),.UNSPECIFIED.,.F.,.F.,.F.,(3,3),(2,2),(0.,1.),(0.,0.0149999999999997),
 .UNSPECIFIED.);
#56766=B_SPLINE_SURFACE_WITH_KNOTS('',2,1,((#81716,#81717),(#81718,#81719),
(#81720,#81721)),.UNSPECIFIED.,.F.,.F.,.F.,(3,3),(2,2),(0.,1.),(0.,0.0149999999999997),
 .UNSPECIFIED.);
#56767=B_SPLINE_SURFACE_WITH_KNOTS('',2,1,((#81731,#81732),(#81733,#81734),
(#81735,#81736)),.UNSPECIFIED.,.F.,.F.,.F.,(3,3),(2,2),(0.,1.),(0.,0.0149999999999997),
 .UNSPECIFIED.);
#56768=B_SPLINE_SURFACE_WITH_KNOTS('',2,1,((#81746,#81747),(#81748,#81749),
(#81750,#81751)),.UNSPECIFIED.,.F.,.F.,.F.,(3,3),(2,2),(0.,1.),(0.,0.0149999999999997),
 .UNSPECIFIED.);
#56769=B_SPLINE_SURFACE_WITH_KNOTS('',2,1,((#81761,#81762),(#81763,#81764),
(#81765,#81766)),.UNSPECIFIED.,.F.,.F.,.F.,(3,3),(2,2),(0.,1.),(0.,0.0149999999999997),
 .UNSPECIFIED.);
#56770=B_SPLINE_SURFACE_WITH_KNOTS('',2,1,((#81776,#81777),(#81778,#81779),
(#81780,#81781)),.UNSPECIFIED.,.F.,.F.,.F.,(3,3),(2,2),(0.,1.),(0.,0.0149999999999997),
 .UNSPECIFIED.);
#56771=B_SPLINE_SURFACE_WITH_KNOTS('',2,1,((#81791,#81792),(#81793,#81794),
(#81795,#81796)),.UNSPECIFIED.,.F.,.F.,.F.,(3,3),(2,2),(0.,1.),(0.,0.0149999999999997),
 .UNSPECIFIED.);
#56772=B_SPLINE_SURFACE_WITH_KNOTS('',2,1,((#81805,#81806),(#81807,#81808),
(#81809,#81810)),.UNSPECIFIED.,.F.,.F.,.F.,(3,3),(2,2),(0.,1.),(0.,0.0149999999999997),
 .UNSPECIFIED.);
#56773=B_SPLINE_SURFACE_WITH_KNOTS('',2,1,((#81823,#81824),(#81825,#81826),
(#81827,#81828)),.UNSPECIFIED.,.F.,.F.,.F.,(3,3),(2,2),(0.,1.),(0.,0.0149999999999997),
 .UNSPECIFIED.);
#56774=B_SPLINE_SURFACE_WITH_KNOTS('',2,1,((#81838,#81839),(#81840,#81841),
(#81842,#81843)),.UNSPECIFIED.,.F.,.F.,.F.,(3,3),(2,2),(0.,1.),(0.,0.0149999999999997),
 .UNSPECIFIED.);
#56775=B_SPLINE_SURFACE_WITH_KNOTS('',2,1,((#81853,#81854),(#81855,#81856),
(#81857,#81858)),.UNSPECIFIED.,.F.,.F.,.F.,(3,3),(2,2),(0.,1.),(0.,0.0149999999999997),
 .UNSPECIFIED.);
#56776=B_SPLINE_SURFACE_WITH_KNOTS('',2,1,((#81868,#81869),(#81870,#81871),
(#81872,#81873)),.UNSPECIFIED.,.F.,.F.,.F.,(3,3),(2,2),(0.,1.),(0.,0.0149999999999997),
 .UNSPECIFIED.);
#56777=B_SPLINE_SURFACE_WITH_KNOTS('',2,1,((#81883,#81884),(#81885,#81886),
(#81887,#81888)),.UNSPECIFIED.,.F.,.F.,.F.,(3,3),(2,2),(0.,1.),(0.,0.0149999999999997),
 .UNSPECIFIED.);
#56778=B_SPLINE_SURFACE_WITH_KNOTS('',2,1,((#81898,#81899),(#81900,#81901),
(#81902,#81903)),.UNSPECIFIED.,.F.,.F.,.F.,(3,3),(2,2),(0.,1.),(0.,0.0149999999999997),
 .UNSPECIFIED.);
#56779=B_SPLINE_SURFACE_WITH_KNOTS('',2,1,((#81913,#81914),(#81915,#81916),
(#81917,#81918)),.UNSPECIFIED.,.F.,.F.,.F.,(3,3),(2,2),(0.,1.),(0.,0.0149999999999997),
 .UNSPECIFIED.);
#56780=B_SPLINE_SURFACE_WITH_KNOTS('',2,1,((#81925,#81926),(#81927,#81928),
(#81929,#81930)),.UNSPECIFIED.,.F.,.F.,.F.,(3,3),(2,2),(0.,1.),(0.,0.0149999999999997),
 .UNSPECIFIED.);
#56781=B_SPLINE_SURFACE_WITH_KNOTS('',2,1,((#81943,#81944),(#81945,#81946),
(#81947,#81948)),.UNSPECIFIED.,.F.,.F.,.F.,(3,3),(2,2),(0.,1.),(0.,0.0149999999999997),
 .UNSPECIFIED.);
#56782=B_SPLINE_SURFACE_WITH_KNOTS('',2,1,((#81958,#81959),(#81960,#81961),
(#81962,#81963)),.UNSPECIFIED.,.F.,.F.,.F.,(3,3),(2,2),(0.,1.),(0.,0.0149999999999997),
 .UNSPECIFIED.);
#56783=B_SPLINE_SURFACE_WITH_KNOTS('',2,1,((#81973,#81974),(#81975,#81976),
(#81977,#81978)),.UNSPECIFIED.,.F.,.F.,.F.,(3,3),(2,2),(0.,1.),(0.,0.0149999999999997),
 .UNSPECIFIED.);
#56784=B_SPLINE_SURFACE_WITH_KNOTS('',2,1,((#81988,#81989),(#81990,#81991),
(#81992,#81993)),.UNSPECIFIED.,.F.,.F.,.F.,(3,3),(2,2),(0.,1.),(0.,0.0149999999999997),
 .UNSPECIFIED.);
#56785=B_SPLINE_SURFACE_WITH_KNOTS('',2,1,((#82003,#82004),(#82005,#82006),
(#82007,#82008)),.UNSPECIFIED.,.F.,.F.,.F.,(3,3),(2,2),(0.,1.),(0.,0.0149999999999997),
 .UNSPECIFIED.);
#56786=B_SPLINE_SURFACE_WITH_KNOTS('',2,1,((#82018,#82019),(#82020,#82021),
(#82022,#82023)),.UNSPECIFIED.,.F.,.F.,.F.,(3,3),(2,2),(0.,1.),(0.,0.0149999999999997),
 .UNSPECIFIED.);
#56787=B_SPLINE_SURFACE_WITH_KNOTS('',2,1,((#82033,#82034),(#82035,#82036),
(#82037,#82038)),.UNSPECIFIED.,.F.,.F.,.F.,(3,3),(2,2),(0.,1.),(0.,0.0149999999999997),
 .UNSPECIFIED.);
#56788=B_SPLINE_SURFACE_WITH_KNOTS('',2,1,((#82048,#82049),(#82050,#82051),
(#82052,#82053)),.UNSPECIFIED.,.F.,.F.,.F.,(3,3),(2,2),(0.,1.),(0.,0.0149999999999997),
 .UNSPECIFIED.);
#56789=B_SPLINE_SURFACE_WITH_KNOTS('',2,1,((#82063,#82064),(#82065,#82066),
(#82067,#82068)),.UNSPECIFIED.,.F.,.F.,.F.,(3,3),(2,2),(0.,1.),(0.,0.0149999999999997),
 .UNSPECIFIED.);
#56790=B_SPLINE_SURFACE_WITH_KNOTS('',2,1,((#82078,#82079),(#82080,#82081),
(#82082,#82083)),.UNSPECIFIED.,.F.,.F.,.F.,(3,3),(2,2),(0.,1.),(0.,0.0149999999999997),
 .UNSPECIFIED.);
#56791=B_SPLINE_SURFACE_WITH_KNOTS('',2,1,((#82093,#82094),(#82095,#82096),
(#82097,#82098)),.UNSPECIFIED.,.F.,.F.,.F.,(3,3),(2,2),(0.,1.),(0.,0.0149999999999997),
 .UNSPECIFIED.);
#56792=B_SPLINE_SURFACE_WITH_KNOTS('',2,1,((#82115,#82116),(#82117,#82118),
(#82119,#82120)),.UNSPECIFIED.,.F.,.F.,.F.,(3,3),(2,2),(0.,1.),(0.,0.0149999999999997),
 .UNSPECIFIED.);
#56793=B_SPLINE_SURFACE_WITH_KNOTS('',2,1,((#82130,#82131),(#82132,#82133),
(#82134,#82135)),.UNSPECIFIED.,.F.,.F.,.F.,(3,3),(2,2),(0.,1.),(0.,0.0149999999999997),
 .UNSPECIFIED.);
#56794=B_SPLINE_SURFACE_WITH_KNOTS('',2,1,((#82151,#82152),(#82153,#82154),
(#82155,#82156)),.UNSPECIFIED.,.F.,.F.,.F.,(3,3),(2,2),(0.,1.),(0.,0.0149999999999997),
 .UNSPECIFIED.);
#56795=B_SPLINE_SURFACE_WITH_KNOTS('',2,1,((#82166,#82167),(#82168,#82169),
(#82170,#82171)),.UNSPECIFIED.,.F.,.F.,.F.,(3,3),(2,2),(0.,1.),(0.,0.0149999999999997),
 .UNSPECIFIED.);
#56796=B_SPLINE_SURFACE_WITH_KNOTS('',2,1,((#82198,#82199),(#82200,#82201),
(#82202,#82203)),.UNSPECIFIED.,.F.,.F.,.F.,(3,3),(2,2),(0.,1.),(0.,0.0149999999999997),
 .UNSPECIFIED.);
#56797=B_SPLINE_SURFACE_WITH_KNOTS('',2,1,((#82216,#82217),(#82218,#82219),
(#82220,#82221)),.UNSPECIFIED.,.F.,.F.,.F.,(3,3),(2,2),(0.,1.),(0.,0.0149999999999997),
 .UNSPECIFIED.);
#56798=B_SPLINE_SURFACE_WITH_KNOTS('',2,1,((#82231,#82232),(#82233,#82234),
(#82235,#82236)),.UNSPECIFIED.,.F.,.F.,.F.,(3,3),(2,2),(0.,1.),(0.,0.0149999999999997),
 .UNSPECIFIED.);
#56799=B_SPLINE_SURFACE_WITH_KNOTS('',2,1,((#82246,#82247),(#82248,#82249),
(#82250,#82251)),.UNSPECIFIED.,.F.,.F.,.F.,(3,3),(2,2),(0.,1.),(0.,0.0149999999999997),
 .UNSPECIFIED.);
#56800=B_SPLINE_SURFACE_WITH_KNOTS('',2,1,((#82261,#82262),(#82263,#82264),
(#82265,#82266)),.UNSPECIFIED.,.F.,.F.,.F.,(3,3),(2,2),(0.,1.),(0.,0.0149999999999997),
 .UNSPECIFIED.);
#56801=B_SPLINE_SURFACE_WITH_KNOTS('',2,1,((#82276,#82277),(#82278,#82279),
(#82280,#82281)),.UNSPECIFIED.,.F.,.F.,.F.,(3,3),(2,2),(0.,1.),(0.,0.0149999999999997),
 .UNSPECIFIED.);
#56802=B_SPLINE_SURFACE_WITH_KNOTS('',2,1,((#82291,#82292),(#82293,#82294),
(#82295,#82296)),.UNSPECIFIED.,.F.,.F.,.F.,(3,3),(2,2),(0.,1.),(0.,0.0149999999999997),
 .UNSPECIFIED.);
#56803=B_SPLINE_SURFACE_WITH_KNOTS('',2,1,((#82306,#82307),(#82308,#82309),
(#82310,#82311)),.UNSPECIFIED.,.F.,.F.,.F.,(3,3),(2,2),(0.,1.),(0.,0.0149999999999997),
 .UNSPECIFIED.);
#56804=B_SPLINE_SURFACE_WITH_KNOTS('',2,1,((#82318,#82319),(#82320,#82321),
(#82322,#82323)),.UNSPECIFIED.,.F.,.F.,.F.,(3,3),(2,2),(0.,1.),(0.,0.0149999999999997),
 .UNSPECIFIED.);
#56805=B_SPLINE_SURFACE_WITH_KNOTS('',2,1,((#82336,#82337),(#82338,#82339),
(#82340,#82341)),.UNSPECIFIED.,.F.,.F.,.F.,(3,3),(2,2),(0.,1.),(0.,0.0149999999999997),
 .UNSPECIFIED.);
#56806=B_SPLINE_SURFACE_WITH_KNOTS('',2,1,((#82351,#82352),(#82353,#82354),
(#82355,#82356)),.UNSPECIFIED.,.F.,.F.,.F.,(3,3),(2,2),(0.,1.),(0.,0.0149999999999997),
 .UNSPECIFIED.);
#56807=B_SPLINE_SURFACE_WITH_KNOTS('',2,1,((#82366,#82367),(#82368,#82369),
(#82370,#82371)),.UNSPECIFIED.,.F.,.F.,.F.,(3,3),(2,2),(0.,1.),(0.,0.0149999999999997),
 .UNSPECIFIED.);
#56808=B_SPLINE_SURFACE_WITH_KNOTS('',2,1,((#82381,#82382),(#82383,#82384),
(#82385,#82386)),.UNSPECIFIED.,.F.,.F.,.F.,(3,3),(2,2),(0.,1.),(0.,0.0149999999999997),
 .UNSPECIFIED.);
#56809=B_SPLINE_SURFACE_WITH_KNOTS('',2,1,((#82396,#82397),(#82398,#82399),
(#82400,#82401)),.UNSPECIFIED.,.F.,.F.,.F.,(3,3),(2,2),(0.,1.),(0.,0.0149999999999997),
 .UNSPECIFIED.);
#56810=B_SPLINE_SURFACE_WITH_KNOTS('',2,1,((#82411,#82412),(#82413,#82414),
(#82415,#82416)),.UNSPECIFIED.,.F.,.F.,.F.,(3,3),(2,2),(0.,1.),(0.,0.0149999999999997),
 .UNSPECIFIED.);
#56811=B_SPLINE_SURFACE_WITH_KNOTS('',2,1,((#82426,#82427),(#82428,#82429),
(#82430,#82431)),.UNSPECIFIED.,.F.,.F.,.F.,(3,3),(2,2),(0.,1.),(0.,0.0149999999999997),
 .UNSPECIFIED.);
#56812=B_SPLINE_SURFACE_WITH_KNOTS('',2,1,((#82441,#82442),(#82443,#82444),
(#82445,#82446)),.UNSPECIFIED.,.F.,.F.,.F.,(3,3),(2,2),(0.,1.),(0.,0.0149999999999997),
 .UNSPECIFIED.);
#56813=B_SPLINE_SURFACE_WITH_KNOTS('',2,1,((#82456,#82457),(#82458,#82459),
(#82460,#82461)),.UNSPECIFIED.,.F.,.F.,.F.,(3,3),(2,2),(0.,1.),(0.,0.0149999999999997),
 .UNSPECIFIED.);
#56814=B_SPLINE_SURFACE_WITH_KNOTS('',2,1,((#82471,#82472),(#82473,#82474),
(#82475,#82476)),.UNSPECIFIED.,.F.,.F.,.F.,(3,3),(2,2),(0.,1.),(0.,0.0149999999999997),
 .UNSPECIFIED.);
#56815=B_SPLINE_SURFACE_WITH_KNOTS('',2,1,((#82486,#82487),(#82488,#82489),
(#82490,#82491)),.UNSPECIFIED.,.F.,.F.,.F.,(3,3),(2,2),(0.,1.),(0.,0.0149999999999997),
 .UNSPECIFIED.);
#56816=B_SPLINE_SURFACE_WITH_KNOTS('',2,1,((#82499,#82500),(#82501,#82502),
(#82503,#82504)),.UNSPECIFIED.,.F.,.F.,.F.,(3,3),(2,2),(0.,1.),(0.,0.0149999999999997),
 .UNSPECIFIED.);
#56817=B_SPLINE_SURFACE_WITH_KNOTS('',2,1,((#82517,#82518),(#82519,#82520),
(#82521,#82522)),.UNSPECIFIED.,.F.,.F.,.F.,(3,3),(2,2),(0.,1.),(0.,0.0149999999999997),
 .UNSPECIFIED.);
#56818=B_SPLINE_SURFACE_WITH_KNOTS('',2,1,((#82532,#82533),(#82534,#82535),
(#82536,#82537)),.UNSPECIFIED.,.F.,.F.,.F.,(3,3),(2,2),(0.,1.),(0.,0.0149999999999997),
 .UNSPECIFIED.);
#56819=B_SPLINE_SURFACE_WITH_KNOTS('',2,1,((#82547,#82548),(#82549,#82550),
(#82551,#82552)),.UNSPECIFIED.,.F.,.F.,.F.,(3,3),(2,2),(0.,1.),(0.,0.0149999999999997),
 .UNSPECIFIED.);
#56820=B_SPLINE_SURFACE_WITH_KNOTS('',2,1,((#82562,#82563),(#82564,#82565),
(#82566,#82567)),.UNSPECIFIED.,.F.,.F.,.F.,(3,3),(2,2),(0.,1.),(0.,0.0149999999999997),
 .UNSPECIFIED.);
#56821=B_SPLINE_SURFACE_WITH_KNOTS('',2,1,((#82577,#82578),(#82579,#82580),
(#82581,#82582)),.UNSPECIFIED.,.F.,.F.,.F.,(3,3),(2,2),(0.,1.),(0.,0.0149999999999997),
 .UNSPECIFIED.);
#56822=B_SPLINE_SURFACE_WITH_KNOTS('',2,1,((#82592,#82593),(#82594,#82595),
(#82596,#82597)),.UNSPECIFIED.,.F.,.F.,.F.,(3,3),(2,2),(0.,1.),(0.,0.0149999999999997),
 .UNSPECIFIED.);
#56823=B_SPLINE_SURFACE_WITH_KNOTS('',2,1,((#82607,#82608),(#82609,#82610),
(#82611,#82612)),.UNSPECIFIED.,.F.,.F.,.F.,(3,3),(2,2),(0.,1.),(0.,0.0149999999999997),
 .UNSPECIFIED.);
#56824=B_SPLINE_SURFACE_WITH_KNOTS('',2,1,((#82622,#82623),(#82624,#82625),
(#82626,#82627)),.UNSPECIFIED.,.F.,.F.,.F.,(3,3),(2,2),(0.,1.),(0.,0.0149999999999997),
 .UNSPECIFIED.);
#56825=B_SPLINE_SURFACE_WITH_KNOTS('',2,1,((#82643,#82644),(#82645,#82646),
(#82647,#82648)),.UNSPECIFIED.,.F.,.F.,.F.,(3,3),(2,2),(0.,1.),(0.,0.0149999999999997),
 .UNSPECIFIED.);
#56826=B_SPLINE_SURFACE_WITH_KNOTS('',2,1,((#82658,#82659),(#82660,#82661),
(#82662,#82663)),.UNSPECIFIED.,.F.,.F.,.F.,(3,3),(2,2),(0.,1.),(0.,0.0149999999999997),
 .UNSPECIFIED.);
#56827=B_SPLINE_SURFACE_WITH_KNOTS('',2,1,((#82673,#82674),(#82675,#82676),
(#82677,#82678)),.UNSPECIFIED.,.F.,.F.,.F.,(3,3),(2,2),(0.,1.),(0.,0.0149999999999997),
 .UNSPECIFIED.);
#56828=B_SPLINE_SURFACE_WITH_KNOTS('',2,1,((#82688,#82689),(#82690,#82691),
(#82692,#82693)),.UNSPECIFIED.,.F.,.F.,.F.,(3,3),(2,2),(0.,1.),(0.,0.0149999999999997),
 .UNSPECIFIED.);
#56829=B_SPLINE_SURFACE_WITH_KNOTS('',2,1,((#82703,#82704),(#82705,#82706),
(#82707,#82708)),.UNSPECIFIED.,.F.,.F.,.F.,(3,3),(2,2),(0.,1.),(0.,0.0149999999999997),
 .UNSPECIFIED.);
#56830=B_SPLINE_SURFACE_WITH_KNOTS('',2,1,((#82718,#82719),(#82720,#82721),
(#82722,#82723)),.UNSPECIFIED.,.F.,.F.,.F.,(3,3),(2,2),(0.,1.),(0.,0.0149999999999997),
 .UNSPECIFIED.);
#56831=B_SPLINE_SURFACE_WITH_KNOTS('',2,1,((#82733,#82734),(#82735,#82736),
(#82737,#82738)),.UNSPECIFIED.,.F.,.F.,.F.,(3,3),(2,2),(0.,1.),(0.,0.0149999999999997),
 .UNSPECIFIED.);
#56832=B_SPLINE_SURFACE_WITH_KNOTS('',2,1,((#82748,#82749),(#82750,#82751),
(#82752,#82753)),.UNSPECIFIED.,.F.,.F.,.F.,(3,3),(2,2),(0.,1.),(0.,0.0149999999999997),
 .UNSPECIFIED.);
#56833=B_SPLINE_SURFACE_WITH_KNOTS('',2,1,((#82763,#82764),(#82765,#82766),
(#82767,#82768)),.UNSPECIFIED.,.F.,.F.,.F.,(3,3),(2,2),(0.,1.),(0.,0.0149999999999997),
 .UNSPECIFIED.);
#56834=B_SPLINE_SURFACE_WITH_KNOTS('',2,1,((#82795,#82796),(#82797,#82798),
(#82799,#82800)),.UNSPECIFIED.,.F.,.F.,.F.,(3,3),(2,2),(0.,1.),(0.,0.0149999999999997),
 .UNSPECIFIED.);
#56835=B_SPLINE_SURFACE_WITH_KNOTS('',2,1,((#82813,#82814),(#82815,#82816),
(#82817,#82818)),.UNSPECIFIED.,.F.,.F.,.F.,(3,3),(2,2),(0.,1.),(0.,0.0149999999999997),
 .UNSPECIFIED.);
#56836=B_SPLINE_SURFACE_WITH_KNOTS('',2,1,((#82828,#82829),(#82830,#82831),
(#82832,#82833)),.UNSPECIFIED.,.F.,.F.,.F.,(3,3),(2,2),(0.,1.),(0.,0.0149999999999997),
 .UNSPECIFIED.);
#56837=B_SPLINE_SURFACE_WITH_KNOTS('',2,1,((#82843,#82844),(#82845,#82846),
(#82847,#82848)),.UNSPECIFIED.,.F.,.F.,.F.,(3,3),(2,2),(0.,1.),(0.,0.0149999999999997),
 .UNSPECIFIED.);
#56838=B_SPLINE_SURFACE_WITH_KNOTS('',2,1,((#82858,#82859),(#82860,#82861),
(#82862,#82863)),.UNSPECIFIED.,.F.,.F.,.F.,(3,3),(2,2),(0.,1.),(0.,0.0149999999999997),
 .UNSPECIFIED.);
#56839=B_SPLINE_SURFACE_WITH_KNOTS('',2,1,((#82873,#82874),(#82875,#82876),
(#82877,#82878)),.UNSPECIFIED.,.F.,.F.,.F.,(3,3),(2,2),(0.,1.),(0.,0.0149999999999997),
 .UNSPECIFIED.);
#56840=B_SPLINE_SURFACE_WITH_KNOTS('',2,1,((#82888,#82889),(#82890,#82891),
(#82892,#82893)),.UNSPECIFIED.,.F.,.F.,.F.,(3,3),(2,2),(0.,1.),(0.,0.0149999999999997),
 .UNSPECIFIED.);
#56841=B_SPLINE_SURFACE_WITH_KNOTS('',2,1,((#82903,#82904),(#82905,#82906),
(#82907,#82908)),.UNSPECIFIED.,.F.,.F.,.F.,(3,3),(2,2),(0.,1.),(0.,0.0149999999999997),
 .UNSPECIFIED.);
#56842=B_SPLINE_SURFACE_WITH_KNOTS('',2,1,((#82915,#82916),(#82917,#82918),
(#82919,#82920)),.UNSPECIFIED.,.F.,.F.,.F.,(3,3),(2,2),(0.,1.),(0.,0.0149999999999997),
 .UNSPECIFIED.);
#56843=B_SPLINE_SURFACE_WITH_KNOTS('',2,1,((#82933,#82934),(#82935,#82936),
(#82937,#82938)),.UNSPECIFIED.,.F.,.F.,.F.,(3,3),(2,2),(0.,1.),(0.,0.0149999999999997),
 .UNSPECIFIED.);
#56844=B_SPLINE_SURFACE_WITH_KNOTS('',2,1,((#82948,#82949),(#82950,#82951),
(#82952,#82953)),.UNSPECIFIED.,.F.,.F.,.F.,(3,3),(2,2),(0.,1.),(0.,0.0149999999999997),
 .UNSPECIFIED.);
#56845=B_SPLINE_SURFACE_WITH_KNOTS('',2,1,((#82963,#82964),(#82965,#82966),
(#82967,#82968)),.UNSPECIFIED.,.F.,.F.,.F.,(3,3),(2,2),(0.,1.),(0.,0.0149999999999997),
 .UNSPECIFIED.);
#56846=B_SPLINE_SURFACE_WITH_KNOTS('',2,1,((#82978,#82979),(#82980,#82981),
(#82982,#82983)),.UNSPECIFIED.,.F.,.F.,.F.,(3,3),(2,2),(0.,1.),(0.,0.0149999999999997),
 .UNSPECIFIED.);
#56847=B_SPLINE_SURFACE_WITH_KNOTS('',2,1,((#82993,#82994),(#82995,#82996),
(#82997,#82998)),.UNSPECIFIED.,.F.,.F.,.F.,(3,3),(2,2),(0.,1.),(0.,0.0149999999999997),
 .UNSPECIFIED.);
#56848=B_SPLINE_SURFACE_WITH_KNOTS('',2,1,((#83008,#83009),(#83010,#83011),
(#83012,#83013)),.UNSPECIFIED.,.F.,.F.,.F.,(3,3),(2,2),(0.,1.),(0.,0.0149999999999997),
 .UNSPECIFIED.);
#56849=B_SPLINE_SURFACE_WITH_KNOTS('',2,1,((#83023,#83024),(#83025,#83026),
(#83027,#83028)),.UNSPECIFIED.,.F.,.F.,.F.,(3,3),(2,2),(0.,1.),(0.,0.0149999999999997),
 .UNSPECIFIED.);
#56850=B_SPLINE_SURFACE_WITH_KNOTS('',2,1,((#83038,#83039),(#83040,#83041),
(#83042,#83043)),.UNSPECIFIED.,.F.,.F.,.F.,(3,3),(2,2),(0.,1.),(0.,0.0149999999999997),
 .UNSPECIFIED.);
#56851=B_SPLINE_SURFACE_WITH_KNOTS('',2,1,((#83053,#83054),(#83055,#83056),
(#83057,#83058)),.UNSPECIFIED.,.F.,.F.,.F.,(3,3),(2,2),(0.,1.),(0.,0.0149999999999997),
 .UNSPECIFIED.);
#56852=B_SPLINE_SURFACE_WITH_KNOTS('',2,1,((#83068,#83069),(#83070,#83071),
(#83072,#83073)),.UNSPECIFIED.,.F.,.F.,.F.,(3,3),(2,2),(0.,1.),(0.,0.0149999999999997),
 .UNSPECIFIED.);
#56853=B_SPLINE_SURFACE_WITH_KNOTS('',2,1,((#83083,#83084),(#83085,#83086),
(#83087,#83088)),.UNSPECIFIED.,.F.,.F.,.F.,(3,3),(2,2),(0.,1.),(0.,0.0149999999999997),
 .UNSPECIFIED.);
#56854=B_SPLINE_SURFACE_WITH_KNOTS('',2,1,((#83096,#83097),(#83098,#83099),
(#83100,#83101)),.UNSPECIFIED.,.F.,.F.,.F.,(3,3),(2,2),(0.,1.),(0.,0.0149999999999997),
 .UNSPECIFIED.);
#56855=B_SPLINE_SURFACE_WITH_KNOTS('',2,1,((#83114,#83115),(#83116,#83117),
(#83118,#83119)),.UNSPECIFIED.,.F.,.F.,.F.,(3,3),(2,2),(0.,1.),(0.,0.0149999999999997),
 .UNSPECIFIED.);
#56856=B_SPLINE_SURFACE_WITH_KNOTS('',2,1,((#83129,#83130),(#83131,#83132),
(#83133,#83134)),.UNSPECIFIED.,.F.,.F.,.F.,(3,3),(2,2),(0.,1.),(0.,0.0149999999999997),
 .UNSPECIFIED.);
#56857=B_SPLINE_SURFACE_WITH_KNOTS('',2,1,((#83144,#83145),(#83146,#83147),
(#83148,#83149)),.UNSPECIFIED.,.F.,.F.,.F.,(3,3),(2,2),(0.,1.),(0.,0.0149999999999997),
 .UNSPECIFIED.);
#56858=B_SPLINE_SURFACE_WITH_KNOTS('',2,1,((#83159,#83160),(#83161,#83162),
(#83163,#83164)),.UNSPECIFIED.,.F.,.F.,.F.,(3,3),(2,2),(0.,1.),(0.,0.0149999999999997),
 .UNSPECIFIED.);
#56859=B_SPLINE_SURFACE_WITH_KNOTS('',2,1,((#83174,#83175),(#83176,#83177),
(#83178,#83179)),.UNSPECIFIED.,.F.,.F.,.F.,(3,3),(2,2),(0.,1.),(0.,0.0149999999999997),
 .UNSPECIFIED.);
#56860=B_SPLINE_SURFACE_WITH_KNOTS('',2,1,((#83189,#83190),(#83191,#83192),
(#83193,#83194)),.UNSPECIFIED.,.F.,.F.,.F.,(3,3),(2,2),(0.,1.),(0.,0.0149999999999997),
 .UNSPECIFIED.);
#56861=B_SPLINE_SURFACE_WITH_KNOTS('',2,1,((#83204,#83205),(#83206,#83207),
(#83208,#83209)),.UNSPECIFIED.,.F.,.F.,.F.,(3,3),(2,2),(0.,1.),(0.,0.0149999999999997),
 .UNSPECIFIED.);
#56862=B_SPLINE_SURFACE_WITH_KNOTS('',2,1,((#83219,#83220),(#83221,#83222),
(#83223,#83224)),.UNSPECIFIED.,.F.,.F.,.F.,(3,3),(2,2),(0.,1.),(0.,0.0149999999999997),
 .UNSPECIFIED.);
#56863=B_SPLINE_SURFACE_WITH_KNOTS('',2,1,((#83234,#83235),(#83236,#83237),
(#83238,#83239)),.UNSPECIFIED.,.F.,.F.,.F.,(3,3),(2,2),(0.,1.),(0.,0.0149999999999997),
 .UNSPECIFIED.);
#56864=B_SPLINE_SURFACE_WITH_KNOTS('',2,1,((#83249,#83250),(#83251,#83252),
(#83253,#83254)),.UNSPECIFIED.,.F.,.F.,.F.,(3,3),(2,2),(0.,1.),(0.,0.0149999999999997),
 .UNSPECIFIED.);
#56865=B_SPLINE_SURFACE_WITH_KNOTS('',2,1,((#83264,#83265),(#83266,#83267),
(#83268,#83269)),.UNSPECIFIED.,.F.,.F.,.F.,(3,3),(2,2),(0.,1.),(0.,0.0149999999999997),
 .UNSPECIFIED.);
#56866=B_SPLINE_SURFACE_WITH_KNOTS('',2,1,((#83285,#83286),(#83287,#83288),
(#83289,#83290)),.UNSPECIFIED.,.F.,.F.,.F.,(3,3),(2,2),(0.,1.),(0.,0.0149999999999997),
 .UNSPECIFIED.);
#56867=B_SPLINE_SURFACE_WITH_KNOTS('',2,1,((#83300,#83301),(#83302,#83303),
(#83304,#83305)),.UNSPECIFIED.,.F.,.F.,.F.,(3,3),(2,2),(0.,1.),(0.,0.0149999999999997),
 .UNSPECIFIED.);
#56868=B_SPLINE_SURFACE_WITH_KNOTS('',2,1,((#83315,#83316),(#83317,#83318),
(#83319,#83320)),.UNSPECIFIED.,.F.,.F.,.F.,(3,3),(2,2),(0.,1.),(0.,0.0149999999999997),
 .UNSPECIFIED.);
#56869=B_SPLINE_SURFACE_WITH_KNOTS('',2,1,((#83330,#83331),(#83332,#83333),
(#83334,#83335)),.UNSPECIFIED.,.F.,.F.,.F.,(3,3),(2,2),(0.,1.),(0.,0.0149999999999997),
 .UNSPECIFIED.);
#56870=B_SPLINE_SURFACE_WITH_KNOTS('',2,1,((#83345,#83346),(#83347,#83348),
(#83349,#83350)),.UNSPECIFIED.,.F.,.F.,.F.,(3,3),(2,2),(0.,1.),(0.,0.0149999999999997),
 .UNSPECIFIED.);
#56871=B_SPLINE_SURFACE_WITH_KNOTS('',2,1,((#83360,#83361),(#83362,#83363),
(#83364,#83365)),.UNSPECIFIED.,.F.,.F.,.F.,(3,3),(2,2),(0.,1.),(0.,0.0149999999999997),
 .UNSPECIFIED.);
#56872=B_SPLINE_SURFACE_WITH_KNOTS('',2,1,((#83375,#83376),(#83377,#83378),
(#83379,#83380)),.UNSPECIFIED.,.F.,.F.,.F.,(3,3),(2,2),(0.,1.),(0.,0.0149999999999997),
 .UNSPECIFIED.);
#56873=B_SPLINE_SURFACE_WITH_KNOTS('',2,1,((#83396,#83397),(#83398,#83399),
(#83400,#83401)),.UNSPECIFIED.,.F.,.F.,.F.,(3,3),(2,2),(0.,1.),(0.,0.0149999999999997),
 .UNSPECIFIED.);
#56874=B_SPLINE_SURFACE_WITH_KNOTS('',2,1,((#83411,#83412),(#83413,#83414),
(#83415,#83416)),.UNSPECIFIED.,.F.,.F.,.F.,(3,3),(2,2),(0.,1.),(0.,0.0149999999999997),
 .UNSPECIFIED.);
#56875=B_SPLINE_SURFACE_WITH_KNOTS('',2,1,((#83426,#83427),(#83428,#83429),
(#83430,#83431)),.UNSPECIFIED.,.F.,.F.,.F.,(3,3),(2,2),(0.,1.),(0.,0.0149999999999997),
 .UNSPECIFIED.);
#56876=B_SPLINE_SURFACE_WITH_KNOTS('',2,1,((#83441,#83442),(#83443,#83444),
(#83445,#83446)),.UNSPECIFIED.,.F.,.F.,.F.,(3,3),(2,2),(0.,1.),(0.,0.0149999999999997),
 .UNSPECIFIED.);
#56877=B_SPLINE_SURFACE_WITH_KNOTS('',2,1,((#83456,#83457),(#83458,#83459),
(#83460,#83461)),.UNSPECIFIED.,.F.,.F.,.F.,(3,3),(2,2),(0.,1.),(0.,0.0149999999999997),
 .UNSPECIFIED.);
#56878=B_SPLINE_SURFACE_WITH_KNOTS('',2,1,((#83471,#83472),(#83473,#83474),
(#83475,#83476)),.UNSPECIFIED.,.F.,.F.,.F.,(3,3),(2,2),(0.,1.),(0.,0.0149999999999997),
 .UNSPECIFIED.);
#56879=B_SPLINE_SURFACE_WITH_KNOTS('',2,1,((#83486,#83487),(#83488,#83489),
(#83490,#83491)),.UNSPECIFIED.,.F.,.F.,.F.,(3,3),(2,2),(0.,1.),(0.,0.0149999999999997),
 .UNSPECIFIED.);
#56880=B_SPLINE_SURFACE_WITH_KNOTS('',2,1,((#83507,#83508),(#83509,#83510),
(#83511,#83512)),.UNSPECIFIED.,.F.,.F.,.F.,(3,3),(2,2),(0.,1.),(0.,0.0149999999999997),
 .UNSPECIFIED.);
#56881=B_SPLINE_SURFACE_WITH_KNOTS('',2,1,((#83521,#83522),(#83523,#83524),
(#83525,#83526)),.UNSPECIFIED.,.F.,.F.,.F.,(3,3),(2,2),(0.,1.),(0.,0.0149999999999997),
 .UNSPECIFIED.);
#56882=B_SPLINE_SURFACE_WITH_KNOTS('',2,1,((#83539,#83540),(#83541,#83542),
(#83543,#83544)),.UNSPECIFIED.,.F.,.F.,.F.,(3,3),(2,2),(0.,1.),(0.,0.0149999999999997),
 .UNSPECIFIED.);
#56883=B_SPLINE_SURFACE_WITH_KNOTS('',2,1,((#83554,#83555),(#83556,#83557),
(#83558,#83559)),.UNSPECIFIED.,.F.,.F.,.F.,(3,3),(2,2),(0.,1.),(0.,0.0149999999999997),
 .UNSPECIFIED.);
#56884=B_SPLINE_SURFACE_WITH_KNOTS('',2,1,((#83569,#83570),(#83571,#83572),
(#83573,#83574)),.UNSPECIFIED.,.F.,.F.,.F.,(3,3),(2,2),(0.,1.),(0.,0.0149999999999997),
 .UNSPECIFIED.);
#56885=B_SPLINE_SURFACE_WITH_KNOTS('',2,1,((#83584,#83585),(#83586,#83587),
(#83588,#83589)),.UNSPECIFIED.,.F.,.F.,.F.,(3,3),(2,2),(0.,1.),(0.,0.0149999999999997),
 .UNSPECIFIED.);
#56886=B_SPLINE_SURFACE_WITH_KNOTS('',2,1,((#83599,#83600),(#83601,#83602),
(#83603,#83604)),.UNSPECIFIED.,.F.,.F.,.F.,(3,3),(2,2),(0.,1.),(0.,0.0149999999999997),
 .UNSPECIFIED.);
#56887=B_SPLINE_SURFACE_WITH_KNOTS('',2,1,((#83614,#83615),(#83616,#83617),
(#83618,#83619)),.UNSPECIFIED.,.F.,.F.,.F.,(3,3),(2,2),(0.,1.),(0.,0.0149999999999997),
 .UNSPECIFIED.);
#56888=B_SPLINE_SURFACE_WITH_KNOTS('',2,1,((#83629,#83630),(#83631,#83632),
(#83633,#83634)),.UNSPECIFIED.,.F.,.F.,.F.,(3,3),(2,2),(0.,1.),(0.,0.0149999999999997),
 .UNSPECIFIED.);
#56889=B_SPLINE_SURFACE_WITH_KNOTS('',2,1,((#83641,#83642),(#83643,#83644),
(#83645,#83646)),.UNSPECIFIED.,.F.,.F.,.F.,(3,3),(2,2),(0.,1.),(0.,0.0149999999999997),
 .UNSPECIFIED.);
#56890=B_SPLINE_SURFACE_WITH_KNOTS('',2,1,((#83659,#83660),(#83661,#83662),
(#83663,#83664)),.UNSPECIFIED.,.F.,.F.,.F.,(3,3),(2,2),(0.,1.),(0.,0.0149999999999997),
 .UNSPECIFIED.);
#56891=B_SPLINE_SURFACE_WITH_KNOTS('',2,1,((#83674,#83675),(#83676,#83677),
(#83678,#83679)),.UNSPECIFIED.,.F.,.F.,.F.,(3,3),(2,2),(0.,1.),(0.,0.0149999999999997),
 .UNSPECIFIED.);
#56892=B_SPLINE_SURFACE_WITH_KNOTS('',2,1,((#83689,#83690),(#83691,#83692),
(#83693,#83694)),.UNSPECIFIED.,.F.,.F.,.F.,(3,3),(2,2),(0.,1.),(0.,0.0149999999999997),
 .UNSPECIFIED.);
#56893=B_SPLINE_SURFACE_WITH_KNOTS('',2,1,((#83704,#83705),(#83706,#83707),
(#83708,#83709)),.UNSPECIFIED.,.F.,.F.,.F.,(3,3),(2,2),(0.,1.),(0.,0.0149999999999997),
 .UNSPECIFIED.);
#56894=B_SPLINE_SURFACE_WITH_KNOTS('',2,1,((#83719,#83720),(#83721,#83722),
(#83723,#83724)),.UNSPECIFIED.,.F.,.F.,.F.,(3,3),(2,2),(0.,1.),(0.,0.0149999999999997),
 .UNSPECIFIED.);
#56895=B_SPLINE_SURFACE_WITH_KNOTS('',2,1,((#83734,#83735),(#83736,#83737),
(#83738,#83739)),.UNSPECIFIED.,.F.,.F.,.F.,(3,3),(2,2),(0.,1.),(0.,0.0149999999999997),
 .UNSPECIFIED.);
#56896=B_SPLINE_SURFACE_WITH_KNOTS('',2,1,((#83749,#83750),(#83751,#83752),
(#83753,#83754)),.UNSPECIFIED.,.F.,.F.,.F.,(3,3),(2,2),(0.,1.),(0.,0.0149999999999997),
 .UNSPECIFIED.);
#56897=B_SPLINE_SURFACE_WITH_KNOTS('',2,1,((#83764,#83765),(#83766,#83767),
(#83768,#83769)),.UNSPECIFIED.,.F.,.F.,.F.,(3,3),(2,2),(0.,1.),(0.,0.0149999999999997),
 .UNSPECIFIED.);
#56898=B_SPLINE_SURFACE_WITH_KNOTS('',2,1,((#83779,#83780),(#83781,#83782),
(#83783,#83784)),.UNSPECIFIED.,.F.,.F.,.F.,(3,3),(2,2),(0.,1.),(0.,0.0149999999999997),
 .UNSPECIFIED.);
#56899=B_SPLINE_SURFACE_WITH_KNOTS('',2,1,((#83794,#83795),(#83796,#83797),
(#83798,#83799)),.UNSPECIFIED.,.F.,.F.,.F.,(3,3),(2,2),(0.,1.),(0.,0.0149999999999997),
 .UNSPECIFIED.);
#56900=B_SPLINE_SURFACE_WITH_KNOTS('',2,1,((#83809,#83810),(#83811,#83812),
(#83813,#83814)),.UNSPECIFIED.,.F.,.F.,.F.,(3,3),(2,2),(0.,1.),(0.,0.0149999999999997),
 .UNSPECIFIED.);
#56901=B_SPLINE_SURFACE_WITH_KNOTS('',2,1,((#83909,#83910),(#83911,#83912),
(#83913,#83914)),.UNSPECIFIED.,.F.,.F.,.F.,(3,3),(2,2),(0.,1.),(0.,0.0149999999999997),
 .UNSPECIFIED.);
#56902=B_SPLINE_SURFACE_WITH_KNOTS('',2,1,((#83927,#83928),(#83929,#83930),
(#83931,#83932)),.UNSPECIFIED.,.F.,.F.,.F.,(3,3),(2,2),(0.,1.),(0.,0.0149999999999997),
 .UNSPECIFIED.);
#56903=B_SPLINE_SURFACE_WITH_KNOTS('',2,1,((#83942,#83943),(#83944,#83945),
(#83946,#83947)),.UNSPECIFIED.,.F.,.F.,.F.,(3,3),(2,2),(0.,1.),(0.,0.0149999999999997),
 .UNSPECIFIED.);
#56904=B_SPLINE_SURFACE_WITH_KNOTS('',2,1,((#83957,#83958),(#83959,#83960),
(#83961,#83962)),.UNSPECIFIED.,.F.,.F.,.F.,(3,3),(2,2),(0.,1.),(0.,0.0149999999999997),
 .UNSPECIFIED.);
#56905=B_SPLINE_SURFACE_WITH_KNOTS('',2,1,((#83972,#83973),(#83974,#83975),
(#83976,#83977)),.UNSPECIFIED.,.F.,.F.,.F.,(3,3),(2,2),(0.,1.),(0.,0.0149999999999997),
 .UNSPECIFIED.);
#56906=B_SPLINE_SURFACE_WITH_KNOTS('',2,1,((#83987,#83988),(#83989,#83990),
(#83991,#83992)),.UNSPECIFIED.,.F.,.F.,.F.,(3,3),(2,2),(0.,1.),(0.,0.0149999999999997),
 .UNSPECIFIED.);
#56907=B_SPLINE_SURFACE_WITH_KNOTS('',2,1,((#84002,#84003),(#84004,#84005),
(#84006,#84007)),.UNSPECIFIED.,.F.,.F.,.F.,(3,3),(2,2),(0.,1.),(0.,0.0149999999999997),
 .UNSPECIFIED.);
#56908=B_SPLINE_SURFACE_WITH_KNOTS('',2,1,((#84017,#84018),(#84019,#84020),
(#84021,#84022)),.UNSPECIFIED.,.F.,.F.,.F.,(3,3),(2,2),(0.,1.),(0.,0.0149999999999997),
 .UNSPECIFIED.);
#56909=B_SPLINE_SURFACE_WITH_KNOTS('',2,1,((#84029,#84030),(#84031,#84032),
(#84033,#84034)),.UNSPECIFIED.,.F.,.F.,.F.,(3,3),(2,2),(0.,1.),(0.,0.0149999999999997),
 .UNSPECIFIED.);
#56910=B_SPLINE_SURFACE_WITH_KNOTS('',2,1,((#84047,#84048),(#84049,#84050),
(#84051,#84052)),.UNSPECIFIED.,.F.,.F.,.F.,(3,3),(2,2),(0.,1.),(0.,0.0149999999999997),
 .UNSPECIFIED.);
#56911=B_SPLINE_SURFACE_WITH_KNOTS('',2,1,((#84062,#84063),(#84064,#84065),
(#84066,#84067)),.UNSPECIFIED.,.F.,.F.,.F.,(3,3),(2,2),(0.,1.),(0.,0.0149999999999997),
 .UNSPECIFIED.);
#56912=B_SPLINE_SURFACE_WITH_KNOTS('',2,1,((#84077,#84078),(#84079,#84080),
(#84081,#84082)),.UNSPECIFIED.,.F.,.F.,.F.,(3,3),(2,2),(0.,1.),(0.,0.0149999999999997),
 .UNSPECIFIED.);
#56913=B_SPLINE_SURFACE_WITH_KNOTS('',2,1,((#84092,#84093),(#84094,#84095),
(#84096,#84097)),.UNSPECIFIED.,.F.,.F.,.F.,(3,3),(2,2),(0.,1.),(0.,0.0149999999999997),
 .UNSPECIFIED.);
#56914=B_SPLINE_SURFACE_WITH_KNOTS('',2,1,((#84107,#84108),(#84109,#84110),
(#84111,#84112)),.UNSPECIFIED.,.F.,.F.,.F.,(3,3),(2,2),(0.,1.),(0.,0.0149999999999997),
 .UNSPECIFIED.);
#56915=B_SPLINE_SURFACE_WITH_KNOTS('',2,1,((#84122,#84123),(#84124,#84125),
(#84126,#84127)),.UNSPECIFIED.,.F.,.F.,.F.,(3,3),(2,2),(0.,1.),(0.,0.0149999999999997),
 .UNSPECIFIED.);
#56916=B_SPLINE_SURFACE_WITH_KNOTS('',2,1,((#84137,#84138),(#84139,#84140),
(#84141,#84142)),.UNSPECIFIED.,.F.,.F.,.F.,(3,3),(2,2),(0.,1.),(0.,0.0149999999999997),
 .UNSPECIFIED.);
#56917=B_SPLINE_SURFACE_WITH_KNOTS('',2,1,((#84152,#84153),(#84154,#84155),
(#84156,#84157)),.UNSPECIFIED.,.F.,.F.,.F.,(3,3),(2,2),(0.,1.),(0.,0.0149999999999997),
 .UNSPECIFIED.);
#56918=B_SPLINE_SURFACE_WITH_KNOTS('',2,1,((#84167,#84168),(#84169,#84170),
(#84171,#84172)),.UNSPECIFIED.,.F.,.F.,.F.,(3,3),(2,2),(0.,1.),(0.,0.0149999999999997),
 .UNSPECIFIED.);
#56919=B_SPLINE_SURFACE_WITH_KNOTS('',2,1,((#84182,#84183),(#84184,#84185),
(#84186,#84187)),.UNSPECIFIED.,.F.,.F.,.F.,(3,3),(2,2),(0.,1.),(0.,0.0149999999999997),
 .UNSPECIFIED.);
#56920=B_SPLINE_SURFACE_WITH_KNOTS('',2,1,((#84197,#84198),(#84199,#84200),
(#84201,#84202)),.UNSPECIFIED.,.F.,.F.,.F.,(3,3),(2,2),(0.,1.),(0.,0.0149999999999997),
 .UNSPECIFIED.);
#56921=B_SPLINE_SURFACE_WITH_KNOTS('',2,1,((#84210,#84211),(#84212,#84213),
(#84214,#84215)),.UNSPECIFIED.,.F.,.F.,.F.,(3,3),(2,2),(0.,1.),(0.,0.0149999999999997),
 .UNSPECIFIED.);
#56922=B_SPLINE_SURFACE_WITH_KNOTS('',2,1,((#84228,#84229),(#84230,#84231),
(#84232,#84233)),.UNSPECIFIED.,.F.,.F.,.F.,(3,3),(2,2),(0.,1.),(0.,0.0149999999999997),
 .UNSPECIFIED.);
#56923=B_SPLINE_SURFACE_WITH_KNOTS('',2,1,((#84243,#84244),(#84245,#84246),
(#84247,#84248)),.UNSPECIFIED.,.F.,.F.,.F.,(3,3),(2,2),(0.,1.),(0.,0.0149999999999997),
 .UNSPECIFIED.);
#56924=B_SPLINE_SURFACE_WITH_KNOTS('',2,1,((#84258,#84259),(#84260,#84261),
(#84262,#84263)),.UNSPECIFIED.,.F.,.F.,.F.,(3,3),(2,2),(0.,1.),(0.,0.0149999999999997),
 .UNSPECIFIED.);
#56925=B_SPLINE_SURFACE_WITH_KNOTS('',2,1,((#84273,#84274),(#84275,#84276),
(#84277,#84278)),.UNSPECIFIED.,.F.,.F.,.F.,(3,3),(2,2),(0.,1.),(0.,0.0149999999999997),
 .UNSPECIFIED.);
#56926=B_SPLINE_SURFACE_WITH_KNOTS('',2,1,((#84288,#84289),(#84290,#84291),
(#84292,#84293)),.UNSPECIFIED.,.F.,.F.,.F.,(3,3),(2,2),(0.,1.),(0.,0.0149999999999997),
 .UNSPECIFIED.);
#56927=B_SPLINE_SURFACE_WITH_KNOTS('',2,1,((#84339,#84340),(#84341,#84342),
(#84343,#84344)),.UNSPECIFIED.,.F.,.F.,.F.,(3,3),(2,2),(0.,1.),(0.,0.0149999999999997),
 .UNSPECIFIED.);
#56928=B_SPLINE_SURFACE_WITH_KNOTS('',2,1,((#84354,#84355),(#84356,#84357),
(#84358,#84359)),.UNSPECIFIED.,.F.,.F.,.F.,(3,3),(2,2),(0.,1.),(0.,0.0149999999999997),
 .UNSPECIFIED.);
#56929=B_SPLINE_SURFACE_WITH_KNOTS('',2,1,((#84369,#84370),(#84371,#84372),
(#84373,#84374)),.UNSPECIFIED.,.F.,.F.,.F.,(3,3),(2,2),(0.,1.),(0.,0.0149999999999997),
 .UNSPECIFIED.);
#56930=B_SPLINE_SURFACE_WITH_KNOTS('',2,1,((#84384,#84385),(#84386,#84387),
(#84388,#84389)),.UNSPECIFIED.,.F.,.F.,.F.,(3,3),(2,2),(0.,1.),(0.,0.0149999999999997),
 .UNSPECIFIED.);
#56931=B_SPLINE_SURFACE_WITH_KNOTS('',2,1,((#84399,#84400),(#84401,#84402),
(#84403,#84404)),.UNSPECIFIED.,.F.,.F.,.F.,(3,3),(2,2),(0.,1.),(0.,0.0149999999999997),
 .UNSPECIFIED.);
#56932=B_SPLINE_SURFACE_WITH_KNOTS('',2,1,((#84414,#84415),(#84416,#84417),
(#84418,#84419)),.UNSPECIFIED.,.F.,.F.,.F.,(3,3),(2,2),(0.,1.),(0.,0.0149999999999997),
 .UNSPECIFIED.);
#56933=B_SPLINE_SURFACE_WITH_KNOTS('',2,1,((#84429,#84430),(#84431,#84432),
(#84433,#84434)),.UNSPECIFIED.,.F.,.F.,.F.,(3,3),(2,2),(0.,1.),(0.,0.0149999999999997),
 .UNSPECIFIED.);
#56934=B_SPLINE_SURFACE_WITH_KNOTS('',2,1,((#84444,#84445),(#84446,#84447),
(#84448,#84449)),.UNSPECIFIED.,.F.,.F.,.F.,(3,3),(2,2),(0.,1.),(0.,0.0149999999999997),
 .UNSPECIFIED.);
#56935=B_SPLINE_SURFACE_WITH_KNOTS('',2,1,((#84465,#84466),(#84467,#84468),
(#84469,#84470)),.UNSPECIFIED.,.F.,.F.,.F.,(3,3),(2,2),(0.,1.),(0.,0.0149999999999997),
 .UNSPECIFIED.);
#56936=B_SPLINE_SURFACE_WITH_KNOTS('',2,1,((#84479,#84480),(#84481,#84482),
(#84483,#84484)),.UNSPECIFIED.,.F.,.F.,.F.,(3,3),(2,2),(0.,1.),(0.,0.0149999999999997),
 .UNSPECIFIED.);
#56937=B_SPLINE_SURFACE_WITH_KNOTS('',2,1,((#84497,#84498),(#84499,#84500),
(#84501,#84502)),.UNSPECIFIED.,.F.,.F.,.F.,(3,3),(2,2),(0.,1.),(0.,0.0149999999999997),
 .UNSPECIFIED.);
#56938=B_SPLINE_SURFACE_WITH_KNOTS('',2,1,((#84512,#84513),(#84514,#84515),
(#84516,#84517)),.UNSPECIFIED.,.F.,.F.,.F.,(3,3),(2,2),(0.,1.),(0.,0.0149999999999997),
 .UNSPECIFIED.);
#56939=B_SPLINE_SURFACE_WITH_KNOTS('',2,1,((#84527,#84528),(#84529,#84530),
(#84531,#84532)),.UNSPECIFIED.,.F.,.F.,.F.,(3,3),(2,2),(0.,1.),(0.,0.0149999999999997),
 .UNSPECIFIED.);
#56940=B_SPLINE_SURFACE_WITH_KNOTS('',2,1,((#84542,#84543),(#84544,#84545),
(#84546,#84547)),.UNSPECIFIED.,.F.,.F.,.F.,(3,3),(2,2),(0.,1.),(0.,0.0149999999999997),
 .UNSPECIFIED.);
#56941=B_SPLINE_SURFACE_WITH_KNOTS('',2,1,((#84557,#84558),(#84559,#84560),
(#84561,#84562)),.UNSPECIFIED.,.F.,.F.,.F.,(3,3),(2,2),(0.,1.),(0.,0.0149999999999997),
 .UNSPECIFIED.);
#56942=B_SPLINE_SURFACE_WITH_KNOTS('',2,1,((#84572,#84573),(#84574,#84575),
(#84576,#84577)),.UNSPECIFIED.,.F.,.F.,.F.,(3,3),(2,2),(0.,1.),(0.,0.0149999999999997),
 .UNSPECIFIED.);
#56943=B_SPLINE_SURFACE_WITH_KNOTS('',2,1,((#84587,#84588),(#84589,#84590),
(#84591,#84592)),.UNSPECIFIED.,.F.,.F.,.F.,(3,3),(2,2),(0.,1.),(0.,0.0149999999999997),
 .UNSPECIFIED.);
#56944=B_SPLINE_SURFACE_WITH_KNOTS('',2,1,((#84599,#84600),(#84601,#84602),
(#84603,#84604)),.UNSPECIFIED.,.F.,.F.,.F.,(3,3),(2,2),(0.,1.),(0.,0.0149999999999997),
 .UNSPECIFIED.);
#56945=B_SPLINE_SURFACE_WITH_KNOTS('',2,1,((#84617,#84618),(#84619,#84620),
(#84621,#84622)),.UNSPECIFIED.,.F.,.F.,.F.,(3,3),(2,2),(0.,1.),(0.,0.0149999999999997),
 .UNSPECIFIED.);
#56946=B_SPLINE_SURFACE_WITH_KNOTS('',2,1,((#84632,#84633),(#84634,#84635),
(#84636,#84637)),.UNSPECIFIED.,.F.,.F.,.F.,(3,3),(2,2),(0.,1.),(0.,0.0149999999999997),
 .UNSPECIFIED.);
#56947=B_SPLINE_SURFACE_WITH_KNOTS('',2,1,((#84647,#84648),(#84649,#84650),
(#84651,#84652)),.UNSPECIFIED.,.F.,.F.,.F.,(3,3),(2,2),(0.,1.),(0.,0.0149999999999997),
 .UNSPECIFIED.);
#56948=B_SPLINE_SURFACE_WITH_KNOTS('',2,1,((#84662,#84663),(#84664,#84665),
(#84666,#84667)),.UNSPECIFIED.,.F.,.F.,.F.,(3,3),(2,2),(0.,1.),(0.,0.0149999999999997),
 .UNSPECIFIED.);
#56949=B_SPLINE_SURFACE_WITH_KNOTS('',2,1,((#84677,#84678),(#84679,#84680),
(#84681,#84682)),.UNSPECIFIED.,.F.,.F.,.F.,(3,3),(2,2),(0.,1.),(0.,0.0149999999999997),
 .UNSPECIFIED.);
#56950=B_SPLINE_SURFACE_WITH_KNOTS('',2,1,((#84692,#84693),(#84694,#84695),
(#84696,#84697)),.UNSPECIFIED.,.F.,.F.,.F.,(3,3),(2,2),(0.,1.),(0.,0.0149999999999997),
 .UNSPECIFIED.);
#56951=B_SPLINE_SURFACE_WITH_KNOTS('',2,1,((#84707,#84708),(#84709,#84710),
(#84711,#84712)),.UNSPECIFIED.,.F.,.F.,.F.,(3,3),(2,2),(0.,1.),(0.,0.0149999999999997),
 .UNSPECIFIED.);
#56952=B_SPLINE_SURFACE_WITH_KNOTS('',2,1,((#84722,#84723),(#84724,#84725),
(#84726,#84727)),.UNSPECIFIED.,.F.,.F.,.F.,(3,3),(2,2),(0.,1.),(0.,0.0149999999999997),
 .UNSPECIFIED.);
#56953=B_SPLINE_SURFACE_WITH_KNOTS('',2,1,((#84737,#84738),(#84739,#84740),
(#84741,#84742)),.UNSPECIFIED.,.F.,.F.,.F.,(3,3),(2,2),(0.,1.),(0.,0.0149999999999997),
 .UNSPECIFIED.);
#56954=B_SPLINE_SURFACE_WITH_KNOTS('',2,1,((#84752,#84753),(#84754,#84755),
(#84756,#84757)),.UNSPECIFIED.,.F.,.F.,.F.,(3,3),(2,2),(0.,1.),(0.,0.0149999999999997),
 .UNSPECIFIED.);
#56955=B_SPLINE_SURFACE_WITH_KNOTS('',2,1,((#84767,#84768),(#84769,#84770),
(#84771,#84772)),.UNSPECIFIED.,.F.,.F.,.F.,(3,3),(2,2),(0.,1.),(0.,0.0149999999999997),
 .UNSPECIFIED.);
#56956=B_SPLINE_SURFACE_WITH_KNOTS('',2,1,((#84780,#84781),(#84782,#84783),
(#84784,#84785)),.UNSPECIFIED.,.F.,.F.,.F.,(3,3),(2,2),(0.,1.),(0.,0.0149999999999997),
 .UNSPECIFIED.);
#56957=B_SPLINE_SURFACE_WITH_KNOTS('',2,1,((#84798,#84799),(#84800,#84801),
(#84802,#84803)),.UNSPECIFIED.,.F.,.F.,.F.,(3,3),(2,2),(0.,1.),(0.,0.0149999999999997),
 .UNSPECIFIED.);
#56958=B_SPLINE_SURFACE_WITH_KNOTS('',2,1,((#84813,#84814),(#84815,#84816),
(#84817,#84818)),.UNSPECIFIED.,.F.,.F.,.F.,(3,3),(2,2),(0.,1.),(0.,0.0149999999999997),
 .UNSPECIFIED.);
#56959=B_SPLINE_SURFACE_WITH_KNOTS('',2,1,((#84828,#84829),(#84830,#84831),
(#84832,#84833)),.UNSPECIFIED.,.F.,.F.,.F.,(3,3),(2,2),(0.,1.),(0.,0.0149999999999997),
 .UNSPECIFIED.);
#56960=B_SPLINE_SURFACE_WITH_KNOTS('',2,1,((#84843,#84844),(#84845,#84846),
(#84847,#84848)),.UNSPECIFIED.,.F.,.F.,.F.,(3,3),(2,2),(0.,1.),(0.,0.0149999999999997),
 .UNSPECIFIED.);
#56961=B_SPLINE_SURFACE_WITH_KNOTS('',2,1,((#84858,#84859),(#84860,#84861),
(#84862,#84863)),.UNSPECIFIED.,.F.,.F.,.F.,(3,3),(2,2),(0.,1.),(0.,0.0149999999999997),
 .UNSPECIFIED.);
#56962=B_SPLINE_SURFACE_WITH_KNOTS('',2,1,((#84873,#84874),(#84875,#84876),
(#84877,#84878)),.UNSPECIFIED.,.F.,.F.,.F.,(3,3),(2,2),(0.,1.),(0.,0.0149999999999997),
 .UNSPECIFIED.);
#56963=B_SPLINE_SURFACE_WITH_KNOTS('',2,1,((#84888,#84889),(#84890,#84891),
(#84892,#84893)),.UNSPECIFIED.,.F.,.F.,.F.,(3,3),(2,2),(0.,1.),(0.,0.0149999999999997),
 .UNSPECIFIED.);
#56964=B_SPLINE_SURFACE_WITH_KNOTS('',2,1,((#84903,#84904),(#84905,#84906),
(#84907,#84908)),.UNSPECIFIED.,.F.,.F.,.F.,(3,3),(2,2),(0.,1.),(0.,0.0149999999999997),
 .UNSPECIFIED.);
#56965=B_SPLINE_SURFACE_WITH_KNOTS('',2,1,((#84915,#84916),(#84917,#84918),
(#84919,#84920)),.UNSPECIFIED.,.F.,.F.,.F.,(3,3),(2,2),(0.,1.),(0.,0.0149999999999997),
 .UNSPECIFIED.);
#56966=B_SPLINE_SURFACE_WITH_KNOTS('',2,1,((#84933,#84934),(#84935,#84936),
(#84937,#84938)),.UNSPECIFIED.,.F.,.F.,.F.,(3,3),(2,2),(0.,1.),(0.,0.0149999999999997),
 .UNSPECIFIED.);
#56967=B_SPLINE_SURFACE_WITH_KNOTS('',2,1,((#84948,#84949),(#84950,#84951),
(#84952,#84953)),.UNSPECIFIED.,.F.,.F.,.F.,(3,3),(2,2),(0.,1.),(0.,0.0149999999999997),
 .UNSPECIFIED.);
#56968=B_SPLINE_SURFACE_WITH_KNOTS('',2,1,((#84963,#84964),(#84965,#84966),
(#84967,#84968)),.UNSPECIFIED.,.F.,.F.,.F.,(3,3),(2,2),(0.,1.),(0.,0.0149999999999997),
 .UNSPECIFIED.);
#56969=B_SPLINE_SURFACE_WITH_KNOTS('',2,1,((#84978,#84979),(#84980,#84981),
(#84982,#84983)),.UNSPECIFIED.,.F.,.F.,.F.,(3,3),(2,2),(0.,1.),(0.,0.0149999999999997),
 .UNSPECIFIED.);
#56970=B_SPLINE_SURFACE_WITH_KNOTS('',2,1,((#84993,#84994),(#84995,#84996),
(#84997,#84998)),.UNSPECIFIED.,.F.,.F.,.F.,(3,3),(2,2),(0.,1.),(0.,0.0149999999999997),
 .UNSPECIFIED.);
#56971=B_SPLINE_SURFACE_WITH_KNOTS('',2,1,((#85008,#85009),(#85010,#85011),
(#85012,#85013)),.UNSPECIFIED.,.F.,.F.,.F.,(3,3),(2,2),(0.,1.),(0.,0.0149999999999997),
 .UNSPECIFIED.);
#56972=B_SPLINE_SURFACE_WITH_KNOTS('',2,1,((#85023,#85024),(#85025,#85026),
(#85027,#85028)),.UNSPECIFIED.,.F.,.F.,.F.,(3,3),(2,2),(0.,1.),(0.,0.0149999999999997),
 .UNSPECIFIED.);
#56973=B_SPLINE_SURFACE_WITH_KNOTS('',2,1,((#85038,#85039),(#85040,#85041),
(#85042,#85043)),.UNSPECIFIED.,.F.,.F.,.F.,(3,3),(2,2),(0.,1.),(0.,0.0149999999999997),
 .UNSPECIFIED.);
#56974=B_SPLINE_SURFACE_WITH_KNOTS('',2,1,((#85053,#85054),(#85055,#85056),
(#85057,#85058)),.UNSPECIFIED.,.F.,.F.,.F.,(3,3),(2,2),(0.,1.),(0.,0.0149999999999997),
 .UNSPECIFIED.);
#56975=B_SPLINE_SURFACE_WITH_KNOTS('',2,1,((#85068,#85069),(#85070,#85071),
(#85072,#85073)),.UNSPECIFIED.,.F.,.F.,.F.,(3,3),(2,2),(0.,1.),(0.,0.0149999999999997),
 .UNSPECIFIED.);
#56976=B_SPLINE_SURFACE_WITH_KNOTS('',2,1,((#85083,#85084),(#85085,#85086),
(#85087,#85088)),.UNSPECIFIED.,.F.,.F.,.F.,(3,3),(2,2),(0.,1.),(0.,0.0149999999999997),
 .UNSPECIFIED.);
#56977=B_SPLINE_SURFACE_WITH_KNOTS('',2,1,((#85098,#85099),(#85100,#85101),
(#85102,#85103)),.UNSPECIFIED.,.F.,.F.,.F.,(3,3),(2,2),(0.,1.),(0.,0.0149999999999997),
 .UNSPECIFIED.);
#56978=B_SPLINE_SURFACE_WITH_KNOTS('',2,1,((#85113,#85114),(#85115,#85116),
(#85117,#85118)),.UNSPECIFIED.,.F.,.F.,.F.,(3,3),(2,2),(0.,1.),(0.,0.0149999999999997),
 .UNSPECIFIED.);
#56979=B_SPLINE_SURFACE_WITH_KNOTS('',2,1,((#85128,#85129),(#85130,#85131),
(#85132,#85133)),.UNSPECIFIED.,.F.,.F.,.F.,(3,3),(2,2),(0.,1.),(0.,0.0149999999999997),
 .UNSPECIFIED.);
#56980=B_SPLINE_SURFACE_WITH_KNOTS('',2,1,((#85143,#85144),(#85145,#85146),
(#85147,#85148)),.UNSPECIFIED.,.F.,.F.,.F.,(3,3),(2,2),(0.,1.),(0.,0.0149999999999997),
 .UNSPECIFIED.);
#56981=B_SPLINE_SURFACE_WITH_KNOTS('',2,1,((#85158,#85159),(#85160,#85161),
(#85162,#85163)),.UNSPECIFIED.,.F.,.F.,.F.,(3,3),(2,2),(0.,1.),(0.,0.0149999999999997),
 .UNSPECIFIED.);
#56982=B_SPLINE_SURFACE_WITH_KNOTS('',2,1,((#85179,#85180),(#85181,#85182),
(#85183,#85184)),.UNSPECIFIED.,.F.,.F.,.F.,(3,3),(2,2),(0.,1.),(0.,0.0149999999999997),
 .UNSPECIFIED.);
#56983=B_SPLINE_SURFACE_WITH_KNOTS('',2,1,((#85194,#85195),(#85196,#85197),
(#85198,#85199)),.UNSPECIFIED.,.F.,.F.,.F.,(3,3),(2,2),(0.,1.),(0.,0.0149999999999997),
 .UNSPECIFIED.);
#56984=B_SPLINE_SURFACE_WITH_KNOTS('',2,1,((#85212,#85213),(#85214,#85215),
(#85216,#85217)),.UNSPECIFIED.,.F.,.F.,.F.,(3,3),(2,2),(0.,1.),(0.,0.0149999999999997),
 .UNSPECIFIED.);
#56985=B_SPLINE_SURFACE_WITH_KNOTS('',2,1,((#85227,#85228),(#85229,#85230),
(#85231,#85232)),.UNSPECIFIED.,.F.,.F.,.F.,(3,3),(2,2),(0.,1.),(0.,0.0149999999999997),
 .UNSPECIFIED.);
#56986=B_SPLINE_SURFACE_WITH_KNOTS('',2,1,((#85242,#85243),(#85244,#85245),
(#85246,#85247)),.UNSPECIFIED.,.F.,.F.,.F.,(3,3),(2,2),(0.,1.),(0.,0.0149999999999997),
 .UNSPECIFIED.);
#56987=B_SPLINE_SURFACE_WITH_KNOTS('',2,1,((#85257,#85258),(#85259,#85260),
(#85261,#85262)),.UNSPECIFIED.,.F.,.F.,.F.,(3,3),(2,2),(0.,1.),(0.,0.0149999999999997),
 .UNSPECIFIED.);
#56988=B_SPLINE_SURFACE_WITH_KNOTS('',2,1,((#85272,#85273),(#85274,#85275),
(#85276,#85277)),.UNSPECIFIED.,.F.,.F.,.F.,(3,3),(2,2),(0.,1.),(0.,0.0149999999999997),
 .UNSPECIFIED.);
#56989=B_SPLINE_SURFACE_WITH_KNOTS('',2,1,((#85287,#85288),(#85289,#85290),
(#85291,#85292)),.UNSPECIFIED.,.F.,.F.,.F.,(3,3),(2,2),(0.,1.),(0.,0.0149999999999997),
 .UNSPECIFIED.);
#56990=B_SPLINE_SURFACE_WITH_KNOTS('',2,1,((#85302,#85303),(#85304,#85305),
(#85306,#85307)),.UNSPECIFIED.,.F.,.F.,.F.,(3,3),(2,2),(0.,1.),(0.,0.0149999999999997),
 .UNSPECIFIED.);
#56991=B_SPLINE_SURFACE_WITH_KNOTS('',2,1,((#85314,#85315),(#85316,#85317),
(#85318,#85319)),.UNSPECIFIED.,.F.,.F.,.F.,(3,3),(2,2),(0.,1.),(0.,0.0149999999999997),
 .UNSPECIFIED.);
#56992=B_SPLINE_SURFACE_WITH_KNOTS('',2,1,((#85332,#85333),(#85334,#85335),
(#85336,#85337)),.UNSPECIFIED.,.F.,.F.,.F.,(3,3),(2,2),(0.,1.),(0.,0.0149999999999997),
 .UNSPECIFIED.);
#56993=B_SPLINE_SURFACE_WITH_KNOTS('',2,1,((#85347,#85348),(#85349,#85350),
(#85351,#85352)),.UNSPECIFIED.,.F.,.F.,.F.,(3,3),(2,2),(0.,1.),(0.,0.0149999999999997),
 .UNSPECIFIED.);
#56994=B_SPLINE_SURFACE_WITH_KNOTS('',2,1,((#85362,#85363),(#85364,#85365),
(#85366,#85367)),.UNSPECIFIED.,.F.,.F.,.F.,(3,3),(2,2),(0.,1.),(0.,0.0149999999999997),
 .UNSPECIFIED.);
#56995=B_SPLINE_SURFACE_WITH_KNOTS('',2,1,((#85377,#85378),(#85379,#85380),
(#85381,#85382)),.UNSPECIFIED.,.F.,.F.,.F.,(3,3),(2,2),(0.,1.),(0.,0.0149999999999997),
 .UNSPECIFIED.);
#56996=B_SPLINE_SURFACE_WITH_KNOTS('',2,1,((#85392,#85393),(#85394,#85395),
(#85396,#85397)),.UNSPECIFIED.,.F.,.F.,.F.,(3,3),(2,2),(0.,1.),(0.,0.0149999999999997),
 .UNSPECIFIED.);
#56997=B_SPLINE_SURFACE_WITH_KNOTS('',2,1,((#85407,#85408),(#85409,#85410),
(#85411,#85412)),.UNSPECIFIED.,.F.,.F.,.F.,(3,3),(2,2),(0.,1.),(0.,0.0149999999999997),
 .UNSPECIFIED.);
#56998=B_SPLINE_SURFACE_WITH_KNOTS('',2,1,((#85422,#85423),(#85424,#85425),
(#85426,#85427)),.UNSPECIFIED.,.F.,.F.,.F.,(3,3),(2,2),(0.,1.),(0.,0.0149999999999997),
 .UNSPECIFIED.);
#56999=B_SPLINE_SURFACE_WITH_KNOTS('',2,1,((#85437,#85438),(#85439,#85440),
(#85441,#85442)),.UNSPECIFIED.,.F.,.F.,.F.,(3,3),(2,2),(0.,1.),(0.,0.0149999999999997),
 .UNSPECIFIED.);
#57000=B_SPLINE_SURFACE_WITH_KNOTS('',2,1,((#85452,#85453),(#85454,#85455),
(#85456,#85457)),.UNSPECIFIED.,.F.,.F.,.F.,(3,3),(2,2),(0.,1.),(0.,0.0149999999999997),
 .UNSPECIFIED.);
#57001=B_SPLINE_SURFACE_WITH_KNOTS('',2,1,((#85467,#85468),(#85469,#85470),
(#85471,#85472)),.UNSPECIFIED.,.F.,.F.,.F.,(3,3),(2,2),(0.,1.),(0.,0.0149999999999997),
 .UNSPECIFIED.);
#57002=B_SPLINE_SURFACE_WITH_KNOTS('',2,1,((#85482,#85483),(#85484,#85485),
(#85486,#85487)),.UNSPECIFIED.,.F.,.F.,.F.,(3,3),(2,2),(0.,1.),(0.,0.0149999999999997),
 .UNSPECIFIED.);
#57003=B_SPLINE_SURFACE_WITH_KNOTS('',2,1,((#85495,#85496),(#85497,#85498),
(#85499,#85500)),.UNSPECIFIED.,.F.,.F.,.F.,(3,3),(2,2),(0.,1.),(0.,0.0149999999999997),
 .UNSPECIFIED.);
#57004=B_SPLINE_SURFACE_WITH_KNOTS('',2,1,((#85513,#85514),(#85515,#85516),
(#85517,#85518)),.UNSPECIFIED.,.F.,.F.,.F.,(3,3),(2,2),(0.,1.),(0.,0.0149999999999997),
 .UNSPECIFIED.);
#57005=B_SPLINE_SURFACE_WITH_KNOTS('',2,1,((#85528,#85529),(#85530,#85531),
(#85532,#85533)),.UNSPECIFIED.,.F.,.F.,.F.,(3,3),(2,2),(0.,1.),(0.,0.0149999999999997),
 .UNSPECIFIED.);
#57006=B_SPLINE_SURFACE_WITH_KNOTS('',2,1,((#85549,#85550),(#85551,#85552),
(#85553,#85554)),.UNSPECIFIED.,.F.,.F.,.F.,(3,3),(2,2),(0.,1.),(0.,0.0149999999999997),
 .UNSPECIFIED.);
#57007=B_SPLINE_SURFACE_WITH_KNOTS('',2,1,((#85564,#85565),(#85566,#85567),
(#85568,#85569)),.UNSPECIFIED.,.F.,.F.,.F.,(3,3),(2,2),(0.,1.),(0.,0.0149999999999997),
 .UNSPECIFIED.);
#57008=B_SPLINE_SURFACE_WITH_KNOTS('',2,1,((#85579,#85580),(#85581,#85582),
(#85583,#85584)),.UNSPECIFIED.,.F.,.F.,.F.,(3,3),(2,2),(0.,1.),(0.,0.0149999999999997),
 .UNSPECIFIED.);
#57009=B_SPLINE_SURFACE_WITH_KNOTS('',2,1,((#85617,#85618),(#85619,#85620),
(#85621,#85622)),.UNSPECIFIED.,.F.,.F.,.F.,(3,3),(2,2),(0.,1.),(0.,0.0149999999999997),
 .UNSPECIFIED.);
#57010=B_SPLINE_SURFACE_WITH_KNOTS('',2,1,((#85635,#85636),(#85637,#85638),
(#85639,#85640)),.UNSPECIFIED.,.F.,.F.,.F.,(3,3),(2,2),(0.,1.),(0.,0.0149999999999997),
 .UNSPECIFIED.);
#57011=B_SPLINE_SURFACE_WITH_KNOTS('',2,1,((#85650,#85651),(#85652,#85653),
(#85654,#85655)),.UNSPECIFIED.,.F.,.F.,.F.,(3,3),(2,2),(0.,1.),(0.,0.0149999999999997),
 .UNSPECIFIED.);
#57012=B_SPLINE_SURFACE_WITH_KNOTS('',2,1,((#85665,#85666),(#85667,#85668),
(#85669,#85670)),.UNSPECIFIED.,.F.,.F.,.F.,(3,3),(2,2),(0.,1.),(0.,0.0149999999999997),
 .UNSPECIFIED.);
#57013=B_SPLINE_SURFACE_WITH_KNOTS('',2,1,((#85680,#85681),(#85682,#85683),
(#85684,#85685)),.UNSPECIFIED.,.F.,.F.,.F.,(3,3),(2,2),(0.,1.),(0.,0.0149999999999997),
 .UNSPECIFIED.);
#57014=B_SPLINE_SURFACE_WITH_KNOTS('',2,1,((#85695,#85696),(#85697,#85698),
(#85699,#85700)),.UNSPECIFIED.,.F.,.F.,.F.,(3,3),(2,2),(0.,1.),(0.,0.0149999999999997),
 .UNSPECIFIED.);
#57015=B_SPLINE_SURFACE_WITH_KNOTS('',2,1,((#85710,#85711),(#85712,#85713),
(#85714,#85715)),.UNSPECIFIED.,.F.,.F.,.F.,(3,3),(2,2),(0.,1.),(0.,0.0149999999999997),
 .UNSPECIFIED.);
#57016=B_SPLINE_SURFACE_WITH_KNOTS('',2,1,((#85725,#85726),(#85727,#85728),
(#85729,#85730)),.UNSPECIFIED.,.F.,.F.,.F.,(3,3),(2,2),(0.,1.),(0.,0.0149999999999997),
 .UNSPECIFIED.);
#57017=B_SPLINE_SURFACE_WITH_KNOTS('',2,1,((#85737,#85738),(#85739,#85740),
(#85741,#85742)),.UNSPECIFIED.,.F.,.F.,.F.,(3,3),(2,2),(0.,1.),(0.,0.0149999999999997),
 .UNSPECIFIED.);
#57018=B_SPLINE_SURFACE_WITH_KNOTS('',2,1,((#85755,#85756),(#85757,#85758),
(#85759,#85760)),.UNSPECIFIED.,.F.,.F.,.F.,(3,3),(2,2),(0.,1.),(0.,0.0149999999999997),
 .UNSPECIFIED.);
#57019=B_SPLINE_SURFACE_WITH_KNOTS('',2,1,((#85770,#85771),(#85772,#85773),
(#85774,#85775)),.UNSPECIFIED.,.F.,.F.,.F.,(3,3),(2,2),(0.,1.),(0.,0.0149999999999997),
 .UNSPECIFIED.);
#57020=B_SPLINE_SURFACE_WITH_KNOTS('',2,1,((#85785,#85786),(#85787,#85788),
(#85789,#85790)),.UNSPECIFIED.,.F.,.F.,.F.,(3,3),(2,2),(0.,1.),(0.,0.0149999999999997),
 .UNSPECIFIED.);
#57021=B_SPLINE_SURFACE_WITH_KNOTS('',2,1,((#85800,#85801),(#85802,#85803),
(#85804,#85805)),.UNSPECIFIED.,.F.,.F.,.F.,(3,3),(2,2),(0.,1.),(0.,0.0149999999999997),
 .UNSPECIFIED.);
#57022=B_SPLINE_SURFACE_WITH_KNOTS('',2,1,((#85815,#85816),(#85817,#85818),
(#85819,#85820)),.UNSPECIFIED.,.F.,.F.,.F.,(3,3),(2,2),(0.,1.),(0.,0.0149999999999997),
 .UNSPECIFIED.);
#57023=B_SPLINE_SURFACE_WITH_KNOTS('',2,1,((#85830,#85831),(#85832,#85833),
(#85834,#85835)),.UNSPECIFIED.,.F.,.F.,.F.,(3,3),(2,2),(0.,1.),(0.,0.0149999999999997),
 .UNSPECIFIED.);
#57024=B_SPLINE_SURFACE_WITH_KNOTS('',2,1,((#85845,#85846),(#85847,#85848),
(#85849,#85850)),.UNSPECIFIED.,.F.,.F.,.F.,(3,3),(2,2),(0.,1.),(0.,0.0149999999999997),
 .UNSPECIFIED.);
#57025=B_SPLINE_SURFACE_WITH_KNOTS('',2,1,((#85860,#85861),(#85862,#85863),
(#85864,#85865)),.UNSPECIFIED.,.F.,.F.,.F.,(3,3),(2,2),(0.,1.),(0.,0.0149999999999997),
 .UNSPECIFIED.);
#57026=B_SPLINE_SURFACE_WITH_KNOTS('',2,1,((#85875,#85876),(#85877,#85878),
(#85879,#85880)),.UNSPECIFIED.,.F.,.F.,.F.,(3,3),(2,2),(0.,1.),(0.,0.0149999999999997),
 .UNSPECIFIED.);
#57027=B_SPLINE_SURFACE_WITH_KNOTS('',2,1,((#85890,#85891),(#85892,#85893),
(#85894,#85895)),.UNSPECIFIED.,.F.,.F.,.F.,(3,3),(2,2),(0.,1.),(0.,0.0149999999999997),
 .UNSPECIFIED.);
#57028=B_SPLINE_SURFACE_WITH_KNOTS('',2,1,((#85905,#85906),(#85907,#85908),
(#85909,#85910)),.UNSPECIFIED.,.F.,.F.,.F.,(3,3),(2,2),(0.,1.),(0.,0.0149999999999997),
 .UNSPECIFIED.);
#57029=B_SPLINE_SURFACE_WITH_KNOTS('',2,1,((#85918,#85919),(#85920,#85921),
(#85922,#85923)),.UNSPECIFIED.,.F.,.F.,.F.,(3,3),(2,2),(0.,1.),(0.,0.0149999999999997),
 .UNSPECIFIED.);
#57030=B_SPLINE_SURFACE_WITH_KNOTS('',2,1,((#85936,#85937),(#85938,#85939),
(#85940,#85941)),.UNSPECIFIED.,.F.,.F.,.F.,(3,3),(2,2),(0.,1.),(0.,0.0149999999999997),
 .UNSPECIFIED.);
#57031=B_SPLINE_SURFACE_WITH_KNOTS('',2,1,((#85951,#85952),(#85953,#85954),
(#85955,#85956)),.UNSPECIFIED.,.F.,.F.,.F.,(3,3),(2,2),(0.,1.),(0.,0.0149999999999997),
 .UNSPECIFIED.);
#57032=B_SPLINE_SURFACE_WITH_KNOTS('',2,1,((#85966,#85967),(#85968,#85969),
(#85970,#85971)),.UNSPECIFIED.,.F.,.F.,.F.,(3,3),(2,2),(0.,1.),(0.,0.0149999999999997),
 .UNSPECIFIED.);
#57033=B_SPLINE_SURFACE_WITH_KNOTS('',2,1,((#85981,#85982),(#85983,#85984),
(#85985,#85986)),.UNSPECIFIED.,.F.,.F.,.F.,(3,3),(2,2),(0.,1.),(0.,0.0149999999999997),
 .UNSPECIFIED.);
#57034=B_SPLINE_SURFACE_WITH_KNOTS('',2,1,((#85996,#85997),(#85998,#85999),
(#86000,#86001)),.UNSPECIFIED.,.F.,.F.,.F.,(3,3),(2,2),(0.,1.),(0.,0.0149999999999997),
 .UNSPECIFIED.);
#57035=B_SPLINE_SURFACE_WITH_KNOTS('',2,1,((#86011,#86012),(#86013,#86014),
(#86015,#86016)),.UNSPECIFIED.,.F.,.F.,.F.,(3,3),(2,2),(0.,1.),(0.,0.0149999999999997),
 .UNSPECIFIED.);
#57036=B_SPLINE_SURFACE_WITH_KNOTS('',2,1,((#86026,#86027),(#86028,#86029),
(#86030,#86031)),.UNSPECIFIED.,.F.,.F.,.F.,(3,3),(2,2),(0.,1.),(0.,0.0149999999999997),
 .UNSPECIFIED.);
#57037=B_SPLINE_SURFACE_WITH_KNOTS('',2,1,((#86038,#86039),(#86040,#86041),
(#86042,#86043)),.UNSPECIFIED.,.F.,.F.,.F.,(3,3),(2,2),(0.,1.),(0.,0.0149999999999997),
 .UNSPECIFIED.);
#57038=B_SPLINE_SURFACE_WITH_KNOTS('',2,1,((#86056,#86057),(#86058,#86059),
(#86060,#86061)),.UNSPECIFIED.,.F.,.F.,.F.,(3,3),(2,2),(0.,1.),(0.,0.0149999999999997),
 .UNSPECIFIED.);
#57039=B_SPLINE_SURFACE_WITH_KNOTS('',2,1,((#86071,#86072),(#86073,#86074),
(#86075,#86076)),.UNSPECIFIED.,.F.,.F.,.F.,(3,3),(2,2),(0.,1.),(0.,0.0149999999999997),
 .UNSPECIFIED.);
#57040=B_SPLINE_SURFACE_WITH_KNOTS('',2,1,((#86086,#86087),(#86088,#86089),
(#86090,#86091)),.UNSPECIFIED.,.F.,.F.,.F.,(3,3),(2,2),(0.,1.),(0.,0.0149999999999997),
 .UNSPECIFIED.);
#57041=B_SPLINE_SURFACE_WITH_KNOTS('',2,1,((#86101,#86102),(#86103,#86104),
(#86105,#86106)),.UNSPECIFIED.,.F.,.F.,.F.,(3,3),(2,2),(0.,1.),(0.,0.0149999999999997),
 .UNSPECIFIED.);
#57042=B_SPLINE_SURFACE_WITH_KNOTS('',2,1,((#86116,#86117),(#86118,#86119),
(#86120,#86121)),.UNSPECIFIED.,.F.,.F.,.F.,(3,3),(2,2),(0.,1.),(0.,0.0149999999999997),
 .UNSPECIFIED.);
#57043=B_SPLINE_SURFACE_WITH_KNOTS('',2,1,((#86131,#86132),(#86133,#86134),
(#86135,#86136)),.UNSPECIFIED.,.F.,.F.,.F.,(3,3),(2,2),(0.,1.),(0.,0.0149999999999997),
 .UNSPECIFIED.);
#57044=B_SPLINE_SURFACE_WITH_KNOTS('',2,1,((#86146,#86147),(#86148,#86149),
(#86150,#86151)),.UNSPECIFIED.,.F.,.F.,.F.,(3,3),(2,2),(0.,1.),(0.,0.0149999999999997),
 .UNSPECIFIED.);
#57045=B_SPLINE_SURFACE_WITH_KNOTS('',2,1,((#86161,#86162),(#86163,#86164),
(#86165,#86166)),.UNSPECIFIED.,.F.,.F.,.F.,(3,3),(2,2),(0.,1.),(0.,0.0149999999999997),
 .UNSPECIFIED.);
#57046=B_SPLINE_SURFACE_WITH_KNOTS('',2,1,((#86173,#86174),(#86175,#86176),
(#86177,#86178)),.UNSPECIFIED.,.F.,.F.,.F.,(3,3),(2,2),(0.,1.),(0.,0.0149999999999997),
 .UNSPECIFIED.);
#57047=B_SPLINE_SURFACE_WITH_KNOTS('',2,1,((#86191,#86192),(#86193,#86194),
(#86195,#86196)),.UNSPECIFIED.,.F.,.F.,.F.,(3,3),(2,2),(0.,1.),(0.,0.0149999999999997),
 .UNSPECIFIED.);
#57048=B_SPLINE_SURFACE_WITH_KNOTS('',2,1,((#86206,#86207),(#86208,#86209),
(#86210,#86211)),.UNSPECIFIED.,.F.,.F.,.F.,(3,3),(2,2),(0.,1.),(0.,0.0149999999999997),
 .UNSPECIFIED.);
#57049=B_SPLINE_SURFACE_WITH_KNOTS('',2,1,((#86221,#86222),(#86223,#86224),
(#86225,#86226)),.UNSPECIFIED.,.F.,.F.,.F.,(3,3),(2,2),(0.,1.),(0.,0.0149999999999997),
 .UNSPECIFIED.);
#57050=B_SPLINE_SURFACE_WITH_KNOTS('',2,1,((#86236,#86237),(#86238,#86239),
(#86240,#86241)),.UNSPECIFIED.,.F.,.F.,.F.,(3,3),(2,2),(0.,1.),(0.,0.0149999999999997),
 .UNSPECIFIED.);
#57051=B_SPLINE_SURFACE_WITH_KNOTS('',2,1,((#86251,#86252),(#86253,#86254),
(#86255,#86256)),.UNSPECIFIED.,.F.,.F.,.F.,(3,3),(2,2),(0.,1.),(0.,0.0149999999999997),
 .UNSPECIFIED.);
#57052=B_SPLINE_SURFACE_WITH_KNOTS('',2,1,((#86266,#86267),(#86268,#86269),
(#86270,#86271)),.UNSPECIFIED.,.F.,.F.,.F.,(3,3),(2,2),(0.,1.),(0.,0.0149999999999997),
 .UNSPECIFIED.);
#57053=B_SPLINE_SURFACE_WITH_KNOTS('',2,1,((#86281,#86282),(#86283,#86284),
(#86285,#86286)),.UNSPECIFIED.,.F.,.F.,.F.,(3,3),(2,2),(0.,1.),(0.,0.0149999999999997),
 .UNSPECIFIED.);
#57054=B_SPLINE_SURFACE_WITH_KNOTS('',2,1,((#86296,#86297),(#86298,#86299),
(#86300,#86301)),.UNSPECIFIED.,.F.,.F.,.F.,(3,3),(2,2),(0.,1.),(0.,0.0149999999999997),
 .UNSPECIFIED.);
#57055=B_SPLINE_SURFACE_WITH_KNOTS('',2,1,((#86311,#86312),(#86313,#86314),
(#86315,#86316)),.UNSPECIFIED.,.F.,.F.,.F.,(3,3),(2,2),(0.,1.),(0.,0.0149999999999997),
 .UNSPECIFIED.);
#57056=B_SPLINE_SURFACE_WITH_KNOTS('',2,1,((#86326,#86327),(#86328,#86329),
(#86330,#86331)),.UNSPECIFIED.,.F.,.F.,.F.,(3,3),(2,2),(0.,1.),(0.,0.0149999999999997),
 .UNSPECIFIED.);
#57057=B_SPLINE_SURFACE_WITH_KNOTS('',2,1,((#86341,#86342),(#86343,#86344),
(#86345,#86346)),.UNSPECIFIED.,.F.,.F.,.F.,(3,3),(2,2),(0.,1.),(0.,0.0149999999999997),
 .UNSPECIFIED.);
#57058=B_SPLINE_SURFACE_WITH_KNOTS('',2,1,((#86356,#86357),(#86358,#86359),
(#86360,#86361)),.UNSPECIFIED.,.F.,.F.,.F.,(3,3),(2,2),(0.,1.),(0.,0.0149999999999997),
 .UNSPECIFIED.);
#57059=B_SPLINE_SURFACE_WITH_KNOTS('',2,1,((#86371,#86372),(#86373,#86374),
(#86375,#86376)),.UNSPECIFIED.,.F.,.F.,.F.,(3,3),(2,2),(0.,1.),(0.,0.0149999999999997),
 .UNSPECIFIED.);
#57060=B_SPLINE_SURFACE_WITH_KNOTS('',2,1,((#86386,#86387),(#86388,#86389),
(#86390,#86391)),.UNSPECIFIED.,.F.,.F.,.F.,(3,3),(2,2),(0.,1.),(0.,0.0149999999999997),
 .UNSPECIFIED.);
#57061=B_SPLINE_SURFACE_WITH_KNOTS('',2,1,((#86401,#86402),(#86403,#86404),
(#86405,#86406)),.UNSPECIFIED.,.F.,.F.,.F.,(3,3),(2,2),(0.,1.),(0.,0.0149999999999997),
 .UNSPECIFIED.);
#57062=B_SPLINE_SURFACE_WITH_KNOTS('',2,1,((#86417,#86418),(#86419,#86420),
(#86421,#86422)),.UNSPECIFIED.,.F.,.F.,.F.,(3,3),(2,2),(0.,1.),(0.,0.0149999999999997),
 .UNSPECIFIED.);
#57063=B_SPLINE_SURFACE_WITH_KNOTS('',2,1,((#86435,#86436),(#86437,#86438),
(#86439,#86440)),.UNSPECIFIED.,.F.,.F.,.F.,(3,3),(2,2),(0.,1.),(0.,0.0149999999999997),
 .UNSPECIFIED.);
#57064=B_SPLINE_SURFACE_WITH_KNOTS('',2,1,((#86450,#86451),(#86452,#86453),
(#86454,#86455)),.UNSPECIFIED.,.F.,.F.,.F.,(3,3),(2,2),(0.,1.),(0.,0.0149999999999997),
 .UNSPECIFIED.);
#57065=B_SPLINE_SURFACE_WITH_KNOTS('',2,1,((#86465,#86466),(#86467,#86468),
(#86469,#86470)),.UNSPECIFIED.,.F.,.F.,.F.,(3,3),(2,2),(0.,1.),(0.,0.0149999999999997),
 .UNSPECIFIED.);
#57066=B_SPLINE_SURFACE_WITH_KNOTS('',2,1,((#86480,#86481),(#86482,#86483),
(#86484,#86485)),.UNSPECIFIED.,.F.,.F.,.F.,(3,3),(2,2),(0.,1.),(0.,0.0149999999999997),
 .UNSPECIFIED.);
#57067=B_SPLINE_SURFACE_WITH_KNOTS('',2,1,((#86495,#86496),(#86497,#86498),
(#86499,#86500)),.UNSPECIFIED.,.F.,.F.,.F.,(3,3),(2,2),(0.,1.),(0.,0.0149999999999997),
 .UNSPECIFIED.);
#57068=B_SPLINE_SURFACE_WITH_KNOTS('',2,1,((#86510,#86511),(#86512,#86513),
(#86514,#86515)),.UNSPECIFIED.,.F.,.F.,.F.,(3,3),(2,2),(0.,1.),(0.,0.0149999999999997),
 .UNSPECIFIED.);
#57069=B_SPLINE_SURFACE_WITH_KNOTS('',2,1,((#86525,#86526),(#86527,#86528),
(#86529,#86530)),.UNSPECIFIED.,.F.,.F.,.F.,(3,3),(2,2),(0.,1.),(0.,0.0149999999999997),
 .UNSPECIFIED.);
#57070=B_SPLINE_SURFACE_WITH_KNOTS('',2,1,((#86537,#86538),(#86539,#86540),
(#86541,#86542)),.UNSPECIFIED.,.F.,.F.,.F.,(3,3),(2,2),(0.,1.),(0.,0.0149999999999997),
 .UNSPECIFIED.);
#57071=B_SPLINE_SURFACE_WITH_KNOTS('',2,1,((#86555,#86556),(#86557,#86558),
(#86559,#86560)),.UNSPECIFIED.,.F.,.F.,.F.,(3,3),(2,2),(0.,1.),(0.,0.0149999999999997),
 .UNSPECIFIED.);
#57072=B_SPLINE_SURFACE_WITH_KNOTS('',2,1,((#86570,#86571),(#86572,#86573),
(#86574,#86575)),.UNSPECIFIED.,.F.,.F.,.F.,(3,3),(2,2),(0.,1.),(0.,0.0149999999999997),
 .UNSPECIFIED.);
#57073=B_SPLINE_SURFACE_WITH_KNOTS('',2,1,((#86585,#86586),(#86587,#86588),
(#86589,#86590)),.UNSPECIFIED.,.F.,.F.,.F.,(3,3),(2,2),(0.,1.),(0.,0.0149999999999997),
 .UNSPECIFIED.);
#57074=B_SPLINE_SURFACE_WITH_KNOTS('',2,1,((#86600,#86601),(#86602,#86603),
(#86604,#86605)),.UNSPECIFIED.,.F.,.F.,.F.,(3,3),(2,2),(0.,1.),(0.,0.0149999999999997),
 .UNSPECIFIED.);
#57075=B_SPLINE_SURFACE_WITH_KNOTS('',2,1,((#86615,#86616),(#86617,#86618),
(#86619,#86620)),.UNSPECIFIED.,.F.,.F.,.F.,(3,3),(2,2),(0.,1.),(0.,0.0149999999999997),
 .UNSPECIFIED.);
#57076=B_SPLINE_SURFACE_WITH_KNOTS('',2,1,((#86630,#86631),(#86632,#86633),
(#86634,#86635)),.UNSPECIFIED.,.F.,.F.,.F.,(3,3),(2,2),(0.,1.),(0.,0.0149999999999997),
 .UNSPECIFIED.);
#57077=B_SPLINE_SURFACE_WITH_KNOTS('',2,1,((#86645,#86646),(#86647,#86648),
(#86649,#86650)),.UNSPECIFIED.,.F.,.F.,.F.,(3,3),(2,2),(0.,1.),(0.,0.0149999999999997),
 .UNSPECIFIED.);
#57078=B_SPLINE_SURFACE_WITH_KNOTS('',2,1,((#86660,#86661),(#86662,#86663),
(#86664,#86665)),.UNSPECIFIED.,.F.,.F.,.F.,(3,3),(2,2),(0.,1.),(0.,0.0149999999999997),
 .UNSPECIFIED.);
#57079=B_SPLINE_SURFACE_WITH_KNOTS('',2,1,((#86675,#86676),(#86677,#86678),
(#86679,#86680)),.UNSPECIFIED.,.F.,.F.,.F.,(3,3),(2,2),(0.,1.),(0.,0.0149999999999997),
 .UNSPECIFIED.);
#57080=B_SPLINE_SURFACE_WITH_KNOTS('',2,1,((#86690,#86691),(#86692,#86693),
(#86694,#86695)),.UNSPECIFIED.,.F.,.F.,.F.,(3,3),(2,2),(0.,1.),(0.,0.0149999999999997),
 .UNSPECIFIED.);
#57081=B_SPLINE_SURFACE_WITH_KNOTS('',2,1,((#86705,#86706),(#86707,#86708),
(#86709,#86710)),.UNSPECIFIED.,.F.,.F.,.F.,(3,3),(2,2),(0.,1.),(0.,0.0149999999999997),
 .UNSPECIFIED.);
#57082=B_SPLINE_SURFACE_WITH_KNOTS('',2,1,((#86718,#86719),(#86720,#86721),
(#86722,#86723)),.UNSPECIFIED.,.F.,.F.,.F.,(3,3),(2,2),(0.,1.),(0.,0.0149999999999997),
 .UNSPECIFIED.);
#57083=B_SPLINE_SURFACE_WITH_KNOTS('',2,1,((#86736,#86737),(#86738,#86739),
(#86740,#86741)),.UNSPECIFIED.,.F.,.F.,.F.,(3,3),(2,2),(0.,1.),(0.,0.0149999999999997),
 .UNSPECIFIED.);
#57084=B_SPLINE_SURFACE_WITH_KNOTS('',2,1,((#86751,#86752),(#86753,#86754),
(#86755,#86756)),.UNSPECIFIED.,.F.,.F.,.F.,(3,3),(2,2),(0.,1.),(0.,0.0149999999999997),
 .UNSPECIFIED.);
#57085=B_SPLINE_SURFACE_WITH_KNOTS('',2,1,((#86766,#86767),(#86768,#86769),
(#86770,#86771)),.UNSPECIFIED.,.F.,.F.,.F.,(3,3),(2,2),(0.,1.),(0.,0.0149999999999997),
 .UNSPECIFIED.);
#57086=B_SPLINE_SURFACE_WITH_KNOTS('',2,1,((#86781,#86782),(#86783,#86784),
(#86785,#86786)),.UNSPECIFIED.,.F.,.F.,.F.,(3,3),(2,2),(0.,1.),(0.,0.0149999999999997),
 .UNSPECIFIED.);
#57087=B_SPLINE_SURFACE_WITH_KNOTS('',2,1,((#86796,#86797),(#86798,#86799),
(#86800,#86801)),.UNSPECIFIED.,.F.,.F.,.F.,(3,3),(2,2),(0.,1.),(0.,0.0149999999999997),
 .UNSPECIFIED.);
#57088=B_SPLINE_SURFACE_WITH_KNOTS('',2,1,((#86811,#86812),(#86813,#86814),
(#86815,#86816)),.UNSPECIFIED.,.F.,.F.,.F.,(3,3),(2,2),(0.,1.),(0.,0.0149999999999997),
 .UNSPECIFIED.);
#57089=B_SPLINE_SURFACE_WITH_KNOTS('',2,1,((#86826,#86827),(#86828,#86829),
(#86830,#86831)),.UNSPECIFIED.,.F.,.F.,.F.,(3,3),(2,2),(0.,1.),(0.,0.0149999999999997),
 .UNSPECIFIED.);
#57090=B_SPLINE_SURFACE_WITH_KNOTS('',2,1,((#86838,#86839),(#86840,#86841),
(#86842,#86843)),.UNSPECIFIED.,.F.,.F.,.F.,(3,3),(2,2),(0.,1.),(0.,0.0149999999999997),
 .UNSPECIFIED.);
#57091=B_SPLINE_SURFACE_WITH_KNOTS('',2,1,((#86856,#86857),(#86858,#86859),
(#86860,#86861)),.UNSPECIFIED.,.F.,.F.,.F.,(3,3),(2,2),(0.,1.),(0.,0.0149999999999997),
 .UNSPECIFIED.);
#57092=B_SPLINE_SURFACE_WITH_KNOTS('',2,1,((#86871,#86872),(#86873,#86874),
(#86875,#86876)),.UNSPECIFIED.,.F.,.F.,.F.,(3,3),(2,2),(0.,1.),(0.,0.0149999999999997),
 .UNSPECIFIED.);
#57093=B_SPLINE_SURFACE_WITH_KNOTS('',2,1,((#86886,#86887),(#86888,#86889),
(#86890,#86891)),.UNSPECIFIED.,.F.,.F.,.F.,(3,3),(2,2),(0.,1.),(0.,0.0149999999999997),
 .UNSPECIFIED.);
#57094=B_SPLINE_SURFACE_WITH_KNOTS('',2,1,((#86901,#86902),(#86903,#86904),
(#86905,#86906)),.UNSPECIFIED.,.F.,.F.,.F.,(3,3),(2,2),(0.,1.),(0.,0.0149999999999997),
 .UNSPECIFIED.);
#57095=B_SPLINE_SURFACE_WITH_KNOTS('',2,1,((#86916,#86917),(#86918,#86919),
(#86920,#86921)),.UNSPECIFIED.,.F.,.F.,.F.,(3,3),(2,2),(0.,1.),(0.,0.0149999999999997),
 .UNSPECIFIED.);
#57096=B_SPLINE_SURFACE_WITH_KNOTS('',2,1,((#86931,#86932),(#86933,#86934),
(#86935,#86936)),.UNSPECIFIED.,.F.,.F.,.F.,(3,3),(2,2),(0.,1.),(0.,0.0149999999999997),
 .UNSPECIFIED.);
#57097=B_SPLINE_SURFACE_WITH_KNOTS('',2,1,((#86946,#86947),(#86948,#86949),
(#86950,#86951)),.UNSPECIFIED.,.F.,.F.,.F.,(3,3),(2,2),(0.,1.),(0.,0.0149999999999997),
 .UNSPECIFIED.);
#57098=B_SPLINE_SURFACE_WITH_KNOTS('',2,1,((#86961,#86962),(#86963,#86964),
(#86965,#86966)),.UNSPECIFIED.,.F.,.F.,.F.,(3,3),(2,2),(0.,1.),(0.,0.0149999999999997),
 .UNSPECIFIED.);
#57099=B_SPLINE_SURFACE_WITH_KNOTS('',2,1,((#86976,#86977),(#86978,#86979),
(#86980,#86981)),.UNSPECIFIED.,.F.,.F.,.F.,(3,3),(2,2),(0.,1.),(0.,0.0149999999999997),
 .UNSPECIFIED.);
#57100=B_SPLINE_SURFACE_WITH_KNOTS('',2,1,((#86991,#86992),(#86993,#86994),
(#86995,#86996)),.UNSPECIFIED.,.F.,.F.,.F.,(3,3),(2,2),(0.,1.),(0.,0.0149999999999997),
 .UNSPECIFIED.);
#57101=B_SPLINE_SURFACE_WITH_KNOTS('',2,1,((#87006,#87007),(#87008,#87009),
(#87010,#87011)),.UNSPECIFIED.,.F.,.F.,.F.,(3,3),(2,2),(0.,1.),(0.,0.0149999999999997),
 .UNSPECIFIED.);
#57102=B_SPLINE_SURFACE_WITH_KNOTS('',2,1,((#87021,#87022),(#87023,#87024),
(#87025,#87026)),.UNSPECIFIED.,.F.,.F.,.F.,(3,3),(2,2),(0.,1.),(0.,0.0149999999999997),
 .UNSPECIFIED.);
#57103=B_SPLINE_SURFACE_WITH_KNOTS('',2,1,((#87036,#87037),(#87038,#87039),
(#87040,#87041)),.UNSPECIFIED.,.F.,.F.,.F.,(3,3),(2,2),(0.,1.),(0.,0.0149999999999997),
 .UNSPECIFIED.);
#57104=B_SPLINE_SURFACE_WITH_KNOTS('',2,1,((#87051,#87052),(#87053,#87054),
(#87055,#87056)),.UNSPECIFIED.,.F.,.F.,.F.,(3,3),(2,2),(0.,1.),(0.,0.0149999999999997),
 .UNSPECIFIED.);
#57105=B_SPLINE_SURFACE_WITH_KNOTS('',2,1,((#87066,#87067),(#87068,#87069),
(#87070,#87071)),.UNSPECIFIED.,.F.,.F.,.F.,(3,3),(2,2),(0.,1.),(0.,0.0149999999999997),
 .UNSPECIFIED.);
#57106=B_SPLINE_SURFACE_WITH_KNOTS('',2,1,((#87081,#87082),(#87083,#87084),
(#87085,#87086)),.UNSPECIFIED.,.F.,.F.,.F.,(3,3),(2,2),(0.,1.),(0.,0.0149999999999997),
 .UNSPECIFIED.);
#57107=B_SPLINE_SURFACE_WITH_KNOTS('',2,1,((#87096,#87097),(#87098,#87099),
(#87100,#87101)),.UNSPECIFIED.,.F.,.F.,.F.,(3,3),(2,2),(0.,1.),(0.,0.0149999999999997),
 .UNSPECIFIED.);
#57108=B_SPLINE_SURFACE_WITH_KNOTS('',2,1,((#87111,#87112),(#87113,#87114),
(#87115,#87116)),.UNSPECIFIED.,.F.,.F.,.F.,(3,3),(2,2),(0.,1.),(0.,0.0149999999999997),
 .UNSPECIFIED.);
#57109=B_SPLINE_SURFACE_WITH_KNOTS('',2,1,((#87126,#87127),(#87128,#87129),
(#87130,#87131)),.UNSPECIFIED.,.F.,.F.,.F.,(3,3),(2,2),(0.,1.),(0.,0.0149999999999997),
 .UNSPECIFIED.);
#57110=B_SPLINE_SURFACE_WITH_KNOTS('',2,1,((#87147,#87148),(#87149,#87150),
(#87151,#87152)),.UNSPECIFIED.,.F.,.F.,.F.,(3,3),(2,2),(0.,1.),(0.,0.0149999999999997),
 .UNSPECIFIED.);
#57125=ADVANCED_FACE('',(#4025),#56413,.F.);
#57126=ADVANCED_FACE('',(#4026),#56414,.F.);
#57127=ADVANCED_FACE('',(#4027),#56415,.F.);
#57128=ADVANCED_FACE('',(#4028),#56416,.F.);
#57129=ADVANCED_FACE('',(#4029),#56417,.F.);
#57130=ADVANCED_FACE('',(#4030),#56418,.F.);
#57131=ADVANCED_FACE('',(#4031),#56419,.F.);
#57132=ADVANCED_FACE('',(#4032),#56420,.F.);
#57133=ADVANCED_FACE('',(#4033),#56421,.F.);
#57134=ADVANCED_FACE('',(#4034),#56422,.F.);
#57135=ADVANCED_FACE('',(#4035),#56423,.F.);
#57136=ADVANCED_FACE('',(#4036),#56424,.F.);
#57137=ADVANCED_FACE('',(#4037),#56425,.F.);
#57138=ADVANCED_FACE('',(#4038),#56426,.F.);
#57139=ADVANCED_FACE('',(#4039),#56427,.F.);
#57140=ADVANCED_FACE('',(#4040),#56428,.F.);
#57141=ADVANCED_FACE('',(#4041),#56429,.F.);
#57142=ADVANCED_FACE('',(#4042),#56430,.F.);
#57143=ADVANCED_FACE('',(#4043),#56431,.F.);
#57144=ADVANCED_FACE('',(#4044),#56432,.F.);
#57145=ADVANCED_FACE('',(#4045,#1542),#1859,.T.);
#57146=ADVANCED_FACE('',(#4046),#56433,.F.);
#57147=ADVANCED_FACE('',(#4047),#56434,.F.);
#57148=ADVANCED_FACE('',(#4048),#56435,.F.);
#57149=ADVANCED_FACE('',(#4049),#56436,.F.);
#57150=ADVANCED_FACE('',(#4050),#56437,.F.);
#57151=ADVANCED_FACE('',(#4051),#56438,.F.);
#57152=ADVANCED_FACE('',(#4052),#56439,.F.);
#57153=ADVANCED_FACE('',(#4053),#56440,.F.);
#57154=ADVANCED_FACE('',(#4054),#56441,.F.);
#57155=ADVANCED_FACE('',(#4055),#56442,.F.);
#57156=ADVANCED_FACE('',(#4056),#56443,.F.);
#57157=ADVANCED_FACE('',(#4057),#56444,.F.);
#57158=ADVANCED_FACE('',(#4058),#56445,.F.);
#57159=ADVANCED_FACE('',(#4059),#56446,.F.);
#57160=ADVANCED_FACE('',(#4060),#56447,.F.);
#57161=ADVANCED_FACE('',(#4061),#56448,.F.);
#57162=ADVANCED_FACE('',(#4062),#56449,.F.);
#57163=ADVANCED_FACE('',(#4063),#56450,.F.);
#57164=ADVANCED_FACE('',(#4064),#56451,.F.);
#57165=ADVANCED_FACE('',(#4065),#56452,.F.);
#57166=ADVANCED_FACE('',(#4066),#56453,.F.);
#57167=ADVANCED_FACE('',(#4067),#56454,.F.);
#57168=ADVANCED_FACE('',(#4068),#56455,.F.);
#57169=ADVANCED_FACE('',(#4069),#56456,.F.);
#57170=ADVANCED_FACE('',(#4070),#56457,.F.);
#57171=ADVANCED_FACE('',(#4071),#56458,.F.);
#57172=ADVANCED_FACE('',(#4072),#56459,.F.);
#57173=ADVANCED_FACE('',(#4073),#56460,.F.);
#57174=ADVANCED_FACE('',(#4074),#1860,.F.);
#57175=ADVANCED_FACE('',(#4075),#56461,.F.);
#57176=ADVANCED_FACE('',(#4076,#1543),#1861,.T.);
#57177=ADVANCED_FACE('',(#4077),#1862,.T.);
#57178=ADVANCED_FACE('',(#4078),#1863,.T.);
#57179=ADVANCED_FACE('',(#4079),#56462,.F.);
#57180=ADVANCED_FACE('',(#4080),#56463,.F.);
#57181=ADVANCED_FACE('',(#4081),#56464,.F.);
#57182=ADVANCED_FACE('',(#4082),#56465,.F.);
#57183=ADVANCED_FACE('',(#4083),#56466,.F.);
#57184=ADVANCED_FACE('',(#4084),#56467,.F.);
#57185=ADVANCED_FACE('',(#4085),#56468,.F.);
#57186=ADVANCED_FACE('',(#4086),#56469,.F.);
#57187=ADVANCED_FACE('',(#4087),#56470,.F.);
#57188=ADVANCED_FACE('',(#4088),#56471,.F.);
#57189=ADVANCED_FACE('',(#4089),#56472,.F.);
#57190=ADVANCED_FACE('',(#4090),#56473,.F.);
#57191=ADVANCED_FACE('',(#4091),#56474,.F.);
#57192=ADVANCED_FACE('',(#4092),#56475,.F.);
#57193=ADVANCED_FACE('',(#4093),#56476,.F.);
#57194=ADVANCED_FACE('',(#4094),#56477,.F.);
#57195=ADVANCED_FACE('',(#4095),#56478,.F.);
#57196=ADVANCED_FACE('',(#4096),#56479,.F.);
#57197=ADVANCED_FACE('',(#4097),#56480,.F.);
#57198=ADVANCED_FACE('',(#4098),#56481,.F.);
#57199=ADVANCED_FACE('',(#4099,#1544),#1864,.T.);
#57200=ADVANCED_FACE('',(#4100),#56482,.F.);
#57201=ADVANCED_FACE('',(#4101),#56483,.F.);
#57202=ADVANCED_FACE('',(#4102),#56484,.F.);
#57203=ADVANCED_FACE('',(#4103),#56485,.F.);
#57204=ADVANCED_FACE('',(#4104),#56486,.F.);
#57205=ADVANCED_FACE('',(#4105),#56487,.F.);
#57206=ADVANCED_FACE('',(#4106),#56488,.F.);
#57207=ADVANCED_FACE('',(#4107),#56489,.F.);
#57208=ADVANCED_FACE('',(#4108),#56490,.F.);
#57209=ADVANCED_FACE('',(#4109),#56491,.F.);
#57210=ADVANCED_FACE('',(#4110),#56492,.F.);
#57211=ADVANCED_FACE('',(#4111),#56493,.F.);
#57212=ADVANCED_FACE('',(#4112),#56494,.F.);
#57213=ADVANCED_FACE('',(#4113),#56495,.F.);
#57214=ADVANCED_FACE('',(#4114),#56496,.F.);
#57215=ADVANCED_FACE('',(#4115),#56497,.F.);
#57216=ADVANCED_FACE('',(#4116),#56498,.F.);
#57217=ADVANCED_FACE('',(#4117),#56499,.F.);
#57218=ADVANCED_FACE('',(#4118),#56500,.F.);
#57219=ADVANCED_FACE('',(#4119),#56501,.F.);
#57220=ADVANCED_FACE('',(#4120),#56502,.F.);
#57221=ADVANCED_FACE('',(#4121),#56503,.F.);
#57222=ADVANCED_FACE('',(#4122),#56504,.F.);
#57223=ADVANCED_FACE('',(#4123),#56505,.F.);
#57224=ADVANCED_FACE('',(#4124),#56506,.F.);
#57225=ADVANCED_FACE('',(#4125),#56507,.F.);
#57226=ADVANCED_FACE('',(#4126),#56508,.F.);
#57227=ADVANCED_FACE('',(#4127),#56509,.F.);
#57228=ADVANCED_FACE('',(#4128),#56510,.F.);
#57229=ADVANCED_FACE('',(#4129),#56511,.F.);
#57230=ADVANCED_FACE('',(#4130),#56512,.F.);
#57231=ADVANCED_FACE('',(#4131),#56513,.F.);
#57232=ADVANCED_FACE('',(#4132),#56514,.F.);
#57233=ADVANCED_FACE('',(#4133,#1545,#1546),#1865,.T.);
#57234=ADVANCED_FACE('',(#4134),#1866,.T.);
#57235=ADVANCED_FACE('',(#4135),#1867,.T.);
#57236=ADVANCED_FACE('',(#4136),#1868,.T.);
#57237=ADVANCED_FACE('',(#4137),#56515,.F.);
#57238=ADVANCED_FACE('',(#4138),#56516,.F.);
#57239=ADVANCED_FACE('',(#4139),#56517,.F.);
#57240=ADVANCED_FACE('',(#4140),#56518,.F.);
#57241=ADVANCED_FACE('',(#4141),#56519,.F.);
#57242=ADVANCED_FACE('',(#4142),#56520,.F.);
#57243=ADVANCED_FACE('',(#4143),#56521,.F.);
#57244=ADVANCED_FACE('',(#4144),#56522,.F.);
#57245=ADVANCED_FACE('',(#4145),#56523,.F.);
#57246=ADVANCED_FACE('',(#4146),#56524,.F.);
#57247=ADVANCED_FACE('',(#4147),#56525,.F.);
#57248=ADVANCED_FACE('',(#4148),#56526,.F.);
#57249=ADVANCED_FACE('',(#4149),#56527,.F.);
#57250=ADVANCED_FACE('',(#4150),#56528,.F.);
#57251=ADVANCED_FACE('',(#4151),#56529,.F.);
#57252=ADVANCED_FACE('',(#4152),#56530,.F.);
#57253=ADVANCED_FACE('',(#4153),#56531,.F.);
#57254=ADVANCED_FACE('',(#4154),#56532,.F.);
#57255=ADVANCED_FACE('',(#4155),#56533,.F.);
#57256=ADVANCED_FACE('',(#4156),#56534,.F.);
#57257=ADVANCED_FACE('',(#4157,#1547),#1869,.T.);
#57258=ADVANCED_FACE('',(#4158),#56535,.F.);
#57259=ADVANCED_FACE('',(#4159),#56536,.F.);
#57260=ADVANCED_FACE('',(#4160),#56537,.F.);
#57261=ADVANCED_FACE('',(#4161),#1870,.F.);
#57262=ADVANCED_FACE('',(#4162),#56538,.F.);
#57263=ADVANCED_FACE('',(#4163),#56539,.F.);
#57264=ADVANCED_FACE('',(#4164),#56540,.F.);
#57265=ADVANCED_FACE('',(#4165),#1871,.F.);
#57266=ADVANCED_FACE('',(#4166),#1872,.F.);
#57267=ADVANCED_FACE('',(#4167),#1873,.F.);
#57268=ADVANCED_FACE('',(#4168),#1874,.F.);
#57269=ADVANCED_FACE('',(#4169),#1875,.T.);
#57270=ADVANCED_FACE('',(#4170),#1876,.T.);
#57271=ADVANCED_FACE('',(#4171),#56541,.F.);
#57272=ADVANCED_FACE('',(#4172),#56542,.F.);
#57273=ADVANCED_FACE('',(#4173),#56543,.F.);
#57274=ADVANCED_FACE('',(#4174),#56544,.F.);
#57275=ADVANCED_FACE('',(#4175),#56545,.F.);
#57276=ADVANCED_FACE('',(#4176),#56546,.F.);
#57277=ADVANCED_FACE('',(#4177),#56547,.F.);
#57278=ADVANCED_FACE('',(#4178),#56548,.F.);
#57279=ADVANCED_FACE('',(#4179),#56549,.F.);
#57280=ADVANCED_FACE('',(#4180),#56550,.F.);
#57281=ADVANCED_FACE('',(#4181),#56551,.F.);
#57282=ADVANCED_FACE('',(#4182),#56552,.F.);
#57283=ADVANCED_FACE('',(#4183),#56553,.F.);
#57284=ADVANCED_FACE('',(#4184),#56554,.F.);
#57285=ADVANCED_FACE('',(#4185),#56555,.F.);
#57286=ADVANCED_FACE('',(#4186),#56556,.F.);
#57287=ADVANCED_FACE('',(#4187),#56557,.F.);
#57288=ADVANCED_FACE('',(#4188),#56558,.F.);
#57289=ADVANCED_FACE('',(#4189),#56559,.F.);
#57290=ADVANCED_FACE('',(#4190),#56560,.F.);
#57291=ADVANCED_FACE('',(#4191,#1548),#1877,.T.);
#57292=ADVANCED_FACE('',(#4192),#56561,.F.);
#57293=ADVANCED_FACE('',(#4193),#56562,.F.);
#57294=ADVANCED_FACE('',(#4194),#56563,.F.);
#57295=ADVANCED_FACE('',(#4195),#56564,.F.);
#57296=ADVANCED_FACE('',(#4196),#56565,.F.);
#57297=ADVANCED_FACE('',(#4197),#56566,.F.);
#57298=ADVANCED_FACE('',(#4198),#56567,.F.);
#57299=ADVANCED_FACE('',(#4199),#56568,.F.);
#57300=ADVANCED_FACE('',(#4200),#56569,.F.);
#57301=ADVANCED_FACE('',(#4201),#56570,.F.);
#57302=ADVANCED_FACE('',(#4202),#56571,.F.);
#57303=ADVANCED_FACE('',(#4203),#56572,.F.);
#57304=ADVANCED_FACE('',(#4204),#56573,.F.);
#57305=ADVANCED_FACE('',(#4205),#56574,.F.);
#57306=ADVANCED_FACE('',(#4206),#56575,.F.);
#57307=ADVANCED_FACE('',(#4207),#56576,.F.);
#57308=ADVANCED_FACE('',(#4208),#56577,.F.);
#57309=ADVANCED_FACE('',(#4209),#56578,.F.);
#57310=ADVANCED_FACE('',(#4210),#56579,.F.);
#57311=ADVANCED_FACE('',(#4211),#56580,.F.);
#57312=ADVANCED_FACE('',(#4212),#56581,.F.);
#57313=ADVANCED_FACE('',(#4213),#56582,.F.);
#57314=ADVANCED_FACE('',(#4214),#56583,.F.);
#57315=ADVANCED_FACE('',(#4215),#56584,.F.);
#57316=ADVANCED_FACE('',(#4216),#56585,.F.);
#57317=ADVANCED_FACE('',(#4217),#56586,.F.);
#57318=ADVANCED_FACE('',(#4218),#1878,.F.);
#57319=ADVANCED_FACE('',(#4219),#56587,.F.);
#57320=ADVANCED_FACE('',(#4220,#1549),#1879,.T.);
#57321=ADVANCED_FACE('',(#4221),#1880,.T.);
#57322=ADVANCED_FACE('',(#4222),#1881,.T.);
#57323=ADVANCED_FACE('',(#4223),#56588,.F.);
#57324=ADVANCED_FACE('',(#4224),#56589,.F.);
#57325=ADVANCED_FACE('',(#4225),#56590,.F.);
#57326=ADVANCED_FACE('',(#4226),#56591,.F.);
#57327=ADVANCED_FACE('',(#4227),#56592,.F.);
#57328=ADVANCED_FACE('',(#4228),#56593,.F.);
#57329=ADVANCED_FACE('',(#4229),#56594,.F.);
#57330=ADVANCED_FACE('',(#4230),#56595,.F.);
#57331=ADVANCED_FACE('',(#4231),#56596,.F.);
#57332=ADVANCED_FACE('',(#4232),#56597,.F.);
#57333=ADVANCED_FACE('',(#4233),#56598,.F.);
#57334=ADVANCED_FACE('',(#4234),#56599,.F.);
#57335=ADVANCED_FACE('',(#4235),#56600,.F.);
#57336=ADVANCED_FACE('',(#4236),#56601,.F.);
#57337=ADVANCED_FACE('',(#4237),#56602,.F.);
#57338=ADVANCED_FACE('',(#4238),#56603,.F.);
#57339=ADVANCED_FACE('',(#4239),#56604,.F.);
#57340=ADVANCED_FACE('',(#4240),#56605,.F.);
#57341=ADVANCED_FACE('',(#4241),#56606,.F.);
#57342=ADVANCED_FACE('',(#4242),#56607,.F.);
#57343=ADVANCED_FACE('',(#4243,#1550),#1882,.T.);
#57344=ADVANCED_FACE('',(#4244),#56608,.F.);
#57345=ADVANCED_FACE('',(#4245),#56609,.F.);
#57346=ADVANCED_FACE('',(#4246),#56610,.F.);
#57347=ADVANCED_FACE('',(#4247),#56611,.F.);
#57348=ADVANCED_FACE('',(#4248),#56612,.F.);
#57349=ADVANCED_FACE('',(#4249),#56613,.F.);
#57350=ADVANCED_FACE('',(#4250),#1883,.F.);
#57351=ADVANCED_FACE('',(#4251),#1884,.F.);
#57352=ADVANCED_FACE('',(#4252),#1885,.F.);
#57353=ADVANCED_FACE('',(#4253),#1886,.F.);
#57354=ADVANCED_FACE('',(#4254),#1887,.F.);
#57355=ADVANCED_FACE('',(#4255),#1888,.F.);
#57356=ADVANCED_FACE('',(#4256),#56614,.F.);
#57357=ADVANCED_FACE('',(#4257),#56615,.F.);
#57358=ADVANCED_FACE('',(#4258),#56616,.F.);
#57359=ADVANCED_FACE('',(#4259),#56617,.F.);
#57360=ADVANCED_FACE('',(#4260),#56618,.F.);
#57361=ADVANCED_FACE('',(#4261),#56619,.F.);
#57362=ADVANCED_FACE('',(#4262),#56620,.F.);
#57363=ADVANCED_FACE('',(#4263),#56621,.F.);
#57364=ADVANCED_FACE('',(#4264),#1889,.F.);
#57365=ADVANCED_FACE('',(#4265),#56622,.F.);
#57366=ADVANCED_FACE('',(#4266),#1890,.T.);
#57367=ADVANCED_FACE('',(#4267),#1891,.T.);
#57368=ADVANCED_FACE('',(#4268),#56623,.F.);
#57369=ADVANCED_FACE('',(#4269),#56624,.F.);
#57370=ADVANCED_FACE('',(#4270),#56625,.F.);
#57371=ADVANCED_FACE('',(#4271),#56626,.F.);
#57372=ADVANCED_FACE('',(#4272),#56627,.F.);
#57373=ADVANCED_FACE('',(#4273),#56628,.F.);
#57374=ADVANCED_FACE('',(#4274),#56629,.F.);
#57375=ADVANCED_FACE('',(#4275),#56630,.F.);
#57376=ADVANCED_FACE('',(#4276),#56631,.F.);
#57377=ADVANCED_FACE('',(#4277),#56632,.F.);
#57378=ADVANCED_FACE('',(#4278),#56633,.F.);
#57379=ADVANCED_FACE('',(#4279),#56634,.F.);
#57380=ADVANCED_FACE('',(#4280),#56635,.F.);
#57381=ADVANCED_FACE('',(#4281),#56636,.F.);
#57382=ADVANCED_FACE('',(#4282),#56637,.F.);
#57383=ADVANCED_FACE('',(#4283),#56638,.F.);
#57384=ADVANCED_FACE('',(#4284),#56639,.F.);
#57385=ADVANCED_FACE('',(#4285),#56640,.F.);
#57386=ADVANCED_FACE('',(#4286),#56641,.F.);
#57387=ADVANCED_FACE('',(#4287),#56642,.F.);
#57388=ADVANCED_FACE('',(#4288,#1551),#1892,.T.);
#57389=ADVANCED_FACE('',(#4289),#1893,.F.);
#57390=ADVANCED_FACE('',(#4290),#1894,.F.);
#57391=ADVANCED_FACE('',(#4291),#1895,.F.);
#57392=ADVANCED_FACE('',(#4292),#1896,.F.);
#57393=ADVANCED_FACE('',(#4293),#1897,.F.);
#57394=ADVANCED_FACE('',(#4294),#1898,.F.);
#57395=ADVANCED_FACE('',(#4295),#1899,.F.);
#57396=ADVANCED_FACE('',(#4296),#1900,.F.);
#57397=ADVANCED_FACE('',(#4297),#1901,.F.);
#57398=ADVANCED_FACE('',(#4298),#1902,.F.);
#57399=ADVANCED_FACE('',(#4299),#1903,.F.);
#57400=ADVANCED_FACE('',(#4300),#1904,.F.);
#57401=ADVANCED_FACE('',(#4301),#1905,.F.);
#57402=ADVANCED_FACE('',(#4302),#1906,.F.);
#57403=ADVANCED_FACE('',(#4303,#1552),#1907,.F.);
#57404=ADVANCED_FACE('',(#4304),#1908,.T.);
#57405=ADVANCED_FACE('',(#4305),#1909,.T.);
#57406=ADVANCED_FACE('',(#4306),#56643,.F.);
#57407=ADVANCED_FACE('',(#4307),#56644,.F.);
#57408=ADVANCED_FACE('',(#4308),#56645,.F.);
#57409=ADVANCED_FACE('',(#4309),#56646,.F.);
#57410=ADVANCED_FACE('',(#4310),#56647,.F.);
#57411=ADVANCED_FACE('',(#4311),#56648,.F.);
#57412=ADVANCED_FACE('',(#4312),#56649,.F.);
#57413=ADVANCED_FACE('',(#4313),#56650,.F.);
#57414=ADVANCED_FACE('',(#4314),#56651,.F.);
#57415=ADVANCED_FACE('',(#4315),#56652,.F.);
#57416=ADVANCED_FACE('',(#4316),#56653,.F.);
#57417=ADVANCED_FACE('',(#4317),#56654,.F.);
#57418=ADVANCED_FACE('',(#4318),#56655,.F.);
#57419=ADVANCED_FACE('',(#4319),#56656,.F.);
#57420=ADVANCED_FACE('',(#4320),#56657,.F.);
#57421=ADVANCED_FACE('',(#4321),#56658,.F.);
#57422=ADVANCED_FACE('',(#4322),#56659,.F.);
#57423=ADVANCED_FACE('',(#4323),#56660,.F.);
#57424=ADVANCED_FACE('',(#4324),#56661,.F.);
#57425=ADVANCED_FACE('',(#4325),#56662,.F.);
#57426=ADVANCED_FACE('',(#4326,#1553),#1910,.T.);
#57427=ADVANCED_FACE('',(#4327),#56663,.F.);
#57428=ADVANCED_FACE('',(#4328),#56664,.F.);
#57429=ADVANCED_FACE('',(#4329),#56665,.F.);
#57430=ADVANCED_FACE('',(#4330),#56666,.F.);
#57431=ADVANCED_FACE('',(#4331),#56667,.F.);
#57432=ADVANCED_FACE('',(#4332),#56668,.F.);
#57433=ADVANCED_FACE('',(#4333),#56669,.F.);
#57434=ADVANCED_FACE('',(#4334),#56670,.F.);
#57435=ADVANCED_FACE('',(#4335),#56671,.F.);
#57436=ADVANCED_FACE('',(#4336),#56672,.F.);
#57437=ADVANCED_FACE('',(#4337),#56673,.F.);
#57438=ADVANCED_FACE('',(#4338),#56674,.F.);
#57439=ADVANCED_FACE('',(#4339),#1911,.F.);
#57440=ADVANCED_FACE('',(#4340),#56675,.F.);
#57441=ADVANCED_FACE('',(#4341),#56676,.F.);
#57442=ADVANCED_FACE('',(#4342),#56677,.F.);
#57443=ADVANCED_FACE('',(#4343),#56678,.F.);
#57444=ADVANCED_FACE('',(#4344),#56679,.F.);
#57445=ADVANCED_FACE('',(#4345),#56680,.F.);
#57446=ADVANCED_FACE('',(#4346),#56681,.F.);
#57447=ADVANCED_FACE('',(#4347),#1912,.F.);
#57448=ADVANCED_FACE('',(#4348),#56682,.F.);
#57449=ADVANCED_FACE('',(#4349),#56683,.F.);
#57450=ADVANCED_FACE('',(#4350),#56684,.F.);
#57451=ADVANCED_FACE('',(#4351),#56685,.F.);
#57452=ADVANCED_FACE('',(#4352),#56686,.F.);
#57453=ADVANCED_FACE('',(#4353),#56687,.F.);
#57454=ADVANCED_FACE('',(#4354),#56688,.F.);
#57455=ADVANCED_FACE('',(#4355),#1913,.F.);
#57456=ADVANCED_FACE('',(#4356),#56689,.F.);
#57457=ADVANCED_FACE('',(#4357),#1914,.T.);
#57458=ADVANCED_FACE('',(#4358),#1915,.T.);
#57459=ADVANCED_FACE('',(#4359),#56690,.F.);
#57460=ADVANCED_FACE('',(#4360),#56691,.F.);
#57461=ADVANCED_FACE('',(#4361),#56692,.F.);
#57462=ADVANCED_FACE('',(#4362),#56693,.F.);
#57463=ADVANCED_FACE('',(#4363),#56694,.F.);
#57464=ADVANCED_FACE('',(#4364),#56695,.F.);
#57465=ADVANCED_FACE('',(#4365),#56696,.F.);
#57466=ADVANCED_FACE('',(#4366),#56697,.F.);
#57467=ADVANCED_FACE('',(#4367),#56698,.F.);
#57468=ADVANCED_FACE('',(#4368),#56699,.F.);
#57469=ADVANCED_FACE('',(#4369),#56700,.F.);
#57470=ADVANCED_FACE('',(#4370),#56701,.F.);
#57471=ADVANCED_FACE('',(#4371),#56702,.F.);
#57472=ADVANCED_FACE('',(#4372),#56703,.F.);
#57473=ADVANCED_FACE('',(#4373),#56704,.F.);
#57474=ADVANCED_FACE('',(#4374),#56705,.F.);
#57475=ADVANCED_FACE('',(#4375),#56706,.F.);
#57476=ADVANCED_FACE('',(#4376),#56707,.F.);
#57477=ADVANCED_FACE('',(#4377),#56708,.F.);
#57478=ADVANCED_FACE('',(#4378),#56709,.F.);
#57479=ADVANCED_FACE('',(#4379,#1554),#1916,.T.);
#57480=ADVANCED_FACE('',(#4380),#56710,.F.);
#57481=ADVANCED_FACE('',(#4381),#56711,.F.);
#57482=ADVANCED_FACE('',(#4382),#56712,.F.);
#57483=ADVANCED_FACE('',(#4383),#56713,.F.);
#57484=ADVANCED_FACE('',(#4384),#56714,.F.);
#57485=ADVANCED_FACE('',(#4385),#56715,.F.);
#57486=ADVANCED_FACE('',(#4386),#56716,.F.);
#57487=ADVANCED_FACE('',(#4387),#56717,.F.);
#57488=ADVANCED_FACE('',(#4388),#56718,.F.);
#57489=ADVANCED_FACE('',(#4389),#1917,.F.);
#57490=ADVANCED_FACE('',(#4390),#56719,.F.);
#57491=ADVANCED_FACE('',(#4391),#56720,.F.);
#57492=ADVANCED_FACE('',(#4392),#56721,.F.);
#57493=ADVANCED_FACE('',(#4393),#56722,.F.);
#57494=ADVANCED_FACE('',(#4394),#56723,.F.);
#57495=ADVANCED_FACE('',(#4395),#56724,.F.);
#57496=ADVANCED_FACE('',(#4396),#56725,.F.);
#57497=ADVANCED_FACE('',(#4397),#56726,.F.);
#57498=ADVANCED_FACE('',(#4398),#56727,.F.);
#57499=ADVANCED_FACE('',(#4399),#1918,.F.);
#57500=ADVANCED_FACE('',(#4400),#1919,.F.);
#57501=ADVANCED_FACE('',(#4401),#1920,.F.);
#57502=ADVANCED_FACE('',(#4402),#1921,.T.);
#57503=ADVANCED_FACE('',(#4403),#1922,.T.);
#57504=ADVANCED_FACE('',(#4404),#56728,.F.);
#57505=ADVANCED_FACE('',(#4405),#56729,.F.);
#57506=ADVANCED_FACE('',(#4406),#56730,.F.);
#57507=ADVANCED_FACE('',(#4407),#56731,.F.);
#57508=ADVANCED_FACE('',(#4408),#56732,.F.);
#57509=ADVANCED_FACE('',(#4409),#56733,.F.);
#57510=ADVANCED_FACE('',(#4410),#56734,.F.);
#57511=ADVANCED_FACE('',(#4411),#56735,.F.);
#57512=ADVANCED_FACE('',(#4412),#56736,.F.);
#57513=ADVANCED_FACE('',(#4413),#56737,.F.);
#57514=ADVANCED_FACE('',(#4414),#56738,.F.);
#57515=ADVANCED_FACE('',(#4415),#56739,.F.);
#57516=ADVANCED_FACE('',(#4416),#56740,.F.);
#57517=ADVANCED_FACE('',(#4417),#56741,.F.);
#57518=ADVANCED_FACE('',(#4418),#56742,.F.);
#57519=ADVANCED_FACE('',(#4419),#56743,.F.);
#57520=ADVANCED_FACE('',(#4420),#56744,.F.);
#57521=ADVANCED_FACE('',(#4421),#56745,.F.);
#57522=ADVANCED_FACE('',(#4422),#56746,.F.);
#57523=ADVANCED_FACE('',(#4423),#56747,.F.);
#57524=ADVANCED_FACE('',(#4424,#1555),#1923,.T.);
#57525=ADVANCED_FACE('',(#4425),#1924,.F.);
#57526=ADVANCED_FACE('',(#4426),#56748,.F.);
#57527=ADVANCED_FACE('',(#4427),#56749,.F.);
#57528=ADVANCED_FACE('',(#4428),#1925,.F.);
#57529=ADVANCED_FACE('',(#4429),#56750,.F.);
#57530=ADVANCED_FACE('',(#4430),#56751,.F.);
#57531=ADVANCED_FACE('',(#4431),#1926,.F.);
#57532=ADVANCED_FACE('',(#4432),#1927,.F.);
#57533=ADVANCED_FACE('',(#4433),#1928,.F.);
#57534=ADVANCED_FACE('',(#4434),#1929,.T.);
#57535=ADVANCED_FACE('',(#4435),#1930,.T.);
#57536=ADVANCED_FACE('',(#4436),#56752,.F.);
#57537=ADVANCED_FACE('',(#4437),#56753,.F.);
#57538=ADVANCED_FACE('',(#4438),#56754,.F.);
#57539=ADVANCED_FACE('',(#4439),#56755,.F.);
#57540=ADVANCED_FACE('',(#4440),#56756,.F.);
#57541=ADVANCED_FACE('',(#4441),#56757,.F.);
#57542=ADVANCED_FACE('',(#4442),#56758,.F.);
#57543=ADVANCED_FACE('',(#4443),#56759,.F.);
#57544=ADVANCED_FACE('',(#4444),#56760,.F.);
#57545=ADVANCED_FACE('',(#4445),#56761,.F.);
#57546=ADVANCED_FACE('',(#4446),#56762,.F.);
#57547=ADVANCED_FACE('',(#4447),#56763,.F.);
#57548=ADVANCED_FACE('',(#4448),#56764,.F.);
#57549=ADVANCED_FACE('',(#4449),#56765,.F.);
#57550=ADVANCED_FACE('',(#4450),#56766,.F.);
#57551=ADVANCED_FACE('',(#4451),#56767,.F.);
#57552=ADVANCED_FACE('',(#4452),#56768,.F.);
#57553=ADVANCED_FACE('',(#4453),#56769,.F.);
#57554=ADVANCED_FACE('',(#4454),#56770,.F.);
#57555=ADVANCED_FACE('',(#4455),#56771,.F.);
#57556=ADVANCED_FACE('',(#4456,#1556),#1931,.T.);
#57557=ADVANCED_FACE('',(#4457),#1932,.T.);
#57558=ADVANCED_FACE('',(#4458),#56772,.F.);
#57559=ADVANCED_FACE('',(#4459),#56773,.F.);
#57560=ADVANCED_FACE('',(#4460),#56774,.F.);
#57561=ADVANCED_FACE('',(#4461),#56775,.F.);
#57562=ADVANCED_FACE('',(#4462),#56776,.F.);
#57563=ADVANCED_FACE('',(#4463),#56777,.F.);
#57564=ADVANCED_FACE('',(#4464),#56778,.F.);
#57565=ADVANCED_FACE('',(#4465),#56779,.F.);
#57566=ADVANCED_FACE('',(#4466),#56780,.F.);
#57567=ADVANCED_FACE('',(#4467),#56781,.F.);
#57568=ADVANCED_FACE('',(#4468),#56782,.F.);
#57569=ADVANCED_FACE('',(#4469),#56783,.F.);
#57570=ADVANCED_FACE('',(#4470),#56784,.F.);
#57571=ADVANCED_FACE('',(#4471),#56785,.F.);
#57572=ADVANCED_FACE('',(#4472),#56786,.F.);
#57573=ADVANCED_FACE('',(#4473),#56787,.F.);
#57574=ADVANCED_FACE('',(#4474),#56788,.F.);
#57575=ADVANCED_FACE('',(#4475),#56789,.F.);
#57576=ADVANCED_FACE('',(#4476),#56790,.F.);
#57577=ADVANCED_FACE('',(#4477),#56791,.F.);
#57578=ADVANCED_FACE('',(#4478,#1557),#1933,.T.);
#57579=ADVANCED_FACE('',(#4479),#1934,.F.);
#57580=ADVANCED_FACE('',(#4480),#56792,.F.);
#57581=ADVANCED_FACE('',(#4481),#56793,.F.);
#57582=ADVANCED_FACE('',(#4482),#1935,.F.);
#57583=ADVANCED_FACE('',(#4483),#56794,.F.);
#57584=ADVANCED_FACE('',(#4484),#56795,.F.);
#57585=ADVANCED_FACE('',(#4485),#1936,.F.);
#57586=ADVANCED_FACE('',(#4486),#1937,.F.);
#57587=ADVANCED_FACE('',(#4487),#1938,.F.);
#57588=ADVANCED_FACE('',(#4488),#1939,.T.);
#57589=ADVANCED_FACE('',(#4489),#1940,.T.);
#57590=ADVANCED_FACE('',(#4490),#56796,.F.);
#57591=ADVANCED_FACE('',(#4491),#56797,.F.);
#57592=ADVANCED_FACE('',(#4492),#56798,.F.);
#57593=ADVANCED_FACE('',(#4493),#56799,.F.);
#57594=ADVANCED_FACE('',(#4494),#56800,.F.);
#57595=ADVANCED_FACE('',(#4495),#56801,.F.);
#57596=ADVANCED_FACE('',(#4496),#56802,.F.);
#57597=ADVANCED_FACE('',(#4497),#56803,.F.);
#57598=ADVANCED_FACE('',(#4498),#56804,.F.);
#57599=ADVANCED_FACE('',(#4499),#56805,.F.);
#57600=ADVANCED_FACE('',(#4500),#56806,.F.);
#57601=ADVANCED_FACE('',(#4501),#56807,.F.);
#57602=ADVANCED_FACE('',(#4502),#56808,.F.);
#57603=ADVANCED_FACE('',(#4503),#56809,.F.);
#57604=ADVANCED_FACE('',(#4504),#56810,.F.);
#57605=ADVANCED_FACE('',(#4505),#56811,.F.);
#57606=ADVANCED_FACE('',(#4506),#56812,.F.);
#57607=ADVANCED_FACE('',(#4507),#56813,.F.);
#57608=ADVANCED_FACE('',(#4508),#56814,.F.);
#57609=ADVANCED_FACE('',(#4509),#56815,.F.);
#57610=ADVANCED_FACE('',(#4510,#1558),#1941,.T.);
#57611=ADVANCED_FACE('',(#4511),#56816,.F.);
#57612=ADVANCED_FACE('',(#4512),#56817,.F.);
#57613=ADVANCED_FACE('',(#4513),#56818,.F.);
#57614=ADVANCED_FACE('',(#4514),#56819,.F.);
#57615=ADVANCED_FACE('',(#4515),#56820,.F.);
#57616=ADVANCED_FACE('',(#4516),#56821,.F.);
#57617=ADVANCED_FACE('',(#4517),#56822,.F.);
#57618=ADVANCED_FACE('',(#4518),#56823,.F.);
#57619=ADVANCED_FACE('',(#4519),#56824,.F.);
#57620=ADVANCED_FACE('',(#4520),#1942,.F.);
#57621=ADVANCED_FACE('',(#4521),#56825,.F.);
#57622=ADVANCED_FACE('',(#4522),#56826,.F.);
#57623=ADVANCED_FACE('',(#4523),#56827,.F.);
#57624=ADVANCED_FACE('',(#4524),#56828,.F.);
#57625=ADVANCED_FACE('',(#4525),#56829,.F.);
#57626=ADVANCED_FACE('',(#4526),#56830,.F.);
#57627=ADVANCED_FACE('',(#4527),#56831,.F.);
#57628=ADVANCED_FACE('',(#4528),#56832,.F.);
#57629=ADVANCED_FACE('',(#4529),#56833,.F.);
#57630=ADVANCED_FACE('',(#4530),#1943,.F.);
#57631=ADVANCED_FACE('',(#4531),#1944,.F.);
#57632=ADVANCED_FACE('',(#4532),#1945,.F.);
#57633=ADVANCED_FACE('',(#4533),#1946,.T.);
#57634=ADVANCED_FACE('',(#4534),#1947,.T.);
#57635=ADVANCED_FACE('',(#4535),#56834,.F.);
#57636=ADVANCED_FACE('',(#4536),#56835,.F.);
#57637=ADVANCED_FACE('',(#4537),#56836,.F.);
#57638=ADVANCED_FACE('',(#4538),#56837,.F.);
#57639=ADVANCED_FACE('',(#4539),#56838,.F.);
#57640=ADVANCED_FACE('',(#4540),#56839,.F.);
#57641=ADVANCED_FACE('',(#4541),#56840,.F.);
#57642=ADVANCED_FACE('',(#4542),#56841,.F.);
#57643=ADVANCED_FACE('',(#4543),#56842,.F.);
#57644=ADVANCED_FACE('',(#4544),#56843,.F.);
#57645=ADVANCED_FACE('',(#4545),#56844,.F.);
#57646=ADVANCED_FACE('',(#4546),#56845,.F.);
#57647=ADVANCED_FACE('',(#4547),#56846,.F.);
#57648=ADVANCED_FACE('',(#4548),#56847,.F.);
#57649=ADVANCED_FACE('',(#4549),#56848,.F.);
#57650=ADVANCED_FACE('',(#4550),#56849,.F.);
#57651=ADVANCED_FACE('',(#4551),#56850,.F.);
#57652=ADVANCED_FACE('',(#4552),#56851,.F.);
#57653=ADVANCED_FACE('',(#4553),#56852,.F.);
#57654=ADVANCED_FACE('',(#4554),#56853,.F.);
#57655=ADVANCED_FACE('',(#4555,#1559),#1948,.T.);
#57656=ADVANCED_FACE('',(#4556),#56854,.F.);
#57657=ADVANCED_FACE('',(#4557),#56855,.F.);
#57658=ADVANCED_FACE('',(#4558),#56856,.F.);
#57659=ADVANCED_FACE('',(#4559),#56857,.F.);
#57660=ADVANCED_FACE('',(#4560),#56858,.F.);
#57661=ADVANCED_FACE('',(#4561),#56859,.F.);
#57662=ADVANCED_FACE('',(#4562),#56860,.F.);
#57663=ADVANCED_FACE('',(#4563),#56861,.F.);
#57664=ADVANCED_FACE('',(#4564),#56862,.F.);
#57665=ADVANCED_FACE('',(#4565),#56863,.F.);
#57666=ADVANCED_FACE('',(#4566),#56864,.F.);
#57667=ADVANCED_FACE('',(#4567),#56865,.F.);
#57668=ADVANCED_FACE('',(#4568),#1949,.F.);
#57669=ADVANCED_FACE('',(#4569),#56866,.F.);
#57670=ADVANCED_FACE('',(#4570),#56867,.F.);
#57671=ADVANCED_FACE('',(#4571),#56868,.F.);
#57672=ADVANCED_FACE('',(#4572),#56869,.F.);
#57673=ADVANCED_FACE('',(#4573),#56870,.F.);
#57674=ADVANCED_FACE('',(#4574),#56871,.F.);
#57675=ADVANCED_FACE('',(#4575),#56872,.F.);
#57676=ADVANCED_FACE('',(#4576),#1950,.F.);
#57677=ADVANCED_FACE('',(#4577),#56873,.F.);
#57678=ADVANCED_FACE('',(#4578),#56874,.F.);
#57679=ADVANCED_FACE('',(#4579),#56875,.F.);
#57680=ADVANCED_FACE('',(#4580),#56876,.F.);
#57681=ADVANCED_FACE('',(#4581),#56877,.F.);
#57682=ADVANCED_FACE('',(#4582),#56878,.F.);
#57683=ADVANCED_FACE('',(#4583),#56879,.F.);
#57684=ADVANCED_FACE('',(#4584),#1951,.F.);
#57685=ADVANCED_FACE('',(#4585),#56880,.F.);
#57686=ADVANCED_FACE('',(#4586),#1952,.T.);
#57687=ADVANCED_FACE('',(#4587),#1953,.T.);
#57688=ADVANCED_FACE('',(#4588),#56881,.F.);
#57689=ADVANCED_FACE('',(#4589),#56882,.F.);
#57690=ADVANCED_FACE('',(#4590),#56883,.F.);
#57691=ADVANCED_FACE('',(#4591),#56884,.F.);
#57692=ADVANCED_FACE('',(#4592),#56885,.F.);
#57693=ADVANCED_FACE('',(#4593),#56886,.F.);
#57694=ADVANCED_FACE('',(#4594),#56887,.F.);
#57695=ADVANCED_FACE('',(#4595),#56888,.F.);
#57696=ADVANCED_FACE('',(#4596),#56889,.F.);
#57697=ADVANCED_FACE('',(#4597),#56890,.F.);
#57698=ADVANCED_FACE('',(#4598),#56891,.F.);
#57699=ADVANCED_FACE('',(#4599),#56892,.F.);
#57700=ADVANCED_FACE('',(#4600),#56893,.F.);
#57701=ADVANCED_FACE('',(#4601),#56894,.F.);
#57702=ADVANCED_FACE('',(#4602),#56895,.F.);
#57703=ADVANCED_FACE('',(#4603),#56896,.F.);
#57704=ADVANCED_FACE('',(#4604),#56897,.F.);
#57705=ADVANCED_FACE('',(#4605),#56898,.F.);
#57706=ADVANCED_FACE('',(#4606),#56899,.F.);
#57707=ADVANCED_FACE('',(#4607),#56900,.F.);
#57708=ADVANCED_FACE('',(#4608,#1560),#1954,.T.);
#57709=ADVANCED_FACE('',(#4609),#1955,.F.);
#57710=ADVANCED_FACE('',(#4610),#1956,.F.);
#57711=ADVANCED_FACE('',(#4611),#1957,.F.);
#57712=ADVANCED_FACE('',(#4612),#1958,.F.);
#57713=ADVANCED_FACE('',(#4613),#1959,.F.);
#57714=ADVANCED_FACE('',(#4614),#1960,.F.);
#57715=ADVANCED_FACE('',(#4615),#1961,.F.);
#57716=ADVANCED_FACE('',(#4616),#1962,.F.);
#57717=ADVANCED_FACE('',(#4617),#1963,.F.);
#57718=ADVANCED_FACE('',(#4618),#1964,.F.);
#57719=ADVANCED_FACE('',(#4619),#1965,.F.);
#57720=ADVANCED_FACE('',(#4620),#1966,.F.);
#57721=ADVANCED_FACE('',(#4621),#1967,.F.);
#57722=ADVANCED_FACE('',(#4622),#1968,.F.);
#57723=ADVANCED_FACE('',(#4623,#1561),#1969,.F.);
#57724=ADVANCED_FACE('',(#4624),#1970,.T.);
#57725=ADVANCED_FACE('',(#4625),#1971,.T.);
#57726=ADVANCED_FACE('',(#4626),#56901,.F.);
#57727=ADVANCED_FACE('',(#4627),#56902,.F.);
#57728=ADVANCED_FACE('',(#4628),#56903,.F.);
#57729=ADVANCED_FACE('',(#4629),#56904,.F.);
#57730=ADVANCED_FACE('',(#4630),#56905,.F.);
#57731=ADVANCED_FACE('',(#4631),#56906,.F.);
#57732=ADVANCED_FACE('',(#4632),#56907,.F.);
#57733=ADVANCED_FACE('',(#4633),#56908,.F.);
#57734=ADVANCED_FACE('',(#4634),#56909,.F.);
#57735=ADVANCED_FACE('',(#4635),#56910,.F.);
#57736=ADVANCED_FACE('',(#4636),#56911,.F.);
#57737=ADVANCED_FACE('',(#4637),#56912,.F.);
#57738=ADVANCED_FACE('',(#4638),#56913,.F.);
#57739=ADVANCED_FACE('',(#4639),#56914,.F.);
#57740=ADVANCED_FACE('',(#4640),#56915,.F.);
#57741=ADVANCED_FACE('',(#4641),#56916,.F.);
#57742=ADVANCED_FACE('',(#4642),#56917,.F.);
#57743=ADVANCED_FACE('',(#4643),#56918,.F.);
#57744=ADVANCED_FACE('',(#4644),#56919,.F.);
#57745=ADVANCED_FACE('',(#4645),#56920,.F.);
#57746=ADVANCED_FACE('',(#4646,#1562),#1972,.T.);
#57747=ADVANCED_FACE('',(#4647),#56921,.F.);
#57748=ADVANCED_FACE('',(#4648),#56922,.F.);
#57749=ADVANCED_FACE('',(#4649),#56923,.F.);
#57750=ADVANCED_FACE('',(#4650),#56924,.F.);
#57751=ADVANCED_FACE('',(#4651),#56925,.F.);
#57752=ADVANCED_FACE('',(#4652),#56926,.F.);
#57753=ADVANCED_FACE('',(#4653),#1973,.F.);
#57754=ADVANCED_FACE('',(#4654),#1974,.F.);
#57755=ADVANCED_FACE('',(#4655),#1975,.F.);
#57756=ADVANCED_FACE('',(#4656),#1976,.F.);
#57757=ADVANCED_FACE('',(#4657),#1977,.F.);
#57758=ADVANCED_FACE('',(#4658),#1978,.F.);
#57759=ADVANCED_FACE('',(#4659),#56927,.F.);
#57760=ADVANCED_FACE('',(#4660),#56928,.F.);
#57761=ADVANCED_FACE('',(#4661),#56929,.F.);
#57762=ADVANCED_FACE('',(#4662),#56930,.F.);
#57763=ADVANCED_FACE('',(#4663),#56931,.F.);
#57764=ADVANCED_FACE('',(#4664),#56932,.F.);
#57765=ADVANCED_FACE('',(#4665),#56933,.F.);
#57766=ADVANCED_FACE('',(#4666),#56934,.F.);
#57767=ADVANCED_FACE('',(#4667),#1979,.F.);
#57768=ADVANCED_FACE('',(#4668),#56935,.F.);
#57769=ADVANCED_FACE('',(#4669),#1980,.T.);
#57770=ADVANCED_FACE('',(#4670),#1981,.T.);
#57771=ADVANCED_FACE('',(#4671),#56936,.F.);
#57772=ADVANCED_FACE('',(#4672),#56937,.F.);
#57773=ADVANCED_FACE('',(#4673),#56938,.F.);
#57774=ADVANCED_FACE('',(#4674),#56939,.F.);
#57775=ADVANCED_FACE('',(#4675),#56940,.F.);
#57776=ADVANCED_FACE('',(#4676),#56941,.F.);
#57777=ADVANCED_FACE('',(#4677),#56942,.F.);
#57778=ADVANCED_FACE('',(#4678),#56943,.F.);
#57779=ADVANCED_FACE('',(#4679),#56944,.F.);
#57780=ADVANCED_FACE('',(#4680),#56945,.F.);
#57781=ADVANCED_FACE('',(#4681),#56946,.F.);
#57782=ADVANCED_FACE('',(#4682),#56947,.F.);
#57783=ADVANCED_FACE('',(#4683),#56948,.F.);
#57784=ADVANCED_FACE('',(#4684),#56949,.F.);
#57785=ADVANCED_FACE('',(#4685),#56950,.F.);
#57786=ADVANCED_FACE('',(#4686),#56951,.F.);
#57787=ADVANCED_FACE('',(#4687),#56952,.F.);
#57788=ADVANCED_FACE('',(#4688),#56953,.F.);
#57789=ADVANCED_FACE('',(#4689),#56954,.F.);
#57790=ADVANCED_FACE('',(#4690),#56955,.F.);
#57791=ADVANCED_FACE('',(#4691,#1563),#1982,.T.);
#57792=ADVANCED_FACE('',(#4692),#56956,.F.);
#57793=ADVANCED_FACE('',(#4693),#56957,.F.);
#57794=ADVANCED_FACE('',(#4694),#56958,.F.);
#57795=ADVANCED_FACE('',(#4695),#56959,.F.);
#57796=ADVANCED_FACE('',(#4696),#56960,.F.);
#57797=ADVANCED_FACE('',(#4697),#56961,.F.);
#57798=ADVANCED_FACE('',(#4698),#56962,.F.);
#57799=ADVANCED_FACE('',(#4699),#56963,.F.);
#57800=ADVANCED_FACE('',(#4700),#56964,.F.);
#57801=ADVANCED_FACE('',(#4701),#56965,.F.);
#57802=ADVANCED_FACE('',(#4702),#56966,.F.);
#57803=ADVANCED_FACE('',(#4703),#56967,.F.);
#57804=ADVANCED_FACE('',(#4704),#56968,.F.);
#57805=ADVANCED_FACE('',(#4705),#56969,.F.);
#57806=ADVANCED_FACE('',(#4706),#56970,.F.);
#57807=ADVANCED_FACE('',(#4707),#56971,.F.);
#57808=ADVANCED_FACE('',(#4708),#56972,.F.);
#57809=ADVANCED_FACE('',(#4709),#56973,.F.);
#57810=ADVANCED_FACE('',(#4710),#56974,.F.);
#57811=ADVANCED_FACE('',(#4711),#56975,.F.);
#57812=ADVANCED_FACE('',(#4712),#56976,.F.);
#57813=ADVANCED_FACE('',(#4713),#56977,.F.);
#57814=ADVANCED_FACE('',(#4714),#56978,.F.);
#57815=ADVANCED_FACE('',(#4715),#56979,.F.);
#57816=ADVANCED_FACE('',(#4716),#56980,.F.);
#57817=ADVANCED_FACE('',(#4717),#56981,.F.);
#57818=ADVANCED_FACE('',(#4718),#1983,.F.);
#57819=ADVANCED_FACE('',(#4719),#56982,.F.);
#57820=ADVANCED_FACE('',(#4720,#1564),#1984,.T.);
#57821=ADVANCED_FACE('',(#4721),#1985,.T.);
#57822=ADVANCED_FACE('',(#4722),#1986,.T.);
#57823=ADVANCED_FACE('',(#4723),#56983,.F.);
#57824=ADVANCED_FACE('',(#4724),#56984,.F.);
#57825=ADVANCED_FACE('',(#4725),#56985,.F.);
#57826=ADVANCED_FACE('',(#4726),#56986,.F.);
#57827=ADVANCED_FACE('',(#4727),#56987,.F.);
#57828=ADVANCED_FACE('',(#4728),#56988,.F.);
#57829=ADVANCED_FACE('',(#4729),#56989,.F.);
#57830=ADVANCED_FACE('',(#4730),#56990,.F.);
#57831=ADVANCED_FACE('',(#4731),#56991,.F.);
#57832=ADVANCED_FACE('',(#4732),#56992,.F.);
#57833=ADVANCED_FACE('',(#4733),#56993,.F.);
#57834=ADVANCED_FACE('',(#4734),#56994,.F.);
#57835=ADVANCED_FACE('',(#4735),#56995,.F.);
#57836=ADVANCED_FACE('',(#4736),#56996,.F.);
#57837=ADVANCED_FACE('',(#4737),#56997,.F.);
#57838=ADVANCED_FACE('',(#4738),#56998,.F.);
#57839=ADVANCED_FACE('',(#4739),#56999,.F.);
#57840=ADVANCED_FACE('',(#4740),#57000,.F.);
#57841=ADVANCED_FACE('',(#4741),#57001,.F.);
#57842=ADVANCED_FACE('',(#4742),#57002,.F.);
#57843=ADVANCED_FACE('',(#4743,#1565),#1987,.T.);
#57844=ADVANCED_FACE('',(#4744),#57003,.F.);
#57845=ADVANCED_FACE('',(#4745),#57004,.F.);
#57846=ADVANCED_FACE('',(#4746),#57005,.F.);
#57847=ADVANCED_FACE('',(#4747),#1988,.F.);
#57848=ADVANCED_FACE('',(#4748),#57006,.F.);
#57849=ADVANCED_FACE('',(#4749),#57007,.F.);
#57850=ADVANCED_FACE('',(#4750),#57008,.F.);
#57851=ADVANCED_FACE('',(#4751),#1989,.F.);
#57852=ADVANCED_FACE('',(#4752),#1990,.F.);
#57853=ADVANCED_FACE('',(#4753),#1991,.F.);
#57854=ADVANCED_FACE('',(#4754),#1992,.F.);
#57855=ADVANCED_FACE('',(#4755),#1993,.T.);
#57856=ADVANCED_FACE('',(#4756),#1994,.T.);
#57857=ADVANCED_FACE('',(#4757),#57009,.F.);
#57858=ADVANCED_FACE('',(#4758),#57010,.F.);
#57859=ADVANCED_FACE('',(#4759),#57011,.F.);
#57860=ADVANCED_FACE('',(#4760),#57012,.F.);
#57861=ADVANCED_FACE('',(#4761),#57013,.F.);
#57862=ADVANCED_FACE('',(#4762),#57014,.F.);
#57863=ADVANCED_FACE('',(#4763),#57015,.F.);
#57864=ADVANCED_FACE('',(#4764),#57016,.F.);
#57865=ADVANCED_FACE('',(#4765),#57017,.F.);
#57866=ADVANCED_FACE('',(#4766),#57018,.F.);
#57867=ADVANCED_FACE('',(#4767),#57019,.F.);
#57868=ADVANCED_FACE('',(#4768),#57020,.F.);
#57869=ADVANCED_FACE('',(#4769),#57021,.F.);
#57870=ADVANCED_FACE('',(#4770),#57022,.F.);
#57871=ADVANCED_FACE('',(#4771),#57023,.F.);
#57872=ADVANCED_FACE('',(#4772),#57024,.F.);
#57873=ADVANCED_FACE('',(#4773),#57025,.F.);
#57874=ADVANCED_FACE('',(#4774),#57026,.F.);
#57875=ADVANCED_FACE('',(#4775),#57027,.F.);
#57876=ADVANCED_FACE('',(#4776),#57028,.F.);
#57877=ADVANCED_FACE('',(#4777,#1566),#1995,.T.);
#57878=ADVANCED_FACE('',(#4778),#57029,.F.);
#57879=ADVANCED_FACE('',(#4779),#57030,.F.);
#57880=ADVANCED_FACE('',(#4780),#57031,.F.);
#57881=ADVANCED_FACE('',(#4781),#57032,.F.);
#57882=ADVANCED_FACE('',(#4782),#57033,.F.);
#57883=ADVANCED_FACE('',(#4783),#57034,.F.);
#57884=ADVANCED_FACE('',(#4784),#57035,.F.);
#57885=ADVANCED_FACE('',(#4785),#57036,.F.);
#57886=ADVANCED_FACE('',(#4786),#57037,.F.);
#57887=ADVANCED_FACE('',(#4787),#57038,.F.);
#57888=ADVANCED_FACE('',(#4788),#57039,.F.);
#57889=ADVANCED_FACE('',(#4789),#57040,.F.);
#57890=ADVANCED_FACE('',(#4790),#57041,.F.);
#57891=ADVANCED_FACE('',(#4791),#57042,.F.);
#57892=ADVANCED_FACE('',(#4792),#57043,.F.);
#57893=ADVANCED_FACE('',(#4793),#57044,.F.);
#57894=ADVANCED_FACE('',(#4794),#57045,.F.);
#57895=ADVANCED_FACE('',(#4795),#57046,.F.);
#57896=ADVANCED_FACE('',(#4796),#57047,.F.);
#57897=ADVANCED_FACE('',(#4797),#57048,.F.);
#57898=ADVANCED_FACE('',(#4798),#57049,.F.);
#57899=ADVANCED_FACE('',(#4799),#57050,.F.);
#57900=ADVANCED_FACE('',(#4800),#57051,.F.);
#57901=ADVANCED_FACE('',(#4801),#57052,.F.);
#57902=ADVANCED_FACE('',(#4802),#57053,.F.);
#57903=ADVANCED_FACE('',(#4803),#57054,.F.);
#57904=ADVANCED_FACE('',(#4804),#57055,.F.);
#57905=ADVANCED_FACE('',(#4805),#57056,.F.);
#57906=ADVANCED_FACE('',(#4806),#57057,.F.);
#57907=ADVANCED_FACE('',(#4807),#57058,.F.);
#57908=ADVANCED_FACE('',(#4808),#57059,.F.);
#57909=ADVANCED_FACE('',(#4809),#57060,.F.);
#57910=ADVANCED_FACE('',(#4810),#57061,.F.);
#57911=ADVANCED_FACE('',(#4811,#1567,#1568),#1996,.T.);
#57912=ADVANCED_FACE('',(#4812),#1997,.T.);
#57913=ADVANCED_FACE('',(#4813),#1998,.T.);
#57914=ADVANCED_FACE('',(#4814),#1999,.T.);
#57915=ADVANCED_FACE('',(#4815),#57062,.F.);
#57916=ADVANCED_FACE('',(#4816),#57063,.F.);
#57917=ADVANCED_FACE('',(#4817),#57064,.F.);
#57918=ADVANCED_FACE('',(#4818),#57065,.F.);
#57919=ADVANCED_FACE('',(#4819),#57066,.F.);
#57920=ADVANCED_FACE('',(#4820),#57067,.F.);
#57921=ADVANCED_FACE('',(#4821),#57068,.F.);
#57922=ADVANCED_FACE('',(#4822),#57069,.F.);
#57923=ADVANCED_FACE('',(#4823),#57070,.F.);
#57924=ADVANCED_FACE('',(#4824),#57071,.F.);
#57925=ADVANCED_FACE('',(#4825),#57072,.F.);
#57926=ADVANCED_FACE('',(#4826),#57073,.F.);
#57927=ADVANCED_FACE('',(#4827),#57074,.F.);
#57928=ADVANCED_FACE('',(#4828),#57075,.F.);
#57929=ADVANCED_FACE('',(#4829),#57076,.F.);
#57930=ADVANCED_FACE('',(#4830),#57077,.F.);
#57931=ADVANCED_FACE('',(#4831),#57078,.F.);
#57932=ADVANCED_FACE('',(#4832),#57079,.F.);
#57933=ADVANCED_FACE('',(#4833),#57080,.F.);
#57934=ADVANCED_FACE('',(#4834),#57081,.F.);
#57935=ADVANCED_FACE('',(#4835,#1569),#2000,.T.);
#57936=ADVANCED_FACE('',(#4836),#57082,.F.);
#57937=ADVANCED_FACE('',(#4837),#57083,.F.);
#57938=ADVANCED_FACE('',(#4838),#57084,.F.);
#57939=ADVANCED_FACE('',(#4839),#57085,.F.);
#57940=ADVANCED_FACE('',(#4840),#57086,.F.);
#57941=ADVANCED_FACE('',(#4841),#57087,.F.);
#57942=ADVANCED_FACE('',(#4842),#57088,.F.);
#57943=ADVANCED_FACE('',(#4843),#57089,.F.);
#57944=ADVANCED_FACE('',(#4844),#57090,.F.);
#57945=ADVANCED_FACE('',(#4845),#57091,.F.);
#57946=ADVANCED_FACE('',(#4846),#57092,.F.);
#57947=ADVANCED_FACE('',(#4847),#57093,.F.);
#57948=ADVANCED_FACE('',(#4848),#57094,.F.);
#57949=ADVANCED_FACE('',(#4849),#57095,.F.);
#57950=ADVANCED_FACE('',(#4850),#57096,.F.);
#57951=ADVANCED_FACE('',(#4851),#57097,.F.);
#57952=ADVANCED_FACE('',(#4852),#57098,.F.);
#57953=ADVANCED_FACE('',(#4853),#57099,.F.);
#57954=ADVANCED_FACE('',(#4854),#57100,.F.);
#57955=ADVANCED_FACE('',(#4855),#57101,.F.);
#57956=ADVANCED_FACE('',(#4856),#57102,.F.);
#57957=ADVANCED_FACE('',(#4857),#57103,.F.);
#57958=ADVANCED_FACE('',(#4858),#57104,.F.);
#57959=ADVANCED_FACE('',(#4859),#57105,.F.);
#57960=ADVANCED_FACE('',(#4860),#57106,.F.);
#57961=ADVANCED_FACE('',(#4861),#57107,.F.);
#57962=ADVANCED_FACE('',(#4862),#57108,.F.);
#57963=ADVANCED_FACE('',(#4863),#57109,.F.);
#57964=ADVANCED_FACE('',(#4864),#2001,.F.);
#57965=ADVANCED_FACE('',(#4865),#57110,.F.);
#57966=ADVANCED_FACE('',(#4866,#1570),#2002,.T.);
#57967=ADVANCED_FACE('',(#4867),#2003,.T.);
#57968=ADVANCED_FACE('',(#4868),#2004,.T.);
#57969=ADVANCED_FACE('',(#4869),#2005,.F.);
#57970=ADVANCED_FACE('',(#4870),#2006,.F.);
#57971=ADVANCED_FACE('',(#4871),#2007,.F.);
#57972=ADVANCED_FACE('',(#4872),#2008,.F.);
#57973=ADVANCED_FACE('',(#4873),#2009,.F.);
#57974=ADVANCED_FACE('',(#4874),#2010,.F.);
#57975=ADVANCED_FACE('',(#4875),#2011,.F.);
#57976=ADVANCED_FACE('',(#4876),#2012,.F.);
#57977=ADVANCED_FACE('',(#4877),#2013,.F.);
#57978=ADVANCED_FACE('',(#4878),#2014,.F.);
#57979=ADVANCED_FACE('',(#4879),#2015,.F.);
#57980=ADVANCED_FACE('',(#4880),#2016,.F.);
#57981=ADVANCED_FACE('',(#4881),#2017,.F.);
#57982=ADVANCED_FACE('',(#4882),#2018,.F.);
#57983=ADVANCED_FACE('',(#4883),#2019,.F.);
#57984=ADVANCED_FACE('',(#4884),#2020,.F.);
#57985=ADVANCED_FACE('',(#4885),#2021,.F.);
#57986=ADVANCED_FACE('',(#4886),#2022,.F.);
#57987=ADVANCED_FACE('',(#4887),#2023,.F.);
#57988=ADVANCED_FACE('',(#4888),#2024,.F.);
#57989=ADVANCED_FACE('',(#4889),#2025,.F.);
#57990=ADVANCED_FACE('',(#4890),#2026,.F.);
#57991=ADVANCED_FACE('',(#4891),#2027,.F.);
#57992=ADVANCED_FACE('',(#4892),#2028,.F.);
#57993=ADVANCED_FACE('',(#4893),#2029,.F.);
#57994=ADVANCED_FACE('',(#4894),#2030,.F.);
#57995=ADVANCED_FACE('',(#4895),#2031,.F.);
#57996=ADVANCED_FACE('',(#4896),#2032,.F.);
#57997=ADVANCED_FACE('',(#4897),#2033,.F.);
#57998=ADVANCED_FACE('',(#4898),#2034,.F.);
#57999=ADVANCED_FACE('',(#4899),#2035,.F.);
#58000=ADVANCED_FACE('',(#4900),#2036,.F.);
#58001=ADVANCED_FACE('',(#4901),#2037,.F.);
#58002=ADVANCED_FACE('',(#4902),#2038,.F.);
#58003=ADVANCED_FACE('',(#4903),#2039,.F.);
#58004=ADVANCED_FACE('',(#4904),#2040,.F.);
#58005=ADVANCED_FACE('',(#4905),#2041,.F.);
#58006=ADVANCED_FACE('',(#4906),#2042,.F.);
#58007=ADVANCED_FACE('',(#4907),#2043,.F.);
#58008=ADVANCED_FACE('',(#4908),#2044,.F.);
#58009=ADVANCED_FACE('',(#4909),#2045,.F.);
#58010=ADVANCED_FACE('',(#4910),#2046,.F.);
#58011=ADVANCED_FACE('',(#4911),#2047,.F.);
#58012=ADVANCED_FACE('',(#4912),#2048,.F.);
#58013=ADVANCED_FACE('',(#4913),#2049,.F.);
#58014=ADVANCED_FACE('',(#4914),#2050,.F.);
#58015=ADVANCED_FACE('',(#4915),#2051,.F.);
#58016=ADVANCED_FACE('',(#4916),#2052,.F.);
#58017=ADVANCED_FACE('',(#4917),#2053,.F.);
#58018=ADVANCED_FACE('',(#4918),#2054,.F.);
#58019=ADVANCED_FACE('',(#4919),#2055,.F.);
#58020=ADVANCED_FACE('',(#4920),#2056,.F.);
#58021=ADVANCED_FACE('',(#4921),#2057,.F.);
#58022=ADVANCED_FACE('',(#4922),#2058,.F.);
#58023=ADVANCED_FACE('',(#4923),#2059,.F.);
#58024=ADVANCED_FACE('',(#4924),#2060,.F.);
#58025=ADVANCED_FACE('',(#4925),#2061,.F.);
#58026=ADVANCED_FACE('',(#4926),#2062,.F.);
#58027=ADVANCED_FACE('',(#4927),#2063,.F.);
#58028=ADVANCED_FACE('',(#4928),#2064,.F.);
#58029=ADVANCED_FACE('',(#4929),#2065,.F.);
#58030=ADVANCED_FACE('',(#4930),#2066,.F.);
#58031=ADVANCED_FACE('',(#4931),#2067,.F.);
#58032=ADVANCED_FACE('',(#4932),#2068,.F.);
#58033=ADVANCED_FACE('',(#4933),#2069,.F.);
#58034=ADVANCED_FACE('',(#4934),#2070,.F.);
#58035=ADVANCED_FACE('',(#4935),#2071,.F.);
#58036=ADVANCED_FACE('',(#4936),#2072,.F.);
#58037=ADVANCED_FACE('',(#4937),#2073,.F.);
#58038=ADVANCED_FACE('',(#4938),#2074,.F.);
#58039=ADVANCED_FACE('',(#4939),#2075,.F.);
#58040=ADVANCED_FACE('',(#4940),#2076,.F.);
#58041=ADVANCED_FACE('',(#4941),#2077,.F.);
#58042=ADVANCED_FACE('',(#4942),#2078,.F.);
#58043=ADVANCED_FACE('',(#4943),#2079,.F.);
#58044=ADVANCED_FACE('',(#4944),#2080,.F.);
#58045=ADVANCED_FACE('',(#4945),#2081,.F.);
#58046=ADVANCED_FACE('',(#4946),#2082,.F.);
#58047=ADVANCED_FACE('',(#4947),#2083,.F.);
#58048=ADVANCED_FACE('',(#4948),#2084,.F.);
#58049=ADVANCED_FACE('',(#4949),#2085,.F.);
#58050=ADVANCED_FACE('',(#4950),#2086,.F.);
#58051=ADVANCED_FACE('',(#4951),#2087,.F.);
#58052=ADVANCED_FACE('',(#4952),#2088,.F.);
#58053=ADVANCED_FACE('',(#4953),#2089,.F.);
#58054=ADVANCED_FACE('',(#4954),#2090,.F.);
#58055=ADVANCED_FACE('',(#4955),#2091,.F.);
#58056=ADVANCED_FACE('',(#4956),#2092,.F.);
#58057=ADVANCED_FACE('',(#4957),#2093,.F.);
#58058=ADVANCED_FACE('',(#4958),#2094,.F.);
#58059=ADVANCED_FACE('',(#4959),#2095,.F.);
#58060=ADVANCED_FACE('',(#4960),#2096,.F.);
#58061=ADVANCED_FACE('',(#4961),#2097,.F.);
#58062=ADVANCED_FACE('',(#4962),#2098,.F.);
#58063=ADVANCED_FACE('',(#4963),#2099,.F.);
#58064=ADVANCED_FACE('',(#4964),#2100,.F.);
#58065=ADVANCED_FACE('',(#4965),#2101,.F.);
#58066=ADVANCED_FACE('',(#4966),#2102,.F.);
#58067=ADVANCED_FACE('',(#4967),#2103,.F.);
#58068=ADVANCED_FACE('',(#4968),#2104,.F.);
#58069=ADVANCED_FACE('',(#4969),#2105,.F.);
#58070=ADVANCED_FACE('',(#4970),#2106,.F.);
#58071=ADVANCED_FACE('',(#4971),#2107,.F.);
#58072=ADVANCED_FACE('',(#4972),#2108,.F.);
#58073=ADVANCED_FACE('',(#4973),#2109,.F.);
#58074=ADVANCED_FACE('',(#4974),#2110,.F.);
#58075=ADVANCED_FACE('',(#4975),#2111,.F.);
#58076=ADVANCED_FACE('',(#4976),#2112,.F.);
#58077=ADVANCED_FACE('',(#4977),#2113,.F.);
#58078=ADVANCED_FACE('',(#4978),#2114,.F.);
#58079=ADVANCED_FACE('',(#4979),#2115,.F.);
#58080=ADVANCED_FACE('',(#4980),#2116,.F.);
#58081=ADVANCED_FACE('',(#4981),#2117,.F.);
#58082=ADVANCED_FACE('',(#4982),#2118,.F.);
#58083=ADVANCED_FACE('',(#4983),#2119,.F.);
#58084=ADVANCED_FACE('',(#4984),#2120,.F.);
#58085=ADVANCED_FACE('',(#4985),#2121,.F.);
#58086=ADVANCED_FACE('',(#4986),#2122,.F.);
#58087=ADVANCED_FACE('',(#4987),#2123,.F.);
#58088=ADVANCED_FACE('',(#4988),#2124,.F.);
#58089=ADVANCED_FACE('',(#4989),#2125,.F.);
#58090=ADVANCED_FACE('',(#4990),#2126,.F.);
#58091=ADVANCED_FACE('',(#4991),#2127,.F.);
#58092=ADVANCED_FACE('',(#4992),#2128,.F.);
#58093=ADVANCED_FACE('',(#4993),#2129,.F.);
#58094=ADVANCED_FACE('',(#4994),#2130,.F.);
#58095=ADVANCED_FACE('',(#4995),#2131,.F.);
#58096=ADVANCED_FACE('',(#4996),#2132,.F.);
#58097=ADVANCED_FACE('',(#4997),#2133,.F.);
#58098=ADVANCED_FACE('',(#4998),#2134,.F.);
#58099=ADVANCED_FACE('',(#4999),#2135,.F.);
#58100=ADVANCED_FACE('',(#5000),#2136,.F.);
#58101=ADVANCED_FACE('',(#5001),#2137,.F.);
#58102=ADVANCED_FACE('',(#5002),#2138,.F.);
#58103=ADVANCED_FACE('',(#5003),#2139,.F.);
#58104=ADVANCED_FACE('',(#5004),#2140,.F.);
#58105=ADVANCED_FACE('',(#5005),#2141,.F.);
#58106=ADVANCED_FACE('',(#5006),#2142,.F.);
#58107=ADVANCED_FACE('',(#5007),#2143,.F.);
#58108=ADVANCED_FACE('',(#5008),#2144,.F.);
#58109=ADVANCED_FACE('',(#5009),#2145,.F.);
#58110=ADVANCED_FACE('',(#5010),#2146,.F.);
#58111=ADVANCED_FACE('',(#5011),#2147,.F.);
#58112=ADVANCED_FACE('',(#5012),#2148,.F.);
#58113=ADVANCED_FACE('',(#5013),#2149,.F.);
#58114=ADVANCED_FACE('',(#5014),#2150,.F.);
#58115=ADVANCED_FACE('',(#5015),#2151,.F.);
#58116=ADVANCED_FACE('',(#5016),#2152,.F.);
#58117=ADVANCED_FACE('',(#5017),#2153,.F.);
#58118=ADVANCED_FACE('',(#5018),#2154,.F.);
#58119=ADVANCED_FACE('',(#5019),#2155,.F.);
#58120=ADVANCED_FACE('',(#5020),#2156,.F.);
#58121=ADVANCED_FACE('',(#5021),#2157,.F.);
#58122=ADVANCED_FACE('',(#5022),#2158,.F.);
#58123=ADVANCED_FACE('',(#5023),#2159,.F.);
#58124=ADVANCED_FACE('',(#5024),#2160,.F.);
#58125=ADVANCED_FACE('',(#5025),#2161,.F.);
#58126=ADVANCED_FACE('',(#5026),#2162,.F.);
#58127=ADVANCED_FACE('',(#5027),#2163,.F.);
#58128=ADVANCED_FACE('',(#5028),#2164,.F.);
#58129=ADVANCED_FACE('',(#5029),#2165,.F.);
#58130=ADVANCED_FACE('',(#5030),#2166,.F.);
#58131=ADVANCED_FACE('',(#5031),#2167,.F.);
#58132=ADVANCED_FACE('',(#5032),#2168,.F.);
#58133=ADVANCED_FACE('',(#5033),#2169,.F.);
#58134=ADVANCED_FACE('',(#5034),#2170,.F.);
#58135=ADVANCED_FACE('',(#5035),#2171,.F.);
#58136=ADVANCED_FACE('',(#5036),#2172,.F.);
#58137=ADVANCED_FACE('',(#5037),#2173,.F.);
#58138=ADVANCED_FACE('',(#5038),#2174,.F.);
#58139=ADVANCED_FACE('',(#5039),#2175,.F.);
#58140=ADVANCED_FACE('',(#5040),#2176,.F.);
#58141=ADVANCED_FACE('',(#5041),#2177,.F.);
#58142=ADVANCED_FACE('',(#5042),#2178,.F.);
#58143=ADVANCED_FACE('',(#5043),#2179,.F.);
#58144=ADVANCED_FACE('',(#5044),#2180,.F.);
#58145=ADVANCED_FACE('',(#5045),#2181,.F.);
#58146=ADVANCED_FACE('',(#5046),#2182,.F.);
#58147=ADVANCED_FACE('',(#5047),#2183,.F.);
#58148=ADVANCED_FACE('',(#5048),#2184,.F.);
#58149=ADVANCED_FACE('',(#5049),#2185,.F.);
#58150=ADVANCED_FACE('',(#5050),#2186,.F.);
#58151=ADVANCED_FACE('',(#5051),#2187,.F.);
#58152=ADVANCED_FACE('',(#5052),#2188,.F.);
#58153=ADVANCED_FACE('',(#5053),#2189,.F.);
#58154=ADVANCED_FACE('',(#5054),#2190,.F.);
#58155=ADVANCED_FACE('',(#5055),#2191,.F.);
#58156=ADVANCED_FACE('',(#5056),#2192,.F.);
#58157=ADVANCED_FACE('',(#5057),#2193,.F.);
#58158=ADVANCED_FACE('',(#5058),#2194,.F.);
#58159=ADVANCED_FACE('',(#5059),#2195,.F.);
#58160=ADVANCED_FACE('',(#5060),#2196,.F.);
#58161=ADVANCED_FACE('',(#5061),#2197,.F.);
#58162=ADVANCED_FACE('',(#5062),#2198,.F.);
#58163=ADVANCED_FACE('',(#5063),#2199,.F.);
#58164=ADVANCED_FACE('',(#5064),#2200,.F.);
#58165=ADVANCED_FACE('',(#5065),#2201,.F.);
#58166=ADVANCED_FACE('',(#5066),#2202,.F.);
#58167=ADVANCED_FACE('',(#5067),#2203,.F.);
#58168=ADVANCED_FACE('',(#5068),#2204,.F.);
#58169=ADVANCED_FACE('',(#5069),#2205,.F.);
#58170=ADVANCED_FACE('',(#5070),#2206,.F.);
#58171=ADVANCED_FACE('',(#5071),#2207,.F.);
#58172=ADVANCED_FACE('',(#5072),#2208,.F.);
#58173=ADVANCED_FACE('',(#5073),#2209,.F.);
#58174=ADVANCED_FACE('',(#5074),#2210,.F.);
#58175=ADVANCED_FACE('',(#5075),#2211,.F.);
#58176=ADVANCED_FACE('',(#5076),#2212,.F.);
#58177=ADVANCED_FACE('',(#5077),#2213,.F.);
#58178=ADVANCED_FACE('',(#5078),#2214,.F.);
#58179=ADVANCED_FACE('',(#5079),#2215,.F.);
#58180=ADVANCED_FACE('',(#5080),#2216,.F.);
#58181=ADVANCED_FACE('',(#5081),#2217,.F.);
#58182=ADVANCED_FACE('',(#5082),#2218,.F.);
#58183=ADVANCED_FACE('',(#5083),#2219,.F.);
#58184=ADVANCED_FACE('',(#5084),#2220,.F.);
#58185=ADVANCED_FACE('',(#5085),#2221,.F.);
#58186=ADVANCED_FACE('',(#5086),#2222,.F.);
#58187=ADVANCED_FACE('',(#5087),#2223,.F.);
#58188=ADVANCED_FACE('',(#5088),#2224,.F.);
#58189=ADVANCED_FACE('',(#5089),#2225,.F.);
#58190=ADVANCED_FACE('',(#5090),#2226,.F.);
#58191=ADVANCED_FACE('',(#5091),#2227,.F.);
#58192=ADVANCED_FACE('',(#5092),#2228,.F.);
#58193=ADVANCED_FACE('',(#5093),#2229,.F.);
#58194=ADVANCED_FACE('',(#5094),#2230,.F.);
#58195=ADVANCED_FACE('',(#5095),#2231,.F.);
#58196=ADVANCED_FACE('',(#5096),#2232,.F.);
#58197=ADVANCED_FACE('',(#5097),#2233,.F.);
#58198=ADVANCED_FACE('',(#5098),#2234,.F.);
#58199=ADVANCED_FACE('',(#5099),#2235,.F.);
#58200=ADVANCED_FACE('',(#5100),#2236,.F.);
#58201=ADVANCED_FACE('',(#5101),#2237,.F.);
#58202=ADVANCED_FACE('',(#5102),#2238,.F.);
#58203=ADVANCED_FACE('',(#5103),#2239,.F.);
#58204=ADVANCED_FACE('',(#5104),#2240,.F.);
#58205=ADVANCED_FACE('',(#5105),#2241,.F.);
#58206=ADVANCED_FACE('',(#5106),#2242,.F.);
#58207=ADVANCED_FACE('',(#5107),#2243,.F.);
#58208=ADVANCED_FACE('',(#5108),#2244,.F.);
#58209=ADVANCED_FACE('',(#5109),#2245,.F.);
#58210=ADVANCED_FACE('',(#5110),#2246,.F.);
#58211=ADVANCED_FACE('',(#5111),#2247,.F.);
#58212=ADVANCED_FACE('',(#5112),#2248,.F.);
#58213=ADVANCED_FACE('',(#5113),#2249,.F.);
#58214=ADVANCED_FACE('',(#5114),#2250,.F.);
#58215=ADVANCED_FACE('',(#5115),#2251,.F.);
#58216=ADVANCED_FACE('',(#5116),#2252,.F.);
#58217=ADVANCED_FACE('',(#5117),#2253,.F.);
#58218=ADVANCED_FACE('',(#5118),#2254,.F.);
#58219=ADVANCED_FACE('',(#5119),#2255,.F.);
#58220=ADVANCED_FACE('',(#5120),#2256,.F.);
#58221=ADVANCED_FACE('',(#5121),#2257,.F.);
#58222=ADVANCED_FACE('',(#5122),#2258,.F.);
#58223=ADVANCED_FACE('',(#5123),#2259,.F.);
#58224=ADVANCED_FACE('',(#5124),#2260,.F.);
#58225=ADVANCED_FACE('',(#5125),#2261,.F.);
#58226=ADVANCED_FACE('',(#5126),#2262,.F.);
#58227=ADVANCED_FACE('',(#5127),#2263,.F.);
#58228=ADVANCED_FACE('',(#5128),#2264,.F.);
#58229=ADVANCED_FACE('',(#5129),#2265,.F.);
#58230=ADVANCED_FACE('',(#5130),#2266,.F.);
#58231=ADVANCED_FACE('',(#5131),#2267,.F.);
#58232=ADVANCED_FACE('',(#5132),#2268,.F.);
#58233=ADVANCED_FACE('',(#5133),#2269,.F.);
#58234=ADVANCED_FACE('',(#5134),#2270,.F.);
#58235=ADVANCED_FACE('',(#5135),#2271,.F.);
#58236=ADVANCED_FACE('',(#5136),#2272,.F.);
#58237=ADVANCED_FACE('',(#5137),#2273,.F.);
#58238=ADVANCED_FACE('',(#5138),#2274,.F.);
#58239=ADVANCED_FACE('',(#5139),#2275,.F.);
#58240=ADVANCED_FACE('',(#5140),#2276,.F.);
#58241=ADVANCED_FACE('',(#5141),#2277,.F.);
#58242=ADVANCED_FACE('',(#5142),#2278,.F.);
#58243=ADVANCED_FACE('',(#5143),#2279,.F.);
#58244=ADVANCED_FACE('',(#5144),#2280,.F.);
#58245=ADVANCED_FACE('',(#5145),#2281,.F.);
#58246=ADVANCED_FACE('',(#5146),#2282,.F.);
#58247=ADVANCED_FACE('',(#5147),#2283,.F.);
#58248=ADVANCED_FACE('',(#5148),#2284,.F.);
#58249=ADVANCED_FACE('',(#5149),#2285,.F.);
#58250=ADVANCED_FACE('',(#5150),#2286,.F.);
#58251=ADVANCED_FACE('',(#5151),#2287,.F.);
#58252=ADVANCED_FACE('',(#5152),#2288,.F.);
#58253=ADVANCED_FACE('',(#5153),#2289,.F.);
#58254=ADVANCED_FACE('',(#5154),#2290,.F.);
#58255=ADVANCED_FACE('',(#5155),#2291,.F.);
#58256=ADVANCED_FACE('',(#5156),#2292,.F.);
#58257=ADVANCED_FACE('',(#5157),#2293,.F.);
#58258=ADVANCED_FACE('',(#5158),#2294,.F.);
#58259=ADVANCED_FACE('',(#5159),#2295,.F.);
#58260=ADVANCED_FACE('',(#5160),#2296,.F.);
#58261=ADVANCED_FACE('',(#5161),#2297,.F.);
#58262=ADVANCED_FACE('',(#5162),#2298,.F.);
#58263=ADVANCED_FACE('',(#5163),#2299,.F.);
#58264=ADVANCED_FACE('',(#5164),#2300,.F.);
#58265=ADVANCED_FACE('',(#5165),#2301,.F.);
#58266=ADVANCED_FACE('',(#5166),#2302,.F.);
#58267=ADVANCED_FACE('',(#5167),#2303,.F.);
#58268=ADVANCED_FACE('',(#5168),#2304,.F.);
#58269=ADVANCED_FACE('',(#5169),#2305,.F.);
#58270=ADVANCED_FACE('',(#5170),#2306,.F.);
#58271=ADVANCED_FACE('',(#5171),#2307,.F.);
#58272=ADVANCED_FACE('',(#5172),#2308,.F.);
#58273=ADVANCED_FACE('',(#5173),#2309,.F.);
#58274=ADVANCED_FACE('',(#5174),#2310,.F.);
#58275=ADVANCED_FACE('',(#5175),#2311,.F.);
#58276=ADVANCED_FACE('',(#5176),#2312,.F.);
#58277=ADVANCED_FACE('',(#5177),#2313,.F.);
#58278=ADVANCED_FACE('',(#5178),#2314,.F.);
#58279=ADVANCED_FACE('',(#5179),#2315,.F.);
#58280=ADVANCED_FACE('',(#5180),#2316,.F.);
#58281=ADVANCED_FACE('',(#5181),#2317,.F.);
#58282=ADVANCED_FACE('',(#5182),#2318,.F.);
#58283=ADVANCED_FACE('',(#5183),#2319,.F.);
#58284=ADVANCED_FACE('',(#5184),#2320,.F.);
#58285=ADVANCED_FACE('',(#5185),#2321,.F.);
#58286=ADVANCED_FACE('',(#5186),#2322,.F.);
#58287=ADVANCED_FACE('',(#5187),#2323,.F.);
#58288=ADVANCED_FACE('',(#5188),#2324,.F.);
#58289=ADVANCED_FACE('',(#5189),#2325,.F.);
#58290=ADVANCED_FACE('',(#5190),#2326,.F.);
#58291=ADVANCED_FACE('',(#5191),#2327,.F.);
#58292=ADVANCED_FACE('',(#5192),#2328,.F.);
#58293=ADVANCED_FACE('',(#5193),#2329,.F.);
#58294=ADVANCED_FACE('',(#5194),#2330,.F.);
#58295=ADVANCED_FACE('',(#5195),#2331,.F.);
#58296=ADVANCED_FACE('',(#5196),#2332,.F.);
#58297=ADVANCED_FACE('',(#5197),#2333,.F.);
#58298=ADVANCED_FACE('',(#5198),#2334,.F.);
#58299=ADVANCED_FACE('',(#5199),#2335,.F.);
#58300=ADVANCED_FACE('',(#5200),#2336,.F.);
#58301=ADVANCED_FACE('',(#5201),#2337,.F.);
#58302=ADVANCED_FACE('',(#5202),#2338,.F.);
#58303=ADVANCED_FACE('',(#5203),#2339,.F.);
#58304=ADVANCED_FACE('',(#5204),#2340,.F.);
#58305=ADVANCED_FACE('',(#5205),#2341,.F.);
#58306=ADVANCED_FACE('',(#5206),#2342,.F.);
#58307=ADVANCED_FACE('',(#5207),#2343,.F.);
#58308=ADVANCED_FACE('',(#5208),#2344,.F.);
#58309=ADVANCED_FACE('',(#5209),#2345,.F.);
#58310=ADVANCED_FACE('',(#5210),#2346,.F.);
#58311=ADVANCED_FACE('',(#5211),#2347,.F.);
#58312=ADVANCED_FACE('',(#5212),#2348,.F.);
#58313=ADVANCED_FACE('',(#5213),#2349,.F.);
#58314=ADVANCED_FACE('',(#5214),#2350,.F.);
#58315=ADVANCED_FACE('',(#5215),#2351,.F.);
#58316=ADVANCED_FACE('',(#5216),#2352,.F.);
#58317=ADVANCED_FACE('',(#5217),#2353,.F.);
#58318=ADVANCED_FACE('',(#5218),#2354,.F.);
#58319=ADVANCED_FACE('',(#5219),#2355,.F.);
#58320=ADVANCED_FACE('',(#5220),#2356,.F.);
#58321=ADVANCED_FACE('',(#5221),#2357,.F.);
#58322=ADVANCED_FACE('',(#5222),#2358,.F.);
#58323=ADVANCED_FACE('',(#5223),#2359,.F.);
#58324=ADVANCED_FACE('',(#5224),#2360,.F.);
#58325=ADVANCED_FACE('',(#5225),#2361,.F.);
#58326=ADVANCED_FACE('',(#5226),#2362,.F.);
#58327=ADVANCED_FACE('',(#5227),#2363,.F.);
#58328=ADVANCED_FACE('',(#5228),#2364,.F.);
#58329=ADVANCED_FACE('',(#5229),#2365,.F.);
#58330=ADVANCED_FACE('',(#5230),#2366,.F.);
#58331=ADVANCED_FACE('',(#5231),#2367,.F.);
#58332=ADVANCED_FACE('',(#5232),#2368,.F.);
#58333=ADVANCED_FACE('',(#5233),#2369,.F.);
#58334=ADVANCED_FACE('',(#5234),#2370,.F.);
#58335=ADVANCED_FACE('',(#5235),#2371,.F.);
#58336=ADVANCED_FACE('',(#5236),#2372,.F.);
#58337=ADVANCED_FACE('',(#5237),#2373,.F.);
#58338=ADVANCED_FACE('',(#5238),#2374,.F.);
#58339=ADVANCED_FACE('',(#5239),#2375,.F.);
#58340=ADVANCED_FACE('',(#5240),#2376,.F.);
#58341=ADVANCED_FACE('',(#5241),#2377,.F.);
#58342=ADVANCED_FACE('',(#5242),#2378,.F.);
#58343=ADVANCED_FACE('',(#5243),#2379,.F.);
#58344=ADVANCED_FACE('',(#5244),#2380,.F.);
#58345=ADVANCED_FACE('',(#5245),#2381,.F.);
#58346=ADVANCED_FACE('',(#5246),#2382,.F.);
#58347=ADVANCED_FACE('',(#5247),#2383,.F.);
#58348=ADVANCED_FACE('',(#5248),#2384,.F.);
#58349=ADVANCED_FACE('',(#5249),#2385,.F.);
#58350=ADVANCED_FACE('',(#5250),#2386,.F.);
#58351=ADVANCED_FACE('',(#5251),#2387,.F.);
#58352=ADVANCED_FACE('',(#5252),#2388,.F.);
#58353=ADVANCED_FACE('',(#5253),#2389,.F.);
#58354=ADVANCED_FACE('',(#5254),#2390,.F.);
#58355=ADVANCED_FACE('',(#5255),#2391,.F.);
#58356=ADVANCED_FACE('',(#5256),#2392,.F.);
#58357=ADVANCED_FACE('',(#5257),#2393,.F.);
#58358=ADVANCED_FACE('',(#5258),#2394,.F.);
#58359=ADVANCED_FACE('',(#5259),#2395,.F.);
#58360=ADVANCED_FACE('',(#5260),#2396,.F.);
#58361=ADVANCED_FACE('',(#5261),#2397,.F.);
#58362=ADVANCED_FACE('',(#5262),#2398,.F.);
#58363=ADVANCED_FACE('',(#5263),#2399,.F.);
#58364=ADVANCED_FACE('',(#5264),#2400,.F.);
#58365=ADVANCED_FACE('',(#5265),#2401,.F.);
#58366=ADVANCED_FACE('',(#5266),#2402,.F.);
#58367=ADVANCED_FACE('',(#5267),#2403,.F.);
#58368=ADVANCED_FACE('',(#5268),#2404,.F.);
#58369=ADVANCED_FACE('',(#5269),#2405,.F.);
#58370=ADVANCED_FACE('',(#5270),#2406,.F.);
#58371=ADVANCED_FACE('',(#5271),#2407,.F.);
#58372=ADVANCED_FACE('',(#5272),#2408,.F.);
#58373=ADVANCED_FACE('',(#5273),#2409,.F.);
#58374=ADVANCED_FACE('',(#5274),#2410,.F.);
#58375=ADVANCED_FACE('',(#5275),#2411,.F.);
#58376=ADVANCED_FACE('',(#5276),#2412,.F.);
#58377=ADVANCED_FACE('',(#5277),#2413,.F.);
#58378=ADVANCED_FACE('',(#5278),#2414,.F.);
#58379=ADVANCED_FACE('',(#5279),#2415,.F.);
#58380=ADVANCED_FACE('',(#5280),#2416,.F.);
#58381=ADVANCED_FACE('',(#5281),#2417,.F.);
#58382=ADVANCED_FACE('',(#5282),#2418,.F.);
#58383=ADVANCED_FACE('',(#5283),#2419,.F.);
#58384=ADVANCED_FACE('',(#5284),#2420,.F.);
#58385=ADVANCED_FACE('',(#5285),#2421,.F.);
#58386=ADVANCED_FACE('',(#5286),#2422,.F.);
#58387=ADVANCED_FACE('',(#5287),#2423,.F.);
#58388=ADVANCED_FACE('',(#5288),#2424,.F.);
#58389=ADVANCED_FACE('',(#5289),#2425,.F.);
#58390=ADVANCED_FACE('',(#5290),#2426,.F.);
#58391=ADVANCED_FACE('',(#5291),#2427,.F.);
#58392=ADVANCED_FACE('',(#5292),#2428,.F.);
#58393=ADVANCED_FACE('',(#5293),#2429,.F.);
#58394=ADVANCED_FACE('',(#5294),#2430,.F.);
#58395=ADVANCED_FACE('',(#5295),#2431,.F.);
#58396=ADVANCED_FACE('',(#5296),#2432,.F.);
#58397=ADVANCED_FACE('',(#5297),#2433,.F.);
#58398=ADVANCED_FACE('',(#5298),#2434,.F.);
#58399=ADVANCED_FACE('',(#5299),#2435,.F.);
#58400=ADVANCED_FACE('',(#5300),#2436,.F.);
#58401=ADVANCED_FACE('',(#5301),#2437,.F.);
#58402=ADVANCED_FACE('',(#5302),#2438,.F.);
#58403=ADVANCED_FACE('',(#5303),#2439,.F.);
#58404=ADVANCED_FACE('',(#5304),#2440,.F.);
#58405=ADVANCED_FACE('',(#5305),#2441,.F.);
#58406=ADVANCED_FACE('',(#5306),#2442,.F.);
#58407=ADVANCED_FACE('',(#5307),#2443,.F.);
#58408=ADVANCED_FACE('',(#5308),#2444,.F.);
#58409=ADVANCED_FACE('',(#5309),#2445,.F.);
#58410=ADVANCED_FACE('',(#5310),#2446,.F.);
#58411=ADVANCED_FACE('',(#5311),#2447,.F.);
#58412=ADVANCED_FACE('',(#5312),#2448,.F.);
#58413=ADVANCED_FACE('',(#5313),#2449,.F.);
#58414=ADVANCED_FACE('',(#5314),#2450,.F.);
#58415=ADVANCED_FACE('',(#5315),#2451,.F.);
#58416=ADVANCED_FACE('',(#5316),#2452,.F.);
#58417=ADVANCED_FACE('',(#5317),#2453,.F.);
#58418=ADVANCED_FACE('',(#5318),#2454,.F.);
#58419=ADVANCED_FACE('',(#5319),#2455,.F.);
#58420=ADVANCED_FACE('',(#5320),#2456,.F.);
#58421=ADVANCED_FACE('',(#5321),#2457,.F.);
#58422=ADVANCED_FACE('',(#5322),#2458,.F.);
#58423=ADVANCED_FACE('',(#5323),#2459,.F.);
#58424=ADVANCED_FACE('',(#5324),#2460,.F.);
#58425=ADVANCED_FACE('',(#5325),#2461,.F.);
#58426=ADVANCED_FACE('',(#5326),#2462,.F.);
#58427=ADVANCED_FACE('',(#5327),#2463,.F.);
#58428=ADVANCED_FACE('',(#5328),#2464,.F.);
#58429=ADVANCED_FACE('',(#5329),#2465,.F.);
#58430=ADVANCED_FACE('',(#5330),#2466,.F.);
#58431=ADVANCED_FACE('',(#5331),#2467,.F.);
#58432=ADVANCED_FACE('',(#5332),#2468,.F.);
#58433=ADVANCED_FACE('',(#5333),#2469,.F.);
#58434=ADVANCED_FACE('',(#5334),#2470,.F.);
#58435=ADVANCED_FACE('',(#5335),#2471,.F.);
#58436=ADVANCED_FACE('',(#5336),#2472,.F.);
#58437=ADVANCED_FACE('',(#5337),#2473,.F.);
#58438=ADVANCED_FACE('',(#5338),#2474,.F.);
#58439=ADVANCED_FACE('',(#5339),#2475,.F.);
#58440=ADVANCED_FACE('',(#5340),#2476,.F.);
#58441=ADVANCED_FACE('',(#5341),#2477,.F.);
#58442=ADVANCED_FACE('',(#5342),#2478,.F.);
#58443=ADVANCED_FACE('',(#5343),#2479,.F.);
#58444=ADVANCED_FACE('',(#5344),#2480,.F.);
#58445=ADVANCED_FACE('',(#5345),#2481,.F.);
#58446=ADVANCED_FACE('',(#5346),#2482,.F.);
#58447=ADVANCED_FACE('',(#5347),#2483,.F.);
#58448=ADVANCED_FACE('',(#5348),#2484,.F.);
#58449=ADVANCED_FACE('',(#5349),#2485,.F.);
#58450=ADVANCED_FACE('',(#5350),#2486,.F.);
#58451=ADVANCED_FACE('',(#5351),#2487,.F.);
#58452=ADVANCED_FACE('',(#5352),#2488,.F.);
#58453=ADVANCED_FACE('',(#5353),#2489,.F.);
#58454=ADVANCED_FACE('',(#5354),#2490,.F.);
#58455=ADVANCED_FACE('',(#5355),#2491,.F.);
#58456=ADVANCED_FACE('',(#5356),#2492,.F.);
#58457=ADVANCED_FACE('',(#5357),#2493,.F.);
#58458=ADVANCED_FACE('',(#5358),#2494,.F.);
#58459=ADVANCED_FACE('',(#5359),#2495,.F.);
#58460=ADVANCED_FACE('',(#5360),#2496,.F.);
#58461=ADVANCED_FACE('',(#5361),#2497,.F.);
#58462=ADVANCED_FACE('',(#5362),#2498,.F.);
#58463=ADVANCED_FACE('',(#5363),#2499,.F.);
#58464=ADVANCED_FACE('',(#5364),#2500,.F.);
#58465=ADVANCED_FACE('',(#5365),#2501,.F.);
#58466=ADVANCED_FACE('',(#5366),#2502,.F.);
#58467=ADVANCED_FACE('',(#5367),#2503,.F.);
#58468=ADVANCED_FACE('',(#5368),#2504,.F.);
#58469=ADVANCED_FACE('',(#5369),#2505,.F.);
#58470=ADVANCED_FACE('',(#5370),#2506,.F.);
#58471=ADVANCED_FACE('',(#5371),#2507,.F.);
#58472=ADVANCED_FACE('',(#5372),#2508,.F.);
#58473=ADVANCED_FACE('',(#5373),#2509,.F.);
#58474=ADVANCED_FACE('',(#5374),#2510,.F.);
#58475=ADVANCED_FACE('',(#5375),#2511,.F.);
#58476=ADVANCED_FACE('',(#5376),#2512,.F.);
#58477=ADVANCED_FACE('',(#5377),#2513,.F.);
#58478=ADVANCED_FACE('',(#5378),#2514,.F.);
#58479=ADVANCED_FACE('',(#5379),#2515,.F.);
#58480=ADVANCED_FACE('',(#5380),#2516,.F.);
#58481=ADVANCED_FACE('',(#5381),#2517,.F.);
#58482=ADVANCED_FACE('',(#5382),#2518,.F.);
#58483=ADVANCED_FACE('',(#5383),#2519,.F.);
#58484=ADVANCED_FACE('',(#5384),#2520,.F.);
#58485=ADVANCED_FACE('',(#5385),#2521,.F.);
#58486=ADVANCED_FACE('',(#5386),#2522,.F.);
#58487=ADVANCED_FACE('',(#5387),#2523,.F.);
#58488=ADVANCED_FACE('',(#5388),#2524,.F.);
#58489=ADVANCED_FACE('',(#5389),#2525,.F.);
#58490=ADVANCED_FACE('',(#5390),#2526,.F.);
#58491=ADVANCED_FACE('',(#5391),#2527,.F.);
#58492=ADVANCED_FACE('',(#5392),#2528,.F.);
#58493=ADVANCED_FACE('',(#5393),#2529,.F.);
#58494=ADVANCED_FACE('',(#5394),#2530,.F.);
#58495=ADVANCED_FACE('',(#5395),#2531,.F.);
#58496=ADVANCED_FACE('',(#5396),#2532,.F.);
#58497=ADVANCED_FACE('',(#5397),#2533,.F.);
#58498=ADVANCED_FACE('',(#5398),#2534,.F.);
#58499=ADVANCED_FACE('',(#5399),#2535,.F.);
#58500=ADVANCED_FACE('',(#5400),#2536,.F.);
#58501=ADVANCED_FACE('',(#5401),#2537,.F.);
#58502=ADVANCED_FACE('',(#5402),#2538,.F.);
#58503=ADVANCED_FACE('',(#5403),#2539,.F.);
#58504=ADVANCED_FACE('',(#5404),#2540,.F.);
#58505=ADVANCED_FACE('',(#5405),#2541,.F.);
#58506=ADVANCED_FACE('',(#5406),#2542,.F.);
#58507=ADVANCED_FACE('',(#5407),#2543,.F.);
#58508=ADVANCED_FACE('',(#5408),#2544,.F.);
#58509=ADVANCED_FACE('',(#5409),#2545,.F.);
#58510=ADVANCED_FACE('',(#5410),#2546,.F.);
#58511=ADVANCED_FACE('',(#5411),#2547,.F.);
#58512=ADVANCED_FACE('',(#5412),#2548,.F.);
#58513=ADVANCED_FACE('',(#5413),#2549,.F.);
#58514=ADVANCED_FACE('',(#5414),#2550,.F.);
#58515=ADVANCED_FACE('',(#5415),#2551,.F.);
#58516=ADVANCED_FACE('',(#5416),#2552,.F.);
#58517=ADVANCED_FACE('',(#5417),#2553,.F.);
#58518=ADVANCED_FACE('',(#5418),#2554,.F.);
#58519=ADVANCED_FACE('',(#5419),#2555,.F.);
#58520=ADVANCED_FACE('',(#5420),#2556,.F.);
#58521=ADVANCED_FACE('',(#5421),#2557,.F.);
#58522=ADVANCED_FACE('',(#5422),#2558,.F.);
#58523=ADVANCED_FACE('',(#5423),#2559,.F.);
#58524=ADVANCED_FACE('',(#5424),#2560,.F.);
#58525=ADVANCED_FACE('',(#5425),#2561,.F.);
#58526=ADVANCED_FACE('',(#5426),#2562,.F.);
#58527=ADVANCED_FACE('',(#5427),#2563,.F.);
#58528=ADVANCED_FACE('',(#5428),#2564,.F.);
#58529=ADVANCED_FACE('',(#5429),#2565,.F.);
#58530=ADVANCED_FACE('',(#5430),#2566,.F.);
#58531=ADVANCED_FACE('',(#5431),#2567,.F.);
#58532=ADVANCED_FACE('',(#5432),#2568,.F.);
#58533=ADVANCED_FACE('',(#5433),#2569,.F.);
#58534=ADVANCED_FACE('',(#5434),#2570,.F.);
#58535=ADVANCED_FACE('',(#5435),#2571,.F.);
#58536=ADVANCED_FACE('',(#5436),#2572,.F.);
#58537=ADVANCED_FACE('',(#5437),#2573,.F.);
#58538=ADVANCED_FACE('',(#5438),#2574,.F.);
#58539=ADVANCED_FACE('',(#5439),#2575,.F.);
#58540=ADVANCED_FACE('',(#5440),#2576,.F.);
#58541=ADVANCED_FACE('',(#5441),#2577,.F.);
#58542=ADVANCED_FACE('',(#5442),#2578,.F.);
#58543=ADVANCED_FACE('',(#5443),#2579,.F.);
#58544=ADVANCED_FACE('',(#5444),#2580,.F.);
#58545=ADVANCED_FACE('',(#5445),#2581,.F.);
#58546=ADVANCED_FACE('',(#5446),#2582,.F.);
#58547=ADVANCED_FACE('',(#5447),#2583,.F.);
#58548=ADVANCED_FACE('',(#5448),#2584,.F.);
#58549=ADVANCED_FACE('',(#5449),#2585,.F.);
#58550=ADVANCED_FACE('',(#5450),#2586,.F.);
#58551=ADVANCED_FACE('',(#5451),#2587,.F.);
#58552=ADVANCED_FACE('',(#5452),#2588,.F.);
#58553=ADVANCED_FACE('',(#5453),#2589,.F.);
#58554=ADVANCED_FACE('',(#5454),#2590,.F.);
#58555=ADVANCED_FACE('',(#5455),#2591,.F.);
#58556=ADVANCED_FACE('',(#5456),#2592,.F.);
#58557=ADVANCED_FACE('',(#5457),#2593,.F.);
#58558=ADVANCED_FACE('',(#5458),#2594,.F.);
#58559=ADVANCED_FACE('',(#5459),#2595,.F.);
#58560=ADVANCED_FACE('',(#5460),#2596,.F.);
#58561=ADVANCED_FACE('',(#5461),#2597,.F.);
#58562=ADVANCED_FACE('',(#5462),#2598,.F.);
#58563=ADVANCED_FACE('',(#5463),#2599,.F.);
#58564=ADVANCED_FACE('',(#5464),#2600,.F.);
#58565=ADVANCED_FACE('',(#5465),#2601,.F.);
#58566=ADVANCED_FACE('',(#5466),#2602,.F.);
#58567=ADVANCED_FACE('',(#5467),#2603,.F.);
#58568=ADVANCED_FACE('',(#5468),#2604,.F.);
#58569=ADVANCED_FACE('',(#5469),#2605,.F.);
#58570=ADVANCED_FACE('',(#5470),#2606,.F.);
#58571=ADVANCED_FACE('',(#5471),#2607,.F.);
#58572=ADVANCED_FACE('',(#5472),#2608,.F.);
#58573=ADVANCED_FACE('',(#5473),#2609,.F.);
#58574=ADVANCED_FACE('',(#5474),#2610,.F.);
#58575=ADVANCED_FACE('',(#5475),#2611,.F.);
#58576=ADVANCED_FACE('',(#5476),#2612,.F.);
#58577=ADVANCED_FACE('',(#5477),#2613,.F.);
#58578=ADVANCED_FACE('',(#5478),#2614,.F.);
#58579=ADVANCED_FACE('',(#5479),#2615,.F.);
#58580=ADVANCED_FACE('',(#5480),#2616,.F.);
#58581=ADVANCED_FACE('',(#5481),#2617,.F.);
#58582=ADVANCED_FACE('',(#5482),#2618,.F.);
#58583=ADVANCED_FACE('',(#5483),#2619,.F.);
#58584=ADVANCED_FACE('',(#5484),#2620,.F.);
#58585=ADVANCED_FACE('',(#5485),#2621,.F.);
#58586=ADVANCED_FACE('',(#5486),#2622,.F.);
#58587=ADVANCED_FACE('',(#5487),#2623,.F.);
#58588=ADVANCED_FACE('',(#5488),#2624,.F.);
#58589=ADVANCED_FACE('',(#5489),#2625,.F.);
#58590=ADVANCED_FACE('',(#5490),#2626,.F.);
#58591=ADVANCED_FACE('',(#5491),#2627,.F.);
#58592=ADVANCED_FACE('',(#5492),#2628,.F.);
#58593=ADVANCED_FACE('',(#5493),#2629,.F.);
#58594=ADVANCED_FACE('',(#5494),#2630,.F.);
#58595=ADVANCED_FACE('',(#5495),#2631,.F.);
#58596=ADVANCED_FACE('',(#5496),#2632,.F.);
#58597=ADVANCED_FACE('',(#5497),#2633,.F.);
#58598=ADVANCED_FACE('',(#5498),#2634,.F.);
#58599=ADVANCED_FACE('',(#5499),#2635,.F.);
#58600=ADVANCED_FACE('',(#5500),#2636,.F.);
#58601=ADVANCED_FACE('',(#5501),#2637,.F.);
#58602=ADVANCED_FACE('',(#5502),#2638,.F.);
#58603=ADVANCED_FACE('',(#5503),#2639,.F.);
#58604=ADVANCED_FACE('',(#5504),#2640,.F.);
#58605=ADVANCED_FACE('',(#5505),#2641,.F.);
#58606=ADVANCED_FACE('',(#5506),#2642,.F.);
#58607=ADVANCED_FACE('',(#5507),#2643,.F.);
#58608=ADVANCED_FACE('',(#5508),#2644,.F.);
#58609=ADVANCED_FACE('',(#5509),#2645,.F.);
#58610=ADVANCED_FACE('',(#5510),#2646,.F.);
#58611=ADVANCED_FACE('',(#5511),#2647,.F.);
#58612=ADVANCED_FACE('',(#5512),#2648,.F.);
#58613=ADVANCED_FACE('',(#5513),#2649,.F.);
#58614=ADVANCED_FACE('',(#5514),#2650,.F.);
#58615=ADVANCED_FACE('',(#5515),#2651,.F.);
#58616=ADVANCED_FACE('',(#5516),#2652,.F.);
#58617=ADVANCED_FACE('',(#5517),#2653,.F.);
#58618=ADVANCED_FACE('',(#5518),#2654,.F.);
#58619=ADVANCED_FACE('',(#5519),#2655,.F.);
#58620=ADVANCED_FACE('',(#5520),#2656,.F.);
#58621=ADVANCED_FACE('',(#5521),#2657,.F.);
#58622=ADVANCED_FACE('',(#5522),#2658,.F.);
#58623=ADVANCED_FACE('',(#5523),#2659,.F.);
#58624=ADVANCED_FACE('',(#5524),#2660,.F.);
#58625=ADVANCED_FACE('',(#5525),#2661,.F.);
#58626=ADVANCED_FACE('',(#5526),#2662,.F.);
#58627=ADVANCED_FACE('',(#5527),#2663,.F.);
#58628=ADVANCED_FACE('',(#5528),#2664,.F.);
#58629=ADVANCED_FACE('',(#5529),#2665,.F.);
#58630=ADVANCED_FACE('',(#5530),#2666,.F.);
#58631=ADVANCED_FACE('',(#5531),#2667,.F.);
#58632=ADVANCED_FACE('',(#5532),#2668,.F.);
#58633=ADVANCED_FACE('',(#5533),#2669,.F.);
#58634=ADVANCED_FACE('',(#5534),#2670,.F.);
#58635=ADVANCED_FACE('',(#5535),#2671,.F.);
#58636=ADVANCED_FACE('',(#5536),#2672,.F.);
#58637=ADVANCED_FACE('',(#5537),#2673,.F.);
#58638=ADVANCED_FACE('',(#5538),#2674,.F.);
#58639=ADVANCED_FACE('',(#5539),#2675,.F.);
#58640=ADVANCED_FACE('',(#5540),#2676,.F.);
#58641=ADVANCED_FACE('',(#5541),#2677,.F.);
#58642=ADVANCED_FACE('',(#5542),#2678,.F.);
#58643=ADVANCED_FACE('',(#5543),#2679,.F.);
#58644=ADVANCED_FACE('',(#5544),#2680,.F.);
#58645=ADVANCED_FACE('',(#5545),#2681,.F.);
#58646=ADVANCED_FACE('',(#5546),#2682,.F.);
#58647=ADVANCED_FACE('',(#5547),#2683,.F.);
#58648=ADVANCED_FACE('',(#5548),#2684,.F.);
#58649=ADVANCED_FACE('',(#5549),#2685,.F.);
#58650=ADVANCED_FACE('',(#5550),#2686,.F.);
#58651=ADVANCED_FACE('',(#5551),#2687,.F.);
#58652=ADVANCED_FACE('',(#5552),#2688,.F.);
#58653=ADVANCED_FACE('',(#5553),#2689,.F.);
#58654=ADVANCED_FACE('',(#5554),#2690,.F.);
#58655=ADVANCED_FACE('',(#5555),#2691,.F.);
#58656=ADVANCED_FACE('',(#5556),#2692,.F.);
#58657=ADVANCED_FACE('',(#5557),#2693,.F.);
#58658=ADVANCED_FACE('',(#5558),#2694,.F.);
#58659=ADVANCED_FACE('',(#5559),#2695,.F.);
#58660=ADVANCED_FACE('',(#5560),#2696,.F.);
#58661=ADVANCED_FACE('',(#5561),#2697,.F.);
#58662=ADVANCED_FACE('',(#5562),#2698,.F.);
#58663=ADVANCED_FACE('',(#5563),#2699,.F.);
#58664=ADVANCED_FACE('',(#5564),#2700,.F.);
#58665=ADVANCED_FACE('',(#5565),#2701,.F.);
#58666=ADVANCED_FACE('',(#5566),#2702,.F.);
#58667=ADVANCED_FACE('',(#5567),#2703,.F.);
#58668=ADVANCED_FACE('',(#5568),#2704,.F.);
#58669=ADVANCED_FACE('',(#5569),#2705,.F.);
#58670=ADVANCED_FACE('',(#5570),#2706,.F.);
#58671=ADVANCED_FACE('',(#5571),#2707,.F.);
#58672=ADVANCED_FACE('',(#5572),#2708,.F.);
#58673=ADVANCED_FACE('',(#5573),#2709,.F.);
#58674=ADVANCED_FACE('',(#5574),#2710,.F.);
#58675=ADVANCED_FACE('',(#5575),#2711,.F.);
#58676=ADVANCED_FACE('',(#5576),#2712,.F.);
#58677=ADVANCED_FACE('',(#5577),#2713,.F.);
#58678=ADVANCED_FACE('',(#5578),#2714,.F.);
#58679=ADVANCED_FACE('',(#5579),#2715,.F.);
#58680=ADVANCED_FACE('',(#5580),#2716,.F.);
#58681=ADVANCED_FACE('',(#5581),#2717,.F.);
#58682=ADVANCED_FACE('',(#5582),#2718,.F.);
#58683=ADVANCED_FACE('',(#5583),#2719,.F.);
#58684=ADVANCED_FACE('',(#5584),#2720,.F.);
#58685=ADVANCED_FACE('',(#5585),#2721,.F.);
#58686=ADVANCED_FACE('',(#5586),#2722,.F.);
#58687=ADVANCED_FACE('',(#5587),#2723,.F.);
#58688=ADVANCED_FACE('',(#5588),#2724,.F.);
#58689=ADVANCED_FACE('',(#5589),#2725,.F.);
#58690=ADVANCED_FACE('',(#5590),#2726,.F.);
#58691=ADVANCED_FACE('',(#5591),#2727,.F.);
#58692=ADVANCED_FACE('',(#5592),#2728,.F.);
#58693=ADVANCED_FACE('',(#5593),#2729,.F.);
#58694=ADVANCED_FACE('',(#5594),#2730,.F.);
#58695=ADVANCED_FACE('',(#5595),#2731,.F.);
#58696=ADVANCED_FACE('',(#5596),#2732,.F.);
#58697=ADVANCED_FACE('',(#5597),#2733,.F.);
#58698=ADVANCED_FACE('',(#5598),#2734,.F.);
#58699=ADVANCED_FACE('',(#5599),#2735,.F.);
#58700=ADVANCED_FACE('',(#5600),#2736,.F.);
#58701=ADVANCED_FACE('',(#5601),#2737,.F.);
#58702=ADVANCED_FACE('',(#5602),#2738,.F.);
#58703=ADVANCED_FACE('',(#5603),#2739,.F.);
#58704=ADVANCED_FACE('',(#5604),#2740,.F.);
#58705=ADVANCED_FACE('',(#5605),#2741,.F.);
#58706=ADVANCED_FACE('',(#5606),#2742,.F.);
#58707=ADVANCED_FACE('',(#5607),#2743,.F.);
#58708=ADVANCED_FACE('',(#5608),#2744,.F.);
#58709=ADVANCED_FACE('',(#5609),#2745,.F.);
#58710=ADVANCED_FACE('',(#5610),#2746,.F.);
#58711=ADVANCED_FACE('',(#5611),#2747,.F.);
#58712=ADVANCED_FACE('',(#5612),#2748,.F.);
#58713=ADVANCED_FACE('',(#5613),#2749,.F.);
#58714=ADVANCED_FACE('',(#5614),#2750,.F.);
#58715=ADVANCED_FACE('',(#5615),#2751,.F.);
#58716=ADVANCED_FACE('',(#5616),#2752,.F.);
#58717=ADVANCED_FACE('',(#5617),#2753,.F.);
#58718=ADVANCED_FACE('',(#5618),#2754,.F.);
#58719=ADVANCED_FACE('',(#5619),#2755,.F.);
#58720=ADVANCED_FACE('',(#5620),#2756,.F.);
#58721=ADVANCED_FACE('',(#5621),#2757,.F.);
#58722=ADVANCED_FACE('',(#5622),#2758,.F.);
#58723=ADVANCED_FACE('',(#5623),#2759,.F.);
#58724=ADVANCED_FACE('',(#5624),#2760,.F.);
#58725=ADVANCED_FACE('',(#5625),#2761,.F.);
#58726=ADVANCED_FACE('',(#5626),#2762,.F.);
#58727=ADVANCED_FACE('',(#5627),#2763,.F.);
#58728=ADVANCED_FACE('',(#5628),#2764,.F.);
#58729=ADVANCED_FACE('',(#5629),#2765,.F.);
#58730=ADVANCED_FACE('',(#5630),#2766,.F.);
#58731=ADVANCED_FACE('',(#5631),#2767,.F.);
#58732=ADVANCED_FACE('',(#5632),#2768,.F.);
#58733=ADVANCED_FACE('',(#5633),#2769,.F.);
#58734=ADVANCED_FACE('',(#5634),#2770,.F.);
#58735=ADVANCED_FACE('',(#5635),#2771,.F.);
#58736=ADVANCED_FACE('',(#5636),#2772,.F.);
#58737=ADVANCED_FACE('',(#5637),#2773,.F.);
#58738=ADVANCED_FACE('',(#5638),#2774,.F.);
#58739=ADVANCED_FACE('',(#5639),#2775,.F.);
#58740=ADVANCED_FACE('',(#5640),#2776,.F.);
#58741=ADVANCED_FACE('',(#5641),#2777,.F.);
#58742=ADVANCED_FACE('',(#5642),#2778,.F.);
#58743=ADVANCED_FACE('',(#5643),#2779,.F.);
#58744=ADVANCED_FACE('',(#5644),#2780,.F.);
#58745=ADVANCED_FACE('',(#5645),#2781,.F.);
#58746=ADVANCED_FACE('',(#5646),#2782,.F.);
#58747=ADVANCED_FACE('',(#5647),#2783,.F.);
#58748=ADVANCED_FACE('',(#5648),#2784,.F.);
#58749=ADVANCED_FACE('',(#5649),#2785,.F.);
#58750=ADVANCED_FACE('',(#5650),#2786,.F.);
#58751=ADVANCED_FACE('',(#5651),#2787,.F.);
#58752=ADVANCED_FACE('',(#5652),#2788,.F.);
#58753=ADVANCED_FACE('',(#5653),#2789,.F.);
#58754=ADVANCED_FACE('',(#5654),#2790,.F.);
#58755=ADVANCED_FACE('',(#5655),#2791,.F.);
#58756=ADVANCED_FACE('',(#5656),#2792,.F.);
#58757=ADVANCED_FACE('',(#5657),#2793,.F.);
#58758=ADVANCED_FACE('',(#5658),#2794,.F.);
#58759=ADVANCED_FACE('',(#5659),#2795,.F.);
#58760=ADVANCED_FACE('',(#5660),#2796,.F.);
#58761=ADVANCED_FACE('',(#5661),#2797,.F.);
#58762=ADVANCED_FACE('',(#5662),#2798,.F.);
#58763=ADVANCED_FACE('',(#5663),#2799,.F.);
#58764=ADVANCED_FACE('',(#5664),#2800,.F.);
#58765=ADVANCED_FACE('',(#5665),#2801,.F.);
#58766=ADVANCED_FACE('',(#5666),#2802,.F.);
#58767=ADVANCED_FACE('',(#5667),#2803,.F.);
#58768=ADVANCED_FACE('',(#5668),#2804,.F.);
#58769=ADVANCED_FACE('',(#5669),#2805,.F.);
#58770=ADVANCED_FACE('',(#5670),#2806,.F.);
#58771=ADVANCED_FACE('',(#5671),#2807,.F.);
#58772=ADVANCED_FACE('',(#5672),#2808,.F.);
#58773=ADVANCED_FACE('',(#5673),#2809,.F.);
#58774=ADVANCED_FACE('',(#5674),#2810,.F.);
#58775=ADVANCED_FACE('',(#5675),#2811,.F.);
#58776=ADVANCED_FACE('',(#5676),#2812,.F.);
#58777=ADVANCED_FACE('',(#5677),#2813,.F.);
#58778=ADVANCED_FACE('',(#5678),#2814,.F.);
#58779=ADVANCED_FACE('',(#5679),#2815,.F.);
#58780=ADVANCED_FACE('',(#5680),#2816,.F.);
#58781=ADVANCED_FACE('',(#5681),#2817,.F.);
#58782=ADVANCED_FACE('',(#5682),#2818,.F.);
#58783=ADVANCED_FACE('',(#5683),#2819,.F.);
#58784=ADVANCED_FACE('',(#5684),#2820,.F.);
#58785=ADVANCED_FACE('',(#5685),#2821,.F.);
#58786=ADVANCED_FACE('',(#5686),#2822,.F.);
#58787=ADVANCED_FACE('',(#5687),#2823,.F.);
#58788=ADVANCED_FACE('',(#5688),#2824,.F.);
#58789=ADVANCED_FACE('',(#5689),#2825,.F.);
#58790=ADVANCED_FACE('',(#5690),#2826,.F.);
#58791=ADVANCED_FACE('',(#5691),#2827,.F.);
#58792=ADVANCED_FACE('',(#5692),#2828,.F.);
#58793=ADVANCED_FACE('',(#5693),#2829,.F.);
#58794=ADVANCED_FACE('',(#5694),#2830,.F.);
#58795=ADVANCED_FACE('',(#5695),#2831,.F.);
#58796=ADVANCED_FACE('',(#5696),#2832,.F.);
#58797=ADVANCED_FACE('',(#5697),#2833,.F.);
#58798=ADVANCED_FACE('',(#5698),#2834,.F.);
#58799=ADVANCED_FACE('',(#5699),#2835,.F.);
#58800=ADVANCED_FACE('',(#5700),#2836,.F.);
#58801=ADVANCED_FACE('',(#5701),#2837,.F.);
#58802=ADVANCED_FACE('',(#5702),#2838,.F.);
#58803=ADVANCED_FACE('',(#5703),#2839,.F.);
#58804=ADVANCED_FACE('',(#5704),#2840,.F.);
#58805=ADVANCED_FACE('',(#5705),#2841,.F.);
#58806=ADVANCED_FACE('',(#5706),#2842,.F.);
#58807=ADVANCED_FACE('',(#5707),#2843,.F.);
#58808=ADVANCED_FACE('',(#5708),#2844,.F.);
#58809=ADVANCED_FACE('',(#5709),#2845,.F.);
#58810=ADVANCED_FACE('',(#5710),#2846,.F.);
#58811=ADVANCED_FACE('',(#5711),#2847,.F.);
#58812=ADVANCED_FACE('',(#5712),#2848,.F.);
#58813=ADVANCED_FACE('',(#5713),#2849,.F.);
#58814=ADVANCED_FACE('',(#5714),#2850,.F.);
#58815=ADVANCED_FACE('',(#5715),#2851,.F.);
#58816=ADVANCED_FACE('',(#5716),#2852,.F.);
#58817=ADVANCED_FACE('',(#5717),#2853,.F.);
#58818=ADVANCED_FACE('',(#5718),#2854,.F.);
#58819=ADVANCED_FACE('',(#5719),#2855,.F.);
#58820=ADVANCED_FACE('',(#5720),#2856,.F.);
#58821=ADVANCED_FACE('',(#5721),#2857,.F.);
#58822=ADVANCED_FACE('',(#5722),#2858,.F.);
#58823=ADVANCED_FACE('',(#5723),#2859,.F.);
#58824=ADVANCED_FACE('',(#5724),#2860,.F.);
#58825=ADVANCED_FACE('',(#5725),#2861,.F.);
#58826=ADVANCED_FACE('',(#5726),#2862,.F.);
#58827=ADVANCED_FACE('',(#5727),#2863,.F.);
#58828=ADVANCED_FACE('',(#5728),#2864,.F.);
#58829=ADVANCED_FACE('',(#5729),#2865,.F.);
#58830=ADVANCED_FACE('',(#5730),#2866,.F.);
#58831=ADVANCED_FACE('',(#5731),#2867,.F.);
#58832=ADVANCED_FACE('',(#5732),#2868,.F.);
#58833=ADVANCED_FACE('',(#5733),#2869,.F.);
#58834=ADVANCED_FACE('',(#5734),#2870,.F.);
#58835=ADVANCED_FACE('',(#5735),#2871,.F.);
#58836=ADVANCED_FACE('',(#5736),#2872,.F.);
#58837=ADVANCED_FACE('',(#5737),#2873,.F.);
#58838=ADVANCED_FACE('',(#5738),#2874,.F.);
#58839=ADVANCED_FACE('',(#5739),#2875,.F.);
#58840=ADVANCED_FACE('',(#5740),#2876,.F.);
#58841=ADVANCED_FACE('',(#5741),#2877,.F.);
#58842=ADVANCED_FACE('',(#5742),#2878,.F.);
#58843=ADVANCED_FACE('',(#5743),#2879,.F.);
#58844=ADVANCED_FACE('',(#5744),#2880,.F.);
#58845=ADVANCED_FACE('',(#5745),#2881,.F.);
#58846=ADVANCED_FACE('',(#5746),#2882,.F.);
#58847=ADVANCED_FACE('',(#5747),#2883,.F.);
#58848=ADVANCED_FACE('',(#5748),#2884,.F.);
#58849=ADVANCED_FACE('',(#5749),#2885,.F.);
#58850=ADVANCED_FACE('',(#5750),#2886,.F.);
#58851=ADVANCED_FACE('',(#5751),#2887,.F.);
#58852=ADVANCED_FACE('',(#5752),#2888,.F.);
#58853=ADVANCED_FACE('',(#5753),#2889,.F.);
#58854=ADVANCED_FACE('',(#5754),#2890,.F.);
#58855=ADVANCED_FACE('',(#5755),#2891,.F.);
#58856=ADVANCED_FACE('',(#5756),#2892,.F.);
#58857=ADVANCED_FACE('',(#5757),#2893,.F.);
#58858=ADVANCED_FACE('',(#5758),#2894,.F.);
#58859=ADVANCED_FACE('',(#5759),#2895,.F.);
#58860=ADVANCED_FACE('',(#5760),#2896,.F.);
#58861=ADVANCED_FACE('',(#5761),#2897,.F.);
#58862=ADVANCED_FACE('',(#5762),#2898,.F.);
#58863=ADVANCED_FACE('',(#5763),#2899,.F.);
#58864=ADVANCED_FACE('',(#5764),#2900,.F.);
#58865=ADVANCED_FACE('',(#5765),#2901,.F.);
#58866=ADVANCED_FACE('',(#5766),#2902,.F.);
#58867=ADVANCED_FACE('',(#5767),#2903,.F.);
#58868=ADVANCED_FACE('',(#5768),#2904,.F.);
#58869=ADVANCED_FACE('',(#5769),#2905,.F.);
#58870=ADVANCED_FACE('',(#5770),#2906,.F.);
#58871=ADVANCED_FACE('',(#5771),#2907,.F.);
#58872=ADVANCED_FACE('',(#5772),#2908,.F.);
#58873=ADVANCED_FACE('',(#5773),#2909,.F.);
#58874=ADVANCED_FACE('',(#5774),#2910,.F.);
#58875=ADVANCED_FACE('',(#5775),#2911,.F.);
#58876=ADVANCED_FACE('',(#5776),#2912,.F.);
#58877=ADVANCED_FACE('',(#5777),#2913,.F.);
#58878=ADVANCED_FACE('',(#5778),#2914,.T.);
#58879=ADVANCED_FACE('',(#5779),#2915,.T.);
#58880=ADVANCED_FACE('',(#5780),#2916,.T.);
#58881=ADVANCED_FACE('',(#5781,#1571,#1572,#1573),#2917,.T.);
#58882=ADVANCED_FACE('',(#5782),#875,.F.);
#58883=ADVANCED_FACE('',(#5783),#876,.F.);
#58884=ADVANCED_FACE('',(#5784),#603,.F.);
#58885=ADVANCED_FACE('',(#5785),#604,.F.);
#58886=ADVANCED_FACE('',(#5786),#877,.F.);
#58887=ADVANCED_FACE('',(#5787),#605,.F.);
#58888=ADVANCED_FACE('',(#5788,#1574,#1575),#2918,.F.);
#58889=ADVANCED_FACE('',(#5789),#878,.F.);
#58890=ADVANCED_FACE('',(#5790),#879,.F.);
#58891=ADVANCED_FACE('',(#5791),#606,.F.);
#58892=ADVANCED_FACE('',(#5792),#880,.F.);
#58893=ADVANCED_FACE('',(#5793),#607,.F.);
#58894=ADVANCED_FACE('',(#5794,#1576),#2919,.T.);
#58895=ADVANCED_FACE('',(#5795),#608,.F.);
#58896=ADVANCED_FACE('',(#5796,#1577),#2920,.T.);
#58897=ADVANCED_FACE('',(#5797),#609,.F.);
#58898=ADVANCED_FACE('',(#5798,#1578),#2921,.T.);
#58899=ADVANCED_FACE('',(#5799),#610,.F.);
#58900=ADVANCED_FACE('',(#5800,#1579),#2922,.T.);
#58901=ADVANCED_FACE('',(#5801),#611,.F.);
#58902=ADVANCED_FACE('',(#5802,#1580),#2923,.T.);
#58903=ADVANCED_FACE('',(#5803),#612,.F.);
#58904=ADVANCED_FACE('',(#5804,#1581),#2924,.T.);
#58905=ADVANCED_FACE('',(#5805),#881,.F.);
#58906=ADVANCED_FACE('',(#5806,#1582,#1583,#1584),#2925,.T.);
#58907=ADVANCED_FACE('',(#5807),#613,.F.);
#58908=ADVANCED_FACE('',(#5808),#882,.F.);
#58909=ADVANCED_FACE('',(#5809),#614,.F.);
#58910=ADVANCED_FACE('',(#5810),#883,.F.);
#58911=ADVANCED_FACE('',(#5811),#615,.F.);
#58912=ADVANCED_FACE('',(#5812),#884,.F.);
#58913=ADVANCED_FACE('',(#5813),#616,.F.);
#58914=ADVANCED_FACE('',(#5814),#885,.F.);
#58915=ADVANCED_FACE('',(#5815),#617,.F.);
#58916=ADVANCED_FACE('',(#5816),#886,.F.);
#58917=ADVANCED_FACE('',(#5817),#618,.F.);
#58918=ADVANCED_FACE('',(#5818),#2926,.T.);
#58919=ADVANCED_FACE('',(#5819),#2927,.T.);
#58920=ADVANCED_FACE('',(#5820),#2928,.T.);
#58921=ADVANCED_FACE('',(#5821),#2929,.T.);
#58922=ADVANCED_FACE('',(#5822),#2930,.T.);
#58923=ADVANCED_FACE('',(#5823),#2931,.T.);
#58924=ADVANCED_FACE('',(#5824),#2932,.T.);
#58925=ADVANCED_FACE('',(#5825),#2933,.T.);
#58926=ADVANCED_FACE('',(#5826),#2934,.T.);
#58927=ADVANCED_FACE('',(#5827),#619,.F.);
#58928=ADVANCED_FACE('',(#5828),#2935,.T.);
#58929=ADVANCED_FACE('',(#5829),#2936,.T.);
#58930=ADVANCED_FACE('',(#5830),#2937,.T.);
#58931=ADVANCED_FACE('',(#5831),#2938,.F.);
#58932=ADVANCED_FACE('',(#5832),#2939,.F.);
#58933=ADVANCED_FACE('',(#5833),#2940,.T.);
#58934=ADVANCED_FACE('',(#5834),#2941,.T.);
#58935=ADVANCED_FACE('',(#5835),#2942,.T.);
#58936=ADVANCED_FACE('',(#5836),#2943,.T.);
#58937=ADVANCED_FACE('',(#5837),#2944,.T.);
#58938=ADVANCED_FACE('',(#5838),#2945,.T.);
#58939=ADVANCED_FACE('',(#5839),#2946,.T.);
#58940=ADVANCED_FACE('',(#5840),#2947,.T.);
#58941=ADVANCED_FACE('',(#5841,#1585,#1586,#1587,#1588),#2948,.T.);
#58942=ADVANCED_FACE('',(#5842),#2949,.T.);
#58943=ADVANCED_FACE('',(#5843),#2950,.T.);
#58944=ADVANCED_FACE('',(#5844),#2951,.T.);
#58945=ADVANCED_FACE('',(#5845),#2952,.T.);
#58946=ADVANCED_FACE('',(#5846,#1589,#1590,#1591,#1592,#1593,#1594,#1595,
#1596,#1597,#1598,#1599,#1600,#1601,#1602,#1603,#1604,#1605,#1606,#1607,
#1608,#1609,#1610,#1611,#1612,#1613,#1614,#1615,#1616,#1617,#1618,#1619,
#1620,#1621,#1622,#1623,#1624,#1625,#1626,#1627,#1628,#1629,#1630,#1631,
#1632,#1633,#1634,#1635,#1636,#1637,#1638,#1639,#1640,#1641,#1642,#1643,
#1644,#1645,#1646,#1647,#1648,#1649,#1650,#1651,#1652,#1653,#1654,#1655,
#1656,#1657,#1658,#1659,#1660,#1661,#1662,#1663,#1664,#1665,#1666,#1667,
#1668,#1669,#1670,#1671,#1672,#1673,#1674,#1675,#1676,#1677,#1678,#1679,
#1680,#1681,#1682,#1683,#1684,#1685,#1686,#1687,#1688,#1689,#1690,#1691,
#1692,#1693,#1694,#1695,#1696,#1697,#1698,#1699,#1700,#1701,#1702,#1703,
#1704,#1705,#1706,#1707,#1708,#1709,#1710,#1711,#1712,#1713,#1714,#1715,
#1716,#1717,#1718,#1719,#1720,#1721,#1722,#1723,#1724,#1725,#1726,#1727,
#1728,#1729,#1730,#1731,#1732,#1733,#1734,#1735,#1736,#1737,#1738,#1739,
#1740,#1741,#1742,#1743,#1744,#1745,#1746,#1747,#1748,#1749,#1750,#1751,
#1752,#1753,#1754,#1755,#1756,#1757,#1758,#1759,#1760,#1761,#1762,#1763,
#1764,#1765,#1766,#1767,#1768,#1769,#1770,#1771,#1772,#1773,#1774,#1775,
#1776,#1777,#1778,#1779,#1780,#1781,#1782,#1783,#1784,#1785,#1786,#1787,
#1788,#1789,#1790,#1791,#1792,#1793,#1794,#1795,#1796,#1797,#1798,#1799,
#1800,#1801,#1802,#1803,#1804,#1805,#1806),#2953,.T.);
#58947=ADVANCED_FACE('',(#5847),#2954,.T.);
#58948=ADVANCED_FACE('',(#5848,#1807,#1808,#1809,#1810),#2955,.T.);
#58949=ADVANCED_FACE('',(#5849),#2956,.T.);
#58950=ADVANCED_FACE('',(#5850),#2957,.T.);
#58951=ADVANCED_FACE('',(#5851),#2958,.T.);
#58952=ADVANCED_FACE('',(#5852),#2959,.T.);
#58953=ADVANCED_FACE('',(#5853),#2960,.T.);
#58954=ADVANCED_FACE('',(#5854),#2961,.T.);
#58955=ADVANCED_FACE('',(#5855),#2962,.T.);
#58956=ADVANCED_FACE('',(#5856),#2963,.T.);
#58957=ADVANCED_FACE('',(#5857),#2964,.T.);
#58958=ADVANCED_FACE('',(#5858),#2965,.T.);
#58959=ADVANCED_FACE('',(#5859),#2966,.T.);
#58960=ADVANCED_FACE('',(#5860),#2967,.T.);
#58961=ADVANCED_FACE('',(#5861),#2968,.T.);
#58962=ADVANCED_FACE('',(#5862),#2969,.T.);
#58963=ADVANCED_FACE('',(#5863),#2970,.T.);
#58964=ADVANCED_FACE('',(#5864),#2971,.T.);
#58965=ADVANCED_FACE('',(#5865),#2972,.T.);
#58966=ADVANCED_FACE('',(#5866),#2973,.T.);
#58967=ADVANCED_FACE('',(#5867),#2974,.T.);
#58968=ADVANCED_FACE('',(#5868),#2975,.T.);
#58969=ADVANCED_FACE('',(#5869),#620,.F.);
#58970=ADVANCED_FACE('',(#5870),#2976,.T.);
#58971=ADVANCED_FACE('',(#5871),#2977,.T.);
#60392=CLOSED_SHELL('',(#57125,#57126,#57127,#57128,#57129,#57130,#57131,
#57132,#57133,#57134,#57135,#57136,#57137,#57138,#57139,#57140,#57141,#57142,
#57143,#57144,#57145,#57146,#57147,#57148,#57149,#57150,#57151,#57152,#57153,
#57154,#57155,#57156,#57157,#57158,#57159,#57160,#57161,#57162,#57163,#57164,
#57165,#57166,#57167,#57168,#57169,#57170,#57171,#57172,#57173,#57174,#57175,
#57176,#57177,#57178,#57179,#57180,#57181,#57182,#57183,#57184,#57185,#57186,
#57187,#57188,#57189,#57190,#57191,#57192,#57193,#57194,#57195,#57196,#57197,
#57198,#57199,#57200,#57201,#57202,#57203,#57204,#57205,#57206,#57207,#57208,
#57209,#57210,#57211,#57212,#57213,#57214,#57215,#57216,#57217,#57218,#57219,
#57220,#57221,#57222,#57223,#57224,#57225,#57226,#57227,#57228,#57229,#57230,
#57231,#57232,#57233,#57234,#57235,#57236,#57237,#57238,#57239,#57240,#57241,
#57242,#57243,#57244,#57245,#57246,#57247,#57248,#57249,#57250,#57251,#57252,
#57253,#57254,#57255,#57256,#57257,#57258,#57259,#57260,#57261,#57262,#57263,
#57264,#57265,#57266,#57267,#57268,#57269,#57270,#57271,#57272,#57273,#57274,
#57275,#57276,#57277,#57278,#57279,#57280,#57281,#57282,#57283,#57284,#57285,
#57286,#57287,#57288,#57289,#57290,#57291,#57292,#57293,#57294,#57295,#57296,
#57297,#57298,#57299,#57300,#57301,#57302,#57303,#57304,#57305,#57306,#57307,
#57308,#57309,#57310,#57311,#57312,#57313,#57314,#57315,#57316,#57317,#57318,
#57319,#57320,#57321,#57322,#57323,#57324,#57325,#57326,#57327,#57328,#57329,
#57330,#57331,#57332,#57333,#57334,#57335,#57336,#57337,#57338,#57339,#57340,
#57341,#57342,#57343,#57344,#57345,#57346,#57347,#57348,#57349,#57350,#57351,
#57352,#57353,#57354,#57355,#57356,#57357,#57358,#57359,#57360,#57361,#57362,
#57363,#57364,#57365,#57366,#57367,#57368,#57369,#57370,#57371,#57372,#57373,
#57374,#57375,#57376,#57377,#57378,#57379,#57380,#57381,#57382,#57383,#57384,
#57385,#57386,#57387,#57388,#57389,#57390,#57391,#57392,#57393,#57394,#57395,
#57396,#57397,#57398,#57399,#57400,#57401,#57402,#57403,#57404,#57405,#57406,
#57407,#57408,#57409,#57410,#57411,#57412,#57413,#57414,#57415,#57416,#57417,
#57418,#57419,#57420,#57421,#57422,#57423,#57424,#57425,#57426,#57427,#57428,
#57429,#57430,#57431,#57432,#57433,#57434,#57435,#57436,#57437,#57438,#57439,
#57440,#57441,#57442,#57443,#57444,#57445,#57446,#57447,#57448,#57449,#57450,
#57451,#57452,#57453,#57454,#57455,#57456,#57457,#57458,#57459,#57460,#57461,
#57462,#57463,#57464,#57465,#57466,#57467,#57468,#57469,#57470,#57471,#57472,
#57473,#57474,#57475,#57476,#57477,#57478,#57479,#57480,#57481,#57482,#57483,
#57484,#57485,#57486,#57487,#57488,#57489,#57490,#57491,#57492,#57493,#57494,
#57495,#57496,#57497,#57498,#57499,#57500,#57501,#57502,#57503,#57504,#57505,
#57506,#57507,#57508,#57509,#57510,#57511,#57512,#57513,#57514,#57515,#57516,
#57517,#57518,#57519,#57520,#57521,#57522,#57523,#57524,#57525,#57526,#57527,
#57528,#57529,#57530,#57531,#57532,#57533,#57534,#57535,#57536,#57537,#57538,
#57539,#57540,#57541,#57542,#57543,#57544,#57545,#57546,#57547,#57548,#57549,
#57550,#57551,#57552,#57553,#57554,#57555,#57556,#57557,#57558,#57559,#57560,
#57561,#57562,#57563,#57564,#57565,#57566,#57567,#57568,#57569,#57570,#57571,
#57572,#57573,#57574,#57575,#57576,#57577,#57578,#57579,#57580,#57581,#57582,
#57583,#57584,#57585,#57586,#57587,#57588,#57589,#57590,#57591,#57592,#57593,
#57594,#57595,#57596,#57597,#57598,#57599,#57600,#57601,#57602,#57603,#57604,
#57605,#57606,#57607,#57608,#57609,#57610,#57611,#57612,#57613,#57614,#57615,
#57616,#57617,#57618,#57619,#57620,#57621,#57622,#57623,#57624,#57625,#57626,
#57627,#57628,#57629,#57630,#57631,#57632,#57633,#57634,#57635,#57636,#57637,
#57638,#57639,#57640,#57641,#57642,#57643,#57644,#57645,#57646,#57647,#57648,
#57649,#57650,#57651,#57652,#57653,#57654,#57655,#57656,#57657,#57658,#57659,
#57660,#57661,#57662,#57663,#57664,#57665,#57666,#57667,#57668,#57669,#57670,
#57671,#57672,#57673,#57674,#57675,#57676,#57677,#57678,#57679,#57680,#57681,
#57682,#57683,#57684,#57685,#57686,#57687,#57688,#57689,#57690,#57691,#57692,
#57693,#57694,#57695,#57696,#57697,#57698,#57699,#57700,#57701,#57702,#57703,
#57704,#57705,#57706,#57707,#57708,#57709,#57710,#57711,#57712,#57713,#57714,
#57715,#57716,#57717,#57718,#57719,#57720,#57721,#57722,#57723,#57724,#57725,
#57726,#57727,#57728,#57729,#57730,#57731,#57732,#57733,#57734,#57735,#57736,
#57737,#57738,#57739,#57740,#57741,#57742,#57743,#57744,#57745,#57746,#57747,
#57748,#57749,#57750,#57751,#57752,#57753,#57754,#57755,#57756,#57757,#57758,
#57759,#57760,#57761,#57762,#57763,#57764,#57765,#57766,#57767,#57768,#57769,
#57770,#57771,#57772,#57773,#57774,#57775,#57776,#57777,#57778,#57779,#57780,
#57781,#57782,#57783,#57784,#57785,#57786,#57787,#57788,#57789,#57790,#57791,
#57792,#57793,#57794,#57795,#57796,#57797,#57798,#57799,#57800,#57801,#57802,
#57803,#57804,#57805,#57806,#57807,#57808,#57809,#57810,#57811,#57812,#57813,
#57814,#57815,#57816,#57817,#57818,#57819,#57820,#57821,#57822,#57823,#57824,
#57825,#57826,#57827,#57828,#57829,#57830,#57831,#57832,#57833,#57834,#57835,
#57836,#57837,#57838,#57839,#57840,#57841,#57842,#57843,#57844,#57845,#57846,
#57847,#57848,#57849,#57850,#57851,#57852,#57853,#57854,#57855,#57856,#57857,
#57858,#57859,#57860,#57861,#57862,#57863,#57864,#57865,#57866,#57867,#57868,
#57869,#57870,#57871,#57872,#57873,#57874,#57875,#57876,#57877,#57878,#57879,
#57880,#57881,#57882,#57883,#57884,#57885,#57886,#57887,#57888,#57889,#57890,
#57891,#57892,#57893,#57894,#57895,#57896,#57897,#57898,#57899,#57900,#57901,
#57902,#57903,#57904,#57905,#57906,#57907,#57908,#57909,#57910,#57911,#57912,
#57913,#57914,#57915,#57916,#57917,#57918,#57919,#57920,#57921,#57922,#57923,
#57924,#57925,#57926,#57927,#57928,#57929,#57930,#57931,#57932,#57933,#57934,
#57935,#57936,#57937,#57938,#57939,#57940,#57941,#57942,#57943,#57944,#57945,
#57946,#57947,#57948,#57949,#57950,#57951,#57952,#57953,#57954,#57955,#57956,
#57957,#57958,#57959,#57960,#57961,#57962,#57963,#57964,#57965,#57966,#57967,
#57968,#57969,#57970,#57971,#57972,#57973,#57974,#57975,#57976,#57977,#57978,
#57979,#57980,#57981,#57982,#57983,#57984,#57985,#57986,#57987,#57988,#57989,
#57990,#57991,#57992,#57993,#57994,#57995,#57996,#57997,#57998,#57999,#58000,
#58001,#58002,#58003,#58004,#58005,#58006,#58007,#58008,#58009,#58010,#58011,
#58012,#58013,#58014,#58015,#58016,#58017,#58018,#58019,#58020,#58021,#58022,
#58023,#58024,#58025,#58026,#58027,#58028,#58029,#58030,#58031,#58032,#58033,
#58034,#58035,#58036,#58037,#58038,#58039,#58040,#58041,#58042,#58043,#58044,
#58045,#58046,#58047,#58048,#58049,#58050,#58051,#58052,#58053,#58054,#58055,
#58056,#58057,#58058,#58059,#58060,#58061,#58062,#58063,#58064,#58065,#58066,
#58067,#58068,#58069,#58070,#58071,#58072,#58073,#58074,#58075,#58076,#58077,
#58078,#58079,#58080,#58081,#58082,#58083,#58084,#58085,#58086,#58087,#58088,
#58089,#58090,#58091,#58092,#58093,#58094,#58095,#58096,#58097,#58098,#58099,
#58100,#58101,#58102,#58103,#58104,#58105,#58106,#58107,#58108,#58109,#58110,
#58111,#58112,#58113,#58114,#58115,#58116,#58117,#58118,#58119,#58120,#58121,
#58122,#58123,#58124,#58125,#58126,#58127,#58128,#58129,#58130,#58131,#58132,
#58133,#58134,#58135,#58136,#58137,#58138,#58139,#58140,#58141,#58142,#58143,
#58144,#58145,#58146,#58147,#58148,#58149,#58150,#58151,#58152,#58153,#58154,
#58155,#58156,#58157,#58158,#58159,#58160,#58161,#58162,#58163,#58164,#58165,
#58166,#58167,#58168,#58169,#58170,#58171,#58172,#58173,#58174,#58175,#58176,
#58177,#58178,#58179,#58180,#58181,#58182,#58183,#58184,#58185,#58186,#58187,
#58188,#58189,#58190,#58191,#58192,#58193,#58194,#58195,#58196,#58197,#58198,
#58199,#58200,#58201,#58202,#58203,#58204,#58205,#58206,#58207,#58208,#58209,
#58210,#58211,#58212,#58213,#58214,#58215,#58216,#58217,#58218,#58219,#58220,
#58221,#58222,#58223,#58224,#58225,#58226,#58227,#58228,#58229,#58230,#58231,
#58232,#58233,#58234,#58235,#58236,#58237,#58238,#58239,#58240,#58241,#58242,
#58243,#58244,#58245,#58246,#58247,#58248,#58249,#58250,#58251,#58252,#58253,
#58254,#58255,#58256,#58257,#58258,#58259,#58260,#58261,#58262,#58263,#58264,
#58265,#58266,#58267,#58268,#58269,#58270,#58271,#58272,#58273,#58274,#58275,
#58276,#58277,#58278,#58279,#58280,#58281,#58282,#58283,#58284,#58285,#58286,
#58287,#58288,#58289,#58290,#58291,#58292,#58293,#58294,#58295,#58296,#58297,
#58298,#58299,#58300,#58301,#58302,#58303,#58304,#58305,#58306,#58307,#58308,
#58309,#58310,#58311,#58312,#58313,#58314,#58315,#58316,#58317,#58318,#58319,
#58320,#58321,#58322,#58323,#58324,#58325,#58326,#58327,#58328,#58329,#58330,
#58331,#58332,#58333,#58334,#58335,#58336,#58337,#58338,#58339,#58340,#58341,
#58342,#58343,#58344,#58345,#58346,#58347,#58348,#58349,#58350,#58351,#58352,
#58353,#58354,#58355,#58356,#58357,#58358,#58359,#58360,#58361,#58362,#58363,
#58364,#58365,#58366,#58367,#58368,#58369,#58370,#58371,#58372,#58373,#58374,
#58375,#58376,#58377,#58378,#58379,#58380,#58381,#58382,#58383,#58384,#58385,
#58386,#58387,#58388,#58389,#58390,#58391,#58392,#58393,#58394,#58395,#58396,
#58397,#58398,#58399,#58400,#58401,#58402,#58403,#58404,#58405,#58406,#58407,
#58408,#58409,#58410,#58411,#58412,#58413,#58414,#58415,#58416,#58417,#58418,
#58419,#58420,#58421,#58422,#58423,#58424,#58425,#58426,#58427,#58428,#58429,
#58430,#58431,#58432,#58433,#58434,#58435,#58436,#58437,#58438,#58439,#58440,
#58441,#58442,#58443,#58444,#58445,#58446,#58447,#58448,#58449,#58450,#58451,
#58452,#58453,#58454,#58455,#58456,#58457,#58458,#58459,#58460,#58461,#58462,
#58463,#58464,#58465,#58466,#58467,#58468,#58469,#58470,#58471,#58472,#58473,
#58474,#58475,#58476,#58477,#58478,#58479,#58480,#58481,#58482,#58483,#58484,
#58485,#58486,#58487,#58488,#58489,#58490,#58491,#58492,#58493,#58494,#58495,
#58496,#58497,#58498,#58499,#58500,#58501,#58502,#58503,#58504,#58505,#58506,
#58507,#58508,#58509,#58510,#58511,#58512,#58513,#58514,#58515,#58516,#58517,
#58518,#58519,#58520,#58521,#58522,#58523,#58524,#58525,#58526,#58527,#58528,
#58529,#58530,#58531,#58532,#58533,#58534,#58535,#58536,#58537,#58538,#58539,
#58540,#58541,#58542,#58543,#58544,#58545,#58546,#58547,#58548,#58549,#58550,
#58551,#58552,#58553,#58554,#58555,#58556,#58557,#58558,#58559,#58560,#58561,
#58562,#58563,#58564,#58565,#58566,#58567,#58568,#58569,#58570,#58571,#58572,
#58573,#58574,#58575,#58576,#58577,#58578,#58579,#58580,#58581,#58582,#58583,
#58584,#58585,#58586,#58587,#58588,#58589,#58590,#58591,#58592,#58593,#58594,
#58595,#58596,#58597,#58598,#58599,#58600,#58601,#58602,#58603,#58604,#58605,
#58606,#58607,#58608,#58609,#58610,#58611,#58612,#58613,#58614,#58615,#58616,
#58617,#58618,#58619,#58620,#58621,#58622,#58623,#58624,#58625,#58626,#58627,
#58628,#58629,#58630,#58631,#58632,#58633,#58634,#58635,#58636,#58637,#58638,
#58639,#58640,#58641,#58642,#58643,#58644,#58645,#58646,#58647,#58648,#58649,
#58650,#58651,#58652,#58653,#58654,#58655,#58656,#58657,#58658,#58659,#58660,
#58661,#58662,#58663,#58664,#58665,#58666,#58667,#58668,#58669,#58670,#58671,
#58672,#58673,#58674,#58675,#58676,#58677,#58678,#58679,#58680,#58681,#58682,
#58683,#58684,#58685,#58686,#58687,#58688,#58689,#58690,#58691,#58692,#58693,
#58694,#58695,#58696,#58697,#58698,#58699,#58700,#58701,#58702,#58703,#58704,
#58705,#58706,#58707,#58708,#58709,#58710,#58711,#58712,#58713,#58714,#58715,
#58716,#58717,#58718,#58719,#58720,#58721,#58722,#58723,#58724,#58725,#58726,
#58727,#58728,#58729,#58730,#58731,#58732,#58733,#58734,#58735,#58736,#58737,
#58738,#58739,#58740,#58741,#58742,#58743,#58744,#58745,#58746,#58747,#58748,
#58749,#58750,#58751,#58752,#58753,#58754,#58755,#58756,#58757,#58758,#58759,
#58760,#58761,#58762,#58763,#58764,#58765,#58766,#58767,#58768,#58769,#58770,
#58771,#58772,#58773,#58774,#58775,#58776,#58777,#58778,#58779,#58780,#58781,
#58782,#58783,#58784,#58785,#58786,#58787,#58788,#58789,#58790,#58791,#58792,
#58793,#58794,#58795,#58796,#58797,#58798,#58799,#58800,#58801,#58802,#58803,
#58804,#58805,#58806,#58807,#58808,#58809,#58810,#58811,#58812,#58813,#58814,
#58815,#58816,#58817,#58818,#58819,#58820,#58821,#58822,#58823,#58824,#58825,
#58826,#58827,#58828,#58829,#58830,#58831,#58832,#58833,#58834,#58835,#58836,
#58837,#58838,#58839,#58840,#58841,#58842,#58843,#58844,#58845,#58846,#58847,
#58848,#58849,#58850,#58851,#58852,#58853,#58854,#58855,#58856,#58857,#58858,
#58859,#58860,#58861,#58862,#58863,#58864,#58865,#58866,#58867,#58868,#58869,
#58870,#58871,#58872,#58873,#58874,#58875,#58876,#58877,#58878,#58879,#58880,
#58881,#58882,#58883,#58884,#58885,#58886,#58887,#58888,#58889,#58890,#58891,
#58892,#58893,#58894,#58895,#58896,#58897,#58898,#58899,#58900,#58901,#58902,
#58903,#58904,#58905,#58906,#58907,#58908,#58909,#58910,#58911,#58912,#58913,
#58914,#58915,#58916,#58917,#58918,#58919,#58920,#58921,#58922,#58923,#58924,
#58925,#58926,#58927,#58928,#58929,#58930,#58931,#58932,#58933,#58934,#58935,
#58936,#58937,#58938,#58939,#58940,#58941,#58942,#58943,#58944,#58945,#58946,
#58947,#58948,#58949,#58950,#58951,#58952,#58953,#58954,#58955,#58956,#58957,
#58958,#58959,#58960,#58961,#58962,#58963,#58964,#58965,#58966,#58967,#58968,
#58969,#58970,#58971));
#60610=AXIS2_PLACEMENT_3D('',#76145,#63778,#63779);
#60611=AXIS2_PLACEMENT_3D('',#76446,#63800,#63801);
#60612=AXIS2_PLACEMENT_3D('',#76870,#63831,#63832);
#60613=AXIS2_PLACEMENT_3D('',#76888,#63836,#63837);
#60614=AXIS2_PLACEMENT_3D('',#76889,#63838,#63839);
#60615=AXIS2_PLACEMENT_3D('',#76890,#63840,#63841);
#60616=AXIS2_PLACEMENT_3D('',#77191,#63862,#63863);
#60617=AXIS2_PLACEMENT_3D('',#77687,#63897,#63898);
#60618=AXIS2_PLACEMENT_3D('',#77688,#63899,#63900);
#60619=AXIS2_PLACEMENT_3D('',#77689,#63901,#63902);
#60620=AXIS2_PLACEMENT_3D('',#77690,#63903,#63904);
#60621=AXIS2_PLACEMENT_3D('',#77991,#63925,#63926);
#60622=AXIS2_PLACEMENT_3D('',#78040,#63931,#63932);
#60623=AXIS2_PLACEMENT_3D('',#78091,#63939,#63940);
#60624=AXIS2_PLACEMENT_3D('',#78097,#63944,#63945);
#60625=AXIS2_PLACEMENT_3D('',#78103,#63949,#63950);
#60626=AXIS2_PLACEMENT_3D('',#78109,#63954,#63955);
#60627=AXIS2_PLACEMENT_3D('',#78112,#63958,#63959);
#60628=AXIS2_PLACEMENT_3D('',#78113,#63960,#63961);
#60629=AXIS2_PLACEMENT_3D('',#78414,#63982,#63983);
#60630=AXIS2_PLACEMENT_3D('',#78808,#64011,#64012);
#60631=AXIS2_PLACEMENT_3D('',#78826,#64016,#64017);
#60632=AXIS2_PLACEMENT_3D('',#78827,#64018,#64019);
#60633=AXIS2_PLACEMENT_3D('',#78828,#64020,#64021);
#60634=AXIS2_PLACEMENT_3D('',#79129,#64042,#64043);
#60635=AXIS2_PLACEMENT_3D('',#79223,#64051,#64052);
#60636=AXIS2_PLACEMENT_3D('',#79229,#64056,#64057);
#60637=AXIS2_PLACEMENT_3D('',#79235,#64061,#64062);
#60638=AXIS2_PLACEMENT_3D('',#79241,#64066,#64067);
#60639=AXIS2_PLACEMENT_3D('',#79247,#64071,#64072);
#60640=AXIS2_PLACEMENT_3D('',#79253,#64076,#64077);
#60641=AXIS2_PLACEMENT_3D('',#79379,#64089,#64090);
#60642=AXIS2_PLACEMENT_3D('',#79397,#64094,#64095);
#60643=AXIS2_PLACEMENT_3D('',#79398,#64096,#64097);
#60644=AXIS2_PLACEMENT_3D('',#79699,#64118,#64119);
#60645=AXIS2_PLACEMENT_3D('',#79700,#64120,#64121);
#60646=AXIS2_PLACEMENT_3D('',#79709,#64126,#64127);
#60647=AXIS2_PLACEMENT_3D('',#79715,#64131,#64132);
#60648=AXIS2_PLACEMENT_3D('',#79718,#64135,#64136);
#60649=AXIS2_PLACEMENT_3D('',#79727,#64141,#64142);
#60650=AXIS2_PLACEMENT_3D('',#79733,#64146,#64147);
#60651=AXIS2_PLACEMENT_3D('',#79739,#64151,#64152);
#60652=AXIS2_PLACEMENT_3D('',#79745,#64156,#64157);
#60653=AXIS2_PLACEMENT_3D('',#79751,#64161,#64162);
#60654=AXIS2_PLACEMENT_3D('',#79757,#64166,#64167);
#60655=AXIS2_PLACEMENT_3D('',#79763,#64171,#64172);
#60656=AXIS2_PLACEMENT_3D('',#79769,#64176,#64177);
#60657=AXIS2_PLACEMENT_3D('',#79775,#64181,#64182);
#60658=AXIS2_PLACEMENT_3D('',#79781,#64186,#64187);
#60659=AXIS2_PLACEMENT_3D('',#79784,#64190,#64191);
#60660=AXIS2_PLACEMENT_3D('',#79785,#64192,#64193);
#60661=AXIS2_PLACEMENT_3D('',#79786,#64194,#64195);
#60662=AXIS2_PLACEMENT_3D('',#80087,#64216,#64217);
#60663=AXIS2_PLACEMENT_3D('',#80271,#64231,#64232);
#60664=AXIS2_PLACEMENT_3D('',#80382,#64243,#64244);
#60665=AXIS2_PLACEMENT_3D('',#80493,#64255,#64256);
#60666=AXIS2_PLACEMENT_3D('',#80511,#64260,#64261);
#60667=AXIS2_PLACEMENT_3D('',#80512,#64262,#64263);
#60668=AXIS2_PLACEMENT_3D('',#80813,#64284,#64285);
#60669=AXIS2_PLACEMENT_3D('',#80952,#64296,#64297);
#60670=AXIS2_PLACEMENT_3D('',#81093,#64310,#64311);
#60671=AXIS2_PLACEMENT_3D('',#81099,#64315,#64316);
#60672=AXIS2_PLACEMENT_3D('',#81105,#64320,#64321);
#60673=AXIS2_PLACEMENT_3D('',#81108,#64324,#64325);
#60674=AXIS2_PLACEMENT_3D('',#81109,#64326,#64327);
#60675=AXIS2_PLACEMENT_3D('',#81410,#64348,#64349);
#60676=AXIS2_PLACEMENT_3D('',#81411,#64350,#64351);
#60677=AXIS2_PLACEMENT_3D('',#81450,#64358,#64359);
#60678=AXIS2_PLACEMENT_3D('',#81486,#64365,#64366);
#60679=AXIS2_PLACEMENT_3D('',#81492,#64370,#64371);
#60680=AXIS2_PLACEMENT_3D('',#81498,#64375,#64376);
#60681=AXIS2_PLACEMENT_3D('',#81501,#64379,#64380);
#60682=AXIS2_PLACEMENT_3D('',#81502,#64381,#64382);
#60683=AXIS2_PLACEMENT_3D('',#81803,#64403,#64404);
#60684=AXIS2_PLACEMENT_3D('',#81804,#64405,#64406);
#60685=AXIS2_PLACEMENT_3D('',#82105,#64427,#64428);
#60686=AXIS2_PLACEMENT_3D('',#82106,#64429,#64430);
#60687=AXIS2_PLACEMENT_3D('',#82145,#64437,#64438);
#60688=AXIS2_PLACEMENT_3D('',#82181,#64444,#64445);
#60689=AXIS2_PLACEMENT_3D('',#82187,#64449,#64450);
#60690=AXIS2_PLACEMENT_3D('',#82193,#64454,#64455);
#60691=AXIS2_PLACEMENT_3D('',#82196,#64458,#64459);
#60692=AXIS2_PLACEMENT_3D('',#82197,#64460,#64461);
#60693=AXIS2_PLACEMENT_3D('',#82498,#64482,#64483);
#60694=AXIS2_PLACEMENT_3D('',#82637,#64494,#64495);
#60695=AXIS2_PLACEMENT_3D('',#82778,#64508,#64509);
#60696=AXIS2_PLACEMENT_3D('',#82784,#64513,#64514);
#60697=AXIS2_PLACEMENT_3D('',#82790,#64518,#64519);
#60698=AXIS2_PLACEMENT_3D('',#82793,#64522,#64523);
#60699=AXIS2_PLACEMENT_3D('',#82794,#64524,#64525);
#60700=AXIS2_PLACEMENT_3D('',#83095,#64546,#64547);
#60701=AXIS2_PLACEMENT_3D('',#83279,#64561,#64562);
#60702=AXIS2_PLACEMENT_3D('',#83390,#64573,#64574);
#60703=AXIS2_PLACEMENT_3D('',#83501,#64585,#64586);
#60704=AXIS2_PLACEMENT_3D('',#83519,#64590,#64591);
#60705=AXIS2_PLACEMENT_3D('',#83520,#64592,#64593);
#60706=AXIS2_PLACEMENT_3D('',#83821,#64614,#64615);
#60707=AXIS2_PLACEMENT_3D('',#83822,#64616,#64617);
#60708=AXIS2_PLACEMENT_3D('',#83831,#64622,#64623);
#60709=AXIS2_PLACEMENT_3D('',#83837,#64627,#64628);
#60710=AXIS2_PLACEMENT_3D('',#83840,#64631,#64632);
#60711=AXIS2_PLACEMENT_3D('',#83849,#64637,#64638);
#60712=AXIS2_PLACEMENT_3D('',#83855,#64642,#64643);
#60713=AXIS2_PLACEMENT_3D('',#83861,#64647,#64648);
#60714=AXIS2_PLACEMENT_3D('',#83867,#64652,#64653);
#60715=AXIS2_PLACEMENT_3D('',#83873,#64657,#64658);
#60716=AXIS2_PLACEMENT_3D('',#83879,#64662,#64663);
#60717=AXIS2_PLACEMENT_3D('',#83885,#64667,#64668);
#60718=AXIS2_PLACEMENT_3D('',#83891,#64672,#64673);
#60719=AXIS2_PLACEMENT_3D('',#83897,#64677,#64678);
#60720=AXIS2_PLACEMENT_3D('',#83903,#64682,#64683);
#60721=AXIS2_PLACEMENT_3D('',#83906,#64686,#64687);
#60722=AXIS2_PLACEMENT_3D('',#83907,#64688,#64689);
#60723=AXIS2_PLACEMENT_3D('',#83908,#64690,#64691);
#60724=AXIS2_PLACEMENT_3D('',#84209,#64712,#64713);
#60725=AXIS2_PLACEMENT_3D('',#84303,#64721,#64722);
#60726=AXIS2_PLACEMENT_3D('',#84309,#64726,#64727);
#60727=AXIS2_PLACEMENT_3D('',#84315,#64731,#64732);
#60728=AXIS2_PLACEMENT_3D('',#84321,#64736,#64737);
#60729=AXIS2_PLACEMENT_3D('',#84327,#64741,#64742);
#60730=AXIS2_PLACEMENT_3D('',#84333,#64746,#64747);
#60731=AXIS2_PLACEMENT_3D('',#84459,#64759,#64760);
#60732=AXIS2_PLACEMENT_3D('',#84477,#64764,#64765);
#60733=AXIS2_PLACEMENT_3D('',#84478,#64766,#64767);
#60734=AXIS2_PLACEMENT_3D('',#84779,#64788,#64789);
#60735=AXIS2_PLACEMENT_3D('',#85173,#64817,#64818);
#60736=AXIS2_PLACEMENT_3D('',#85191,#64822,#64823);
#60737=AXIS2_PLACEMENT_3D('',#85192,#64824,#64825);
#60738=AXIS2_PLACEMENT_3D('',#85193,#64826,#64827);
#60739=AXIS2_PLACEMENT_3D('',#85494,#64848,#64849);
#60740=AXIS2_PLACEMENT_3D('',#85543,#64854,#64855);
#60741=AXIS2_PLACEMENT_3D('',#85594,#64862,#64863);
#60742=AXIS2_PLACEMENT_3D('',#85600,#64867,#64868);
#60743=AXIS2_PLACEMENT_3D('',#85606,#64872,#64873);
#60744=AXIS2_PLACEMENT_3D('',#85612,#64877,#64878);
#60745=AXIS2_PLACEMENT_3D('',#85615,#64881,#64882);
#60746=AXIS2_PLACEMENT_3D('',#85616,#64883,#64884);
#60747=AXIS2_PLACEMENT_3D('',#85917,#64905,#64906);
#60748=AXIS2_PLACEMENT_3D('',#86413,#64940,#64941);
#60749=AXIS2_PLACEMENT_3D('',#86414,#64942,#64943);
#60750=AXIS2_PLACEMENT_3D('',#86415,#64944,#64945);
#60751=AXIS2_PLACEMENT_3D('',#86416,#64946,#64947);
#60752=AXIS2_PLACEMENT_3D('',#86717,#64968,#64969);
#60753=AXIS2_PLACEMENT_3D('',#87141,#64999,#65000);
#60754=AXIS2_PLACEMENT_3D('',#87159,#65004,#65005);
#60755=AXIS2_PLACEMENT_3D('',#87160,#65006,#65007);
#60756=AXIS2_PLACEMENT_3D('',#87161,#65008,#65009);
#60757=AXIS2_PLACEMENT_3D('',#87162,#65010,#65011);
#60758=AXIS2_PLACEMENT_3D('',#87171,#65016,#65017);
#60759=AXIS2_PLACEMENT_3D('',#87177,#65021,#65022);
#60760=AXIS2_PLACEMENT_3D('',#87183,#65026,#65027);
#60761=AXIS2_PLACEMENT_3D('',#87186,#65030,#65031);
#60762=AXIS2_PLACEMENT_3D('',#87187,#65032,#65033);
#60763=AXIS2_PLACEMENT_3D('',#87196,#65038,#65039);
#60764=AXIS2_PLACEMENT_3D('',#87202,#65043,#65044);
#60765=AXIS2_PLACEMENT_3D('',#87208,#65048,#65049);
#60766=AXIS2_PLACEMENT_3D('',#87211,#65052,#65053);
#60767=AXIS2_PLACEMENT_3D('',#87212,#65054,#65055);
#60768=AXIS2_PLACEMENT_3D('',#87221,#65060,#65061);
#60769=AXIS2_PLACEMENT_3D('',#87227,#65065,#65066);
#60770=AXIS2_PLACEMENT_3D('',#87233,#65070,#65071);
#60771=AXIS2_PLACEMENT_3D('',#87236,#65074,#65075);
#60772=AXIS2_PLACEMENT_3D('',#87237,#65076,#65077);
#60773=AXIS2_PLACEMENT_3D('',#87246,#65082,#65083);
#60774=AXIS2_PLACEMENT_3D('',#87252,#65087,#65088);
#60775=AXIS2_PLACEMENT_3D('',#87258,#65092,#65093);
#60776=AXIS2_PLACEMENT_3D('',#87261,#65096,#65097);
#60777=AXIS2_PLACEMENT_3D('',#87262,#65098,#65099);
#60778=AXIS2_PLACEMENT_3D('',#87271,#65104,#65105);
#60779=AXIS2_PLACEMENT_3D('',#87277,#65109,#65110);
#60780=AXIS2_PLACEMENT_3D('',#87283,#65114,#65115);
#60781=AXIS2_PLACEMENT_3D('',#87286,#65118,#65119);
#60782=AXIS2_PLACEMENT_3D('',#87287,#65120,#65121);
#60783=AXIS2_PLACEMENT_3D('',#87296,#65126,#65127);
#60784=AXIS2_PLACEMENT_3D('',#87302,#65131,#65132);
#60785=AXIS2_PLACEMENT_3D('',#87308,#65136,#65137);
#60786=AXIS2_PLACEMENT_3D('',#87311,#65140,#65141);
#60787=AXIS2_PLACEMENT_3D('',#87312,#65142,#65143);
#60788=AXIS2_PLACEMENT_3D('',#87321,#65148,#65149);
#60789=AXIS2_PLACEMENT_3D('',#87327,#65153,#65154);
#60790=AXIS2_PLACEMENT_3D('',#87333,#65158,#65159);
#60791=AXIS2_PLACEMENT_3D('',#87336,#65162,#65163);
#60792=AXIS2_PLACEMENT_3D('',#87337,#65164,#65165);
#60793=AXIS2_PLACEMENT_3D('',#87346,#65170,#65171);
#60794=AXIS2_PLACEMENT_3D('',#87352,#65175,#65176);
#60795=AXIS2_PLACEMENT_3D('',#87358,#65180,#65181);
#60796=AXIS2_PLACEMENT_3D('',#87361,#65184,#65185);
#60797=AXIS2_PLACEMENT_3D('',#87362,#65186,#65187);
#60798=AXIS2_PLACEMENT_3D('',#87371,#65192,#65193);
#60799=AXIS2_PLACEMENT_3D('',#87377,#65197,#65198);
#60800=AXIS2_PLACEMENT_3D('',#87383,#65202,#65203);
#60801=AXIS2_PLACEMENT_3D('',#87386,#65206,#65207);
#60802=AXIS2_PLACEMENT_3D('',#87387,#65208,#65209);
#60803=AXIS2_PLACEMENT_3D('',#87396,#65214,#65215);
#60804=AXIS2_PLACEMENT_3D('',#87402,#65219,#65220);
#60805=AXIS2_PLACEMENT_3D('',#87408,#65224,#65225);
#60806=AXIS2_PLACEMENT_3D('',#87411,#65228,#65229);
#60807=AXIS2_PLACEMENT_3D('',#87412,#65230,#65231);
#60808=AXIS2_PLACEMENT_3D('',#87421,#65236,#65237);
#60809=AXIS2_PLACEMENT_3D('',#87427,#65241,#65242);
#60810=AXIS2_PLACEMENT_3D('',#87433,#65246,#65247);
#60811=AXIS2_PLACEMENT_3D('',#87436,#65250,#65251);
#60812=AXIS2_PLACEMENT_3D('',#87437,#65252,#65253);
#60813=AXIS2_PLACEMENT_3D('',#87446,#65258,#65259);
#60814=AXIS2_PLACEMENT_3D('',#87452,#65263,#65264);
#60815=AXIS2_PLACEMENT_3D('',#87458,#65268,#65269);
#60816=AXIS2_PLACEMENT_3D('',#87461,#65272,#65273);
#60817=AXIS2_PLACEMENT_3D('',#87462,#65274,#65275);
#60818=AXIS2_PLACEMENT_3D('',#87471,#65280,#65281);
#60819=AXIS2_PLACEMENT_3D('',#87477,#65285,#65286);
#60820=AXIS2_PLACEMENT_3D('',#87483,#65290,#65291);
#60821=AXIS2_PLACEMENT_3D('',#87486,#65294,#65295);
#60822=AXIS2_PLACEMENT_3D('',#87487,#65296,#65297);
#60823=AXIS2_PLACEMENT_3D('',#87496,#65302,#65303);
#60824=AXIS2_PLACEMENT_3D('',#87502,#65307,#65308);
#60825=AXIS2_PLACEMENT_3D('',#87508,#65312,#65313);
#60826=AXIS2_PLACEMENT_3D('',#87511,#65316,#65317);
#60827=AXIS2_PLACEMENT_3D('',#87512,#65318,#65319);
#60828=AXIS2_PLACEMENT_3D('',#87521,#65324,#65325);
#60829=AXIS2_PLACEMENT_3D('',#87527,#65329,#65330);
#60830=AXIS2_PLACEMENT_3D('',#87533,#65334,#65335);
#60831=AXIS2_PLACEMENT_3D('',#87536,#65338,#65339);
#60832=AXIS2_PLACEMENT_3D('',#87537,#65340,#65341);
#60833=AXIS2_PLACEMENT_3D('',#87546,#65346,#65347);
#60834=AXIS2_PLACEMENT_3D('',#87552,#65351,#65352);
#60835=AXIS2_PLACEMENT_3D('',#87558,#65356,#65357);
#60836=AXIS2_PLACEMENT_3D('',#87561,#65360,#65361);
#60837=AXIS2_PLACEMENT_3D('',#87562,#65362,#65363);
#60838=AXIS2_PLACEMENT_3D('',#87571,#65368,#65369);
#60839=AXIS2_PLACEMENT_3D('',#87577,#65373,#65374);
#60840=AXIS2_PLACEMENT_3D('',#87583,#65378,#65379);
#60841=AXIS2_PLACEMENT_3D('',#87586,#65382,#65383);
#60842=AXIS2_PLACEMENT_3D('',#87587,#65384,#65385);
#60843=AXIS2_PLACEMENT_3D('',#87596,#65390,#65391);
#60844=AXIS2_PLACEMENT_3D('',#87602,#65395,#65396);
#60845=AXIS2_PLACEMENT_3D('',#87608,#65400,#65401);
#60846=AXIS2_PLACEMENT_3D('',#87611,#65404,#65405);
#60847=AXIS2_PLACEMENT_3D('',#87612,#65406,#65407);
#60848=AXIS2_PLACEMENT_3D('',#87621,#65412,#65413);
#60849=AXIS2_PLACEMENT_3D('',#87627,#65417,#65418);
#60850=AXIS2_PLACEMENT_3D('',#87633,#65422,#65423);
#60851=AXIS2_PLACEMENT_3D('',#87636,#65426,#65427);
#60852=AXIS2_PLACEMENT_3D('',#87637,#65428,#65429);
#60853=AXIS2_PLACEMENT_3D('',#87646,#65434,#65435);
#60854=AXIS2_PLACEMENT_3D('',#87652,#65439,#65440);
#60855=AXIS2_PLACEMENT_3D('',#87658,#65444,#65445);
#60856=AXIS2_PLACEMENT_3D('',#87661,#65448,#65449);
#60857=AXIS2_PLACEMENT_3D('',#87662,#65450,#65451);
#60858=AXIS2_PLACEMENT_3D('',#87671,#65456,#65457);
#60859=AXIS2_PLACEMENT_3D('',#87677,#65461,#65462);
#60860=AXIS2_PLACEMENT_3D('',#87683,#65466,#65467);
#60861=AXIS2_PLACEMENT_3D('',#87686,#65470,#65471);
#60862=AXIS2_PLACEMENT_3D('',#87687,#65472,#65473);
#60863=AXIS2_PLACEMENT_3D('',#87696,#65478,#65479);
#60864=AXIS2_PLACEMENT_3D('',#87702,#65483,#65484);
#60865=AXIS2_PLACEMENT_3D('',#87708,#65488,#65489);
#60866=AXIS2_PLACEMENT_3D('',#87711,#65492,#65493);
#60867=AXIS2_PLACEMENT_3D('',#87712,#65494,#65495);
#60868=AXIS2_PLACEMENT_3D('',#87721,#65500,#65501);
#60869=AXIS2_PLACEMENT_3D('',#87727,#65505,#65506);
#60870=AXIS2_PLACEMENT_3D('',#87733,#65510,#65511);
#60871=AXIS2_PLACEMENT_3D('',#87736,#65514,#65515);
#60872=AXIS2_PLACEMENT_3D('',#87737,#65516,#65517);
#60873=AXIS2_PLACEMENT_3D('',#87746,#65522,#65523);
#60874=AXIS2_PLACEMENT_3D('',#87752,#65527,#65528);
#60875=AXIS2_PLACEMENT_3D('',#87758,#65532,#65533);
#60876=AXIS2_PLACEMENT_3D('',#87761,#65536,#65537);
#60877=AXIS2_PLACEMENT_3D('',#87762,#65538,#65539);
#60878=AXIS2_PLACEMENT_3D('',#87771,#65544,#65545);
#60879=AXIS2_PLACEMENT_3D('',#87777,#65549,#65550);
#60880=AXIS2_PLACEMENT_3D('',#87783,#65554,#65555);
#60881=AXIS2_PLACEMENT_3D('',#87786,#65558,#65559);
#60882=AXIS2_PLACEMENT_3D('',#87787,#65560,#65561);
#60883=AXIS2_PLACEMENT_3D('',#87796,#65566,#65567);
#60884=AXIS2_PLACEMENT_3D('',#87802,#65571,#65572);
#60885=AXIS2_PLACEMENT_3D('',#87808,#65576,#65577);
#60886=AXIS2_PLACEMENT_3D('',#87811,#65580,#65581);
#60887=AXIS2_PLACEMENT_3D('',#87812,#65582,#65583);
#60888=AXIS2_PLACEMENT_3D('',#87821,#65588,#65589);
#60889=AXIS2_PLACEMENT_3D('',#87827,#65593,#65594);
#60890=AXIS2_PLACEMENT_3D('',#87833,#65598,#65599);
#60891=AXIS2_PLACEMENT_3D('',#87836,#65602,#65603);
#60892=AXIS2_PLACEMENT_3D('',#87837,#65604,#65605);
#60893=AXIS2_PLACEMENT_3D('',#87846,#65610,#65611);
#60894=AXIS2_PLACEMENT_3D('',#87852,#65615,#65616);
#60895=AXIS2_PLACEMENT_3D('',#87858,#65620,#65621);
#60896=AXIS2_PLACEMENT_3D('',#87861,#65624,#65625);
#60897=AXIS2_PLACEMENT_3D('',#87862,#65626,#65627);
#60898=AXIS2_PLACEMENT_3D('',#87871,#65632,#65633);
#60899=AXIS2_PLACEMENT_3D('',#87877,#65637,#65638);
#60900=AXIS2_PLACEMENT_3D('',#87883,#65642,#65643);
#60901=AXIS2_PLACEMENT_3D('',#87886,#65646,#65647);
#60902=AXIS2_PLACEMENT_3D('',#87887,#65648,#65649);
#60903=AXIS2_PLACEMENT_3D('',#87896,#65654,#65655);
#60904=AXIS2_PLACEMENT_3D('',#87902,#65659,#65660);
#60905=AXIS2_PLACEMENT_3D('',#87908,#65664,#65665);
#60906=AXIS2_PLACEMENT_3D('',#87911,#65668,#65669);
#60907=AXIS2_PLACEMENT_3D('',#87912,#65670,#65671);
#60908=AXIS2_PLACEMENT_3D('',#87921,#65676,#65677);
#60909=AXIS2_PLACEMENT_3D('',#87927,#65681,#65682);
#60910=AXIS2_PLACEMENT_3D('',#87933,#65686,#65687);
#60911=AXIS2_PLACEMENT_3D('',#87936,#65690,#65691);
#60912=AXIS2_PLACEMENT_3D('',#87937,#65692,#65693);
#60913=AXIS2_PLACEMENT_3D('',#87946,#65698,#65699);
#60914=AXIS2_PLACEMENT_3D('',#87952,#65703,#65704);
#60915=AXIS2_PLACEMENT_3D('',#87958,#65708,#65709);
#60916=AXIS2_PLACEMENT_3D('',#87961,#65712,#65713);
#60917=AXIS2_PLACEMENT_3D('',#87962,#65714,#65715);
#60918=AXIS2_PLACEMENT_3D('',#87971,#65720,#65721);
#60919=AXIS2_PLACEMENT_3D('',#87977,#65725,#65726);
#60920=AXIS2_PLACEMENT_3D('',#87983,#65730,#65731);
#60921=AXIS2_PLACEMENT_3D('',#87986,#65734,#65735);
#60922=AXIS2_PLACEMENT_3D('',#87987,#65736,#65737);
#60923=AXIS2_PLACEMENT_3D('',#87996,#65742,#65743);
#60924=AXIS2_PLACEMENT_3D('',#88002,#65747,#65748);
#60925=AXIS2_PLACEMENT_3D('',#88008,#65752,#65753);
#60926=AXIS2_PLACEMENT_3D('',#88011,#65756,#65757);
#60927=AXIS2_PLACEMENT_3D('',#88012,#65758,#65759);
#60928=AXIS2_PLACEMENT_3D('',#88021,#65764,#65765);
#60929=AXIS2_PLACEMENT_3D('',#88027,#65769,#65770);
#60930=AXIS2_PLACEMENT_3D('',#88033,#65774,#65775);
#60931=AXIS2_PLACEMENT_3D('',#88036,#65778,#65779);
#60932=AXIS2_PLACEMENT_3D('',#88037,#65780,#65781);
#60933=AXIS2_PLACEMENT_3D('',#88046,#65786,#65787);
#60934=AXIS2_PLACEMENT_3D('',#88052,#65791,#65792);
#60935=AXIS2_PLACEMENT_3D('',#88058,#65796,#65797);
#60936=AXIS2_PLACEMENT_3D('',#88061,#65800,#65801);
#60937=AXIS2_PLACEMENT_3D('',#88062,#65802,#65803);
#60938=AXIS2_PLACEMENT_3D('',#88071,#65808,#65809);
#60939=AXIS2_PLACEMENT_3D('',#88077,#65813,#65814);
#60940=AXIS2_PLACEMENT_3D('',#88083,#65818,#65819);
#60941=AXIS2_PLACEMENT_3D('',#88086,#65822,#65823);
#60942=AXIS2_PLACEMENT_3D('',#88087,#65824,#65825);
#60943=AXIS2_PLACEMENT_3D('',#88096,#65830,#65831);
#60944=AXIS2_PLACEMENT_3D('',#88102,#65835,#65836);
#60945=AXIS2_PLACEMENT_3D('',#88108,#65840,#65841);
#60946=AXIS2_PLACEMENT_3D('',#88111,#65844,#65845);
#60947=AXIS2_PLACEMENT_3D('',#88112,#65846,#65847);
#60948=AXIS2_PLACEMENT_3D('',#88121,#65852,#65853);
#60949=AXIS2_PLACEMENT_3D('',#88127,#65857,#65858);
#60950=AXIS2_PLACEMENT_3D('',#88133,#65862,#65863);
#60951=AXIS2_PLACEMENT_3D('',#88136,#65866,#65867);
#60952=AXIS2_PLACEMENT_3D('',#88137,#65868,#65869);
#60953=AXIS2_PLACEMENT_3D('',#88146,#65874,#65875);
#60954=AXIS2_PLACEMENT_3D('',#88152,#65879,#65880);
#60955=AXIS2_PLACEMENT_3D('',#88158,#65884,#65885);
#60956=AXIS2_PLACEMENT_3D('',#88161,#65888,#65889);
#60957=AXIS2_PLACEMENT_3D('',#88162,#65890,#65891);
#60958=AXIS2_PLACEMENT_3D('',#88171,#65896,#65897);
#60959=AXIS2_PLACEMENT_3D('',#88177,#65901,#65902);
#60960=AXIS2_PLACEMENT_3D('',#88183,#65906,#65907);
#60961=AXIS2_PLACEMENT_3D('',#88186,#65910,#65911);
#60962=AXIS2_PLACEMENT_3D('',#88187,#65912,#65913);
#60963=AXIS2_PLACEMENT_3D('',#88196,#65918,#65919);
#60964=AXIS2_PLACEMENT_3D('',#88202,#65923,#65924);
#60965=AXIS2_PLACEMENT_3D('',#88208,#65928,#65929);
#60966=AXIS2_PLACEMENT_3D('',#88211,#65932,#65933);
#60967=AXIS2_PLACEMENT_3D('',#88212,#65934,#65935);
#60968=AXIS2_PLACEMENT_3D('',#88221,#65940,#65941);
#60969=AXIS2_PLACEMENT_3D('',#88227,#65945,#65946);
#60970=AXIS2_PLACEMENT_3D('',#88233,#65950,#65951);
#60971=AXIS2_PLACEMENT_3D('',#88236,#65954,#65955);
#60972=AXIS2_PLACEMENT_3D('',#88237,#65956,#65957);
#60973=AXIS2_PLACEMENT_3D('',#88246,#65962,#65963);
#60974=AXIS2_PLACEMENT_3D('',#88252,#65967,#65968);
#60975=AXIS2_PLACEMENT_3D('',#88258,#65972,#65973);
#60976=AXIS2_PLACEMENT_3D('',#88261,#65976,#65977);
#60977=AXIS2_PLACEMENT_3D('',#88262,#65978,#65979);
#60978=AXIS2_PLACEMENT_3D('',#88271,#65984,#65985);
#60979=AXIS2_PLACEMENT_3D('',#88277,#65989,#65990);
#60980=AXIS2_PLACEMENT_3D('',#88283,#65994,#65995);
#60981=AXIS2_PLACEMENT_3D('',#88286,#65998,#65999);
#60982=AXIS2_PLACEMENT_3D('',#88287,#66000,#66001);
#60983=AXIS2_PLACEMENT_3D('',#88296,#66006,#66007);
#60984=AXIS2_PLACEMENT_3D('',#88302,#66011,#66012);
#60985=AXIS2_PLACEMENT_3D('',#88308,#66016,#66017);
#60986=AXIS2_PLACEMENT_3D('',#88311,#66020,#66021);
#60987=AXIS2_PLACEMENT_3D('',#88312,#66022,#66023);
#60988=AXIS2_PLACEMENT_3D('',#88321,#66028,#66029);
#60989=AXIS2_PLACEMENT_3D('',#88327,#66033,#66034);
#60990=AXIS2_PLACEMENT_3D('',#88333,#66038,#66039);
#60991=AXIS2_PLACEMENT_3D('',#88336,#66042,#66043);
#60992=AXIS2_PLACEMENT_3D('',#88337,#66044,#66045);
#60993=AXIS2_PLACEMENT_3D('',#88346,#66050,#66051);
#60994=AXIS2_PLACEMENT_3D('',#88352,#66055,#66056);
#60995=AXIS2_PLACEMENT_3D('',#88358,#66060,#66061);
#60996=AXIS2_PLACEMENT_3D('',#88361,#66064,#66065);
#60997=AXIS2_PLACEMENT_3D('',#88362,#66066,#66067);
#60998=AXIS2_PLACEMENT_3D('',#88371,#66072,#66073);
#60999=AXIS2_PLACEMENT_3D('',#88377,#66077,#66078);
#61000=AXIS2_PLACEMENT_3D('',#88383,#66082,#66083);
#61001=AXIS2_PLACEMENT_3D('',#88386,#66086,#66087);
#61002=AXIS2_PLACEMENT_3D('',#88387,#66088,#66089);
#61003=AXIS2_PLACEMENT_3D('',#88396,#66094,#66095);
#61004=AXIS2_PLACEMENT_3D('',#88402,#66099,#66100);
#61005=AXIS2_PLACEMENT_3D('',#88408,#66104,#66105);
#61006=AXIS2_PLACEMENT_3D('',#88411,#66108,#66109);
#61007=AXIS2_PLACEMENT_3D('',#88412,#66110,#66111);
#61008=AXIS2_PLACEMENT_3D('',#88421,#66116,#66117);
#61009=AXIS2_PLACEMENT_3D('',#88427,#66121,#66122);
#61010=AXIS2_PLACEMENT_3D('',#88433,#66126,#66127);
#61011=AXIS2_PLACEMENT_3D('',#88436,#66130,#66131);
#61012=AXIS2_PLACEMENT_3D('',#88437,#66132,#66133);
#61013=AXIS2_PLACEMENT_3D('',#88446,#66138,#66139);
#61014=AXIS2_PLACEMENT_3D('',#88452,#66143,#66144);
#61015=AXIS2_PLACEMENT_3D('',#88458,#66148,#66149);
#61016=AXIS2_PLACEMENT_3D('',#88461,#66152,#66153);
#61017=AXIS2_PLACEMENT_3D('',#88462,#66154,#66155);
#61018=AXIS2_PLACEMENT_3D('',#88471,#66160,#66161);
#61019=AXIS2_PLACEMENT_3D('',#88477,#66165,#66166);
#61020=AXIS2_PLACEMENT_3D('',#88483,#66170,#66171);
#61021=AXIS2_PLACEMENT_3D('',#88486,#66174,#66175);
#61022=AXIS2_PLACEMENT_3D('',#88487,#66176,#66177);
#61023=AXIS2_PLACEMENT_3D('',#88496,#66182,#66183);
#61024=AXIS2_PLACEMENT_3D('',#88502,#66187,#66188);
#61025=AXIS2_PLACEMENT_3D('',#88508,#66192,#66193);
#61026=AXIS2_PLACEMENT_3D('',#88511,#66196,#66197);
#61027=AXIS2_PLACEMENT_3D('',#88512,#66198,#66199);
#61028=AXIS2_PLACEMENT_3D('',#88521,#66204,#66205);
#61029=AXIS2_PLACEMENT_3D('',#88527,#66209,#66210);
#61030=AXIS2_PLACEMENT_3D('',#88533,#66214,#66215);
#61031=AXIS2_PLACEMENT_3D('',#88536,#66218,#66219);
#61032=AXIS2_PLACEMENT_3D('',#88537,#66220,#66221);
#61033=AXIS2_PLACEMENT_3D('',#88546,#66226,#66227);
#61034=AXIS2_PLACEMENT_3D('',#88552,#66231,#66232);
#61035=AXIS2_PLACEMENT_3D('',#88558,#66236,#66237);
#61036=AXIS2_PLACEMENT_3D('',#88561,#66240,#66241);
#61037=AXIS2_PLACEMENT_3D('',#88562,#66242,#66243);
#61038=AXIS2_PLACEMENT_3D('',#88571,#66248,#66249);
#61039=AXIS2_PLACEMENT_3D('',#88577,#66253,#66254);
#61040=AXIS2_PLACEMENT_3D('',#88583,#66258,#66259);
#61041=AXIS2_PLACEMENT_3D('',#88586,#66262,#66263);
#61042=AXIS2_PLACEMENT_3D('',#88587,#66264,#66265);
#61043=AXIS2_PLACEMENT_3D('',#88596,#66270,#66271);
#61044=AXIS2_PLACEMENT_3D('',#88602,#66275,#66276);
#61045=AXIS2_PLACEMENT_3D('',#88608,#66280,#66281);
#61046=AXIS2_PLACEMENT_3D('',#88611,#66284,#66285);
#61047=AXIS2_PLACEMENT_3D('',#88612,#66286,#66287);
#61048=AXIS2_PLACEMENT_3D('',#88621,#66292,#66293);
#61049=AXIS2_PLACEMENT_3D('',#88627,#66297,#66298);
#61050=AXIS2_PLACEMENT_3D('',#88633,#66302,#66303);
#61051=AXIS2_PLACEMENT_3D('',#88636,#66306,#66307);
#61052=AXIS2_PLACEMENT_3D('',#88637,#66308,#66309);
#61053=AXIS2_PLACEMENT_3D('',#88646,#66314,#66315);
#61054=AXIS2_PLACEMENT_3D('',#88652,#66319,#66320);
#61055=AXIS2_PLACEMENT_3D('',#88658,#66324,#66325);
#61056=AXIS2_PLACEMENT_3D('',#88661,#66328,#66329);
#61057=AXIS2_PLACEMENT_3D('',#88662,#66330,#66331);
#61058=AXIS2_PLACEMENT_3D('',#88671,#66336,#66337);
#61059=AXIS2_PLACEMENT_3D('',#88677,#66341,#66342);
#61060=AXIS2_PLACEMENT_3D('',#88683,#66346,#66347);
#61061=AXIS2_PLACEMENT_3D('',#88686,#66350,#66351);
#61062=AXIS2_PLACEMENT_3D('',#88687,#66352,#66353);
#61063=AXIS2_PLACEMENT_3D('',#88696,#66358,#66359);
#61064=AXIS2_PLACEMENT_3D('',#88702,#66363,#66364);
#61065=AXIS2_PLACEMENT_3D('',#88708,#66368,#66369);
#61066=AXIS2_PLACEMENT_3D('',#88711,#66372,#66373);
#61067=AXIS2_PLACEMENT_3D('',#88712,#66374,#66375);
#61068=AXIS2_PLACEMENT_3D('',#88721,#66380,#66381);
#61069=AXIS2_PLACEMENT_3D('',#88727,#66385,#66386);
#61070=AXIS2_PLACEMENT_3D('',#88733,#66390,#66391);
#61071=AXIS2_PLACEMENT_3D('',#88736,#66394,#66395);
#61072=AXIS2_PLACEMENT_3D('',#88737,#66396,#66397);
#61073=AXIS2_PLACEMENT_3D('',#88746,#66402,#66403);
#61074=AXIS2_PLACEMENT_3D('',#88752,#66407,#66408);
#61075=AXIS2_PLACEMENT_3D('',#88758,#66412,#66413);
#61076=AXIS2_PLACEMENT_3D('',#88761,#66416,#66417);
#61077=AXIS2_PLACEMENT_3D('',#88762,#66418,#66419);
#61078=AXIS2_PLACEMENT_3D('',#88771,#66424,#66425);
#61079=AXIS2_PLACEMENT_3D('',#88777,#66429,#66430);
#61080=AXIS2_PLACEMENT_3D('',#88783,#66434,#66435);
#61081=AXIS2_PLACEMENT_3D('',#88786,#66438,#66439);
#61082=AXIS2_PLACEMENT_3D('',#88787,#66440,#66441);
#61083=AXIS2_PLACEMENT_3D('',#88796,#66446,#66447);
#61084=AXIS2_PLACEMENT_3D('',#88802,#66451,#66452);
#61085=AXIS2_PLACEMENT_3D('',#88808,#66456,#66457);
#61086=AXIS2_PLACEMENT_3D('',#88811,#66460,#66461);
#61087=AXIS2_PLACEMENT_3D('',#88812,#66462,#66463);
#61088=AXIS2_PLACEMENT_3D('',#88821,#66468,#66469);
#61089=AXIS2_PLACEMENT_3D('',#88827,#66473,#66474);
#61090=AXIS2_PLACEMENT_3D('',#88833,#66478,#66479);
#61091=AXIS2_PLACEMENT_3D('',#88836,#66482,#66483);
#61092=AXIS2_PLACEMENT_3D('',#88837,#66484,#66485);
#61093=AXIS2_PLACEMENT_3D('',#88846,#66490,#66491);
#61094=AXIS2_PLACEMENT_3D('',#88852,#66495,#66496);
#61095=AXIS2_PLACEMENT_3D('',#88858,#66500,#66501);
#61096=AXIS2_PLACEMENT_3D('',#88861,#66504,#66505);
#61097=AXIS2_PLACEMENT_3D('',#88862,#66506,#66507);
#61098=AXIS2_PLACEMENT_3D('',#88871,#66512,#66513);
#61099=AXIS2_PLACEMENT_3D('',#88877,#66517,#66518);
#61100=AXIS2_PLACEMENT_3D('',#88883,#66522,#66523);
#61101=AXIS2_PLACEMENT_3D('',#88886,#66526,#66527);
#61102=AXIS2_PLACEMENT_3D('',#88887,#66528,#66529);
#61103=AXIS2_PLACEMENT_3D('',#88896,#66534,#66535);
#61104=AXIS2_PLACEMENT_3D('',#88902,#66539,#66540);
#61105=AXIS2_PLACEMENT_3D('',#88908,#66544,#66545);
#61106=AXIS2_PLACEMENT_3D('',#88911,#66548,#66549);
#61107=AXIS2_PLACEMENT_3D('',#88912,#66550,#66551);
#61108=AXIS2_PLACEMENT_3D('',#88921,#66556,#66557);
#61109=AXIS2_PLACEMENT_3D('',#88927,#66561,#66562);
#61110=AXIS2_PLACEMENT_3D('',#88933,#66566,#66567);
#61111=AXIS2_PLACEMENT_3D('',#88936,#66570,#66571);
#61112=AXIS2_PLACEMENT_3D('',#88937,#66572,#66573);
#61113=AXIS2_PLACEMENT_3D('',#88946,#66578,#66579);
#61114=AXIS2_PLACEMENT_3D('',#88952,#66583,#66584);
#61115=AXIS2_PLACEMENT_3D('',#88958,#66588,#66589);
#61116=AXIS2_PLACEMENT_3D('',#88961,#66592,#66593);
#61117=AXIS2_PLACEMENT_3D('',#88962,#66594,#66595);
#61118=AXIS2_PLACEMENT_3D('',#88971,#66600,#66601);
#61119=AXIS2_PLACEMENT_3D('',#88977,#66605,#66606);
#61120=AXIS2_PLACEMENT_3D('',#88983,#66610,#66611);
#61121=AXIS2_PLACEMENT_3D('',#88986,#66614,#66615);
#61122=AXIS2_PLACEMENT_3D('',#88987,#66616,#66617);
#61123=AXIS2_PLACEMENT_3D('',#88996,#66622,#66623);
#61124=AXIS2_PLACEMENT_3D('',#89002,#66627,#66628);
#61125=AXIS2_PLACEMENT_3D('',#89008,#66632,#66633);
#61126=AXIS2_PLACEMENT_3D('',#89011,#66636,#66637);
#61127=AXIS2_PLACEMENT_3D('',#89012,#66638,#66639);
#61128=AXIS2_PLACEMENT_3D('',#89021,#66644,#66645);
#61129=AXIS2_PLACEMENT_3D('',#89027,#66649,#66650);
#61130=AXIS2_PLACEMENT_3D('',#89033,#66654,#66655);
#61131=AXIS2_PLACEMENT_3D('',#89036,#66658,#66659);
#61132=AXIS2_PLACEMENT_3D('',#89037,#66660,#66661);
#61133=AXIS2_PLACEMENT_3D('',#89046,#66666,#66667);
#61134=AXIS2_PLACEMENT_3D('',#89052,#66671,#66672);
#61135=AXIS2_PLACEMENT_3D('',#89058,#66676,#66677);
#61136=AXIS2_PLACEMENT_3D('',#89061,#66680,#66681);
#61137=AXIS2_PLACEMENT_3D('',#89062,#66682,#66683);
#61138=AXIS2_PLACEMENT_3D('',#89071,#66688,#66689);
#61139=AXIS2_PLACEMENT_3D('',#89077,#66693,#66694);
#61140=AXIS2_PLACEMENT_3D('',#89083,#66698,#66699);
#61141=AXIS2_PLACEMENT_3D('',#89086,#66702,#66703);
#61142=AXIS2_PLACEMENT_3D('',#89087,#66704,#66705);
#61143=AXIS2_PLACEMENT_3D('',#89096,#66710,#66711);
#61144=AXIS2_PLACEMENT_3D('',#89102,#66715,#66716);
#61145=AXIS2_PLACEMENT_3D('',#89108,#66720,#66721);
#61146=AXIS2_PLACEMENT_3D('',#89111,#66724,#66725);
#61147=AXIS2_PLACEMENT_3D('',#89112,#66726,#66727);
#61148=AXIS2_PLACEMENT_3D('',#89121,#66732,#66733);
#61149=AXIS2_PLACEMENT_3D('',#89127,#66737,#66738);
#61150=AXIS2_PLACEMENT_3D('',#89133,#66742,#66743);
#61151=AXIS2_PLACEMENT_3D('',#89136,#66746,#66747);
#61152=AXIS2_PLACEMENT_3D('',#89137,#66748,#66749);
#61153=AXIS2_PLACEMENT_3D('',#89146,#66754,#66755);
#61154=AXIS2_PLACEMENT_3D('',#89152,#66759,#66760);
#61155=AXIS2_PLACEMENT_3D('',#89158,#66764,#66765);
#61156=AXIS2_PLACEMENT_3D('',#89161,#66768,#66769);
#61157=AXIS2_PLACEMENT_3D('',#89162,#66770,#66771);
#61158=AXIS2_PLACEMENT_3D('',#89171,#66776,#66777);
#61159=AXIS2_PLACEMENT_3D('',#89177,#66781,#66782);
#61160=AXIS2_PLACEMENT_3D('',#89183,#66786,#66787);
#61161=AXIS2_PLACEMENT_3D('',#89186,#66790,#66791);
#61162=AXIS2_PLACEMENT_3D('',#89187,#66792,#66793);
#61163=AXIS2_PLACEMENT_3D('',#89196,#66798,#66799);
#61164=AXIS2_PLACEMENT_3D('',#89202,#66803,#66804);
#61165=AXIS2_PLACEMENT_3D('',#89208,#66808,#66809);
#61166=AXIS2_PLACEMENT_3D('',#89211,#66812,#66813);
#61167=AXIS2_PLACEMENT_3D('',#89212,#66814,#66815);
#61168=AXIS2_PLACEMENT_3D('',#89221,#66820,#66821);
#61169=AXIS2_PLACEMENT_3D('',#89227,#66825,#66826);
#61170=AXIS2_PLACEMENT_3D('',#89233,#66830,#66831);
#61171=AXIS2_PLACEMENT_3D('',#89236,#66834,#66835);
#61172=AXIS2_PLACEMENT_3D('',#89237,#66836,#66837);
#61173=AXIS2_PLACEMENT_3D('',#89246,#66842,#66843);
#61174=AXIS2_PLACEMENT_3D('',#89252,#66847,#66848);
#61175=AXIS2_PLACEMENT_3D('',#89258,#66852,#66853);
#61176=AXIS2_PLACEMENT_3D('',#89261,#66856,#66857);
#61177=AXIS2_PLACEMENT_3D('',#89262,#66858,#66859);
#61178=AXIS2_PLACEMENT_3D('',#89271,#66864,#66865);
#61179=AXIS2_PLACEMENT_3D('',#89277,#66869,#66870);
#61180=AXIS2_PLACEMENT_3D('',#89283,#66874,#66875);
#61181=AXIS2_PLACEMENT_3D('',#89286,#66878,#66879);
#61182=AXIS2_PLACEMENT_3D('',#89287,#66880,#66881);
#61183=AXIS2_PLACEMENT_3D('',#89296,#66886,#66887);
#61184=AXIS2_PLACEMENT_3D('',#89302,#66891,#66892);
#61185=AXIS2_PLACEMENT_3D('',#89308,#66896,#66897);
#61186=AXIS2_PLACEMENT_3D('',#89311,#66900,#66901);
#61187=AXIS2_PLACEMENT_3D('',#89312,#66902,#66903);
#61188=AXIS2_PLACEMENT_3D('',#89321,#66908,#66909);
#61189=AXIS2_PLACEMENT_3D('',#89327,#66913,#66914);
#61190=AXIS2_PLACEMENT_3D('',#89333,#66918,#66919);
#61191=AXIS2_PLACEMENT_3D('',#89336,#66922,#66923);
#61192=AXIS2_PLACEMENT_3D('',#89337,#66924,#66925);
#61193=AXIS2_PLACEMENT_3D('',#89346,#66930,#66931);
#61194=AXIS2_PLACEMENT_3D('',#89352,#66935,#66936);
#61195=AXIS2_PLACEMENT_3D('',#89358,#66940,#66941);
#61196=AXIS2_PLACEMENT_3D('',#89361,#66944,#66945);
#61197=AXIS2_PLACEMENT_3D('',#89362,#66946,#66947);
#61198=AXIS2_PLACEMENT_3D('',#89371,#66952,#66953);
#61199=AXIS2_PLACEMENT_3D('',#89377,#66957,#66958);
#61200=AXIS2_PLACEMENT_3D('',#89383,#66962,#66963);
#61201=AXIS2_PLACEMENT_3D('',#89386,#66966,#66967);
#61202=AXIS2_PLACEMENT_3D('',#89387,#66968,#66969);
#61203=AXIS2_PLACEMENT_3D('',#89396,#66974,#66975);
#61204=AXIS2_PLACEMENT_3D('',#89402,#66979,#66980);
#61205=AXIS2_PLACEMENT_3D('',#89408,#66984,#66985);
#61206=AXIS2_PLACEMENT_3D('',#89411,#66988,#66989);
#61207=AXIS2_PLACEMENT_3D('',#89412,#66990,#66991);
#61208=AXIS2_PLACEMENT_3D('',#89421,#66996,#66997);
#61209=AXIS2_PLACEMENT_3D('',#89427,#67001,#67002);
#61210=AXIS2_PLACEMENT_3D('',#89433,#67006,#67007);
#61211=AXIS2_PLACEMENT_3D('',#89436,#67010,#67011);
#61212=AXIS2_PLACEMENT_3D('',#89437,#67012,#67013);
#61213=AXIS2_PLACEMENT_3D('',#89446,#67018,#67019);
#61214=AXIS2_PLACEMENT_3D('',#89452,#67023,#67024);
#61215=AXIS2_PLACEMENT_3D('',#89458,#67028,#67029);
#61216=AXIS2_PLACEMENT_3D('',#89461,#67032,#67033);
#61217=AXIS2_PLACEMENT_3D('',#89462,#67034,#67035);
#61218=AXIS2_PLACEMENT_3D('',#89471,#67040,#67041);
#61219=AXIS2_PLACEMENT_3D('',#89477,#67045,#67046);
#61220=AXIS2_PLACEMENT_3D('',#89483,#67050,#67051);
#61221=AXIS2_PLACEMENT_3D('',#89486,#67054,#67055);
#61222=AXIS2_PLACEMENT_3D('',#89487,#67056,#67057);
#61223=AXIS2_PLACEMENT_3D('',#89496,#67062,#67063);
#61224=AXIS2_PLACEMENT_3D('',#89502,#67067,#67068);
#61225=AXIS2_PLACEMENT_3D('',#89508,#67072,#67073);
#61226=AXIS2_PLACEMENT_3D('',#89511,#67076,#67077);
#61227=AXIS2_PLACEMENT_3D('',#89512,#67078,#67079);
#61228=AXIS2_PLACEMENT_3D('',#89521,#67084,#67085);
#61229=AXIS2_PLACEMENT_3D('',#89527,#67089,#67090);
#61230=AXIS2_PLACEMENT_3D('',#89533,#67094,#67095);
#61231=AXIS2_PLACEMENT_3D('',#89536,#67098,#67099);
#61232=AXIS2_PLACEMENT_3D('',#89537,#67100,#67101);
#61233=AXIS2_PLACEMENT_3D('',#89546,#67106,#67107);
#61234=AXIS2_PLACEMENT_3D('',#89552,#67111,#67112);
#61235=AXIS2_PLACEMENT_3D('',#89558,#67116,#67117);
#61236=AXIS2_PLACEMENT_3D('',#89561,#67120,#67121);
#61237=AXIS2_PLACEMENT_3D('',#89562,#67122,#67123);
#61238=AXIS2_PLACEMENT_3D('',#89571,#67128,#67129);
#61239=AXIS2_PLACEMENT_3D('',#89577,#67133,#67134);
#61240=AXIS2_PLACEMENT_3D('',#89583,#67138,#67139);
#61241=AXIS2_PLACEMENT_3D('',#89586,#67142,#67143);
#61242=AXIS2_PLACEMENT_3D('',#89587,#67144,#67145);
#61243=AXIS2_PLACEMENT_3D('',#89596,#67150,#67151);
#61244=AXIS2_PLACEMENT_3D('',#89602,#67155,#67156);
#61245=AXIS2_PLACEMENT_3D('',#89608,#67160,#67161);
#61246=AXIS2_PLACEMENT_3D('',#89611,#67164,#67165);
#61247=AXIS2_PLACEMENT_3D('',#89612,#67166,#67167);
#61248=AXIS2_PLACEMENT_3D('',#89621,#67172,#67173);
#61249=AXIS2_PLACEMENT_3D('',#89627,#67177,#67178);
#61250=AXIS2_PLACEMENT_3D('',#89633,#67182,#67183);
#61251=AXIS2_PLACEMENT_3D('',#89636,#67186,#67187);
#61252=AXIS2_PLACEMENT_3D('',#89637,#67188,#67189);
#61253=AXIS2_PLACEMENT_3D('',#89646,#67194,#67195);
#61254=AXIS2_PLACEMENT_3D('',#89652,#67199,#67200);
#61255=AXIS2_PLACEMENT_3D('',#89658,#67204,#67205);
#61256=AXIS2_PLACEMENT_3D('',#89661,#67208,#67209);
#61257=AXIS2_PLACEMENT_3D('',#89662,#67210,#67211);
#61258=AXIS2_PLACEMENT_3D('',#89671,#67216,#67217);
#61259=AXIS2_PLACEMENT_3D('',#89677,#67221,#67222);
#61260=AXIS2_PLACEMENT_3D('',#89683,#67226,#67227);
#61261=AXIS2_PLACEMENT_3D('',#89686,#67230,#67231);
#61262=AXIS2_PLACEMENT_3D('',#89687,#67232,#67233);
#61263=AXIS2_PLACEMENT_3D('',#89696,#67238,#67239);
#61264=AXIS2_PLACEMENT_3D('',#89702,#67243,#67244);
#61265=AXIS2_PLACEMENT_3D('',#89708,#67248,#67249);
#61266=AXIS2_PLACEMENT_3D('',#89711,#67252,#67253);
#61267=AXIS2_PLACEMENT_3D('',#89712,#67254,#67255);
#61268=AXIS2_PLACEMENT_3D('',#89721,#67260,#67261);
#61269=AXIS2_PLACEMENT_3D('',#89727,#67265,#67266);
#61270=AXIS2_PLACEMENT_3D('',#89733,#67270,#67271);
#61271=AXIS2_PLACEMENT_3D('',#89736,#67274,#67275);
#61272=AXIS2_PLACEMENT_3D('',#89737,#67276,#67277);
#61273=AXIS2_PLACEMENT_3D('',#89746,#67282,#67283);
#61274=AXIS2_PLACEMENT_3D('',#89752,#67287,#67288);
#61275=AXIS2_PLACEMENT_3D('',#89758,#67292,#67293);
#61276=AXIS2_PLACEMENT_3D('',#89761,#67296,#67297);
#61277=AXIS2_PLACEMENT_3D('',#89762,#67298,#67299);
#61278=AXIS2_PLACEMENT_3D('',#89771,#67304,#67305);
#61279=AXIS2_PLACEMENT_3D('',#89777,#67309,#67310);
#61280=AXIS2_PLACEMENT_3D('',#89783,#67314,#67315);
#61281=AXIS2_PLACEMENT_3D('',#89786,#67318,#67319);
#61282=AXIS2_PLACEMENT_3D('',#89787,#67320,#67321);
#61283=AXIS2_PLACEMENT_3D('',#89796,#67326,#67327);
#61284=AXIS2_PLACEMENT_3D('',#89802,#67331,#67332);
#61285=AXIS2_PLACEMENT_3D('',#89808,#67336,#67337);
#61286=AXIS2_PLACEMENT_3D('',#89811,#67340,#67341);
#61287=AXIS2_PLACEMENT_3D('',#89812,#67342,#67343);
#61288=AXIS2_PLACEMENT_3D('',#89821,#67348,#67349);
#61289=AXIS2_PLACEMENT_3D('',#89827,#67353,#67354);
#61290=AXIS2_PLACEMENT_3D('',#89833,#67358,#67359);
#61291=AXIS2_PLACEMENT_3D('',#89836,#67362,#67363);
#61292=AXIS2_PLACEMENT_3D('',#89837,#67364,#67365);
#61293=AXIS2_PLACEMENT_3D('',#89846,#67370,#67371);
#61294=AXIS2_PLACEMENT_3D('',#89852,#67375,#67376);
#61295=AXIS2_PLACEMENT_3D('',#89858,#67380,#67381);
#61296=AXIS2_PLACEMENT_3D('',#89861,#67384,#67385);
#61297=AXIS2_PLACEMENT_3D('',#89862,#67386,#67387);
#61298=AXIS2_PLACEMENT_3D('',#89871,#67392,#67393);
#61299=AXIS2_PLACEMENT_3D('',#89877,#67397,#67398);
#61300=AXIS2_PLACEMENT_3D('',#89883,#67402,#67403);
#61301=AXIS2_PLACEMENT_3D('',#89886,#67406,#67407);
#61302=AXIS2_PLACEMENT_3D('',#89887,#67408,#67409);
#61303=AXIS2_PLACEMENT_3D('',#89896,#67414,#67415);
#61304=AXIS2_PLACEMENT_3D('',#89902,#67419,#67420);
#61305=AXIS2_PLACEMENT_3D('',#89908,#67424,#67425);
#61306=AXIS2_PLACEMENT_3D('',#89911,#67428,#67429);
#61307=AXIS2_PLACEMENT_3D('',#89912,#67430,#67431);
#61308=AXIS2_PLACEMENT_3D('',#89921,#67436,#67437);
#61309=AXIS2_PLACEMENT_3D('',#89927,#67441,#67442);
#61310=AXIS2_PLACEMENT_3D('',#89933,#67446,#67447);
#61311=AXIS2_PLACEMENT_3D('',#89936,#67450,#67451);
#61312=AXIS2_PLACEMENT_3D('',#89937,#67452,#67453);
#61313=AXIS2_PLACEMENT_3D('',#89946,#67458,#67459);
#61314=AXIS2_PLACEMENT_3D('',#89952,#67463,#67464);
#61315=AXIS2_PLACEMENT_3D('',#89958,#67468,#67469);
#61316=AXIS2_PLACEMENT_3D('',#89961,#67472,#67473);
#61317=AXIS2_PLACEMENT_3D('',#89962,#67474,#67475);
#61318=AXIS2_PLACEMENT_3D('',#89971,#67480,#67481);
#61319=AXIS2_PLACEMENT_3D('',#89977,#67485,#67486);
#61320=AXIS2_PLACEMENT_3D('',#89983,#67490,#67491);
#61321=AXIS2_PLACEMENT_3D('',#89986,#67494,#67495);
#61322=AXIS2_PLACEMENT_3D('',#89987,#67496,#67497);
#61323=AXIS2_PLACEMENT_3D('',#89996,#67502,#67503);
#61324=AXIS2_PLACEMENT_3D('',#90002,#67507,#67508);
#61325=AXIS2_PLACEMENT_3D('',#90008,#67512,#67513);
#61326=AXIS2_PLACEMENT_3D('',#90011,#67516,#67517);
#61327=AXIS2_PLACEMENT_3D('',#90012,#67518,#67519);
#61328=AXIS2_PLACEMENT_3D('',#90021,#67524,#67525);
#61329=AXIS2_PLACEMENT_3D('',#90027,#67529,#67530);
#61330=AXIS2_PLACEMENT_3D('',#90033,#67534,#67535);
#61331=AXIS2_PLACEMENT_3D('',#90036,#67538,#67539);
#61332=AXIS2_PLACEMENT_3D('',#90037,#67540,#67541);
#61333=AXIS2_PLACEMENT_3D('',#90046,#67546,#67547);
#61334=AXIS2_PLACEMENT_3D('',#90052,#67551,#67552);
#61335=AXIS2_PLACEMENT_3D('',#90058,#67556,#67557);
#61336=AXIS2_PLACEMENT_3D('',#90061,#67560,#67561);
#61337=AXIS2_PLACEMENT_3D('',#90062,#67562,#67563);
#61338=AXIS2_PLACEMENT_3D('',#90071,#67568,#67569);
#61339=AXIS2_PLACEMENT_3D('',#90077,#67573,#67574);
#61340=AXIS2_PLACEMENT_3D('',#90083,#67578,#67579);
#61341=AXIS2_PLACEMENT_3D('',#90086,#67582,#67583);
#61342=AXIS2_PLACEMENT_3D('',#90087,#67584,#67585);
#61343=AXIS2_PLACEMENT_3D('',#90096,#67590,#67591);
#61344=AXIS2_PLACEMENT_3D('',#90102,#67595,#67596);
#61345=AXIS2_PLACEMENT_3D('',#90108,#67600,#67601);
#61346=AXIS2_PLACEMENT_3D('',#90111,#67604,#67605);
#61347=AXIS2_PLACEMENT_3D('',#90112,#67606,#67607);
#61348=AXIS2_PLACEMENT_3D('',#90121,#67612,#67613);
#61349=AXIS2_PLACEMENT_3D('',#90127,#67617,#67618);
#61350=AXIS2_PLACEMENT_3D('',#90133,#67622,#67623);
#61351=AXIS2_PLACEMENT_3D('',#90136,#67626,#67627);
#61352=AXIS2_PLACEMENT_3D('',#90137,#67628,#67629);
#61353=AXIS2_PLACEMENT_3D('',#90146,#67634,#67635);
#61354=AXIS2_PLACEMENT_3D('',#90152,#67639,#67640);
#61355=AXIS2_PLACEMENT_3D('',#90158,#67644,#67645);
#61356=AXIS2_PLACEMENT_3D('',#90161,#67648,#67649);
#61357=AXIS2_PLACEMENT_3D('',#90162,#67650,#67651);
#61358=AXIS2_PLACEMENT_3D('',#90171,#67656,#67657);
#61359=AXIS2_PLACEMENT_3D('',#90177,#67661,#67662);
#61360=AXIS2_PLACEMENT_3D('',#90183,#67666,#67667);
#61361=AXIS2_PLACEMENT_3D('',#90186,#67670,#67671);
#61362=AXIS2_PLACEMENT_3D('',#90187,#67672,#67673);
#61363=AXIS2_PLACEMENT_3D('',#90196,#67678,#67679);
#61364=AXIS2_PLACEMENT_3D('',#90202,#67683,#67684);
#61365=AXIS2_PLACEMENT_3D('',#90208,#67688,#67689);
#61366=AXIS2_PLACEMENT_3D('',#90211,#67692,#67693);
#61367=AXIS2_PLACEMENT_3D('',#90212,#67694,#67695);
#61368=AXIS2_PLACEMENT_3D('',#90221,#67700,#67701);
#61369=AXIS2_PLACEMENT_3D('',#90227,#67705,#67706);
#61370=AXIS2_PLACEMENT_3D('',#90233,#67710,#67711);
#61371=AXIS2_PLACEMENT_3D('',#90236,#67714,#67715);
#61372=AXIS2_PLACEMENT_3D('',#90237,#67716,#67717);
#61373=AXIS2_PLACEMENT_3D('',#90246,#67722,#67723);
#61374=AXIS2_PLACEMENT_3D('',#90252,#67727,#67728);
#61375=AXIS2_PLACEMENT_3D('',#90258,#67732,#67733);
#61376=AXIS2_PLACEMENT_3D('',#90261,#67736,#67737);
#61377=AXIS2_PLACEMENT_3D('',#90262,#67738,#67739);
#61378=AXIS2_PLACEMENT_3D('',#90271,#67744,#67745);
#61379=AXIS2_PLACEMENT_3D('',#90277,#67749,#67750);
#61380=AXIS2_PLACEMENT_3D('',#90283,#67754,#67755);
#61381=AXIS2_PLACEMENT_3D('',#90286,#67758,#67759);
#61382=AXIS2_PLACEMENT_3D('',#90287,#67760,#67761);
#61383=AXIS2_PLACEMENT_3D('',#90296,#67766,#67767);
#61384=AXIS2_PLACEMENT_3D('',#90302,#67771,#67772);
#61385=AXIS2_PLACEMENT_3D('',#90308,#67776,#67777);
#61386=AXIS2_PLACEMENT_3D('',#90311,#67780,#67781);
#61387=AXIS2_PLACEMENT_3D('',#90312,#67782,#67783);
#61388=AXIS2_PLACEMENT_3D('',#90321,#67788,#67789);
#61389=AXIS2_PLACEMENT_3D('',#90327,#67793,#67794);
#61390=AXIS2_PLACEMENT_3D('',#90333,#67798,#67799);
#61391=AXIS2_PLACEMENT_3D('',#90336,#67802,#67803);
#61392=AXIS2_PLACEMENT_3D('',#90337,#67804,#67805);
#61393=AXIS2_PLACEMENT_3D('',#90346,#67810,#67811);
#61394=AXIS2_PLACEMENT_3D('',#90352,#67815,#67816);
#61395=AXIS2_PLACEMENT_3D('',#90358,#67820,#67821);
#61396=AXIS2_PLACEMENT_3D('',#90361,#67824,#67825);
#61397=AXIS2_PLACEMENT_3D('',#90362,#67826,#67827);
#61398=AXIS2_PLACEMENT_3D('',#90371,#67832,#67833);
#61399=AXIS2_PLACEMENT_3D('',#90377,#67837,#67838);
#61400=AXIS2_PLACEMENT_3D('',#90383,#67842,#67843);
#61401=AXIS2_PLACEMENT_3D('',#90386,#67846,#67847);
#61402=AXIS2_PLACEMENT_3D('',#90387,#67848,#67849);
#61403=AXIS2_PLACEMENT_3D('',#90396,#67854,#67855);
#61404=AXIS2_PLACEMENT_3D('',#90402,#67859,#67860);
#61405=AXIS2_PLACEMENT_3D('',#90408,#67864,#67865);
#61406=AXIS2_PLACEMENT_3D('',#90411,#67868,#67869);
#61407=AXIS2_PLACEMENT_3D('',#90412,#67870,#67871);
#61408=AXIS2_PLACEMENT_3D('',#90421,#67876,#67877);
#61409=AXIS2_PLACEMENT_3D('',#90427,#67881,#67882);
#61410=AXIS2_PLACEMENT_3D('',#90433,#67886,#67887);
#61411=AXIS2_PLACEMENT_3D('',#90436,#67890,#67891);
#61412=AXIS2_PLACEMENT_3D('',#90437,#67892,#67893);
#61413=AXIS2_PLACEMENT_3D('',#90446,#67898,#67899);
#61414=AXIS2_PLACEMENT_3D('',#90452,#67903,#67904);
#61415=AXIS2_PLACEMENT_3D('',#90458,#67908,#67909);
#61416=AXIS2_PLACEMENT_3D('',#90461,#67912,#67913);
#61417=AXIS2_PLACEMENT_3D('',#90462,#67914,#67915);
#61418=AXIS2_PLACEMENT_3D('',#90471,#67920,#67921);
#61419=AXIS2_PLACEMENT_3D('',#90477,#67925,#67926);
#61420=AXIS2_PLACEMENT_3D('',#90483,#67930,#67931);
#61421=AXIS2_PLACEMENT_3D('',#90486,#67934,#67935);
#61422=AXIS2_PLACEMENT_3D('',#90487,#67936,#67937);
#61423=AXIS2_PLACEMENT_3D('',#90496,#67942,#67943);
#61424=AXIS2_PLACEMENT_3D('',#90502,#67947,#67948);
#61425=AXIS2_PLACEMENT_3D('',#90508,#67952,#67953);
#61426=AXIS2_PLACEMENT_3D('',#90511,#67956,#67957);
#61427=AXIS2_PLACEMENT_3D('',#90512,#67958,#67959);
#61428=AXIS2_PLACEMENT_3D('',#90521,#67964,#67965);
#61429=AXIS2_PLACEMENT_3D('',#90527,#67969,#67970);
#61430=AXIS2_PLACEMENT_3D('',#90533,#67974,#67975);
#61431=AXIS2_PLACEMENT_3D('',#90536,#67978,#67979);
#61432=AXIS2_PLACEMENT_3D('',#90537,#67980,#67981);
#61433=AXIS2_PLACEMENT_3D('',#90546,#67986,#67987);
#61434=AXIS2_PLACEMENT_3D('',#90552,#67991,#67992);
#61435=AXIS2_PLACEMENT_3D('',#90558,#67996,#67997);
#61436=AXIS2_PLACEMENT_3D('',#90561,#68000,#68001);
#61437=AXIS2_PLACEMENT_3D('',#90562,#68002,#68003);
#61438=AXIS2_PLACEMENT_3D('',#90571,#68008,#68009);
#61439=AXIS2_PLACEMENT_3D('',#90577,#68013,#68014);
#61440=AXIS2_PLACEMENT_3D('',#90583,#68018,#68019);
#61441=AXIS2_PLACEMENT_3D('',#90586,#68022,#68023);
#61442=AXIS2_PLACEMENT_3D('',#90587,#68024,#68025);
#61443=AXIS2_PLACEMENT_3D('',#90596,#68030,#68031);
#61444=AXIS2_PLACEMENT_3D('',#90602,#68035,#68036);
#61445=AXIS2_PLACEMENT_3D('',#90608,#68040,#68041);
#61446=AXIS2_PLACEMENT_3D('',#90611,#68044,#68045);
#61447=AXIS2_PLACEMENT_3D('',#90612,#68046,#68047);
#61448=AXIS2_PLACEMENT_3D('',#90621,#68052,#68053);
#61449=AXIS2_PLACEMENT_3D('',#90627,#68057,#68058);
#61450=AXIS2_PLACEMENT_3D('',#90633,#68062,#68063);
#61451=AXIS2_PLACEMENT_3D('',#90636,#68066,#68067);
#61452=AXIS2_PLACEMENT_3D('',#90637,#68068,#68069);
#61453=AXIS2_PLACEMENT_3D('',#90646,#68074,#68075);
#61454=AXIS2_PLACEMENT_3D('',#90652,#68079,#68080);
#61455=AXIS2_PLACEMENT_3D('',#90658,#68084,#68085);
#61456=AXIS2_PLACEMENT_3D('',#90661,#68088,#68089);
#61457=AXIS2_PLACEMENT_3D('',#90662,#68090,#68091);
#61458=AXIS2_PLACEMENT_3D('',#90671,#68096,#68097);
#61459=AXIS2_PLACEMENT_3D('',#90677,#68101,#68102);
#61460=AXIS2_PLACEMENT_3D('',#90683,#68106,#68107);
#61461=AXIS2_PLACEMENT_3D('',#90686,#68110,#68111);
#61462=AXIS2_PLACEMENT_3D('',#90687,#68112,#68113);
#61463=AXIS2_PLACEMENT_3D('',#90696,#68118,#68119);
#61464=AXIS2_PLACEMENT_3D('',#90702,#68123,#68124);
#61465=AXIS2_PLACEMENT_3D('',#90708,#68128,#68129);
#61466=AXIS2_PLACEMENT_3D('',#90711,#68132,#68133);
#61467=AXIS2_PLACEMENT_3D('',#90712,#68134,#68135);
#61468=AXIS2_PLACEMENT_3D('',#90721,#68140,#68141);
#61469=AXIS2_PLACEMENT_3D('',#90727,#68145,#68146);
#61470=AXIS2_PLACEMENT_3D('',#90733,#68150,#68151);
#61471=AXIS2_PLACEMENT_3D('',#90736,#68154,#68155);
#61472=AXIS2_PLACEMENT_3D('',#90737,#68156,#68157);
#61473=AXIS2_PLACEMENT_3D('',#90746,#68162,#68163);
#61474=AXIS2_PLACEMENT_3D('',#90752,#68167,#68168);
#61475=AXIS2_PLACEMENT_3D('',#90758,#68172,#68173);
#61476=AXIS2_PLACEMENT_3D('',#90761,#68176,#68177);
#61477=AXIS2_PLACEMENT_3D('',#90762,#68178,#68179);
#61478=AXIS2_PLACEMENT_3D('',#90771,#68184,#68185);
#61479=AXIS2_PLACEMENT_3D('',#90777,#68189,#68190);
#61480=AXIS2_PLACEMENT_3D('',#90783,#68194,#68195);
#61481=AXIS2_PLACEMENT_3D('',#90786,#68198,#68199);
#61482=AXIS2_PLACEMENT_3D('',#90787,#68200,#68201);
#61483=AXIS2_PLACEMENT_3D('',#90796,#68206,#68207);
#61484=AXIS2_PLACEMENT_3D('',#90802,#68211,#68212);
#61485=AXIS2_PLACEMENT_3D('',#90808,#68216,#68217);
#61486=AXIS2_PLACEMENT_3D('',#90811,#68220,#68221);
#61487=AXIS2_PLACEMENT_3D('',#90812,#68222,#68223);
#61488=AXIS2_PLACEMENT_3D('',#90821,#68228,#68229);
#61489=AXIS2_PLACEMENT_3D('',#90827,#68233,#68234);
#61490=AXIS2_PLACEMENT_3D('',#90833,#68238,#68239);
#61491=AXIS2_PLACEMENT_3D('',#90836,#68242,#68243);
#61492=AXIS2_PLACEMENT_3D('',#90837,#68244,#68245);
#61493=AXIS2_PLACEMENT_3D('',#90846,#68250,#68251);
#61494=AXIS2_PLACEMENT_3D('',#90852,#68255,#68256);
#61495=AXIS2_PLACEMENT_3D('',#90858,#68260,#68261);
#61496=AXIS2_PLACEMENT_3D('',#90861,#68264,#68265);
#61497=AXIS2_PLACEMENT_3D('',#90862,#68266,#68267);
#61498=AXIS2_PLACEMENT_3D('',#90871,#68272,#68273);
#61499=AXIS2_PLACEMENT_3D('',#90877,#68277,#68278);
#61500=AXIS2_PLACEMENT_3D('',#90883,#68282,#68283);
#61501=AXIS2_PLACEMENT_3D('',#90886,#68286,#68287);
#61502=AXIS2_PLACEMENT_3D('',#90887,#68288,#68289);
#61503=AXIS2_PLACEMENT_3D('',#90896,#68294,#68295);
#61504=AXIS2_PLACEMENT_3D('',#90902,#68299,#68300);
#61505=AXIS2_PLACEMENT_3D('',#90908,#68304,#68305);
#61506=AXIS2_PLACEMENT_3D('',#90911,#68308,#68309);
#61507=AXIS2_PLACEMENT_3D('',#90912,#68310,#68311);
#61508=AXIS2_PLACEMENT_3D('',#90921,#68316,#68317);
#61509=AXIS2_PLACEMENT_3D('',#90927,#68321,#68322);
#61510=AXIS2_PLACEMENT_3D('',#90933,#68326,#68327);
#61511=AXIS2_PLACEMENT_3D('',#90936,#68330,#68331);
#61512=AXIS2_PLACEMENT_3D('',#90937,#68332,#68333);
#61513=AXIS2_PLACEMENT_3D('',#90946,#68338,#68339);
#61514=AXIS2_PLACEMENT_3D('',#90952,#68343,#68344);
#61515=AXIS2_PLACEMENT_3D('',#90958,#68348,#68349);
#61516=AXIS2_PLACEMENT_3D('',#90961,#68352,#68353);
#61517=AXIS2_PLACEMENT_3D('',#90962,#68354,#68355);
#61518=AXIS2_PLACEMENT_3D('',#90971,#68360,#68361);
#61519=AXIS2_PLACEMENT_3D('',#90977,#68365,#68366);
#61520=AXIS2_PLACEMENT_3D('',#90983,#68370,#68371);
#61521=AXIS2_PLACEMENT_3D('',#90986,#68374,#68375);
#61522=AXIS2_PLACEMENT_3D('',#90987,#68376,#68377);
#61523=AXIS2_PLACEMENT_3D('',#90996,#68382,#68383);
#61524=AXIS2_PLACEMENT_3D('',#91002,#68387,#68388);
#61525=AXIS2_PLACEMENT_3D('',#91008,#68392,#68393);
#61526=AXIS2_PLACEMENT_3D('',#91011,#68396,#68397);
#61527=AXIS2_PLACEMENT_3D('',#91012,#68398,#68399);
#61528=AXIS2_PLACEMENT_3D('',#91021,#68404,#68405);
#61529=AXIS2_PLACEMENT_3D('',#91027,#68409,#68410);
#61530=AXIS2_PLACEMENT_3D('',#91033,#68414,#68415);
#61531=AXIS2_PLACEMENT_3D('',#91036,#68418,#68419);
#61532=AXIS2_PLACEMENT_3D('',#91037,#68420,#68421);
#61533=AXIS2_PLACEMENT_3D('',#91046,#68426,#68427);
#61534=AXIS2_PLACEMENT_3D('',#91052,#68431,#68432);
#61535=AXIS2_PLACEMENT_3D('',#91058,#68436,#68437);
#61536=AXIS2_PLACEMENT_3D('',#91061,#68440,#68441);
#61537=AXIS2_PLACEMENT_3D('',#91062,#68442,#68443);
#61538=AXIS2_PLACEMENT_3D('',#91071,#68448,#68449);
#61539=AXIS2_PLACEMENT_3D('',#91077,#68453,#68454);
#61540=AXIS2_PLACEMENT_3D('',#91083,#68458,#68459);
#61541=AXIS2_PLACEMENT_3D('',#91086,#68462,#68463);
#61542=AXIS2_PLACEMENT_3D('',#91087,#68464,#68465);
#61543=AXIS2_PLACEMENT_3D('',#91096,#68470,#68471);
#61544=AXIS2_PLACEMENT_3D('',#91102,#68475,#68476);
#61545=AXIS2_PLACEMENT_3D('',#91108,#68480,#68481);
#61546=AXIS2_PLACEMENT_3D('',#91111,#68484,#68485);
#61547=AXIS2_PLACEMENT_3D('',#91112,#68486,#68487);
#61548=AXIS2_PLACEMENT_3D('',#91121,#68492,#68493);
#61549=AXIS2_PLACEMENT_3D('',#91127,#68497,#68498);
#61550=AXIS2_PLACEMENT_3D('',#91133,#68502,#68503);
#61551=AXIS2_PLACEMENT_3D('',#91136,#68506,#68507);
#61552=AXIS2_PLACEMENT_3D('',#91137,#68508,#68509);
#61553=AXIS2_PLACEMENT_3D('',#91146,#68514,#68515);
#61554=AXIS2_PLACEMENT_3D('',#91152,#68519,#68520);
#61555=AXIS2_PLACEMENT_3D('',#91158,#68524,#68525);
#61556=AXIS2_PLACEMENT_3D('',#91161,#68528,#68529);
#61557=AXIS2_PLACEMENT_3D('',#91162,#68530,#68531);
#61558=AXIS2_PLACEMENT_3D('',#91171,#68536,#68537);
#61559=AXIS2_PLACEMENT_3D('',#91177,#68541,#68542);
#61560=AXIS2_PLACEMENT_3D('',#91183,#68546,#68547);
#61561=AXIS2_PLACEMENT_3D('',#91186,#68550,#68551);
#61562=AXIS2_PLACEMENT_3D('',#91187,#68552,#68553);
#61563=AXIS2_PLACEMENT_3D('',#91196,#68558,#68559);
#61564=AXIS2_PLACEMENT_3D('',#91202,#68563,#68564);
#61565=AXIS2_PLACEMENT_3D('',#91208,#68568,#68569);
#61566=AXIS2_PLACEMENT_3D('',#91211,#68572,#68573);
#61567=AXIS2_PLACEMENT_3D('',#91212,#68574,#68575);
#61568=AXIS2_PLACEMENT_3D('',#91221,#68580,#68581);
#61569=AXIS2_PLACEMENT_3D('',#91227,#68585,#68586);
#61570=AXIS2_PLACEMENT_3D('',#91233,#68590,#68591);
#61571=AXIS2_PLACEMENT_3D('',#91236,#68594,#68595);
#61572=AXIS2_PLACEMENT_3D('',#91237,#68596,#68597);
#61573=AXIS2_PLACEMENT_3D('',#91246,#68602,#68603);
#61574=AXIS2_PLACEMENT_3D('',#91252,#68607,#68608);
#61575=AXIS2_PLACEMENT_3D('',#91258,#68612,#68613);
#61576=AXIS2_PLACEMENT_3D('',#91261,#68616,#68617);
#61577=AXIS2_PLACEMENT_3D('',#91262,#68618,#68619);
#61578=AXIS2_PLACEMENT_3D('',#91271,#68624,#68625);
#61579=AXIS2_PLACEMENT_3D('',#91277,#68629,#68630);
#61580=AXIS2_PLACEMENT_3D('',#91283,#68634,#68635);
#61581=AXIS2_PLACEMENT_3D('',#91286,#68638,#68639);
#61582=AXIS2_PLACEMENT_3D('',#91287,#68640,#68641);
#61583=AXIS2_PLACEMENT_3D('',#91296,#68646,#68647);
#61584=AXIS2_PLACEMENT_3D('',#91302,#68651,#68652);
#61585=AXIS2_PLACEMENT_3D('',#91308,#68656,#68657);
#61586=AXIS2_PLACEMENT_3D('',#91311,#68660,#68661);
#61587=AXIS2_PLACEMENT_3D('',#91312,#68662,#68663);
#61588=AXIS2_PLACEMENT_3D('',#91321,#68668,#68669);
#61589=AXIS2_PLACEMENT_3D('',#91327,#68673,#68674);
#61590=AXIS2_PLACEMENT_3D('',#91333,#68678,#68679);
#61591=AXIS2_PLACEMENT_3D('',#91336,#68682,#68683);
#61592=AXIS2_PLACEMENT_3D('',#91337,#68684,#68685);
#61593=AXIS2_PLACEMENT_3D('',#91346,#68690,#68691);
#61594=AXIS2_PLACEMENT_3D('',#91352,#68695,#68696);
#61595=AXIS2_PLACEMENT_3D('',#91358,#68700,#68701);
#61596=AXIS2_PLACEMENT_3D('',#91361,#68704,#68705);
#61597=AXIS2_PLACEMENT_3D('',#91362,#68706,#68707);
#61598=AXIS2_PLACEMENT_3D('',#91371,#68712,#68713);
#61599=AXIS2_PLACEMENT_3D('',#91377,#68717,#68718);
#61600=AXIS2_PLACEMENT_3D('',#91383,#68722,#68723);
#61601=AXIS2_PLACEMENT_3D('',#91386,#68726,#68727);
#61602=AXIS2_PLACEMENT_3D('',#91387,#68728,#68729);
#61603=AXIS2_PLACEMENT_3D('',#91396,#68734,#68735);
#61604=AXIS2_PLACEMENT_3D('',#91402,#68739,#68740);
#61605=AXIS2_PLACEMENT_3D('',#91408,#68744,#68745);
#61606=AXIS2_PLACEMENT_3D('',#91411,#68748,#68749);
#61607=AXIS2_PLACEMENT_3D('',#91412,#68750,#68751);
#61608=AXIS2_PLACEMENT_3D('',#91421,#68756,#68757);
#61609=AXIS2_PLACEMENT_3D('',#91427,#68761,#68762);
#61610=AXIS2_PLACEMENT_3D('',#91433,#68766,#68767);
#61611=AXIS2_PLACEMENT_3D('',#91436,#68770,#68771);
#61612=AXIS2_PLACEMENT_3D('',#91437,#68772,#68773);
#61613=AXIS2_PLACEMENT_3D('',#91446,#68778,#68779);
#61614=AXIS2_PLACEMENT_3D('',#91452,#68783,#68784);
#61615=AXIS2_PLACEMENT_3D('',#91458,#68788,#68789);
#61616=AXIS2_PLACEMENT_3D('',#91461,#68792,#68793);
#61617=AXIS2_PLACEMENT_3D('',#91462,#68794,#68795);
#61618=AXIS2_PLACEMENT_3D('',#91471,#68800,#68801);
#61619=AXIS2_PLACEMENT_3D('',#91477,#68805,#68806);
#61620=AXIS2_PLACEMENT_3D('',#91483,#68810,#68811);
#61621=AXIS2_PLACEMENT_3D('',#91486,#68814,#68815);
#61622=AXIS2_PLACEMENT_3D('',#91487,#68816,#68817);
#61623=AXIS2_PLACEMENT_3D('',#91496,#68822,#68823);
#61624=AXIS2_PLACEMENT_3D('',#91502,#68827,#68828);
#61625=AXIS2_PLACEMENT_3D('',#91508,#68832,#68833);
#61626=AXIS2_PLACEMENT_3D('',#91511,#68836,#68837);
#61627=AXIS2_PLACEMENT_3D('',#91512,#68838,#68839);
#61628=AXIS2_PLACEMENT_3D('',#91521,#68844,#68845);
#61629=AXIS2_PLACEMENT_3D('',#91527,#68849,#68850);
#61630=AXIS2_PLACEMENT_3D('',#91533,#68854,#68855);
#61631=AXIS2_PLACEMENT_3D('',#91536,#68858,#68859);
#61632=AXIS2_PLACEMENT_3D('',#91537,#68860,#68861);
#61633=AXIS2_PLACEMENT_3D('',#91546,#68866,#68867);
#61634=AXIS2_PLACEMENT_3D('',#91552,#68871,#68872);
#61635=AXIS2_PLACEMENT_3D('',#91558,#68876,#68877);
#61636=AXIS2_PLACEMENT_3D('',#91561,#68880,#68881);
#61637=AXIS2_PLACEMENT_3D('',#91562,#68882,#68883);
#61638=AXIS2_PLACEMENT_3D('',#91571,#68888,#68889);
#61639=AXIS2_PLACEMENT_3D('',#91577,#68893,#68894);
#61640=AXIS2_PLACEMENT_3D('',#91583,#68898,#68899);
#61641=AXIS2_PLACEMENT_3D('',#91586,#68902,#68903);
#61642=AXIS2_PLACEMENT_3D('',#91587,#68904,#68905);
#61643=AXIS2_PLACEMENT_3D('',#91596,#68910,#68911);
#61644=AXIS2_PLACEMENT_3D('',#91602,#68915,#68916);
#61645=AXIS2_PLACEMENT_3D('',#91608,#68920,#68921);
#61646=AXIS2_PLACEMENT_3D('',#91611,#68924,#68925);
#61647=AXIS2_PLACEMENT_3D('',#91612,#68926,#68927);
#61648=AXIS2_PLACEMENT_3D('',#91621,#68932,#68933);
#61649=AXIS2_PLACEMENT_3D('',#91627,#68937,#68938);
#61650=AXIS2_PLACEMENT_3D('',#91633,#68942,#68943);
#61651=AXIS2_PLACEMENT_3D('',#91636,#68946,#68947);
#61652=AXIS2_PLACEMENT_3D('',#91637,#68948,#68949);
#61653=AXIS2_PLACEMENT_3D('',#91646,#68954,#68955);
#61654=AXIS2_PLACEMENT_3D('',#91652,#68959,#68960);
#61655=AXIS2_PLACEMENT_3D('',#91658,#68964,#68965);
#61656=AXIS2_PLACEMENT_3D('',#91661,#68968,#68969);
#61657=AXIS2_PLACEMENT_3D('',#91662,#68970,#68971);
#61658=AXIS2_PLACEMENT_3D('',#91671,#68976,#68977);
#61659=AXIS2_PLACEMENT_3D('',#91677,#68981,#68982);
#61660=AXIS2_PLACEMENT_3D('',#91683,#68986,#68987);
#61661=AXIS2_PLACEMENT_3D('',#91686,#68990,#68991);
#61662=AXIS2_PLACEMENT_3D('',#91687,#68992,#68993);
#61663=AXIS2_PLACEMENT_3D('',#91700,#69000,#69001);
#61664=AXIS2_PLACEMENT_3D('',#91713,#69008,#69009);
#61665=AXIS2_PLACEMENT_3D('',#91716,#69012,#69013);
#61666=AXIS2_PLACEMENT_3D('',#91728,#69019,#69020);
#61667=AXIS2_PLACEMENT_3D('',#91748,#69030,#69031);
#61668=AXIS2_PLACEMENT_3D('',#91758,#69037,#69038);
#61669=AXIS2_PLACEMENT_3D('',#91764,#69042,#69043);
#61670=AXIS2_PLACEMENT_3D('',#91770,#69047,#69048);
#61671=AXIS2_PLACEMENT_3D('',#91774,#69051,#69052);
#61672=AXIS2_PLACEMENT_3D('',#91777,#69054,#69055);
#61673=AXIS2_PLACEMENT_3D('',#91779,#69056,#69057);
#61674=AXIS2_PLACEMENT_3D('',#91781,#69058,#69059);
#61675=AXIS2_PLACEMENT_3D('',#91782,#69060,#69061);
#61676=AXIS2_PLACEMENT_3D('',#91784,#69062,#69063);
#61677=AXIS2_PLACEMENT_3D('',#91787,#69065,#69066);
#61678=AXIS2_PLACEMENT_3D('',#91789,#69067,#69068);
#61679=AXIS2_PLACEMENT_3D('',#91792,#69070,#69071);
#61680=AXIS2_PLACEMENT_3D('',#91794,#69072,#69073);
#61681=AXIS2_PLACEMENT_3D('',#91796,#69075,#69076);
#61682=AXIS2_PLACEMENT_3D('',#91798,#69077,#69078);
#61683=AXIS2_PLACEMENT_3D('',#91800,#69080,#69081);
#61684=AXIS2_PLACEMENT_3D('',#91802,#69082,#69083);
#61685=AXIS2_PLACEMENT_3D('',#91805,#69085,#69086);
#61686=AXIS2_PLACEMENT_3D('',#91806,#69087,#69088);
#61687=AXIS2_PLACEMENT_3D('',#91809,#69090,#69091);
#61688=AXIS2_PLACEMENT_3D('',#91810,#69092,#69093);
#61689=AXIS2_PLACEMENT_3D('',#91820,#69098,#69099);
#61690=AXIS2_PLACEMENT_3D('',#91821,#69100,#69101);
#61691=AXIS2_PLACEMENT_3D('',#91824,#69103,#69104);
#61692=AXIS2_PLACEMENT_3D('',#91827,#69106,#69107);
#61693=AXIS2_PLACEMENT_3D('',#91828,#69108,#69109);
#61694=AXIS2_PLACEMENT_3D('',#91831,#69111,#69112);
#61695=AXIS2_PLACEMENT_3D('',#91832,#69113,#69114);
#61696=AXIS2_PLACEMENT_3D('',#91835,#69116,#69117);
#61697=AXIS2_PLACEMENT_3D('',#91837,#69118,#69119);
#61698=AXIS2_PLACEMENT_3D('',#91840,#69121,#69122);
#61699=AXIS2_PLACEMENT_3D('',#91841,#69123,#69124);
#61700=AXIS2_PLACEMENT_3D('',#91843,#69125,#69126);
#61701=AXIS2_PLACEMENT_3D('',#91844,#69127,#69128);
#61702=AXIS2_PLACEMENT_3D('',#91846,#69129,#69130);
#61703=AXIS2_PLACEMENT_3D('',#91849,#69132,#69133);
#61704=AXIS2_PLACEMENT_3D('',#91850,#69134,#69135);
#61705=AXIS2_PLACEMENT_3D('',#91852,#69136,#69137);
#61706=AXIS2_PLACEMENT_3D('',#91853,#69138,#69139);
#61707=AXIS2_PLACEMENT_3D('',#91855,#69140,#69141);
#61708=AXIS2_PLACEMENT_3D('',#91858,#69143,#69144);
#61709=AXIS2_PLACEMENT_3D('',#91859,#69145,#69146);
#61710=AXIS2_PLACEMENT_3D('',#91861,#69147,#69148);
#61711=AXIS2_PLACEMENT_3D('',#91862,#69149,#69150);
#61712=AXIS2_PLACEMENT_3D('',#91864,#69151,#69152);
#61713=AXIS2_PLACEMENT_3D('',#91867,#69154,#69155);
#61714=AXIS2_PLACEMENT_3D('',#91868,#69156,#69157);
#61715=AXIS2_PLACEMENT_3D('',#91870,#69158,#69159);
#61716=AXIS2_PLACEMENT_3D('',#91871,#69160,#69161);
#61717=AXIS2_PLACEMENT_3D('',#91873,#69162,#69163);
#61718=AXIS2_PLACEMENT_3D('',#91876,#69165,#69166);
#61719=AXIS2_PLACEMENT_3D('',#91877,#69167,#69168);
#61720=AXIS2_PLACEMENT_3D('',#91879,#69169,#69170);
#61721=AXIS2_PLACEMENT_3D('',#91880,#69171,#69172);
#61722=AXIS2_PLACEMENT_3D('',#91882,#69173,#69174);
#61723=AXIS2_PLACEMENT_3D('',#91885,#69176,#69177);
#61724=AXIS2_PLACEMENT_3D('',#91886,#69178,#69179);
#61725=AXIS2_PLACEMENT_3D('',#91888,#69180,#69181);
#61726=AXIS2_PLACEMENT_3D('',#91889,#69182,#69183);
#61727=AXIS2_PLACEMENT_3D('',#91892,#69185,#69186);
#61728=AXIS2_PLACEMENT_3D('',#91893,#69187,#69188);
#61729=AXIS2_PLACEMENT_3D('',#91898,#69191,#69192);
#61730=AXIS2_PLACEMENT_3D('',#91900,#69193,#69194);
#61731=AXIS2_PLACEMENT_3D('',#91902,#69195,#69196);
#61732=AXIS2_PLACEMENT_3D('',#91903,#69197,#69198);
#61733=AXIS2_PLACEMENT_3D('',#91905,#69200,#69201);
#61734=AXIS2_PLACEMENT_3D('',#91908,#69203,#69204);
#61735=AXIS2_PLACEMENT_3D('',#91909,#69205,#69206);
#61736=AXIS2_PLACEMENT_3D('',#91911,#69208,#69209);
#61737=AXIS2_PLACEMENT_3D('',#91914,#69211,#69212);
#61738=AXIS2_PLACEMENT_3D('',#91915,#69213,#69214);
#61739=AXIS2_PLACEMENT_3D('',#91917,#69216,#69217);
#61740=AXIS2_PLACEMENT_3D('',#91920,#69219,#69220);
#61741=AXIS2_PLACEMENT_3D('',#91921,#69221,#69222);
#61742=AXIS2_PLACEMENT_3D('',#91923,#69224,#69225);
#61743=AXIS2_PLACEMENT_3D('',#91926,#69227,#69228);
#61744=AXIS2_PLACEMENT_3D('',#91927,#69229,#69230);
#61745=AXIS2_PLACEMENT_3D('',#91929,#69232,#69233);
#61746=AXIS2_PLACEMENT_3D('',#91932,#69235,#69236);
#61747=AXIS2_PLACEMENT_3D('',#91933,#69237,#69238);
#61748=AXIS2_PLACEMENT_3D('',#91935,#69240,#69241);
#61749=AXIS2_PLACEMENT_3D('',#91940,#69243,#69244);
#61750=AXIS2_PLACEMENT_3D('',#91944,#69247,#69248);
#61751=AXIS2_PLACEMENT_3D('',#91950,#69252,#69253);
#61752=AXIS2_PLACEMENT_3D('',#91956,#69257,#69258);
#61753=AXIS2_PLACEMENT_3D('',#91964,#69263,#69264);
#61754=AXIS2_PLACEMENT_3D('',#91970,#69268,#69269);
#61755=AXIS2_PLACEMENT_3D('',#91976,#69273,#69274);
#61756=AXIS2_PLACEMENT_3D('',#91980,#69276,#69277);
#61757=AXIS2_PLACEMENT_3D('',#91982,#69279,#69280);
#61758=AXIS2_PLACEMENT_3D('',#91986,#69283,#69284);
#61759=AXIS2_PLACEMENT_3D('',#91989,#69287,#69288);
#61760=AXIS2_PLACEMENT_3D('',#91992,#69290,#69291);
#61761=AXIS2_PLACEMENT_3D('',#91994,#69292,#69293);
#61762=AXIS2_PLACEMENT_3D('',#91998,#69295,#69296);
#61763=AXIS2_PLACEMENT_3D('',#91999,#69297,#69298);
#61764=AXIS2_PLACEMENT_3D('',#92000,#69299,#69300);
#61765=AXIS2_PLACEMENT_3D('',#92004,#69303,#69304);
#61766=AXIS2_PLACEMENT_3D('',#92008,#69307,#69308);
#61767=AXIS2_PLACEMENT_3D('',#92012,#69311,#69312);
#61768=AXIS2_PLACEMENT_3D('',#92014,#69314,#69315);
#61769=AXIS2_PLACEMENT_3D('',#92018,#69318,#69319);
#61770=AXIS2_PLACEMENT_3D('',#92023,#69321,#69322);
#61771=AXIS2_PLACEMENT_3D('',#92027,#69325,#69326);
#61772=AXIS2_PLACEMENT_3D('',#92033,#69330,#69331);
#61773=AXIS2_PLACEMENT_3D('',#92039,#69335,#69336);
#61774=AXIS2_PLACEMENT_3D('',#92042,#69339,#69340);
#61775=AXIS2_PLACEMENT_3D('',#92048,#69344,#69345);
#61776=AXIS2_PLACEMENT_3D('',#92054,#69349,#69350);
#61777=AXIS2_PLACEMENT_3D('',#92060,#69354,#69355);
#61778=AXIS2_PLACEMENT_3D('',#92063,#69358,#69359);
#61779=AXIS2_PLACEMENT_3D('',#92069,#69363,#69364);
#61780=AXIS2_PLACEMENT_3D('',#92073,#69367,#69368);
#61781=AXIS2_PLACEMENT_3D('',#92077,#69371,#69372);
#61782=AXIS2_PLACEMENT_3D('',#92079,#69374,#69375);
#61783=AXIS2_PLACEMENT_3D('',#92083,#69378,#69379);
#61784=AXIS2_PLACEMENT_3D('',#92087,#69382,#69383);
#61785=AXIS2_PLACEMENT_3D('',#92091,#69386,#69387);
#61786=AXIS2_PLACEMENT_3D('',#92093,#69389,#69390);
#61787=AXIS2_PLACEMENT_3D('',#92097,#69392,#69393);
#61788=AXIS2_PLACEMENT_3D('',#92099,#69395,#69396);
#61789=AXIS2_PLACEMENT_3D('',#92103,#69399,#69400);
#61790=AXIS2_PLACEMENT_3D('',#92106,#69403,#69404);
#61791=AXIS2_PLACEMENT_3D('',#92108,#69406,#69407);
#61792=AXIS2_PLACEMENT_3D('',#92110,#69409,#69410);
#61793=AXIS2_PLACEMENT_3D('',#92112,#69412,#69413);
#61794=AXIS2_PLACEMENT_3D('',#92114,#69415,#69416);
#61795=AXIS2_PLACEMENT_3D('',#92116,#69418,#69419);
#61796=AXIS2_PLACEMENT_3D('',#92117,#69420,#69421);
#61797=AXIS2_PLACEMENT_3D('',#92119,#69423,#69424);
#61798=AXIS2_PLACEMENT_3D('',#92121,#69426,#69427);
#61799=AXIS2_PLACEMENT_3D('',#92123,#69429,#69430);
#61800=AXIS2_PLACEMENT_3D('',#92124,#69431,#69432);
#61801=AXIS2_PLACEMENT_3D('',#92126,#69434,#69435);
#61802=AXIS2_PLACEMENT_3D('',#92128,#69437,#69438);
#61803=AXIS2_PLACEMENT_3D('',#92130,#69440,#69441);
#61804=AXIS2_PLACEMENT_3D('',#92132,#69443,#69444);
#61805=AXIS2_PLACEMENT_3D('',#92133,#69445,#69446);
#61806=AXIS2_PLACEMENT_3D('',#92134,#69447,#69448);
#61807=AXIS2_PLACEMENT_3D('',#92135,#69449,#69450);
#61808=AXIS2_PLACEMENT_3D('',#92136,#69451,#69452);
#61809=AXIS2_PLACEMENT_3D('',#92138,#69454,#69455);
#61810=AXIS2_PLACEMENT_3D('',#92140,#69457,#69458);
#61811=AXIS2_PLACEMENT_3D('',#92142,#69460,#69461);
#63778=DIRECTION('axis',(0.,0.,1.));
#63779=DIRECTION('refdir',(1.,0.,0.));
#63780=DIRECTION('',(0.,0.,-1.));
#63781=DIRECTION('',(0.,0.,-1.));
#63782=DIRECTION('',(0.,0.,-1.));
#63783=DIRECTION('',(0.,0.,-1.));
#63784=DIRECTION('',(0.,0.,-1.));
#63785=DIRECTION('',(0.,0.,-1.));
#63786=DIRECTION('',(0.,0.,-1.));
#63787=DIRECTION('',(0.,0.,-1.));
#63788=DIRECTION('',(0.,0.,-1.));
#63789=DIRECTION('',(0.,0.,-1.));
#63790=DIRECTION('',(0.,0.,-1.));
#63791=DIRECTION('',(0.,0.,-1.));
#63792=DIRECTION('',(0.,0.,-1.));
#63793=DIRECTION('',(0.,0.,-1.));
#63794=DIRECTION('',(0.,0.,-1.));
#63795=DIRECTION('',(0.,0.,-1.));
#63796=DIRECTION('',(0.,0.,-1.));
#63797=DIRECTION('',(0.,0.,-1.));
#63798=DIRECTION('',(0.,0.,-1.));
#63799=DIRECTION('',(0.,0.,-1.));
#63800=DIRECTION('center_axis',(0.,0.,1.));
#63801=DIRECTION('ref_axis',(1.,0.,0.));
#63802=DIRECTION('',(0.,0.,-1.));
#63803=DIRECTION('',(0.,0.,-1.));
#63804=DIRECTION('',(0.,0.,-1.));
#63805=DIRECTION('',(0.,0.,-1.));
#63806=DIRECTION('',(0.,0.,-1.));
#63807=DIRECTION('',(0.,0.,-1.));
#63808=DIRECTION('',(0.,0.,-1.));
#63809=DIRECTION('',(0.,0.,-1.));
#63810=DIRECTION('',(0.,0.,-1.));
#63811=DIRECTION('',(0.,0.,-1.));
#63812=DIRECTION('',(0.,0.,-1.));
#63813=DIRECTION('',(0.,0.,-1.));
#63814=DIRECTION('',(0.,0.,-1.));
#63815=DIRECTION('',(0.,0.,-1.));
#63816=DIRECTION('',(0.,0.,-1.));
#63817=DIRECTION('',(0.,0.,-1.));
#63818=DIRECTION('',(0.,0.,-1.));
#63819=DIRECTION('',(0.,0.,-1.));
#63820=DIRECTION('',(0.,0.,-1.));
#63821=DIRECTION('',(0.,0.,-1.));
#63822=DIRECTION('',(0.,0.,-1.));
#63823=DIRECTION('',(0.,0.,-1.));
#63824=DIRECTION('',(0.,0.,-1.));
#63825=DIRECTION('',(0.,0.,-1.));
#63826=DIRECTION('',(0.,0.,-1.));
#63827=DIRECTION('',(0.,0.,-1.));
#63828=DIRECTION('',(0.,0.,-1.));
#63829=DIRECTION('',(0.,0.,-1.));
#63830=DIRECTION('',(0.,0.,-1.));
#63831=DIRECTION('center_axis',(-0.0920922327212455,0.995750481130899,0.));
#63832=DIRECTION('ref_axis',(0.995750481130899,0.0920922327212455,0.));
#63833=DIRECTION('',(0.995750481130899,0.0920922327212455,0.));
#63834=DIRECTION('',(0.,0.,-1.));
#63835=DIRECTION('',(0.995750481130898,0.0920922327212455,0.));
#63836=DIRECTION('center_axis',(0.,0.,1.));
#63837=DIRECTION('ref_axis',(1.,0.,0.));
#63838=DIRECTION('center_axis',(0.,0.,1.));
#63839=DIRECTION('ref_axis',(0.,-1.,0.));
#63840=DIRECTION('center_axis',(0.,0.,1.));
#63841=DIRECTION('ref_axis',(0.,-1.,0.));
#63842=DIRECTION('',(0.,0.,-1.));
#63843=DIRECTION('',(0.,0.,-1.));
#63844=DIRECTION('',(0.,0.,-1.));
#63845=DIRECTION('',(0.,0.,-1.));
#63846=DIRECTION('',(0.,0.,-1.));
#63847=DIRECTION('',(0.,0.,-1.));
#63848=DIRECTION('',(0.,0.,-1.));
#63849=DIRECTION('',(0.,0.,-1.));
#63850=DIRECTION('',(0.,0.,-1.));
#63851=DIRECTION('',(0.,0.,-1.));
#63852=DIRECTION('',(0.,0.,-1.));
#63853=DIRECTION('',(0.,0.,-1.));
#63854=DIRECTION('',(0.,0.,-1.));
#63855=DIRECTION('',(0.,0.,-1.));
#63856=DIRECTION('',(0.,0.,-1.));
#63857=DIRECTION('',(0.,0.,-1.));
#63858=DIRECTION('',(0.,0.,-1.));
#63859=DIRECTION('',(0.,0.,-1.));
#63860=DIRECTION('',(0.,0.,-1.));
#63861=DIRECTION('',(0.,0.,-1.));
#63862=DIRECTION('center_axis',(0.,0.,1.));
#63863=DIRECTION('ref_axis',(1.,0.,0.));
#63864=DIRECTION('',(0.,0.,-1.));
#63865=DIRECTION('',(0.,0.,-1.));
#63866=DIRECTION('',(0.,0.,-1.));
#63867=DIRECTION('',(0.,0.,-1.));
#63868=DIRECTION('',(0.,0.,-1.));
#63869=DIRECTION('',(0.,0.,-1.));
#63870=DIRECTION('',(0.,0.,-1.));
#63871=DIRECTION('',(0.,0.,-1.));
#63872=DIRECTION('',(0.,0.,-1.));
#63873=DIRECTION('',(0.,0.,-1.));
#63874=DIRECTION('',(0.,0.,-1.));
#63875=DIRECTION('',(0.,0.,-1.));
#63876=DIRECTION('',(0.,0.,-1.));
#63877=DIRECTION('',(0.,0.,-1.));
#63878=DIRECTION('',(0.,0.,-1.));
#63879=DIRECTION('',(0.,0.,-1.));
#63880=DIRECTION('',(0.,0.,-1.));
#63881=DIRECTION('',(0.,0.,-1.));
#63882=DIRECTION('',(0.,0.,-1.));
#63883=DIRECTION('',(0.,0.,-1.));
#63884=DIRECTION('',(0.,0.,-1.));
#63885=DIRECTION('',(0.,0.,-1.));
#63886=DIRECTION('',(0.,0.,-1.));
#63887=DIRECTION('',(0.,0.,-1.));
#63888=DIRECTION('',(0.,0.,-1.));
#63889=DIRECTION('',(0.,0.,-1.));
#63890=DIRECTION('',(0.,0.,-1.));
#63891=DIRECTION('',(0.,0.,-1.));
#63892=DIRECTION('',(0.,0.,-1.));
#63893=DIRECTION('',(0.,0.,-1.));
#63894=DIRECTION('',(0.,0.,-1.));
#63895=DIRECTION('',(0.,0.,-1.));
#63896=DIRECTION('',(0.,0.,-1.));
#63897=DIRECTION('center_axis',(0.,0.,1.));
#63898=DIRECTION('ref_axis',(1.,0.,0.));
#63899=DIRECTION('center_axis',(0.,0.,1.));
#63900=DIRECTION('ref_axis',(0.,-1.,0.));
#63901=DIRECTION('center_axis',(0.,0.,1.));
#63902=DIRECTION('ref_axis',(0.,-1.,0.));
#63903=DIRECTION('center_axis',(0.,0.,1.));
#63904=DIRECTION('ref_axis',(0.,-1.,0.));
#63905=DIRECTION('',(0.,0.,-1.));
#63906=DIRECTION('',(0.,0.,-1.));
#63907=DIRECTION('',(0.,0.,-1.));
#63908=DIRECTION('',(0.,0.,-1.));
#63909=DIRECTION('',(0.,0.,-1.));
#63910=DIRECTION('',(0.,0.,-1.));
#63911=DIRECTION('',(0.,0.,-1.));
#63912=DIRECTION('',(0.,0.,-1.));
#63913=DIRECTION('',(0.,0.,-1.));
#63914=DIRECTION('',(0.,0.,-1.));
#63915=DIRECTION('',(0.,0.,-1.));
#63916=DIRECTION('',(0.,0.,-1.));
#63917=DIRECTION('',(0.,0.,-1.));
#63918=DIRECTION('',(0.,0.,-1.));
#63919=DIRECTION('',(0.,0.,-1.));
#63920=DIRECTION('',(0.,0.,-1.));
#63921=DIRECTION('',(0.,0.,-1.));
#63922=DIRECTION('',(0.,0.,-1.));
#63923=DIRECTION('',(0.,0.,-1.));
#63924=DIRECTION('',(0.,0.,-1.));
#63925=DIRECTION('center_axis',(0.,0.,1.));
#63926=DIRECTION('ref_axis',(1.,0.,0.));
#63927=DIRECTION('',(0.,0.,-1.));
#63928=DIRECTION('',(0.,0.,-1.));
#63929=DIRECTION('',(0.,0.,-1.));
#63930=DIRECTION('',(0.,0.,-1.));
#63931=DIRECTION('center_axis',(0.,-1.,0.));
#63932=DIRECTION('ref_axis',(-1.,0.,0.));
#63933=DIRECTION('',(-1.,0.,0.));
#63934=DIRECTION('',(0.,0.,-1.));
#63935=DIRECTION('',(-1.,0.,0.));
#63936=DIRECTION('',(0.,0.,-1.));
#63937=DIRECTION('',(0.,0.,-1.));
#63938=DIRECTION('',(0.,0.,-1.));
#63939=DIRECTION('center_axis',(1.,0.,0.));
#63940=DIRECTION('ref_axis',(0.,-1.,0.));
#63941=DIRECTION('',(0.,-1.,0.));
#63942=DIRECTION('',(0.,0.,-1.));
#63943=DIRECTION('',(0.,-1.,0.));
#63944=DIRECTION('center_axis',(0.,1.,0.));
#63945=DIRECTION('ref_axis',(1.,0.,0.));
#63946=DIRECTION('',(1.,0.,0.));
#63947=DIRECTION('',(0.,0.,-1.));
#63948=DIRECTION('',(1.,0.,0.));
#63949=DIRECTION('center_axis',(-1.,0.,0.));
#63950=DIRECTION('ref_axis',(0.,1.,0.));
#63951=DIRECTION('',(0.,1.,0.));
#63952=DIRECTION('',(0.,0.,-1.));
#63953=DIRECTION('',(0.,1.,0.));
#63954=DIRECTION('center_axis',(0.,-1.,0.));
#63955=DIRECTION('ref_axis',(-1.,0.,0.));
#63956=DIRECTION('',(-1.,0.,0.));
#63957=DIRECTION('',(-1.,0.,0.));
#63958=DIRECTION('center_axis',(0.,0.,1.));
#63959=DIRECTION('ref_axis',(1.,0.,0.));
#63960=DIRECTION('center_axis',(0.,0.,1.));
#63961=DIRECTION('ref_axis',(0.,-1.,0.));
#63962=DIRECTION('',(0.,0.,-1.));
#63963=DIRECTION('',(0.,0.,-1.));
#63964=DIRECTION('',(0.,0.,-1.));
#63965=DIRECTION('',(0.,0.,-1.));
#63966=DIRECTION('',(0.,0.,-1.));
#63967=DIRECTION('',(0.,0.,-1.));
#63968=DIRECTION('',(0.,0.,-1.));
#63969=DIRECTION('',(0.,0.,-1.));
#63970=DIRECTION('',(0.,0.,-1.));
#63971=DIRECTION('',(0.,0.,-1.));
#63972=DIRECTION('',(0.,0.,-1.));
#63973=DIRECTION('',(0.,0.,-1.));
#63974=DIRECTION('',(0.,0.,-1.));
#63975=DIRECTION('',(0.,0.,-1.));
#63976=DIRECTION('',(0.,0.,-1.));
#63977=DIRECTION('',(0.,0.,-1.));
#63978=DIRECTION('',(0.,0.,-1.));
#63979=DIRECTION('',(0.,0.,-1.));
#63980=DIRECTION('',(0.,0.,-1.));
#63981=DIRECTION('',(0.,0.,-1.));
#63982=DIRECTION('center_axis',(0.,0.,1.));
#63983=DIRECTION('ref_axis',(1.,0.,0.));
#63984=DIRECTION('',(0.,0.,-1.));
#63985=DIRECTION('',(0.,0.,-1.));
#63986=DIRECTION('',(0.,0.,-1.));
#63987=DIRECTION('',(0.,0.,-1.));
#63988=DIRECTION('',(0.,0.,-1.));
#63989=DIRECTION('',(0.,0.,-1.));
#63990=DIRECTION('',(0.,0.,-1.));
#63991=DIRECTION('',(0.,0.,-1.));
#63992=DIRECTION('',(0.,0.,-1.));
#63993=DIRECTION('',(0.,0.,-1.));
#63994=DIRECTION('',(0.,0.,-1.));
#63995=DIRECTION('',(0.,0.,-1.));
#63996=DIRECTION('',(0.,0.,-1.));
#63997=DIRECTION('',(0.,0.,-1.));
#63998=DIRECTION('',(0.,0.,-1.));
#63999=DIRECTION('',(0.,0.,-1.));
#64000=DIRECTION('',(0.,0.,-1.));
#64001=DIRECTION('',(0.,0.,-1.));
#64002=DIRECTION('',(0.,0.,-1.));
#64003=DIRECTION('',(0.,0.,-1.));
#64004=DIRECTION('',(0.,0.,-1.));
#64005=DIRECTION('',(0.,0.,-1.));
#64006=DIRECTION('',(0.,0.,-1.));
#64007=DIRECTION('',(0.,0.,-1.));
#64008=DIRECTION('',(0.,0.,-1.));
#64009=DIRECTION('',(0.,0.,-1.));
#64010=DIRECTION('',(0.,0.,-1.));
#64011=DIRECTION('center_axis',(0.0779743449792121,-0.99695536586402,0.));
#64012=DIRECTION('ref_axis',(-0.99695536586402,-0.0779743449792121,0.));
#64013=DIRECTION('',(-0.99695536586402,-0.0779743449792121,0.));
#64014=DIRECTION('',(0.,0.,-1.));
#64015=DIRECTION('',(-0.99695536586402,-0.0779743449792121,0.));
#64016=DIRECTION('center_axis',(0.,0.,1.));
#64017=DIRECTION('ref_axis',(1.,0.,0.));
#64018=DIRECTION('center_axis',(0.,0.,1.));
#64019=DIRECTION('ref_axis',(0.,-1.,0.));
#64020=DIRECTION('center_axis',(0.,0.,1.));
#64021=DIRECTION('ref_axis',(0.,-1.,0.));
#64022=DIRECTION('',(0.,0.,-1.));
#64023=DIRECTION('',(0.,0.,-1.));
#64024=DIRECTION('',(0.,0.,-1.));
#64025=DIRECTION('',(0.,0.,-1.));
#64026=DIRECTION('',(0.,0.,-1.));
#64027=DIRECTION('',(0.,0.,-1.));
#64028=DIRECTION('',(0.,0.,-1.));
#64029=DIRECTION('',(0.,0.,-1.));
#64030=DIRECTION('',(0.,0.,-1.));
#64031=DIRECTION('',(0.,0.,-1.));
#64032=DIRECTION('',(0.,0.,-1.));
#64033=DIRECTION('',(0.,0.,-1.));
#64034=DIRECTION('',(0.,0.,-1.));
#64035=DIRECTION('',(0.,0.,-1.));
#64036=DIRECTION('',(0.,0.,-1.));
#64037=DIRECTION('',(0.,0.,-1.));
#64038=DIRECTION('',(0.,0.,-1.));
#64039=DIRECTION('',(0.,0.,-1.));
#64040=DIRECTION('',(0.,0.,-1.));
#64041=DIRECTION('',(0.,0.,-1.));
#64042=DIRECTION('center_axis',(0.,0.,1.));
#64043=DIRECTION('ref_axis',(1.,0.,0.));
#64044=DIRECTION('',(0.,0.,-1.));
#64045=DIRECTION('',(0.,0.,-1.));
#64046=DIRECTION('',(0.,0.,-1.));
#64047=DIRECTION('',(0.,0.,-1.));
#64048=DIRECTION('',(0.,0.,-1.));
#64049=DIRECTION('',(0.,0.,-1.));
#64050=DIRECTION('',(0.,0.,-1.));
#64051=DIRECTION('center_axis',(0.980484873509324,-0.196594539139329,0.));
#64052=DIRECTION('ref_axis',(-0.196594539139329,-0.980484873509324,0.));
#64053=DIRECTION('',(-0.196594539139329,-0.980484873509324,0.));
#64054=DIRECTION('',(0.,0.,-1.));
#64055=DIRECTION('',(-0.196594539139329,-0.980484873509324,0.));
#64056=DIRECTION('center_axis',(0.,-1.,0.));
#64057=DIRECTION('ref_axis',(-1.,0.,0.));
#64058=DIRECTION('',(-1.,0.,0.));
#64059=DIRECTION('',(0.,0.,-1.));
#64060=DIRECTION('',(-1.,0.,0.));
#64061=DIRECTION('center_axis',(1.,0.,0.));
#64062=DIRECTION('ref_axis',(0.,-1.,0.));
#64063=DIRECTION('',(0.,-1.,0.));
#64064=DIRECTION('',(0.,0.,-1.));
#64065=DIRECTION('',(0.,-1.,0.));
#64066=DIRECTION('center_axis',(0.,1.,0.));
#64067=DIRECTION('ref_axis',(1.,0.,0.));
#64068=DIRECTION('',(1.,0.,0.));
#64069=DIRECTION('',(0.,0.,-1.));
#64070=DIRECTION('',(1.,0.,0.));
#64071=DIRECTION('center_axis',(-0.982679588991295,0.185312777163097,0.));
#64072=DIRECTION('ref_axis',(0.185312777163097,0.982679588991295,0.));
#64073=DIRECTION('',(0.185312777163097,0.982679588991295,0.));
#64074=DIRECTION('',(0.,0.,-1.));
#64075=DIRECTION('',(0.185312777163097,0.982679588991295,0.));
#64076=DIRECTION('center_axis',(-0.129088379836863,-0.991633092525201,0.));
#64077=DIRECTION('ref_axis',(-0.991633092525201,0.129088379836863,0.));
#64078=DIRECTION('',(-0.991633092525201,0.129088379836863,0.));
#64079=DIRECTION('',(0.,0.,-1.));
#64080=DIRECTION('',(-0.991633092525201,0.129088379836863,0.));
#64081=DIRECTION('',(0.,0.,-1.));
#64082=DIRECTION('',(0.,0.,-1.));
#64083=DIRECTION('',(0.,0.,-1.));
#64084=DIRECTION('',(0.,0.,-1.));
#64085=DIRECTION('',(0.,0.,-1.));
#64086=DIRECTION('',(0.,0.,-1.));
#64087=DIRECTION('',(0.,0.,-1.));
#64088=DIRECTION('',(0.,0.,-1.));
#64089=DIRECTION('center_axis',(-0.0843540635911639,0.99643584437517,0.));
#64090=DIRECTION('ref_axis',(0.99643584437517,0.0843540635911639,0.));
#64091=DIRECTION('',(0.99643584437517,0.0843540635911639,0.));
#64092=DIRECTION('',(0.,0.,-1.));
#64093=DIRECTION('',(0.99643584437517,0.0843540635911639,0.));
#64094=DIRECTION('center_axis',(0.,0.,1.));
#64095=DIRECTION('ref_axis',(1.,0.,0.));
#64096=DIRECTION('center_axis',(0.,0.,1.));
#64097=DIRECTION('ref_axis',(0.,-1.,0.));
#64098=DIRECTION('',(0.,0.,-1.));
#64099=DIRECTION('',(0.,0.,-1.));
#64100=DIRECTION('',(0.,0.,-1.));
#64101=DIRECTION('',(0.,0.,-1.));
#64102=DIRECTION('',(0.,0.,-1.));
#64103=DIRECTION('',(0.,0.,-1.));
#64104=DIRECTION('',(0.,0.,-1.));
#64105=DIRECTION('',(0.,0.,-1.));
#64106=DIRECTION('',(0.,0.,-1.));
#64107=DIRECTION('',(0.,0.,-1.));
#64108=DIRECTION('',(0.,0.,-1.));
#64109=DIRECTION('',(0.,0.,-1.));
#64110=DIRECTION('',(0.,0.,-1.));
#64111=DIRECTION('',(0.,0.,-1.));
#64112=DIRECTION('',(0.,0.,-1.));
#64113=DIRECTION('',(0.,0.,-1.));
#64114=DIRECTION('',(0.,0.,-1.));
#64115=DIRECTION('',(0.,0.,-1.));
#64116=DIRECTION('',(0.,0.,-1.));
#64117=DIRECTION('',(0.,0.,-1.));
#64118=DIRECTION('center_axis',(0.,0.,1.));
#64119=DIRECTION('ref_axis',(1.,0.,0.));
#64120=DIRECTION('center_axis',(0.821386116423605,-0.570372551712079,0.));
#64121=DIRECTION('ref_axis',(-0.570372551712079,-0.821386116423605,0.));
#64122=DIRECTION('',(-0.570372551712079,-0.821386116423605,0.));
#64123=DIRECTION('',(0.,0.,-1.));
#64124=DIRECTION('',(-0.570372551712079,-0.821386116423605,0.));
#64125=DIRECTION('',(0.,0.,-1.));
#64126=DIRECTION('center_axis',(-1.,0.,0.));
#64127=DIRECTION('ref_axis',(0.,1.,0.));
#64128=DIRECTION('',(0.,1.,0.));
#64129=DIRECTION('',(0.,0.,-1.));
#64130=DIRECTION('',(0.,1.,0.));
#64131=DIRECTION('center_axis',(0.,1.,0.));
#64132=DIRECTION('ref_axis',(1.,0.,0.));
#64133=DIRECTION('',(1.,0.,0.));
#64134=DIRECTION('',(1.,0.,0.));
#64135=DIRECTION('center_axis',(1.,0.,0.));
#64136=DIRECTION('ref_axis',(0.,-1.,0.));
#64137=DIRECTION('',(0.,-1.,0.));
#64138=DIRECTION('',(0.,0.,-1.));
#64139=DIRECTION('',(0.,-1.,0.));
#64140=DIRECTION('',(0.,0.,-1.));
#64141=DIRECTION('center_axis',(0.,-1.,0.));
#64142=DIRECTION('ref_axis',(-1.,0.,0.));
#64143=DIRECTION('',(-1.,0.,0.));
#64144=DIRECTION('',(0.,0.,-1.));
#64145=DIRECTION('',(-1.,0.,0.));
#64146=DIRECTION('center_axis',(1.,0.,0.));
#64147=DIRECTION('ref_axis',(0.,-1.,0.));
#64148=DIRECTION('',(0.,-1.,0.));
#64149=DIRECTION('',(0.,0.,-1.));
#64150=DIRECTION('',(0.,-1.,0.));
#64151=DIRECTION('center_axis',(0.,1.,0.));
#64152=DIRECTION('ref_axis',(1.,0.,0.));
#64153=DIRECTION('',(1.,0.,0.));
#64154=DIRECTION('',(0.,0.,-1.));
#64155=DIRECTION('',(1.,0.,0.));
#64156=DIRECTION('center_axis',(1.,0.,0.));
#64157=DIRECTION('ref_axis',(0.,-1.,0.));
#64158=DIRECTION('',(0.,-1.,0.));
#64159=DIRECTION('',(0.,0.,-1.));
#64160=DIRECTION('',(0.,-1.,0.));
#64161=DIRECTION('center_axis',(0.,1.,0.));
#64162=DIRECTION('ref_axis',(1.,0.,0.));
#64163=DIRECTION('',(1.,0.,0.));
#64164=DIRECTION('',(0.,0.,-1.));
#64165=DIRECTION('',(1.,0.,0.));
#64166=DIRECTION('center_axis',(-0.817611346967032,0.575770514450641,0.));
#64167=DIRECTION('ref_axis',(0.575770514450641,0.817611346967032,0.));
#64168=DIRECTION('',(0.575770514450641,0.817611346967032,0.));
#64169=DIRECTION('',(0.,0.,-1.));
#64170=DIRECTION('',(0.575770514450641,0.817611346967032,0.));
#64171=DIRECTION('center_axis',(-1.,0.,0.));
#64172=DIRECTION('ref_axis',(0.,1.,0.));
#64173=DIRECTION('',(0.,1.,0.));
#64174=DIRECTION('',(0.,0.,-1.));
#64175=DIRECTION('',(0.,1.,0.));
#64176=DIRECTION('center_axis',(0.,-1.,0.));
#64177=DIRECTION('ref_axis',(-1.,0.,0.));
#64178=DIRECTION('',(-1.,0.,0.));
#64179=DIRECTION('',(0.,0.,-1.));
#64180=DIRECTION('',(-1.,0.,0.));
#64181=DIRECTION('center_axis',(-1.,0.,0.));
#64182=DIRECTION('ref_axis',(0.,1.,0.));
#64183=DIRECTION('',(0.,1.,0.));
#64184=DIRECTION('',(0.,0.,-1.));
#64185=DIRECTION('',(0.,1.,0.));
#64186=DIRECTION('center_axis',(0.,-1.,0.));
#64187=DIRECTION('ref_axis',(-1.,0.,0.));
#64188=DIRECTION('',(-1.,0.,0.));
#64189=DIRECTION('',(-1.,0.,0.));
#64190=DIRECTION('center_axis',(0.,0.,-1.));
#64191=DIRECTION('ref_axis',(-1.,0.,0.));
#64192=DIRECTION('center_axis',(0.,0.,1.));
#64193=DIRECTION('ref_axis',(0.,-1.,0.));
#64194=DIRECTION('center_axis',(0.,0.,1.));
#64195=DIRECTION('ref_axis',(0.,-1.,0.));
#64196=DIRECTION('',(0.,0.,-1.));
#64197=DIRECTION('',(0.,0.,-1.));
#64198=DIRECTION('',(0.,0.,-1.));
#64199=DIRECTION('',(0.,0.,-1.));
#64200=DIRECTION('',(0.,0.,-1.));
#64201=DIRECTION('',(0.,0.,-1.));
#64202=DIRECTION('',(0.,0.,-1.));
#64203=DIRECTION('',(0.,0.,-1.));
#64204=DIRECTION('',(0.,0.,-1.));
#64205=DIRECTION('',(0.,0.,-1.));
#64206=DIRECTION('',(0.,0.,-1.));
#64207=DIRECTION('',(0.,0.,-1.));
#64208=DIRECTION('',(0.,0.,-1.));
#64209=DIRECTION('',(0.,0.,-1.));
#64210=DIRECTION('',(0.,0.,-1.));
#64211=DIRECTION('',(0.,0.,-1.));
#64212=DIRECTION('',(0.,0.,-1.));
#64213=DIRECTION('',(0.,0.,-1.));
#64214=DIRECTION('',(0.,0.,-1.));
#64215=DIRECTION('',(0.,0.,-1.));
#64216=DIRECTION('center_axis',(0.,0.,1.));
#64217=DIRECTION('ref_axis',(1.,0.,0.));
#64218=DIRECTION('',(0.,0.,-1.));
#64219=DIRECTION('',(0.,0.,-1.));
#64220=DIRECTION('',(0.,0.,-1.));
#64221=DIRECTION('',(0.,0.,-1.));
#64222=DIRECTION('',(0.,0.,-1.));
#64223=DIRECTION('',(0.,0.,-1.));
#64224=DIRECTION('',(0.,0.,-1.));
#64225=DIRECTION('',(0.,0.,-1.));
#64226=DIRECTION('',(0.,0.,-1.));
#64227=DIRECTION('',(0.,0.,-1.));
#64228=DIRECTION('',(0.,0.,-1.));
#64229=DIRECTION('',(0.,0.,-1.));
#64230=DIRECTION('',(0.,0.,-1.));
#64231=DIRECTION('center_axis',(-0.175033346417238,-0.984562505705952,0.));
#64232=DIRECTION('ref_axis',(-0.984562505705952,0.175033346417238,0.));
#64233=DIRECTION('',(-0.984562505705952,0.175033346417238,0.));
#64234=DIRECTION('',(0.,0.,-1.));
#64235=DIRECTION('',(-0.984562505705952,0.175033346417238,0.));
#64236=DIRECTION('',(0.,0.,-1.));
#64237=DIRECTION('',(0.,0.,-1.));
#64238=DIRECTION('',(0.,0.,-1.));
#64239=DIRECTION('',(0.,0.,-1.));
#64240=DIRECTION('',(0.,0.,-1.));
#64241=DIRECTION('',(0.,0.,-1.));
#64242=DIRECTION('',(0.,0.,-1.));
#64243=DIRECTION('center_axis',(-0.992083480553514,0.125580124274607,0.));
#64244=DIRECTION('ref_axis',(0.125580124274607,0.992083480553514,0.));
#64245=DIRECTION('',(0.125580124274607,0.992083480553514,0.));
#64246=DIRECTION('',(0.,0.,-1.));
#64247=DIRECTION('',(0.125580124274607,0.992083480553514,0.));
#64248=DIRECTION('',(0.,0.,-1.));
#64249=DIRECTION('',(0.,0.,-1.));
#64250=DIRECTION('',(0.,0.,-1.));
#64251=DIRECTION('',(0.,0.,-1.));
#64252=DIRECTION('',(0.,0.,-1.));
#64253=DIRECTION('',(0.,0.,-1.));
#64254=DIRECTION('',(0.,0.,-1.));
#64255=DIRECTION('center_axis',(-0.132163863358704,0.991227881580266,0.));
#64256=DIRECTION('ref_axis',(0.991227881580266,0.132163863358704,0.));
#64257=DIRECTION('',(0.991227881580266,0.132163863358704,0.));
#64258=DIRECTION('',(0.,0.,-1.));
#64259=DIRECTION('',(0.991227881580266,0.132163863358704,0.));
#64260=DIRECTION('center_axis',(0.,0.,1.));
#64261=DIRECTION('ref_axis',(1.,0.,0.));
#64262=DIRECTION('center_axis',(0.,0.,1.));
#64263=DIRECTION('ref_axis',(0.,-1.,0.));
#64264=DIRECTION('',(0.,0.,-1.));
#64265=DIRECTION('',(0.,0.,-1.));
#64266=DIRECTION('',(0.,0.,-1.));
#64267=DIRECTION('',(0.,0.,-1.));
#64268=DIRECTION('',(0.,0.,-1.));
#64269=DIRECTION('',(0.,0.,-1.));
#64270=DIRECTION('',(0.,0.,-1.));
#64271=DIRECTION('',(0.,0.,-1.));
#64272=DIRECTION('',(0.,0.,-1.));
#64273=DIRECTION('',(0.,0.,-1.));
#64274=DIRECTION('',(0.,0.,-1.));
#64275=DIRECTION('',(0.,0.,-1.));
#64276=DIRECTION('',(0.,0.,-1.));
#64277=DIRECTION('',(0.,0.,-1.));
#64278=DIRECTION('',(0.,0.,-1.));
#64279=DIRECTION('',(0.,0.,-1.));
#64280=DIRECTION('',(0.,0.,-1.));
#64281=DIRECTION('',(0.,0.,-1.));
#64282=DIRECTION('',(0.,0.,-1.));
#64283=DIRECTION('',(0.,0.,-1.));
#64284=DIRECTION('center_axis',(0.,0.,1.));
#64285=DIRECTION('ref_axis',(1.,0.,0.));
#64286=DIRECTION('',(0.,0.,-1.));
#64287=DIRECTION('',(0.,0.,-1.));
#64288=DIRECTION('',(0.,0.,-1.));
#64289=DIRECTION('',(0.,0.,-1.));
#64290=DIRECTION('',(0.,0.,-1.));
#64291=DIRECTION('',(0.,0.,-1.));
#64292=DIRECTION('',(0.,0.,-1.));
#64293=DIRECTION('',(0.,0.,-1.));
#64294=DIRECTION('',(0.,0.,-1.));
#64295=DIRECTION('',(0.,0.,-1.));
#64296=DIRECTION('center_axis',(-0.102165169950561,-0.99476744923071,0.));
#64297=DIRECTION('ref_axis',(-0.99476744923071,0.102165169950561,0.));
#64298=DIRECTION('',(-0.99476744923071,0.102165169950561,0.));
#64299=DIRECTION('',(0.,0.,-1.));
#64300=DIRECTION('',(-0.99476744923071,0.102165169950561,0.));
#64301=DIRECTION('',(0.,0.,-1.));
#64302=DIRECTION('',(0.,0.,-1.));
#64303=DIRECTION('',(0.,0.,-1.));
#64304=DIRECTION('',(0.,0.,-1.));
#64305=DIRECTION('',(0.,0.,-1.));
#64306=DIRECTION('',(0.,0.,-1.));
#64307=DIRECTION('',(0.,0.,-1.));
#64308=DIRECTION('',(0.,0.,-1.));
#64309=DIRECTION('',(0.,0.,-1.));
#64310=DIRECTION('center_axis',(0.,-1.,0.));
#64311=DIRECTION('ref_axis',(-1.,0.,0.));
#64312=DIRECTION('',(-1.,0.,0.));
#64313=DIRECTION('',(0.,0.,-1.));
#64314=DIRECTION('',(-1.,0.,0.));
#64315=DIRECTION('center_axis',(1.,0.,0.));
#64316=DIRECTION('ref_axis',(0.,-1.,0.));
#64317=DIRECTION('',(0.,-1.,0.));
#64318=DIRECTION('',(0.,0.,-1.));
#64319=DIRECTION('',(0.,-1.,0.));
#64320=DIRECTION('center_axis',(0.,1.,0.));
#64321=DIRECTION('ref_axis',(1.,0.,0.));
#64322=DIRECTION('',(1.,0.,0.));
#64323=DIRECTION('',(1.,0.,0.));
#64324=DIRECTION('center_axis',(0.,0.,1.));
#64325=DIRECTION('ref_axis',(1.,0.,0.));
#64326=DIRECTION('center_axis',(0.,0.,1.));
#64327=DIRECTION('ref_axis',(0.,-1.,0.));
#64328=DIRECTION('',(0.,0.,-1.));
#64329=DIRECTION('',(0.,0.,-1.));
#64330=DIRECTION('',(0.,0.,-1.));
#64331=DIRECTION('',(0.,0.,-1.));
#64332=DIRECTION('',(0.,0.,-1.));
#64333=DIRECTION('',(0.,0.,-1.));
#64334=DIRECTION('',(0.,0.,-1.));
#64335=DIRECTION('',(0.,0.,-1.));
#64336=DIRECTION('',(0.,0.,-1.));
#64337=DIRECTION('',(0.,0.,-1.));
#64338=DIRECTION('',(0.,0.,-1.));
#64339=DIRECTION('',(0.,0.,-1.));
#64340=DIRECTION('',(0.,0.,-1.));
#64341=DIRECTION('',(0.,0.,-1.));
#64342=DIRECTION('',(0.,0.,-1.));
#64343=DIRECTION('',(0.,0.,-1.));
#64344=DIRECTION('',(0.,0.,-1.));
#64345=DIRECTION('',(0.,0.,-1.));
#64346=DIRECTION('',(0.,0.,-1.));
#64347=DIRECTION('',(0.,0.,-1.));
#64348=DIRECTION('center_axis',(0.,0.,1.));
#64349=DIRECTION('ref_axis',(1.,0.,0.));
#64350=DIRECTION('center_axis',(0.,1.,0.));
#64351=DIRECTION('ref_axis',(1.,0.,0.));
#64352=DIRECTION('',(1.,0.,0.));
#64353=DIRECTION('',(0.,0.,-1.));
#64354=DIRECTION('',(1.,0.,0.));
#64355=DIRECTION('',(0.,0.,-1.));
#64356=DIRECTION('',(0.,0.,-1.));
#64357=DIRECTION('',(0.,0.,-1.));
#64358=DIRECTION('center_axis',(-1.,0.,0.));
#64359=DIRECTION('ref_axis',(0.,1.,0.));
#64360=DIRECTION('',(0.,1.,0.));
#64361=DIRECTION('',(0.,0.,-1.));
#64362=DIRECTION('',(0.,1.,0.));
#64363=DIRECTION('',(0.,0.,-1.));
#64364=DIRECTION('',(0.,0.,-1.));
#64365=DIRECTION('center_axis',(-1.,0.,0.));
#64366=DIRECTION('ref_axis',(0.,1.,0.));
#64367=DIRECTION('',(0.,1.,0.));
#64368=DIRECTION('',(0.,0.,-1.));
#64369=DIRECTION('',(0.,1.,0.));
#64370=DIRECTION('center_axis',(0.,-1.,0.));
#64371=DIRECTION('ref_axis',(-1.,0.,0.));
#64372=DIRECTION('',(-1.,0.,0.));
#64373=DIRECTION('',(0.,0.,-1.));
#64374=DIRECTION('',(-1.,0.,0.));
#64375=DIRECTION('center_axis',(1.,0.,0.));
#64376=DIRECTION('ref_axis',(0.,-1.,0.));
#64377=DIRECTION('',(0.,-1.,0.));
#64378=DIRECTION('',(0.,-1.,0.));
#64379=DIRECTION('center_axis',(0.,0.,1.));
#64380=DIRECTION('ref_axis',(1.,0.,0.));
#64381=DIRECTION('center_axis',(0.,0.,1.));
#64382=DIRECTION('ref_axis',(0.,-1.,0.));
#64383=DIRECTION('',(0.,0.,-1.));
#64384=DIRECTION('',(0.,0.,-1.));
#64385=DIRECTION('',(0.,0.,-1.));
#64386=DIRECTION('',(0.,0.,-1.));
#64387=DIRECTION('',(0.,0.,-1.));
#64388=DIRECTION('',(0.,0.,-1.));
#64389=DIRECTION('',(0.,0.,-1.));
#64390=DIRECTION('',(0.,0.,-1.));
#64391=DIRECTION('',(0.,0.,-1.));
#64392=DIRECTION('',(0.,0.,-1.));
#64393=DIRECTION('',(0.,0.,-1.));
#64394=DIRECTION('',(0.,0.,-1.));
#64395=DIRECTION('',(0.,0.,-1.));
#64396=DIRECTION('',(0.,0.,-1.));
#64397=DIRECTION('',(0.,0.,-1.));
#64398=DIRECTION('',(0.,0.,-1.));
#64399=DIRECTION('',(0.,0.,-1.));
#64400=DIRECTION('',(0.,0.,-1.));
#64401=DIRECTION('',(0.,0.,-1.));
#64402=DIRECTION('',(0.,0.,-1.));
#64403=DIRECTION('center_axis',(0.,0.,1.));
#64404=DIRECTION('ref_axis',(1.,0.,0.));
#64405=DIRECTION('center_axis',(0.,0.,1.));
#64406=DIRECTION('ref_axis',(0.,-1.,0.));
#64407=DIRECTION('',(0.,0.,-1.));
#64408=DIRECTION('',(0.,0.,-1.));
#64409=DIRECTION('',(0.,0.,-1.));
#64410=DIRECTION('',(0.,0.,-1.));
#64411=DIRECTION('',(0.,0.,-1.));
#64412=DIRECTION('',(0.,0.,-1.));
#64413=DIRECTION('',(0.,0.,-1.));
#64414=DIRECTION('',(0.,0.,-1.));
#64415=DIRECTION('',(0.,0.,-1.));
#64416=DIRECTION('',(0.,0.,-1.));
#64417=DIRECTION('',(0.,0.,-1.));
#64418=DIRECTION('',(0.,0.,-1.));
#64419=DIRECTION('',(0.,0.,-1.));
#64420=DIRECTION('',(0.,0.,-1.));
#64421=DIRECTION('',(0.,0.,-1.));
#64422=DIRECTION('',(0.,0.,-1.));
#64423=DIRECTION('',(0.,0.,-1.));
#64424=DIRECTION('',(0.,0.,-1.));
#64425=DIRECTION('',(0.,0.,-1.));
#64426=DIRECTION('',(0.,0.,-1.));
#64427=DIRECTION('center_axis',(0.,0.,1.));
#64428=DIRECTION('ref_axis',(1.,0.,0.));
#64429=DIRECTION('center_axis',(0.,1.,0.));
#64430=DIRECTION('ref_axis',(1.,0.,0.));
#64431=DIRECTION('',(1.,0.,0.));
#64432=DIRECTION('',(0.,0.,-1.));
#64433=DIRECTION('',(1.,0.,0.));
#64434=DIRECTION('',(0.,0.,-1.));
#64435=DIRECTION('',(0.,0.,-1.));
#64436=DIRECTION('',(0.,0.,-1.));
#64437=DIRECTION('center_axis',(-1.,0.,0.));
#64438=DIRECTION('ref_axis',(0.,1.,0.));
#64439=DIRECTION('',(0.,1.,0.));
#64440=DIRECTION('',(0.,0.,-1.));
#64441=DIRECTION('',(0.,1.,0.));
#64442=DIRECTION('',(0.,0.,-1.));
#64443=DIRECTION('',(0.,0.,-1.));
#64444=DIRECTION('center_axis',(-1.,0.,0.));
#64445=DIRECTION('ref_axis',(0.,1.,0.));
#64446=DIRECTION('',(0.,1.,0.));
#64447=DIRECTION('',(0.,0.,-1.));
#64448=DIRECTION('',(0.,1.,0.));
#64449=DIRECTION('center_axis',(0.,-1.,0.));
#64450=DIRECTION('ref_axis',(-1.,0.,0.));
#64451=DIRECTION('',(-1.,0.,0.));
#64452=DIRECTION('',(0.,0.,-1.));
#64453=DIRECTION('',(-1.,0.,0.));
#64454=DIRECTION('center_axis',(1.,0.,0.));
#64455=DIRECTION('ref_axis',(0.,-1.,0.));
#64456=DIRECTION('',(0.,-1.,0.));
#64457=DIRECTION('',(0.,-1.,0.));
#64458=DIRECTION('center_axis',(0.,0.,1.));
#64459=DIRECTION('ref_axis',(1.,0.,0.));
#64460=DIRECTION('center_axis',(0.,0.,1.));
#64461=DIRECTION('ref_axis',(0.,-1.,0.));
#64462=DIRECTION('',(0.,0.,-1.));
#64463=DIRECTION('',(0.,0.,-1.));
#64464=DIRECTION('',(0.,0.,-1.));
#64465=DIRECTION('',(0.,0.,-1.));
#64466=DIRECTION('',(0.,0.,-1.));
#64467=DIRECTION('',(0.,0.,-1.));
#64468=DIRECTION('',(0.,0.,-1.));
#64469=DIRECTION('',(0.,0.,-1.));
#64470=DIRECTION('',(0.,0.,-1.));
#64471=DIRECTION('',(0.,0.,-1.));
#64472=DIRECTION('',(0.,0.,-1.));
#64473=DIRECTION('',(0.,0.,-1.));
#64474=DIRECTION('',(0.,0.,-1.));
#64475=DIRECTION('',(0.,0.,-1.));
#64476=DIRECTION('',(0.,0.,-1.));
#64477=DIRECTION('',(0.,0.,-1.));
#64478=DIRECTION('',(0.,0.,-1.));
#64479=DIRECTION('',(0.,0.,-1.));
#64480=DIRECTION('',(0.,0.,-1.));
#64481=DIRECTION('',(0.,0.,-1.));
#64482=DIRECTION('center_axis',(0.,0.,1.));
#64483=DIRECTION('ref_axis',(1.,0.,0.));
#64484=DIRECTION('',(0.,0.,-1.));
#64485=DIRECTION('',(0.,0.,-1.));
#64486=DIRECTION('',(0.,0.,-1.));
#64487=DIRECTION('',(0.,0.,-1.));
#64488=DIRECTION('',(0.,0.,-1.));
#64489=DIRECTION('',(0.,0.,-1.));
#64490=DIRECTION('',(0.,0.,-1.));
#64491=DIRECTION('',(0.,0.,-1.));
#64492=DIRECTION('',(0.,0.,-1.));
#64493=DIRECTION('',(0.,0.,-1.));
#64494=DIRECTION('center_axis',(-0.102165169950561,-0.99476744923071,0.));
#64495=DIRECTION('ref_axis',(-0.99476744923071,0.102165169950561,0.));
#64496=DIRECTION('',(-0.99476744923071,0.102165169950561,0.));
#64497=DIRECTION('',(0.,0.,-1.));
#64498=DIRECTION('',(-0.99476744923071,0.102165169950561,0.));
#64499=DIRECTION('',(0.,0.,-1.));
#64500=DIRECTION('',(0.,0.,-1.));
#64501=DIRECTION('',(0.,0.,-1.));
#64502=DIRECTION('',(0.,0.,-1.));
#64503=DIRECTION('',(0.,0.,-1.));
#64504=DIRECTION('',(0.,0.,-1.));
#64505=DIRECTION('',(0.,0.,-1.));
#64506=DIRECTION('',(0.,0.,-1.));
#64507=DIRECTION('',(0.,0.,-1.));
#64508=DIRECTION('center_axis',(0.,-1.,0.));
#64509=DIRECTION('ref_axis',(-1.,0.,0.));
#64510=DIRECTION('',(-1.,0.,0.));
#64511=DIRECTION('',(0.,0.,-1.));
#64512=DIRECTION('',(-1.,0.,0.));
#64513=DIRECTION('center_axis',(1.,0.,0.));
#64514=DIRECTION('ref_axis',(0.,-1.,0.));
#64515=DIRECTION('',(0.,-1.,0.));
#64516=DIRECTION('',(0.,0.,-1.));
#64517=DIRECTION('',(0.,-1.,0.));
#64518=DIRECTION('center_axis',(0.,1.,0.));
#64519=DIRECTION('ref_axis',(1.,0.,0.));
#64520=DIRECTION('',(1.,0.,0.));
#64521=DIRECTION('',(1.,0.,0.));
#64522=DIRECTION('center_axis',(0.,0.,1.));
#64523=DIRECTION('ref_axis',(1.,0.,0.));
#64524=DIRECTION('center_axis',(0.,0.,1.));
#64525=DIRECTION('ref_axis',(0.,-1.,0.));
#64526=DIRECTION('',(0.,0.,-1.));
#64527=DIRECTION('',(0.,0.,-1.));
#64528=DIRECTION('',(0.,0.,-1.));
#64529=DIRECTION('',(0.,0.,-1.));
#64530=DIRECTION('',(0.,0.,-1.));
#64531=DIRECTION('',(0.,0.,-1.));
#64532=DIRECTION('',(0.,0.,-1.));
#64533=DIRECTION('',(0.,0.,-1.));
#64534=DIRECTION('',(0.,0.,-1.));
#64535=DIRECTION('',(0.,0.,-1.));
#64536=DIRECTION('',(0.,0.,-1.));
#64537=DIRECTION('',(0.,0.,-1.));
#64538=DIRECTION('',(0.,0.,-1.));
#64539=DIRECTION('',(0.,0.,-1.));
#64540=DIRECTION('',(0.,0.,-1.));
#64541=DIRECTION('',(0.,0.,-1.));
#64542=DIRECTION('',(0.,0.,-1.));
#64543=DIRECTION('',(0.,0.,-1.));
#64544=DIRECTION('',(0.,0.,-1.));
#64545=DIRECTION('',(0.,0.,-1.));
#64546=DIRECTION('center_axis',(0.,0.,1.));
#64547=DIRECTION('ref_axis',(1.,0.,0.));
#64548=DIRECTION('',(0.,0.,-1.));
#64549=DIRECTION('',(0.,0.,-1.));
#64550=DIRECTION('',(0.,0.,-1.));
#64551=DIRECTION('',(0.,0.,-1.));
#64552=DIRECTION('',(0.,0.,-1.));
#64553=DIRECTION('',(0.,0.,-1.));
#64554=DIRECTION('',(0.,0.,-1.));
#64555=DIRECTION('',(0.,0.,-1.));
#64556=DIRECTION('',(0.,0.,-1.));
#64557=DIRECTION('',(0.,0.,-1.));
#64558=DIRECTION('',(0.,0.,-1.));
#64559=DIRECTION('',(0.,0.,-1.));
#64560=DIRECTION('',(0.,0.,-1.));
#64561=DIRECTION('center_axis',(-0.175033346417238,-0.984562505705952,0.));
#64562=DIRECTION('ref_axis',(-0.984562505705952,0.175033346417238,0.));
#64563=DIRECTION('',(-0.984562505705952,0.175033346417238,0.));
#64564=DIRECTION('',(0.,0.,-1.));
#64565=DIRECTION('',(-0.984562505705952,0.175033346417238,0.));
#64566=DIRECTION('',(0.,0.,-1.));
#64567=DIRECTION('',(0.,0.,-1.));
#64568=DIRECTION('',(0.,0.,-1.));
#64569=DIRECTION('',(0.,0.,-1.));
#64570=DIRECTION('',(0.,0.,-1.));
#64571=DIRECTION('',(0.,0.,-1.));
#64572=DIRECTION('',(0.,0.,-1.));
#64573=DIRECTION('center_axis',(-0.992083480553514,0.125580124274607,0.));
#64574=DIRECTION('ref_axis',(0.125580124274607,0.992083480553514,0.));
#64575=DIRECTION('',(0.125580124274607,0.992083480553514,0.));
#64576=DIRECTION('',(0.,0.,-1.));
#64577=DIRECTION('',(0.125580124274607,0.992083480553514,0.));
#64578=DIRECTION('',(0.,0.,-1.));
#64579=DIRECTION('',(0.,0.,-1.));
#64580=DIRECTION('',(0.,0.,-1.));
#64581=DIRECTION('',(0.,0.,-1.));
#64582=DIRECTION('',(0.,0.,-1.));
#64583=DIRECTION('',(0.,0.,-1.));
#64584=DIRECTION('',(0.,0.,-1.));
#64585=DIRECTION('center_axis',(-0.132163863358704,0.991227881580266,0.));
#64586=DIRECTION('ref_axis',(0.991227881580266,0.132163863358704,0.));
#64587=DIRECTION('',(0.991227881580266,0.132163863358704,0.));
#64588=DIRECTION('',(0.,0.,-1.));
#64589=DIRECTION('',(0.991227881580266,0.132163863358704,0.));
#64590=DIRECTION('center_axis',(0.,0.,1.));
#64591=DIRECTION('ref_axis',(1.,0.,0.));
#64592=DIRECTION('center_axis',(0.,0.,1.));
#64593=DIRECTION('ref_axis',(0.,-1.,0.));
#64594=DIRECTION('',(0.,0.,-1.));
#64595=DIRECTION('',(0.,0.,-1.));
#64596=DIRECTION('',(0.,0.,-1.));
#64597=DIRECTION('',(0.,0.,-1.));
#64598=DIRECTION('',(0.,0.,-1.));
#64599=DIRECTION('',(0.,0.,-1.));
#64600=DIRECTION('',(0.,0.,-1.));
#64601=DIRECTION('',(0.,0.,-1.));
#64602=DIRECTION('',(0.,0.,-1.));
#64603=DIRECTION('',(0.,0.,-1.));
#64604=DIRECTION('',(0.,0.,-1.));
#64605=DIRECTION('',(0.,0.,-1.));
#64606=DIRECTION('',(0.,0.,-1.));
#64607=DIRECTION('',(0.,0.,-1.));
#64608=DIRECTION('',(0.,0.,-1.));
#64609=DIRECTION('',(0.,0.,-1.));
#64610=DIRECTION('',(0.,0.,-1.));
#64611=DIRECTION('',(0.,0.,-1.));
#64612=DIRECTION('',(0.,0.,-1.));
#64613=DIRECTION('',(0.,0.,-1.));
#64614=DIRECTION('center_axis',(0.,0.,1.));
#64615=DIRECTION('ref_axis',(1.,0.,0.));
#64616=DIRECTION('center_axis',(0.821386116423605,-0.570372551712079,0.));
#64617=DIRECTION('ref_axis',(-0.570372551712079,-0.821386116423605,0.));
#64618=DIRECTION('',(-0.570372551712079,-0.821386116423605,0.));
#64619=DIRECTION('',(0.,0.,-1.));
#64620=DIRECTION('',(-0.570372551712079,-0.821386116423605,0.));
#64621=DIRECTION('',(0.,0.,-1.));
#64622=DIRECTION('center_axis',(-1.,0.,0.));
#64623=DIRECTION('ref_axis',(0.,1.,0.));
#64624=DIRECTION('',(0.,1.,0.));
#64625=DIRECTION('',(0.,0.,-1.));
#64626=DIRECTION('',(0.,1.,0.));
#64627=DIRECTION('center_axis',(0.,1.,0.));
#64628=DIRECTION('ref_axis',(1.,0.,0.));
#64629=DIRECTION('',(1.,0.,0.));
#64630=DIRECTION('',(1.,0.,0.));
#64631=DIRECTION('center_axis',(1.,0.,0.));
#64632=DIRECTION('ref_axis',(0.,-1.,0.));
#64633=DIRECTION('',(0.,-1.,0.));
#64634=DIRECTION('',(0.,0.,-1.));
#64635=DIRECTION('',(0.,-1.,0.));
#64636=DIRECTION('',(0.,0.,-1.));
#64637=DIRECTION('center_axis',(0.,-1.,0.));
#64638=DIRECTION('ref_axis',(-1.,0.,0.));
#64639=DIRECTION('',(-1.,0.,0.));
#64640=DIRECTION('',(0.,0.,-1.));
#64641=DIRECTION('',(-1.,0.,0.));
#64642=DIRECTION('center_axis',(1.,0.,0.));
#64643=DIRECTION('ref_axis',(0.,-1.,0.));
#64644=DIRECTION('',(0.,-1.,0.));
#64645=DIRECTION('',(0.,0.,-1.));
#64646=DIRECTION('',(0.,-1.,0.));
#64647=DIRECTION('center_axis',(0.,1.,0.));
#64648=DIRECTION('ref_axis',(1.,0.,0.));
#64649=DIRECTION('',(1.,0.,0.));
#64650=DIRECTION('',(0.,0.,-1.));
#64651=DIRECTION('',(1.,0.,0.));
#64652=DIRECTION('center_axis',(1.,0.,0.));
#64653=DIRECTION('ref_axis',(0.,-1.,0.));
#64654=DIRECTION('',(0.,-1.,0.));
#64655=DIRECTION('',(0.,0.,-1.));
#64656=DIRECTION('',(0.,-1.,0.));
#64657=DIRECTION('center_axis',(0.,1.,0.));
#64658=DIRECTION('ref_axis',(1.,0.,0.));
#64659=DIRECTION('',(1.,0.,0.));
#64660=DIRECTION('',(0.,0.,-1.));
#64661=DIRECTION('',(1.,0.,0.));
#64662=DIRECTION('center_axis',(-0.817611346967032,0.575770514450641,0.));
#64663=DIRECTION('ref_axis',(0.575770514450641,0.817611346967032,0.));
#64664=DIRECTION('',(0.575770514450641,0.817611346967032,0.));
#64665=DIRECTION('',(0.,0.,-1.));
#64666=DIRECTION('',(0.575770514450641,0.817611346967032,0.));
#64667=DIRECTION('center_axis',(-1.,0.,0.));
#64668=DIRECTION('ref_axis',(0.,1.,0.));
#64669=DIRECTION('',(0.,1.,0.));
#64670=DIRECTION('',(0.,0.,-1.));
#64671=DIRECTION('',(0.,1.,0.));
#64672=DIRECTION('center_axis',(0.,-1.,0.));
#64673=DIRECTION('ref_axis',(-1.,0.,0.));
#64674=DIRECTION('',(-1.,0.,0.));
#64675=DIRECTION('',(0.,0.,-1.));
#64676=DIRECTION('',(-1.,0.,0.));
#64677=DIRECTION('center_axis',(-1.,0.,0.));
#64678=DIRECTION('ref_axis',(0.,1.,0.));
#64679=DIRECTION('',(0.,1.,0.));
#64680=DIRECTION('',(0.,0.,-1.));
#64681=DIRECTION('',(0.,1.,0.));
#64682=DIRECTION('center_axis',(0.,-1.,0.));
#64683=DIRECTION('ref_axis',(-1.,0.,0.));
#64684=DIRECTION('',(-1.,0.,0.));
#64685=DIRECTION('',(-1.,0.,0.));
#64686=DIRECTION('center_axis',(0.,0.,-1.));
#64687=DIRECTION('ref_axis',(-1.,0.,0.));
#64688=DIRECTION('center_axis',(0.,0.,1.));
#64689=DIRECTION('ref_axis',(0.,-1.,0.));
#64690=DIRECTION('center_axis',(0.,0.,1.));
#64691=DIRECTION('ref_axis',(0.,-1.,0.));
#64692=DIRECTION('',(0.,0.,-1.));
#64693=DIRECTION('',(0.,0.,-1.));
#64694=DIRECTION('',(0.,0.,-1.));
#64695=DIRECTION('',(0.,0.,-1.));
#64696=DIRECTION('',(0.,0.,-1.));
#64697=DIRECTION('',(0.,0.,-1.));
#64698=DIRECTION('',(0.,0.,-1.));
#64699=DIRECTION('',(0.,0.,-1.));
#64700=DIRECTION('',(0.,0.,-1.));
#64701=DIRECTION('',(0.,0.,-1.));
#64702=DIRECTION('',(0.,0.,-1.));
#64703=DIRECTION('',(0.,0.,-1.));
#64704=DIRECTION('',(0.,0.,-1.));
#64705=DIRECTION('',(0.,0.,-1.));
#64706=DIRECTION('',(0.,0.,-1.));
#64707=DIRECTION('',(0.,0.,-1.));
#64708=DIRECTION('',(0.,0.,-1.));
#64709=DIRECTION('',(0.,0.,-1.));
#64710=DIRECTION('',(0.,0.,-1.));
#64711=DIRECTION('',(0.,0.,-1.));
#64712=DIRECTION('center_axis',(0.,0.,1.));
#64713=DIRECTION('ref_axis',(1.,0.,0.));
#64714=DIRECTION('',(0.,0.,-1.));
#64715=DIRECTION('',(0.,0.,-1.));
#64716=DIRECTION('',(0.,0.,-1.));
#64717=DIRECTION('',(0.,0.,-1.));
#64718=DIRECTION('',(0.,0.,-1.));
#64719=DIRECTION('',(0.,0.,-1.));
#64720=DIRECTION('',(0.,0.,-1.));
#64721=DIRECTION('center_axis',(0.980484873509324,-0.196594539139329,0.));
#64722=DIRECTION('ref_axis',(-0.196594539139329,-0.980484873509324,0.));
#64723=DIRECTION('',(-0.196594539139329,-0.980484873509324,0.));
#64724=DIRECTION('',(0.,0.,-1.));
#64725=DIRECTION('',(-0.196594539139329,-0.980484873509324,0.));
#64726=DIRECTION('center_axis',(0.,-1.,0.));
#64727=DIRECTION('ref_axis',(-1.,0.,0.));
#64728=DIRECTION('',(-1.,0.,0.));
#64729=DIRECTION('',(0.,0.,-1.));
#64730=DIRECTION('',(-1.,0.,0.));
#64731=DIRECTION('center_axis',(1.,0.,0.));
#64732=DIRECTION('ref_axis',(0.,-1.,0.));
#64733=DIRECTION('',(0.,-1.,0.));
#64734=DIRECTION('',(0.,0.,-1.));
#64735=DIRECTION('',(0.,-1.,0.));
#64736=DIRECTION('center_axis',(0.,1.,0.));
#64737=DIRECTION('ref_axis',(1.,0.,0.));
#64738=DIRECTION('',(1.,0.,0.));
#64739=DIRECTION('',(0.,0.,-1.));
#64740=DIRECTION('',(1.,0.,0.));
#64741=DIRECTION('center_axis',(-0.982679588991295,0.185312777163097,0.));
#64742=DIRECTION('ref_axis',(0.185312777163097,0.982679588991295,0.));
#64743=DIRECTION('',(0.185312777163097,0.982679588991295,0.));
#64744=DIRECTION('',(0.,0.,-1.));
#64745=DIRECTION('',(0.185312777163097,0.982679588991295,0.));
#64746=DIRECTION('center_axis',(-0.129088379836863,-0.991633092525201,0.));
#64747=DIRECTION('ref_axis',(-0.991633092525201,0.129088379836863,0.));
#64748=DIRECTION('',(-0.991633092525201,0.129088379836863,0.));
#64749=DIRECTION('',(0.,0.,-1.));
#64750=DIRECTION('',(-0.991633092525201,0.129088379836863,0.));
#64751=DIRECTION('',(0.,0.,-1.));
#64752=DIRECTION('',(0.,0.,-1.));
#64753=DIRECTION('',(0.,0.,-1.));
#64754=DIRECTION('',(0.,0.,-1.));
#64755=DIRECTION('',(0.,0.,-1.));
#64756=DIRECTION('',(0.,0.,-1.));
#64757=DIRECTION('',(0.,0.,-1.));
#64758=DIRECTION('',(0.,0.,-1.));
#64759=DIRECTION('center_axis',(-0.0843540635911639,0.99643584437517,0.));
#64760=DIRECTION('ref_axis',(0.99643584437517,0.0843540635911639,0.));
#64761=DIRECTION('',(0.99643584437517,0.0843540635911639,0.));
#64762=DIRECTION('',(0.,0.,-1.));
#64763=DIRECTION('',(0.99643584437517,0.0843540635911639,0.));
#64764=DIRECTION('center_axis',(0.,0.,1.));
#64765=DIRECTION('ref_axis',(1.,0.,0.));
#64766=DIRECTION('center_axis',(0.,0.,1.));
#64767=DIRECTION('ref_axis',(0.,-1.,0.));
#64768=DIRECTION('',(0.,0.,-1.));
#64769=DIRECTION('',(0.,0.,-1.));
#64770=DIRECTION('',(0.,0.,-1.));
#64771=DIRECTION('',(0.,0.,-1.));
#64772=DIRECTION('',(0.,0.,-1.));
#64773=DIRECTION('',(0.,0.,-1.));
#64774=DIRECTION('',(0.,0.,-1.));
#64775=DIRECTION('',(0.,0.,-1.));
#64776=DIRECTION('',(0.,0.,-1.));
#64777=DIRECTION('',(0.,0.,-1.));
#64778=DIRECTION('',(0.,0.,-1.));
#64779=DIRECTION('',(0.,0.,-1.));
#64780=DIRECTION('',(0.,0.,-1.));
#64781=DIRECTION('',(0.,0.,-1.));
#64782=DIRECTION('',(0.,0.,-1.));
#64783=DIRECTION('',(0.,0.,-1.));
#64784=DIRECTION('',(0.,0.,-1.));
#64785=DIRECTION('',(0.,0.,-1.));
#64786=DIRECTION('',(0.,0.,-1.));
#64787=DIRECTION('',(0.,0.,-1.));
#64788=DIRECTION('center_axis',(0.,0.,1.));
#64789=DIRECTION('ref_axis',(1.,0.,0.));
#64790=DIRECTION('',(0.,0.,-1.));
#64791=DIRECTION('',(0.,0.,-1.));
#64792=DIRECTION('',(0.,0.,-1.));
#64793=DIRECTION('',(0.,0.,-1.));
#64794=DIRECTION('',(0.,0.,-1.));
#64795=DIRECTION('',(0.,0.,-1.));
#64796=DIRECTION('',(0.,0.,-1.));
#64797=DIRECTION('',(0.,0.,-1.));
#64798=DIRECTION('',(0.,0.,-1.));
#64799=DIRECTION('',(0.,0.,-1.));
#64800=DIRECTION('',(0.,0.,-1.));
#64801=DIRECTION('',(0.,0.,-1.));
#64802=DIRECTION('',(0.,0.,-1.));
#64803=DIRECTION('',(0.,0.,-1.));
#64804=DIRECTION('',(0.,0.,-1.));
#64805=DIRECTION('',(0.,0.,-1.));
#64806=DIRECTION('',(0.,0.,-1.));
#64807=DIRECTION('',(0.,0.,-1.));
#64808=DIRECTION('',(0.,0.,-1.));
#64809=DIRECTION('',(0.,0.,-1.));
#64810=DIRECTION('',(0.,0.,-1.));
#64811=DIRECTION('',(0.,0.,-1.));
#64812=DIRECTION('',(0.,0.,-1.));
#64813=DIRECTION('',(0.,0.,-1.));
#64814=DIRECTION('',(0.,0.,-1.));
#64815=DIRECTION('',(0.,0.,-1.));
#64816=DIRECTION('',(0.,0.,-1.));
#64817=DIRECTION('center_axis',(0.0779743449792121,-0.99695536586402,0.));
#64818=DIRECTION('ref_axis',(-0.99695536586402,-0.0779743449792121,0.));
#64819=DIRECTION('',(-0.99695536586402,-0.0779743449792121,0.));
#64820=DIRECTION('',(0.,0.,-1.));
#64821=DIRECTION('',(-0.99695536586402,-0.0779743449792121,0.));
#64822=DIRECTION('center_axis',(0.,0.,1.));
#64823=DIRECTION('ref_axis',(1.,0.,0.));
#64824=DIRECTION('center_axis',(0.,0.,1.));
#64825=DIRECTION('ref_axis',(0.,-1.,0.));
#64826=DIRECTION('center_axis',(0.,0.,1.));
#64827=DIRECTION('ref_axis',(0.,-1.,0.));
#64828=DIRECTION('',(0.,0.,-1.));
#64829=DIRECTION('',(0.,0.,-1.));
#64830=DIRECTION('',(0.,0.,-1.));
#64831=DIRECTION('',(0.,0.,-1.));
#64832=DIRECTION('',(0.,0.,-1.));
#64833=DIRECTION('',(0.,0.,-1.));
#64834=DIRECTION('',(0.,0.,-1.));
#64835=DIRECTION('',(0.,0.,-1.));
#64836=DIRECTION('',(0.,0.,-1.));
#64837=DIRECTION('',(0.,0.,-1.));
#64838=DIRECTION('',(0.,0.,-1.));
#64839=DIRECTION('',(0.,0.,-1.));
#64840=DIRECTION('',(0.,0.,-1.));
#64841=DIRECTION('',(0.,0.,-1.));
#64842=DIRECTION('',(0.,0.,-1.));
#64843=DIRECTION('',(0.,0.,-1.));
#64844=DIRECTION('',(0.,0.,-1.));
#64845=DIRECTION('',(0.,0.,-1.));
#64846=DIRECTION('',(0.,0.,-1.));
#64847=DIRECTION('',(0.,0.,-1.));
#64848=DIRECTION('center_axis',(0.,0.,1.));
#64849=DIRECTION('ref_axis',(1.,0.,0.));
#64850=DIRECTION('',(0.,0.,-1.));
#64851=DIRECTION('',(0.,0.,-1.));
#64852=DIRECTION('',(0.,0.,-1.));
#64853=DIRECTION('',(0.,0.,-1.));
#64854=DIRECTION('center_axis',(0.,-1.,0.));
#64855=DIRECTION('ref_axis',(-1.,0.,0.));
#64856=DIRECTION('',(-1.,0.,0.));
#64857=DIRECTION('',(0.,0.,-1.));
#64858=DIRECTION('',(-1.,0.,0.));
#64859=DIRECTION('',(0.,0.,-1.));
#64860=DIRECTION('',(0.,0.,-1.));
#64861=DIRECTION('',(0.,0.,-1.));
#64862=DIRECTION('center_axis',(1.,0.,0.));
#64863=DIRECTION('ref_axis',(0.,-1.,0.));
#64864=DIRECTION('',(0.,-1.,0.));
#64865=DIRECTION('',(0.,0.,-1.));
#64866=DIRECTION('',(0.,-1.,0.));
#64867=DIRECTION('center_axis',(0.,1.,0.));
#64868=DIRECTION('ref_axis',(1.,0.,0.));
#64869=DIRECTION('',(1.,0.,0.));
#64870=DIRECTION('',(0.,0.,-1.));
#64871=DIRECTION('',(1.,0.,0.));
#64872=DIRECTION('center_axis',(-1.,0.,0.));
#64873=DIRECTION('ref_axis',(0.,1.,0.));
#64874=DIRECTION('',(0.,1.,0.));
#64875=DIRECTION('',(0.,0.,-1.));
#64876=DIRECTION('',(0.,1.,0.));
#64877=DIRECTION('center_axis',(0.,-1.,0.));
#64878=DIRECTION('ref_axis',(-1.,0.,0.));
#64879=DIRECTION('',(-1.,0.,0.));
#64880=DIRECTION('',(-1.,0.,0.));
#64881=DIRECTION('center_axis',(0.,0.,1.));
#64882=DIRECTION('ref_axis',(1.,0.,0.));
#64883=DIRECTION('center_axis',(0.,0.,1.));
#64884=DIRECTION('ref_axis',(0.,-1.,0.));
#64885=DIRECTION('',(0.,0.,-1.));
#64886=DIRECTION('',(0.,0.,-1.));
#64887=DIRECTION('',(0.,0.,-1.));
#64888=DIRECTION('',(0.,0.,-1.));
#64889=DIRECTION('',(0.,0.,-1.));
#64890=DIRECTION('',(0.,0.,-1.));
#64891=DIRECTION('',(0.,0.,-1.));
#64892=DIRECTION('',(0.,0.,-1.));
#64893=DIRECTION('',(0.,0.,-1.));
#64894=DIRECTION('',(0.,0.,-1.));
#64895=DIRECTION('',(0.,0.,-1.));
#64896=DIRECTION('',(0.,0.,-1.));
#64897=DIRECTION('',(0.,0.,-1.));
#64898=DIRECTION('',(0.,0.,-1.));
#64899=DIRECTION('',(0.,0.,-1.));
#64900=DIRECTION('',(0.,0.,-1.));
#64901=DIRECTION('',(0.,0.,-1.));
#64902=DIRECTION('',(0.,0.,-1.));
#64903=DIRECTION('',(0.,0.,-1.));
#64904=DIRECTION('',(0.,0.,-1.));
#64905=DIRECTION('center_axis',(0.,0.,1.));
#64906=DIRECTION('ref_axis',(1.,0.,0.));
#64907=DIRECTION('',(0.,0.,-1.));
#64908=DIRECTION('',(0.,0.,-1.));
#64909=DIRECTION('',(0.,0.,-1.));
#64910=DIRECTION('',(0.,0.,-1.));
#64911=DIRECTION('',(0.,0.,-1.));
#64912=DIRECTION('',(0.,0.,-1.));
#64913=DIRECTION('',(0.,0.,-1.));
#64914=DIRECTION('',(0.,0.,-1.));
#64915=DIRECTION('',(0.,0.,-1.));
#64916=DIRECTION('',(0.,0.,-1.));
#64917=DIRECTION('',(0.,0.,-1.));
#64918=DIRECTION('',(0.,0.,-1.));
#64919=DIRECTION('',(0.,0.,-1.));
#64920=DIRECTION('',(0.,0.,-1.));
#64921=DIRECTION('',(0.,0.,-1.));
#64922=DIRECTION('',(0.,0.,-1.));
#64923=DIRECTION('',(0.,0.,-1.));
#64924=DIRECTION('',(0.,0.,-1.));
#64925=DIRECTION('',(0.,0.,-1.));
#64926=DIRECTION('',(0.,0.,-1.));
#64927=DIRECTION('',(0.,0.,-1.));
#64928=DIRECTION('',(0.,0.,-1.));
#64929=DIRECTION('',(0.,0.,-1.));
#64930=DIRECTION('',(0.,0.,-1.));
#64931=DIRECTION('',(0.,0.,-1.));
#64932=DIRECTION('',(0.,0.,-1.));
#64933=DIRECTION('',(0.,0.,-1.));
#64934=DIRECTION('',(0.,0.,-1.));
#64935=DIRECTION('',(0.,0.,-1.));
#64936=DIRECTION('',(0.,0.,-1.));
#64937=DIRECTION('',(0.,0.,-1.));
#64938=DIRECTION('',(0.,0.,-1.));
#64939=DIRECTION('',(0.,0.,-1.));
#64940=DIRECTION('center_axis',(0.,0.,1.));
#64941=DIRECTION('ref_axis',(1.,0.,0.));
#64942=DIRECTION('center_axis',(0.,0.,1.));
#64943=DIRECTION('ref_axis',(0.,-1.,0.));
#64944=DIRECTION('center_axis',(0.,0.,1.));
#64945=DIRECTION('ref_axis',(0.,-1.,0.));
#64946=DIRECTION('center_axis',(0.,0.,1.));
#64947=DIRECTION('ref_axis',(0.,-1.,0.));
#64948=DIRECTION('',(0.,0.,-1.));
#64949=DIRECTION('',(0.,0.,-1.));
#64950=DIRECTION('',(0.,0.,-1.));
#64951=DIRECTION('',(0.,0.,-1.));
#64952=DIRECTION('',(0.,0.,-1.));
#64953=DIRECTION('',(0.,0.,-1.));
#64954=DIRECTION('',(0.,0.,-1.));
#64955=DIRECTION('',(0.,0.,-1.));
#64956=DIRECTION('',(0.,0.,-1.));
#64957=DIRECTION('',(0.,0.,-1.));
#64958=DIRECTION('',(0.,0.,-1.));
#64959=DIRECTION('',(0.,0.,-1.));
#64960=DIRECTION('',(0.,0.,-1.));
#64961=DIRECTION('',(0.,0.,-1.));
#64962=DIRECTION('',(0.,0.,-1.));
#64963=DIRECTION('',(0.,0.,-1.));
#64964=DIRECTION('',(0.,0.,-1.));
#64965=DIRECTION('',(0.,0.,-1.));
#64966=DIRECTION('',(0.,0.,-1.));
#64967=DIRECTION('',(0.,0.,-1.));
#64968=DIRECTION('center_axis',(0.,0.,1.));
#64969=DIRECTION('ref_axis',(1.,0.,0.));
#64970=DIRECTION('',(0.,0.,-1.));
#64971=DIRECTION('',(0.,0.,-1.));
#64972=DIRECTION('',(0.,0.,-1.));
#64973=DIRECTION('',(0.,0.,-1.));
#64974=DIRECTION('',(0.,0.,-1.));
#64975=DIRECTION('',(0.,0.,-1.));
#64976=DIRECTION('',(0.,0.,-1.));
#64977=DIRECTION('',(0.,0.,-1.));
#64978=DIRECTION('',(0.,0.,-1.));
#64979=DIRECTION('',(0.,0.,-1.));
#64980=DIRECTION('',(0.,0.,-1.));
#64981=DIRECTION('',(0.,0.,-1.));
#64982=DIRECTION('',(0.,0.,-1.));
#64983=DIRECTION('',(0.,0.,-1.));
#64984=DIRECTION('',(0.,0.,-1.));
#64985=DIRECTION('',(0.,0.,-1.));
#64986=DIRECTION('',(0.,0.,-1.));
#64987=DIRECTION('',(0.,0.,-1.));
#64988=DIRECTION('',(0.,0.,-1.));
#64989=DIRECTION('',(0.,0.,-1.));
#64990=DIRECTION('',(0.,0.,-1.));
#64991=DIRECTION('',(0.,0.,-1.));
#64992=DIRECTION('',(0.,0.,-1.));
#64993=DIRECTION('',(0.,0.,-1.));
#64994=DIRECTION('',(0.,0.,-1.));
#64995=DIRECTION('',(0.,0.,-1.));
#64996=DIRECTION('',(0.,0.,-1.));
#64997=DIRECTION('',(0.,0.,-1.));
#64998=DIRECTION('',(0.,0.,-1.));
#64999=DIRECTION('center_axis',(-0.0920922327212455,0.995750481130899,0.));
#65000=DIRECTION('ref_axis',(0.995750481130899,0.0920922327212455,0.));
#65001=DIRECTION('',(0.995750481130899,0.0920922327212455,0.));
#65002=DIRECTION('',(0.,0.,-1.));
#65003=DIRECTION('',(0.995750481130898,0.0920922327212455,0.));
#65004=DIRECTION('center_axis',(0.,0.,1.));
#65005=DIRECTION('ref_axis',(1.,0.,0.));
#65006=DIRECTION('center_axis',(0.,0.,1.));
#65007=DIRECTION('ref_axis',(0.,-1.,0.));
#65008=DIRECTION('center_axis',(0.,0.,1.));
#65009=DIRECTION('ref_axis',(0.,-1.,0.));
#65010=DIRECTION('center_axis',(0.,-1.,0.));
#65011=DIRECTION('ref_axis',(-1.,0.,0.));
#65012=DIRECTION('',(-1.,0.,0.));
#65013=DIRECTION('',(0.,0.,-1.));
#65014=DIRECTION('',(-1.,0.,0.));
#65015=DIRECTION('',(0.,0.,-1.));
#65016=DIRECTION('center_axis',(1.,0.,0.));
#65017=DIRECTION('ref_axis',(0.,-1.,0.));
#65018=DIRECTION('',(0.,-1.,0.));
#65019=DIRECTION('',(0.,0.,-1.));
#65020=DIRECTION('',(0.,-1.,0.));
#65021=DIRECTION('center_axis',(0.,1.,0.));
#65022=DIRECTION('ref_axis',(1.,0.,0.));
#65023=DIRECTION('',(1.,0.,0.));
#65024=DIRECTION('',(0.,0.,-1.));
#65025=DIRECTION('',(1.,0.,0.));
#65026=DIRECTION('center_axis',(-1.,0.,0.));
#65027=DIRECTION('ref_axis',(0.,1.,0.));
#65028=DIRECTION('',(0.,1.,0.));
#65029=DIRECTION('',(0.,1.,0.));
#65030=DIRECTION('center_axis',(0.,0.,-1.));
#65031=DIRECTION('ref_axis',(-1.,0.,0.));
#65032=DIRECTION('center_axis',(0.,-1.,0.));
#65033=DIRECTION('ref_axis',(-1.,0.,0.));
#65034=DIRECTION('',(-1.,0.,0.));
#65035=DIRECTION('',(0.,0.,-1.));
#65036=DIRECTION('',(-1.,0.,0.));
#65037=DIRECTION('',(0.,0.,-1.));
#65038=DIRECTION('center_axis',(1.,0.,0.));
#65039=DIRECTION('ref_axis',(0.,-1.,0.));
#65040=DIRECTION('',(0.,-1.,0.));
#65041=DIRECTION('',(0.,0.,-1.));
#65042=DIRECTION('',(0.,-1.,0.));
#65043=DIRECTION('center_axis',(0.,1.,0.));
#65044=DIRECTION('ref_axis',(1.,0.,0.));
#65045=DIRECTION('',(1.,0.,0.));
#65046=DIRECTION('',(0.,0.,-1.));
#65047=DIRECTION('',(1.,0.,0.));
#65048=DIRECTION('center_axis',(-1.,0.,0.));
#65049=DIRECTION('ref_axis',(0.,1.,0.));
#65050=DIRECTION('',(0.,1.,0.));
#65051=DIRECTION('',(0.,1.,0.));
#65052=DIRECTION('center_axis',(0.,0.,-1.));
#65053=DIRECTION('ref_axis',(-1.,0.,0.));
#65054=DIRECTION('center_axis',(0.,-1.,0.));
#65055=DIRECTION('ref_axis',(-1.,0.,0.));
#65056=DIRECTION('',(-1.,0.,0.));
#65057=DIRECTION('',(0.,0.,-1.));
#65058=DIRECTION('',(-1.,0.,0.));
#65059=DIRECTION('',(0.,0.,-1.));
#65060=DIRECTION('center_axis',(1.,0.,0.));
#65061=DIRECTION('ref_axis',(0.,-1.,0.));
#65062=DIRECTION('',(0.,-1.,0.));
#65063=DIRECTION('',(0.,0.,-1.));
#65064=DIRECTION('',(0.,-1.,0.));
#65065=DIRECTION('center_axis',(0.,1.,0.));
#65066=DIRECTION('ref_axis',(1.,0.,0.));
#65067=DIRECTION('',(1.,0.,0.));
#65068=DIRECTION('',(0.,0.,-1.));
#65069=DIRECTION('',(1.,0.,0.));
#65070=DIRECTION('center_axis',(-1.,0.,0.));
#65071=DIRECTION('ref_axis',(0.,1.,0.));
#65072=DIRECTION('',(0.,1.,0.));
#65073=DIRECTION('',(0.,1.,0.));
#65074=DIRECTION('center_axis',(0.,0.,-1.));
#65075=DIRECTION('ref_axis',(-1.,0.,0.));
#65076=DIRECTION('center_axis',(0.,-1.,0.));
#65077=DIRECTION('ref_axis',(-1.,0.,0.));
#65078=DIRECTION('',(-1.,0.,0.));
#65079=DIRECTION('',(0.,0.,-1.));
#65080=DIRECTION('',(-1.,0.,0.));
#65081=DIRECTION('',(0.,0.,-1.));
#65082=DIRECTION('center_axis',(1.,0.,0.));
#65083=DIRECTION('ref_axis',(0.,-1.,0.));
#65084=DIRECTION('',(0.,-1.,0.));
#65085=DIRECTION('',(0.,0.,-1.));
#65086=DIRECTION('',(0.,-1.,0.));
#65087=DIRECTION('center_axis',(0.,1.,0.));
#65088=DIRECTION('ref_axis',(1.,0.,0.));
#65089=DIRECTION('',(1.,0.,0.));
#65090=DIRECTION('',(0.,0.,-1.));
#65091=DIRECTION('',(1.,0.,0.));
#65092=DIRECTION('center_axis',(-1.,0.,0.));
#65093=DIRECTION('ref_axis',(0.,1.,0.));
#65094=DIRECTION('',(0.,1.,0.));
#65095=DIRECTION('',(0.,1.,0.));
#65096=DIRECTION('center_axis',(0.,0.,-1.));
#65097=DIRECTION('ref_axis',(-1.,0.,0.));
#65098=DIRECTION('center_axis',(0.,-1.,0.));
#65099=DIRECTION('ref_axis',(-1.,0.,0.));
#65100=DIRECTION('',(-1.,0.,0.));
#65101=DIRECTION('',(0.,0.,-1.));
#65102=DIRECTION('',(-1.,0.,0.));
#65103=DIRECTION('',(0.,0.,-1.));
#65104=DIRECTION('center_axis',(1.,0.,0.));
#65105=DIRECTION('ref_axis',(0.,-1.,0.));
#65106=DIRECTION('',(0.,-1.,0.));
#65107=DIRECTION('',(0.,0.,-1.));
#65108=DIRECTION('',(0.,-1.,0.));
#65109=DIRECTION('center_axis',(0.,1.,0.));
#65110=DIRECTION('ref_axis',(1.,0.,0.));
#65111=DIRECTION('',(1.,0.,0.));
#65112=DIRECTION('',(0.,0.,-1.));
#65113=DIRECTION('',(1.,0.,0.));
#65114=DIRECTION('center_axis',(-1.,0.,0.));
#65115=DIRECTION('ref_axis',(0.,1.,0.));
#65116=DIRECTION('',(0.,1.,0.));
#65117=DIRECTION('',(0.,1.,0.));
#65118=DIRECTION('center_axis',(0.,0.,-1.));
#65119=DIRECTION('ref_axis',(-1.,0.,0.));
#65120=DIRECTION('center_axis',(0.,-1.,0.));
#65121=DIRECTION('ref_axis',(-1.,0.,0.));
#65122=DIRECTION('',(-1.,0.,0.));
#65123=DIRECTION('',(0.,0.,-1.));
#65124=DIRECTION('',(-1.,0.,0.));
#65125=DIRECTION('',(0.,0.,-1.));
#65126=DIRECTION('center_axis',(1.,0.,0.));
#65127=DIRECTION('ref_axis',(0.,-1.,0.));
#65128=DIRECTION('',(0.,-1.,0.));
#65129=DIRECTION('',(0.,0.,-1.));
#65130=DIRECTION('',(0.,-1.,0.));
#65131=DIRECTION('center_axis',(0.,1.,0.));
#65132=DIRECTION('ref_axis',(1.,0.,0.));
#65133=DIRECTION('',(1.,0.,0.));
#65134=DIRECTION('',(0.,0.,-1.));
#65135=DIRECTION('',(1.,0.,0.));
#65136=DIRECTION('center_axis',(-1.,0.,0.));
#65137=DIRECTION('ref_axis',(0.,1.,0.));
#65138=DIRECTION('',(0.,1.,0.));
#65139=DIRECTION('',(0.,1.,0.));
#65140=DIRECTION('center_axis',(0.,0.,-1.));
#65141=DIRECTION('ref_axis',(-1.,0.,0.));
#65142=DIRECTION('center_axis',(0.,-1.,0.));
#65143=DIRECTION('ref_axis',(-1.,0.,0.));
#65144=DIRECTION('',(-1.,0.,0.));
#65145=DIRECTION('',(0.,0.,-1.));
#65146=DIRECTION('',(-1.,0.,0.));
#65147=DIRECTION('',(0.,0.,-1.));
#65148=DIRECTION('center_axis',(1.,0.,0.));
#65149=DIRECTION('ref_axis',(0.,-1.,0.));
#65150=DIRECTION('',(0.,-1.,0.));
#65151=DIRECTION('',(0.,0.,-1.));
#65152=DIRECTION('',(0.,-1.,0.));
#65153=DIRECTION('center_axis',(0.,1.,0.));
#65154=DIRECTION('ref_axis',(1.,0.,0.));
#65155=DIRECTION('',(1.,0.,0.));
#65156=DIRECTION('',(0.,0.,-1.));
#65157=DIRECTION('',(1.,0.,0.));
#65158=DIRECTION('center_axis',(-1.,0.,0.));
#65159=DIRECTION('ref_axis',(0.,1.,0.));
#65160=DIRECTION('',(0.,1.,0.));
#65161=DIRECTION('',(0.,1.,0.));
#65162=DIRECTION('center_axis',(0.,0.,-1.));
#65163=DIRECTION('ref_axis',(-1.,0.,0.));
#65164=DIRECTION('center_axis',(0.,-1.,0.));
#65165=DIRECTION('ref_axis',(-1.,0.,0.));
#65166=DIRECTION('',(-1.,0.,0.));
#65167=DIRECTION('',(0.,0.,-1.));
#65168=DIRECTION('',(-1.,0.,0.));
#65169=DIRECTION('',(0.,0.,-1.));
#65170=DIRECTION('center_axis',(1.,0.,0.));
#65171=DIRECTION('ref_axis',(0.,-1.,0.));
#65172=DIRECTION('',(0.,-1.,0.));
#65173=DIRECTION('',(0.,0.,-1.));
#65174=DIRECTION('',(0.,-1.,0.));
#65175=DIRECTION('center_axis',(0.,1.,0.));
#65176=DIRECTION('ref_axis',(1.,0.,0.));
#65177=DIRECTION('',(1.,0.,0.));
#65178=DIRECTION('',(0.,0.,-1.));
#65179=DIRECTION('',(1.,0.,0.));
#65180=DIRECTION('center_axis',(-1.,0.,0.));
#65181=DIRECTION('ref_axis',(0.,1.,0.));
#65182=DIRECTION('',(0.,1.,0.));
#65183=DIRECTION('',(0.,1.,0.));
#65184=DIRECTION('center_axis',(0.,0.,-1.));
#65185=DIRECTION('ref_axis',(-1.,0.,0.));
#65186=DIRECTION('center_axis',(0.,-1.,0.));
#65187=DIRECTION('ref_axis',(-1.,0.,0.));
#65188=DIRECTION('',(-1.,0.,0.));
#65189=DIRECTION('',(0.,0.,-1.));
#65190=DIRECTION('',(-1.,0.,0.));
#65191=DIRECTION('',(0.,0.,-1.));
#65192=DIRECTION('center_axis',(1.,0.,0.));
#65193=DIRECTION('ref_axis',(0.,-1.,0.));
#65194=DIRECTION('',(0.,-1.,0.));
#65195=DIRECTION('',(0.,0.,-1.));
#65196=DIRECTION('',(0.,-1.,0.));
#65197=DIRECTION('center_axis',(0.,1.,0.));
#65198=DIRECTION('ref_axis',(1.,0.,0.));
#65199=DIRECTION('',(1.,0.,0.));
#65200=DIRECTION('',(0.,0.,-1.));
#65201=DIRECTION('',(1.,0.,0.));
#65202=DIRECTION('center_axis',(-1.,0.,0.));
#65203=DIRECTION('ref_axis',(0.,1.,0.));
#65204=DIRECTION('',(0.,1.,0.));
#65205=DIRECTION('',(0.,1.,0.));
#65206=DIRECTION('center_axis',(0.,0.,-1.));
#65207=DIRECTION('ref_axis',(-1.,0.,0.));
#65208=DIRECTION('center_axis',(0.,-1.,0.));
#65209=DIRECTION('ref_axis',(-1.,0.,0.));
#65210=DIRECTION('',(-1.,0.,0.));
#65211=DIRECTION('',(0.,0.,-1.));
#65212=DIRECTION('',(-1.,0.,0.));
#65213=DIRECTION('',(0.,0.,-1.));
#65214=DIRECTION('center_axis',(1.,0.,0.));
#65215=DIRECTION('ref_axis',(0.,-1.,0.));
#65216=DIRECTION('',(0.,-1.,0.));
#65217=DIRECTION('',(0.,0.,-1.));
#65218=DIRECTION('',(0.,-1.,0.));
#65219=DIRECTION('center_axis',(0.,1.,0.));
#65220=DIRECTION('ref_axis',(1.,0.,0.));
#65221=DIRECTION('',(1.,0.,0.));
#65222=DIRECTION('',(0.,0.,-1.));
#65223=DIRECTION('',(1.,0.,0.));
#65224=DIRECTION('center_axis',(-1.,0.,0.));
#65225=DIRECTION('ref_axis',(0.,1.,0.));
#65226=DIRECTION('',(0.,1.,0.));
#65227=DIRECTION('',(0.,1.,0.));
#65228=DIRECTION('center_axis',(0.,0.,-1.));
#65229=DIRECTION('ref_axis',(-1.,0.,0.));
#65230=DIRECTION('center_axis',(0.,-1.,0.));
#65231=DIRECTION('ref_axis',(-1.,0.,0.));
#65232=DIRECTION('',(-1.,0.,0.));
#65233=DIRECTION('',(0.,0.,-1.));
#65234=DIRECTION('',(-1.,0.,0.));
#65235=DIRECTION('',(0.,0.,-1.));
#65236=DIRECTION('center_axis',(1.,0.,0.));
#65237=DIRECTION('ref_axis',(0.,-1.,0.));
#65238=DIRECTION('',(0.,-1.,0.));
#65239=DIRECTION('',(0.,0.,-1.));
#65240=DIRECTION('',(0.,-1.,0.));
#65241=DIRECTION('center_axis',(0.,1.,0.));
#65242=DIRECTION('ref_axis',(1.,0.,0.));
#65243=DIRECTION('',(1.,0.,0.));
#65244=DIRECTION('',(0.,0.,-1.));
#65245=DIRECTION('',(1.,0.,0.));
#65246=DIRECTION('center_axis',(-1.,0.,0.));
#65247=DIRECTION('ref_axis',(0.,1.,0.));
#65248=DIRECTION('',(0.,1.,0.));
#65249=DIRECTION('',(0.,1.,0.));
#65250=DIRECTION('center_axis',(0.,0.,-1.));
#65251=DIRECTION('ref_axis',(-1.,0.,0.));
#65252=DIRECTION('center_axis',(0.,-1.,0.));
#65253=DIRECTION('ref_axis',(-1.,0.,0.));
#65254=DIRECTION('',(-1.,0.,0.));
#65255=DIRECTION('',(0.,0.,-1.));
#65256=DIRECTION('',(-1.,0.,0.));
#65257=DIRECTION('',(0.,0.,-1.));
#65258=DIRECTION('center_axis',(1.,0.,0.));
#65259=DIRECTION('ref_axis',(0.,-1.,0.));
#65260=DIRECTION('',(0.,-1.,0.));
#65261=DIRECTION('',(0.,0.,-1.));
#65262=DIRECTION('',(0.,-1.,0.));
#65263=DIRECTION('center_axis',(0.,1.,0.));
#65264=DIRECTION('ref_axis',(1.,0.,0.));
#65265=DIRECTION('',(1.,0.,0.));
#65266=DIRECTION('',(0.,0.,-1.));
#65267=DIRECTION('',(1.,0.,0.));
#65268=DIRECTION('center_axis',(-1.,0.,0.));
#65269=DIRECTION('ref_axis',(0.,1.,0.));
#65270=DIRECTION('',(0.,1.,0.));
#65271=DIRECTION('',(0.,1.,0.));
#65272=DIRECTION('center_axis',(0.,0.,-1.));
#65273=DIRECTION('ref_axis',(-1.,0.,0.));
#65274=DIRECTION('center_axis',(0.,-1.,0.));
#65275=DIRECTION('ref_axis',(-1.,0.,0.));
#65276=DIRECTION('',(-1.,0.,0.));
#65277=DIRECTION('',(0.,0.,-1.));
#65278=DIRECTION('',(-1.,0.,0.));
#65279=DIRECTION('',(0.,0.,-1.));
#65280=DIRECTION('center_axis',(1.,0.,0.));
#65281=DIRECTION('ref_axis',(0.,-1.,0.));
#65282=DIRECTION('',(0.,-1.,0.));
#65283=DIRECTION('',(0.,0.,-1.));
#65284=DIRECTION('',(0.,-1.,0.));
#65285=DIRECTION('center_axis',(0.,1.,0.));
#65286=DIRECTION('ref_axis',(1.,0.,0.));
#65287=DIRECTION('',(1.,0.,0.));
#65288=DIRECTION('',(0.,0.,-1.));
#65289=DIRECTION('',(1.,0.,0.));
#65290=DIRECTION('center_axis',(-1.,0.,0.));
#65291=DIRECTION('ref_axis',(0.,1.,0.));
#65292=DIRECTION('',(0.,1.,0.));
#65293=DIRECTION('',(0.,1.,0.));
#65294=DIRECTION('center_axis',(0.,0.,-1.));
#65295=DIRECTION('ref_axis',(-1.,0.,0.));
#65296=DIRECTION('center_axis',(0.,-1.,0.));
#65297=DIRECTION('ref_axis',(-1.,0.,0.));
#65298=DIRECTION('',(-1.,0.,0.));
#65299=DIRECTION('',(0.,0.,-1.));
#65300=DIRECTION('',(-1.,0.,0.));
#65301=DIRECTION('',(0.,0.,-1.));
#65302=DIRECTION('center_axis',(1.,0.,0.));
#65303=DIRECTION('ref_axis',(0.,-1.,0.));
#65304=DIRECTION('',(0.,-1.,0.));
#65305=DIRECTION('',(0.,0.,-1.));
#65306=DIRECTION('',(0.,-1.,0.));
#65307=DIRECTION('center_axis',(0.,1.,0.));
#65308=DIRECTION('ref_axis',(1.,0.,0.));
#65309=DIRECTION('',(1.,0.,0.));
#65310=DIRECTION('',(0.,0.,-1.));
#65311=DIRECTION('',(1.,0.,0.));
#65312=DIRECTION('center_axis',(-1.,0.,0.));
#65313=DIRECTION('ref_axis',(0.,1.,0.));
#65314=DIRECTION('',(0.,1.,0.));
#65315=DIRECTION('',(0.,1.,0.));
#65316=DIRECTION('center_axis',(0.,0.,-1.));
#65317=DIRECTION('ref_axis',(-1.,0.,0.));
#65318=DIRECTION('center_axis',(0.,-1.,0.));
#65319=DIRECTION('ref_axis',(-1.,0.,0.));
#65320=DIRECTION('',(-1.,0.,0.));
#65321=DIRECTION('',(0.,0.,-1.));
#65322=DIRECTION('',(-1.,0.,0.));
#65323=DIRECTION('',(0.,0.,-1.));
#65324=DIRECTION('center_axis',(1.,0.,0.));
#65325=DIRECTION('ref_axis',(0.,-1.,0.));
#65326=DIRECTION('',(0.,-1.,0.));
#65327=DIRECTION('',(0.,0.,-1.));
#65328=DIRECTION('',(0.,-1.,0.));
#65329=DIRECTION('center_axis',(0.,1.,0.));
#65330=DIRECTION('ref_axis',(1.,0.,0.));
#65331=DIRECTION('',(1.,0.,0.));
#65332=DIRECTION('',(0.,0.,-1.));
#65333=DIRECTION('',(1.,0.,0.));
#65334=DIRECTION('center_axis',(-1.,0.,0.));
#65335=DIRECTION('ref_axis',(0.,1.,0.));
#65336=DIRECTION('',(0.,1.,0.));
#65337=DIRECTION('',(0.,1.,0.));
#65338=DIRECTION('center_axis',(0.,0.,-1.));
#65339=DIRECTION('ref_axis',(-1.,0.,0.));
#65340=DIRECTION('center_axis',(0.,-1.,0.));
#65341=DIRECTION('ref_axis',(-1.,0.,0.));
#65342=DIRECTION('',(-1.,0.,0.));
#65343=DIRECTION('',(0.,0.,-1.));
#65344=DIRECTION('',(-1.,0.,0.));
#65345=DIRECTION('',(0.,0.,-1.));
#65346=DIRECTION('center_axis',(1.,0.,0.));
#65347=DIRECTION('ref_axis',(0.,-1.,0.));
#65348=DIRECTION('',(0.,-1.,0.));
#65349=DIRECTION('',(0.,0.,-1.));
#65350=DIRECTION('',(0.,-1.,0.));
#65351=DIRECTION('center_axis',(0.,1.,0.));
#65352=DIRECTION('ref_axis',(1.,0.,0.));
#65353=DIRECTION('',(1.,0.,0.));
#65354=DIRECTION('',(0.,0.,-1.));
#65355=DIRECTION('',(1.,0.,0.));
#65356=DIRECTION('center_axis',(-1.,0.,0.));
#65357=DIRECTION('ref_axis',(0.,1.,0.));
#65358=DIRECTION('',(0.,1.,0.));
#65359=DIRECTION('',(0.,1.,0.));
#65360=DIRECTION('center_axis',(0.,0.,-1.));
#65361=DIRECTION('ref_axis',(-1.,0.,0.));
#65362=DIRECTION('center_axis',(0.,-1.,0.));
#65363=DIRECTION('ref_axis',(-1.,0.,0.));
#65364=DIRECTION('',(-1.,0.,0.));
#65365=DIRECTION('',(0.,0.,-1.));
#65366=DIRECTION('',(-1.,0.,0.));
#65367=DIRECTION('',(0.,0.,-1.));
#65368=DIRECTION('center_axis',(1.,0.,0.));
#65369=DIRECTION('ref_axis',(0.,-1.,0.));
#65370=DIRECTION('',(0.,-1.,0.));
#65371=DIRECTION('',(0.,0.,-1.));
#65372=DIRECTION('',(0.,-1.,0.));
#65373=DIRECTION('center_axis',(0.,1.,0.));
#65374=DIRECTION('ref_axis',(1.,0.,0.));
#65375=DIRECTION('',(1.,0.,0.));
#65376=DIRECTION('',(0.,0.,-1.));
#65377=DIRECTION('',(1.,0.,0.));
#65378=DIRECTION('center_axis',(-1.,0.,0.));
#65379=DIRECTION('ref_axis',(0.,1.,0.));
#65380=DIRECTION('',(0.,1.,0.));
#65381=DIRECTION('',(0.,1.,0.));
#65382=DIRECTION('center_axis',(0.,0.,-1.));
#65383=DIRECTION('ref_axis',(-1.,0.,0.));
#65384=DIRECTION('center_axis',(0.,-1.,0.));
#65385=DIRECTION('ref_axis',(-1.,0.,0.));
#65386=DIRECTION('',(-1.,0.,0.));
#65387=DIRECTION('',(0.,0.,-1.));
#65388=DIRECTION('',(-1.,0.,0.));
#65389=DIRECTION('',(0.,0.,-1.));
#65390=DIRECTION('center_axis',(1.,0.,0.));
#65391=DIRECTION('ref_axis',(0.,-1.,0.));
#65392=DIRECTION('',(0.,-1.,0.));
#65393=DIRECTION('',(0.,0.,-1.));
#65394=DIRECTION('',(0.,-1.,0.));
#65395=DIRECTION('center_axis',(0.,1.,0.));
#65396=DIRECTION('ref_axis',(1.,0.,0.));
#65397=DIRECTION('',(1.,0.,0.));
#65398=DIRECTION('',(0.,0.,-1.));
#65399=DIRECTION('',(1.,0.,0.));
#65400=DIRECTION('center_axis',(-1.,0.,0.));
#65401=DIRECTION('ref_axis',(0.,1.,0.));
#65402=DIRECTION('',(0.,1.,0.));
#65403=DIRECTION('',(0.,1.,0.));
#65404=DIRECTION('center_axis',(0.,0.,-1.));
#65405=DIRECTION('ref_axis',(-1.,0.,0.));
#65406=DIRECTION('center_axis',(0.,-1.,0.));
#65407=DIRECTION('ref_axis',(-1.,0.,0.));
#65408=DIRECTION('',(-1.,0.,0.));
#65409=DIRECTION('',(0.,0.,-1.));
#65410=DIRECTION('',(-1.,0.,0.));
#65411=DIRECTION('',(0.,0.,-1.));
#65412=DIRECTION('center_axis',(1.,0.,0.));
#65413=DIRECTION('ref_axis',(0.,-1.,0.));
#65414=DIRECTION('',(0.,-1.,0.));
#65415=DIRECTION('',(0.,0.,-1.));
#65416=DIRECTION('',(0.,-1.,0.));
#65417=DIRECTION('center_axis',(0.,1.,0.));
#65418=DIRECTION('ref_axis',(1.,0.,0.));
#65419=DIRECTION('',(1.,0.,0.));
#65420=DIRECTION('',(0.,0.,-1.));
#65421=DIRECTION('',(1.,0.,0.));
#65422=DIRECTION('center_axis',(-1.,0.,0.));
#65423=DIRECTION('ref_axis',(0.,1.,0.));
#65424=DIRECTION('',(0.,1.,0.));
#65425=DIRECTION('',(0.,1.,0.));
#65426=DIRECTION('center_axis',(0.,0.,-1.));
#65427=DIRECTION('ref_axis',(-1.,0.,0.));
#65428=DIRECTION('center_axis',(0.,-1.,0.));
#65429=DIRECTION('ref_axis',(-1.,0.,0.));
#65430=DIRECTION('',(-1.,0.,0.));
#65431=DIRECTION('',(0.,0.,-1.));
#65432=DIRECTION('',(-1.,0.,0.));
#65433=DIRECTION('',(0.,0.,-1.));
#65434=DIRECTION('center_axis',(1.,0.,0.));
#65435=DIRECTION('ref_axis',(0.,-1.,0.));
#65436=DIRECTION('',(0.,-1.,0.));
#65437=DIRECTION('',(0.,0.,-1.));
#65438=DIRECTION('',(0.,-1.,0.));
#65439=DIRECTION('center_axis',(0.,1.,0.));
#65440=DIRECTION('ref_axis',(1.,0.,0.));
#65441=DIRECTION('',(1.,0.,0.));
#65442=DIRECTION('',(0.,0.,-1.));
#65443=DIRECTION('',(1.,0.,0.));
#65444=DIRECTION('center_axis',(-1.,0.,0.));
#65445=DIRECTION('ref_axis',(0.,1.,0.));
#65446=DIRECTION('',(0.,1.,0.));
#65447=DIRECTION('',(0.,1.,0.));
#65448=DIRECTION('center_axis',(0.,0.,-1.));
#65449=DIRECTION('ref_axis',(-1.,0.,0.));
#65450=DIRECTION('center_axis',(0.,-1.,0.));
#65451=DIRECTION('ref_axis',(-1.,0.,0.));
#65452=DIRECTION('',(-1.,0.,0.));
#65453=DIRECTION('',(0.,0.,-1.));
#65454=DIRECTION('',(-1.,0.,0.));
#65455=DIRECTION('',(0.,0.,-1.));
#65456=DIRECTION('center_axis',(1.,0.,0.));
#65457=DIRECTION('ref_axis',(0.,-1.,0.));
#65458=DIRECTION('',(0.,-1.,0.));
#65459=DIRECTION('',(0.,0.,-1.));
#65460=DIRECTION('',(0.,-1.,0.));
#65461=DIRECTION('center_axis',(0.,1.,0.));
#65462=DIRECTION('ref_axis',(1.,0.,0.));
#65463=DIRECTION('',(1.,0.,0.));
#65464=DIRECTION('',(0.,0.,-1.));
#65465=DIRECTION('',(1.,0.,0.));
#65466=DIRECTION('center_axis',(-1.,0.,0.));
#65467=DIRECTION('ref_axis',(0.,1.,0.));
#65468=DIRECTION('',(0.,1.,0.));
#65469=DIRECTION('',(0.,1.,0.));
#65470=DIRECTION('center_axis',(0.,0.,-1.));
#65471=DIRECTION('ref_axis',(-1.,0.,0.));
#65472=DIRECTION('center_axis',(0.,-1.,0.));
#65473=DIRECTION('ref_axis',(-1.,0.,0.));
#65474=DIRECTION('',(-1.,0.,0.));
#65475=DIRECTION('',(0.,0.,-1.));
#65476=DIRECTION('',(-1.,0.,0.));
#65477=DIRECTION('',(0.,0.,-1.));
#65478=DIRECTION('center_axis',(1.,0.,0.));
#65479=DIRECTION('ref_axis',(0.,-1.,0.));
#65480=DIRECTION('',(0.,-1.,0.));
#65481=DIRECTION('',(0.,0.,-1.));
#65482=DIRECTION('',(0.,-1.,0.));
#65483=DIRECTION('center_axis',(0.,1.,0.));
#65484=DIRECTION('ref_axis',(1.,0.,0.));
#65485=DIRECTION('',(1.,0.,0.));
#65486=DIRECTION('',(0.,0.,-1.));
#65487=DIRECTION('',(1.,0.,0.));
#65488=DIRECTION('center_axis',(-1.,0.,0.));
#65489=DIRECTION('ref_axis',(0.,1.,0.));
#65490=DIRECTION('',(0.,1.,0.));
#65491=DIRECTION('',(0.,1.,0.));
#65492=DIRECTION('center_axis',(0.,0.,-1.));
#65493=DIRECTION('ref_axis',(-1.,0.,0.));
#65494=DIRECTION('center_axis',(0.,-1.,0.));
#65495=DIRECTION('ref_axis',(-1.,0.,0.));
#65496=DIRECTION('',(-1.,0.,0.));
#65497=DIRECTION('',(0.,0.,-1.));
#65498=DIRECTION('',(-1.,0.,0.));
#65499=DIRECTION('',(0.,0.,-1.));
#65500=DIRECTION('center_axis',(1.,0.,0.));
#65501=DIRECTION('ref_axis',(0.,-1.,0.));
#65502=DIRECTION('',(0.,-1.,0.));
#65503=DIRECTION('',(0.,0.,-1.));
#65504=DIRECTION('',(0.,-1.,0.));
#65505=DIRECTION('center_axis',(0.,1.,0.));
#65506=DIRECTION('ref_axis',(1.,0.,0.));
#65507=DIRECTION('',(1.,0.,0.));
#65508=DIRECTION('',(0.,0.,-1.));
#65509=DIRECTION('',(1.,0.,0.));
#65510=DIRECTION('center_axis',(-1.,0.,0.));
#65511=DIRECTION('ref_axis',(0.,1.,0.));
#65512=DIRECTION('',(0.,1.,0.));
#65513=DIRECTION('',(0.,1.,0.));
#65514=DIRECTION('center_axis',(0.,0.,-1.));
#65515=DIRECTION('ref_axis',(-1.,0.,0.));
#65516=DIRECTION('center_axis',(0.,-1.,0.));
#65517=DIRECTION('ref_axis',(-1.,0.,0.));
#65518=DIRECTION('',(-1.,0.,0.));
#65519=DIRECTION('',(0.,0.,-1.));
#65520=DIRECTION('',(-1.,0.,0.));
#65521=DIRECTION('',(0.,0.,-1.));
#65522=DIRECTION('center_axis',(1.,0.,0.));
#65523=DIRECTION('ref_axis',(0.,-1.,0.));
#65524=DIRECTION('',(0.,-1.,0.));
#65525=DIRECTION('',(0.,0.,-1.));
#65526=DIRECTION('',(0.,-1.,0.));
#65527=DIRECTION('center_axis',(0.,1.,0.));
#65528=DIRECTION('ref_axis',(1.,0.,0.));
#65529=DIRECTION('',(1.,0.,0.));
#65530=DIRECTION('',(0.,0.,-1.));
#65531=DIRECTION('',(1.,0.,0.));
#65532=DIRECTION('center_axis',(-1.,0.,0.));
#65533=DIRECTION('ref_axis',(0.,1.,0.));
#65534=DIRECTION('',(0.,1.,0.));
#65535=DIRECTION('',(0.,1.,0.));
#65536=DIRECTION('center_axis',(0.,0.,-1.));
#65537=DIRECTION('ref_axis',(-1.,0.,0.));
#65538=DIRECTION('center_axis',(0.,-1.,0.));
#65539=DIRECTION('ref_axis',(-1.,0.,0.));
#65540=DIRECTION('',(-1.,0.,0.));
#65541=DIRECTION('',(0.,0.,-1.));
#65542=DIRECTION('',(-1.,0.,0.));
#65543=DIRECTION('',(0.,0.,-1.));
#65544=DIRECTION('center_axis',(1.,0.,0.));
#65545=DIRECTION('ref_axis',(0.,-1.,0.));
#65546=DIRECTION('',(0.,-1.,0.));
#65547=DIRECTION('',(0.,0.,-1.));
#65548=DIRECTION('',(0.,-1.,0.));
#65549=DIRECTION('center_axis',(0.,1.,0.));
#65550=DIRECTION('ref_axis',(1.,0.,0.));
#65551=DIRECTION('',(1.,0.,0.));
#65552=DIRECTION('',(0.,0.,-1.));
#65553=DIRECTION('',(1.,0.,0.));
#65554=DIRECTION('center_axis',(-1.,0.,0.));
#65555=DIRECTION('ref_axis',(0.,1.,0.));
#65556=DIRECTION('',(0.,1.,0.));
#65557=DIRECTION('',(0.,1.,0.));
#65558=DIRECTION('center_axis',(0.,0.,-1.));
#65559=DIRECTION('ref_axis',(-1.,0.,0.));
#65560=DIRECTION('center_axis',(0.,-1.,0.));
#65561=DIRECTION('ref_axis',(-1.,0.,0.));
#65562=DIRECTION('',(-1.,0.,0.));
#65563=DIRECTION('',(0.,0.,-1.));
#65564=DIRECTION('',(-1.,0.,0.));
#65565=DIRECTION('',(0.,0.,-1.));
#65566=DIRECTION('center_axis',(1.,0.,0.));
#65567=DIRECTION('ref_axis',(0.,-1.,0.));
#65568=DIRECTION('',(0.,-1.,0.));
#65569=DIRECTION('',(0.,0.,-1.));
#65570=DIRECTION('',(0.,-1.,0.));
#65571=DIRECTION('center_axis',(0.,1.,0.));
#65572=DIRECTION('ref_axis',(1.,0.,0.));
#65573=DIRECTION('',(1.,0.,0.));
#65574=DIRECTION('',(0.,0.,-1.));
#65575=DIRECTION('',(1.,0.,0.));
#65576=DIRECTION('center_axis',(-1.,0.,0.));
#65577=DIRECTION('ref_axis',(0.,1.,0.));
#65578=DIRECTION('',(0.,1.,0.));
#65579=DIRECTION('',(0.,1.,0.));
#65580=DIRECTION('center_axis',(0.,0.,-1.));
#65581=DIRECTION('ref_axis',(-1.,0.,0.));
#65582=DIRECTION('center_axis',(0.,-1.,0.));
#65583=DIRECTION('ref_axis',(-1.,0.,0.));
#65584=DIRECTION('',(-1.,0.,0.));
#65585=DIRECTION('',(0.,0.,-1.));
#65586=DIRECTION('',(-1.,0.,0.));
#65587=DIRECTION('',(0.,0.,-1.));
#65588=DIRECTION('center_axis',(1.,0.,0.));
#65589=DIRECTION('ref_axis',(0.,-1.,0.));
#65590=DIRECTION('',(0.,-1.,0.));
#65591=DIRECTION('',(0.,0.,-1.));
#65592=DIRECTION('',(0.,-1.,0.));
#65593=DIRECTION('center_axis',(0.,1.,0.));
#65594=DIRECTION('ref_axis',(1.,0.,0.));
#65595=DIRECTION('',(1.,0.,0.));
#65596=DIRECTION('',(0.,0.,-1.));
#65597=DIRECTION('',(1.,0.,0.));
#65598=DIRECTION('center_axis',(-1.,0.,0.));
#65599=DIRECTION('ref_axis',(0.,1.,0.));
#65600=DIRECTION('',(0.,1.,0.));
#65601=DIRECTION('',(0.,1.,0.));
#65602=DIRECTION('center_axis',(0.,0.,-1.));
#65603=DIRECTION('ref_axis',(-1.,0.,0.));
#65604=DIRECTION('center_axis',(0.,-1.,0.));
#65605=DIRECTION('ref_axis',(-1.,0.,0.));
#65606=DIRECTION('',(-1.,0.,0.));
#65607=DIRECTION('',(0.,0.,-1.));
#65608=DIRECTION('',(-1.,0.,0.));
#65609=DIRECTION('',(0.,0.,-1.));
#65610=DIRECTION('center_axis',(1.,0.,0.));
#65611=DIRECTION('ref_axis',(0.,-1.,0.));
#65612=DIRECTION('',(0.,-1.,0.));
#65613=DIRECTION('',(0.,0.,-1.));
#65614=DIRECTION('',(0.,-1.,0.));
#65615=DIRECTION('center_axis',(0.,1.,0.));
#65616=DIRECTION('ref_axis',(1.,0.,0.));
#65617=DIRECTION('',(1.,0.,0.));
#65618=DIRECTION('',(0.,0.,-1.));
#65619=DIRECTION('',(1.,0.,0.));
#65620=DIRECTION('center_axis',(-1.,0.,0.));
#65621=DIRECTION('ref_axis',(0.,1.,0.));
#65622=DIRECTION('',(0.,1.,0.));
#65623=DIRECTION('',(0.,1.,0.));
#65624=DIRECTION('center_axis',(0.,0.,-1.));
#65625=DIRECTION('ref_axis',(-1.,0.,0.));
#65626=DIRECTION('center_axis',(0.,-1.,0.));
#65627=DIRECTION('ref_axis',(-1.,0.,0.));
#65628=DIRECTION('',(-1.,0.,0.));
#65629=DIRECTION('',(0.,0.,-1.));
#65630=DIRECTION('',(-1.,0.,0.));
#65631=DIRECTION('',(0.,0.,-1.));
#65632=DIRECTION('center_axis',(1.,0.,0.));
#65633=DIRECTION('ref_axis',(0.,-1.,0.));
#65634=DIRECTION('',(0.,-1.,0.));
#65635=DIRECTION('',(0.,0.,-1.));
#65636=DIRECTION('',(0.,-1.,0.));
#65637=DIRECTION('center_axis',(0.,1.,0.));
#65638=DIRECTION('ref_axis',(1.,0.,0.));
#65639=DIRECTION('',(1.,0.,0.));
#65640=DIRECTION('',(0.,0.,-1.));
#65641=DIRECTION('',(1.,0.,0.));
#65642=DIRECTION('center_axis',(-1.,0.,0.));
#65643=DIRECTION('ref_axis',(0.,1.,0.));
#65644=DIRECTION('',(0.,1.,0.));
#65645=DIRECTION('',(0.,1.,0.));
#65646=DIRECTION('center_axis',(0.,0.,-1.));
#65647=DIRECTION('ref_axis',(-1.,0.,0.));
#65648=DIRECTION('center_axis',(0.,-1.,0.));
#65649=DIRECTION('ref_axis',(-1.,0.,0.));
#65650=DIRECTION('',(-1.,0.,0.));
#65651=DIRECTION('',(0.,0.,-1.));
#65652=DIRECTION('',(-1.,0.,0.));
#65653=DIRECTION('',(0.,0.,-1.));
#65654=DIRECTION('center_axis',(1.,0.,0.));
#65655=DIRECTION('ref_axis',(0.,-1.,0.));
#65656=DIRECTION('',(0.,-1.,0.));
#65657=DIRECTION('',(0.,0.,-1.));
#65658=DIRECTION('',(0.,-1.,0.));
#65659=DIRECTION('center_axis',(0.,1.,0.));
#65660=DIRECTION('ref_axis',(1.,0.,0.));
#65661=DIRECTION('',(1.,0.,0.));
#65662=DIRECTION('',(0.,0.,-1.));
#65663=DIRECTION('',(1.,0.,0.));
#65664=DIRECTION('center_axis',(-1.,0.,0.));
#65665=DIRECTION('ref_axis',(0.,1.,0.));
#65666=DIRECTION('',(0.,1.,0.));
#65667=DIRECTION('',(0.,1.,0.));
#65668=DIRECTION('center_axis',(0.,0.,-1.));
#65669=DIRECTION('ref_axis',(-1.,0.,0.));
#65670=DIRECTION('center_axis',(0.,-1.,0.));
#65671=DIRECTION('ref_axis',(-1.,0.,0.));
#65672=DIRECTION('',(-1.,0.,0.));
#65673=DIRECTION('',(0.,0.,-1.));
#65674=DIRECTION('',(-1.,0.,0.));
#65675=DIRECTION('',(0.,0.,-1.));
#65676=DIRECTION('center_axis',(1.,0.,0.));
#65677=DIRECTION('ref_axis',(0.,-1.,0.));
#65678=DIRECTION('',(0.,-1.,0.));
#65679=DIRECTION('',(0.,0.,-1.));
#65680=DIRECTION('',(0.,-1.,0.));
#65681=DIRECTION('center_axis',(0.,1.,0.));
#65682=DIRECTION('ref_axis',(1.,0.,0.));
#65683=DIRECTION('',(1.,0.,0.));
#65684=DIRECTION('',(0.,0.,-1.));
#65685=DIRECTION('',(1.,0.,0.));
#65686=DIRECTION('center_axis',(-1.,0.,0.));
#65687=DIRECTION('ref_axis',(0.,1.,0.));
#65688=DIRECTION('',(0.,1.,0.));
#65689=DIRECTION('',(0.,1.,0.));
#65690=DIRECTION('center_axis',(0.,0.,-1.));
#65691=DIRECTION('ref_axis',(-1.,0.,0.));
#65692=DIRECTION('center_axis',(0.,-1.,0.));
#65693=DIRECTION('ref_axis',(-1.,0.,0.));
#65694=DIRECTION('',(-1.,0.,0.));
#65695=DIRECTION('',(0.,0.,-1.));
#65696=DIRECTION('',(-1.,0.,0.));
#65697=DIRECTION('',(0.,0.,-1.));
#65698=DIRECTION('center_axis',(1.,0.,0.));
#65699=DIRECTION('ref_axis',(0.,-1.,0.));
#65700=DIRECTION('',(0.,-1.,0.));
#65701=DIRECTION('',(0.,0.,-1.));
#65702=DIRECTION('',(0.,-1.,0.));
#65703=DIRECTION('center_axis',(0.,1.,0.));
#65704=DIRECTION('ref_axis',(1.,0.,0.));
#65705=DIRECTION('',(1.,0.,0.));
#65706=DIRECTION('',(0.,0.,-1.));
#65707=DIRECTION('',(1.,0.,0.));
#65708=DIRECTION('center_axis',(-1.,0.,0.));
#65709=DIRECTION('ref_axis',(0.,1.,0.));
#65710=DIRECTION('',(0.,1.,0.));
#65711=DIRECTION('',(0.,1.,0.));
#65712=DIRECTION('center_axis',(0.,0.,-1.));
#65713=DIRECTION('ref_axis',(-1.,0.,0.));
#65714=DIRECTION('center_axis',(0.,-1.,0.));
#65715=DIRECTION('ref_axis',(-1.,0.,0.));
#65716=DIRECTION('',(-1.,0.,0.));
#65717=DIRECTION('',(0.,0.,-1.));
#65718=DIRECTION('',(-1.,0.,0.));
#65719=DIRECTION('',(0.,0.,-1.));
#65720=DIRECTION('center_axis',(1.,0.,0.));
#65721=DIRECTION('ref_axis',(0.,-1.,0.));
#65722=DIRECTION('',(0.,-1.,0.));
#65723=DIRECTION('',(0.,0.,-1.));
#65724=DIRECTION('',(0.,-1.,0.));
#65725=DIRECTION('center_axis',(0.,1.,0.));
#65726=DIRECTION('ref_axis',(1.,0.,0.));
#65727=DIRECTION('',(1.,0.,0.));
#65728=DIRECTION('',(0.,0.,-1.));
#65729=DIRECTION('',(1.,0.,0.));
#65730=DIRECTION('center_axis',(-1.,0.,0.));
#65731=DIRECTION('ref_axis',(0.,1.,0.));
#65732=DIRECTION('',(0.,1.,0.));
#65733=DIRECTION('',(0.,1.,0.));
#65734=DIRECTION('center_axis',(0.,0.,-1.));
#65735=DIRECTION('ref_axis',(-1.,0.,0.));
#65736=DIRECTION('center_axis',(0.,-1.,0.));
#65737=DIRECTION('ref_axis',(-1.,0.,0.));
#65738=DIRECTION('',(-1.,0.,0.));
#65739=DIRECTION('',(0.,0.,-1.));
#65740=DIRECTION('',(-1.,0.,0.));
#65741=DIRECTION('',(0.,0.,-1.));
#65742=DIRECTION('center_axis',(1.,0.,0.));
#65743=DIRECTION('ref_axis',(0.,-1.,0.));
#65744=DIRECTION('',(0.,-1.,0.));
#65745=DIRECTION('',(0.,0.,-1.));
#65746=DIRECTION('',(0.,-1.,0.));
#65747=DIRECTION('center_axis',(0.,1.,0.));
#65748=DIRECTION('ref_axis',(1.,0.,0.));
#65749=DIRECTION('',(1.,0.,0.));
#65750=DIRECTION('',(0.,0.,-1.));
#65751=DIRECTION('',(1.,0.,0.));
#65752=DIRECTION('center_axis',(-1.,0.,0.));
#65753=DIRECTION('ref_axis',(0.,1.,0.));
#65754=DIRECTION('',(0.,1.,0.));
#65755=DIRECTION('',(0.,1.,0.));
#65756=DIRECTION('center_axis',(0.,0.,-1.));
#65757=DIRECTION('ref_axis',(-1.,0.,0.));
#65758=DIRECTION('center_axis',(0.,-1.,0.));
#65759=DIRECTION('ref_axis',(-1.,0.,0.));
#65760=DIRECTION('',(-1.,0.,0.));
#65761=DIRECTION('',(0.,0.,-1.));
#65762=DIRECTION('',(-1.,0.,0.));
#65763=DIRECTION('',(0.,0.,-1.));
#65764=DIRECTION('center_axis',(1.,0.,0.));
#65765=DIRECTION('ref_axis',(0.,-1.,0.));
#65766=DIRECTION('',(0.,-1.,0.));
#65767=DIRECTION('',(0.,0.,-1.));
#65768=DIRECTION('',(0.,-1.,0.));
#65769=DIRECTION('center_axis',(0.,1.,0.));
#65770=DIRECTION('ref_axis',(1.,0.,0.));
#65771=DIRECTION('',(1.,0.,0.));
#65772=DIRECTION('',(0.,0.,-1.));
#65773=DIRECTION('',(1.,0.,0.));
#65774=DIRECTION('center_axis',(-1.,0.,0.));
#65775=DIRECTION('ref_axis',(0.,1.,0.));
#65776=DIRECTION('',(0.,1.,0.));
#65777=DIRECTION('',(0.,1.,0.));
#65778=DIRECTION('center_axis',(0.,0.,-1.));
#65779=DIRECTION('ref_axis',(-1.,0.,0.));
#65780=DIRECTION('center_axis',(0.,-1.,0.));
#65781=DIRECTION('ref_axis',(-1.,0.,0.));
#65782=DIRECTION('',(-1.,0.,0.));
#65783=DIRECTION('',(0.,0.,-1.));
#65784=DIRECTION('',(-1.,0.,0.));
#65785=DIRECTION('',(0.,0.,-1.));
#65786=DIRECTION('center_axis',(1.,0.,0.));
#65787=DIRECTION('ref_axis',(0.,-1.,0.));
#65788=DIRECTION('',(0.,-1.,0.));
#65789=DIRECTION('',(0.,0.,-1.));
#65790=DIRECTION('',(0.,-1.,0.));
#65791=DIRECTION('center_axis',(0.,1.,0.));
#65792=DIRECTION('ref_axis',(1.,0.,0.));
#65793=DIRECTION('',(1.,0.,0.));
#65794=DIRECTION('',(0.,0.,-1.));
#65795=DIRECTION('',(1.,0.,0.));
#65796=DIRECTION('center_axis',(-1.,0.,0.));
#65797=DIRECTION('ref_axis',(0.,1.,0.));
#65798=DIRECTION('',(0.,1.,0.));
#65799=DIRECTION('',(0.,1.,0.));
#65800=DIRECTION('center_axis',(0.,0.,-1.));
#65801=DIRECTION('ref_axis',(-1.,0.,0.));
#65802=DIRECTION('center_axis',(0.,-1.,0.));
#65803=DIRECTION('ref_axis',(-1.,0.,0.));
#65804=DIRECTION('',(-1.,0.,0.));
#65805=DIRECTION('',(0.,0.,-1.));
#65806=DIRECTION('',(-1.,0.,0.));
#65807=DIRECTION('',(0.,0.,-1.));
#65808=DIRECTION('center_axis',(1.,0.,0.));
#65809=DIRECTION('ref_axis',(0.,-1.,0.));
#65810=DIRECTION('',(0.,-1.,0.));
#65811=DIRECTION('',(0.,0.,-1.));
#65812=DIRECTION('',(0.,-1.,0.));
#65813=DIRECTION('center_axis',(0.,1.,0.));
#65814=DIRECTION('ref_axis',(1.,0.,0.));
#65815=DIRECTION('',(1.,0.,0.));
#65816=DIRECTION('',(0.,0.,-1.));
#65817=DIRECTION('',(1.,0.,0.));
#65818=DIRECTION('center_axis',(-1.,0.,0.));
#65819=DIRECTION('ref_axis',(0.,1.,0.));
#65820=DIRECTION('',(0.,1.,0.));
#65821=DIRECTION('',(0.,1.,0.));
#65822=DIRECTION('center_axis',(0.,0.,-1.));
#65823=DIRECTION('ref_axis',(-1.,0.,0.));
#65824=DIRECTION('center_axis',(0.,-1.,0.));
#65825=DIRECTION('ref_axis',(-1.,0.,0.));
#65826=DIRECTION('',(-1.,0.,0.));
#65827=DIRECTION('',(0.,0.,-1.));
#65828=DIRECTION('',(-1.,0.,0.));
#65829=DIRECTION('',(0.,0.,-1.));
#65830=DIRECTION('center_axis',(1.,0.,0.));
#65831=DIRECTION('ref_axis',(0.,-1.,0.));
#65832=DIRECTION('',(0.,-1.,0.));
#65833=DIRECTION('',(0.,0.,-1.));
#65834=DIRECTION('',(0.,-1.,0.));
#65835=DIRECTION('center_axis',(0.,1.,0.));
#65836=DIRECTION('ref_axis',(1.,0.,0.));
#65837=DIRECTION('',(1.,0.,0.));
#65838=DIRECTION('',(0.,0.,-1.));
#65839=DIRECTION('',(1.,0.,0.));
#65840=DIRECTION('center_axis',(-1.,0.,0.));
#65841=DIRECTION('ref_axis',(0.,1.,0.));
#65842=DIRECTION('',(0.,1.,0.));
#65843=DIRECTION('',(0.,1.,0.));
#65844=DIRECTION('center_axis',(0.,0.,-1.));
#65845=DIRECTION('ref_axis',(-1.,0.,0.));
#65846=DIRECTION('center_axis',(0.,-1.,0.));
#65847=DIRECTION('ref_axis',(-1.,0.,0.));
#65848=DIRECTION('',(-1.,0.,0.));
#65849=DIRECTION('',(0.,0.,-1.));
#65850=DIRECTION('',(-1.,0.,0.));
#65851=DIRECTION('',(0.,0.,-1.));
#65852=DIRECTION('center_axis',(1.,0.,0.));
#65853=DIRECTION('ref_axis',(0.,-1.,0.));
#65854=DIRECTION('',(0.,-1.,0.));
#65855=DIRECTION('',(0.,0.,-1.));
#65856=DIRECTION('',(0.,-1.,0.));
#65857=DIRECTION('center_axis',(0.,1.,0.));
#65858=DIRECTION('ref_axis',(1.,0.,0.));
#65859=DIRECTION('',(1.,0.,0.));
#65860=DIRECTION('',(0.,0.,-1.));
#65861=DIRECTION('',(1.,0.,0.));
#65862=DIRECTION('center_axis',(-1.,0.,0.));
#65863=DIRECTION('ref_axis',(0.,1.,0.));
#65864=DIRECTION('',(0.,1.,0.));
#65865=DIRECTION('',(0.,1.,0.));
#65866=DIRECTION('center_axis',(0.,0.,-1.));
#65867=DIRECTION('ref_axis',(-1.,0.,0.));
#65868=DIRECTION('center_axis',(0.,-1.,0.));
#65869=DIRECTION('ref_axis',(-1.,0.,0.));
#65870=DIRECTION('',(-1.,0.,0.));
#65871=DIRECTION('',(0.,0.,-1.));
#65872=DIRECTION('',(-1.,0.,0.));
#65873=DIRECTION('',(0.,0.,-1.));
#65874=DIRECTION('center_axis',(1.,0.,0.));
#65875=DIRECTION('ref_axis',(0.,-1.,0.));
#65876=DIRECTION('',(0.,-1.,0.));
#65877=DIRECTION('',(0.,0.,-1.));
#65878=DIRECTION('',(0.,-1.,0.));
#65879=DIRECTION('center_axis',(0.,1.,0.));
#65880=DIRECTION('ref_axis',(1.,0.,0.));
#65881=DIRECTION('',(1.,0.,0.));
#65882=DIRECTION('',(0.,0.,-1.));
#65883=DIRECTION('',(1.,0.,0.));
#65884=DIRECTION('center_axis',(-1.,0.,0.));
#65885=DIRECTION('ref_axis',(0.,1.,0.));
#65886=DIRECTION('',(0.,1.,0.));
#65887=DIRECTION('',(0.,1.,0.));
#65888=DIRECTION('center_axis',(0.,0.,-1.));
#65889=DIRECTION('ref_axis',(-1.,0.,0.));
#65890=DIRECTION('center_axis',(0.,-1.,0.));
#65891=DIRECTION('ref_axis',(-1.,0.,0.));
#65892=DIRECTION('',(-1.,0.,0.));
#65893=DIRECTION('',(0.,0.,-1.));
#65894=DIRECTION('',(-1.,0.,0.));
#65895=DIRECTION('',(0.,0.,-1.));
#65896=DIRECTION('center_axis',(1.,0.,0.));
#65897=DIRECTION('ref_axis',(0.,-1.,0.));
#65898=DIRECTION('',(0.,-1.,0.));
#65899=DIRECTION('',(0.,0.,-1.));
#65900=DIRECTION('',(0.,-1.,0.));
#65901=DIRECTION('center_axis',(0.,1.,0.));
#65902=DIRECTION('ref_axis',(1.,0.,0.));
#65903=DIRECTION('',(1.,0.,0.));
#65904=DIRECTION('',(0.,0.,-1.));
#65905=DIRECTION('',(1.,0.,0.));
#65906=DIRECTION('center_axis',(-1.,0.,0.));
#65907=DIRECTION('ref_axis',(0.,1.,0.));
#65908=DIRECTION('',(0.,1.,0.));
#65909=DIRECTION('',(0.,1.,0.));
#65910=DIRECTION('center_axis',(0.,0.,-1.));
#65911=DIRECTION('ref_axis',(-1.,0.,0.));
#65912=DIRECTION('center_axis',(0.,-1.,0.));
#65913=DIRECTION('ref_axis',(-1.,0.,0.));
#65914=DIRECTION('',(-1.,0.,0.));
#65915=DIRECTION('',(0.,0.,-1.));
#65916=DIRECTION('',(-1.,0.,0.));
#65917=DIRECTION('',(0.,0.,-1.));
#65918=DIRECTION('center_axis',(1.,0.,0.));
#65919=DIRECTION('ref_axis',(0.,-1.,0.));
#65920=DIRECTION('',(0.,-1.,0.));
#65921=DIRECTION('',(0.,0.,-1.));
#65922=DIRECTION('',(0.,-1.,0.));
#65923=DIRECTION('center_axis',(0.,1.,0.));
#65924=DIRECTION('ref_axis',(1.,0.,0.));
#65925=DIRECTION('',(1.,0.,0.));
#65926=DIRECTION('',(0.,0.,-1.));
#65927=DIRECTION('',(1.,0.,0.));
#65928=DIRECTION('center_axis',(-1.,0.,0.));
#65929=DIRECTION('ref_axis',(0.,1.,0.));
#65930=DIRECTION('',(0.,1.,0.));
#65931=DIRECTION('',(0.,1.,0.));
#65932=DIRECTION('center_axis',(0.,0.,-1.));
#65933=DIRECTION('ref_axis',(-1.,0.,0.));
#65934=DIRECTION('center_axis',(0.,-1.,0.));
#65935=DIRECTION('ref_axis',(-1.,0.,0.));
#65936=DIRECTION('',(-1.,0.,0.));
#65937=DIRECTION('',(0.,0.,-1.));
#65938=DIRECTION('',(-1.,0.,0.));
#65939=DIRECTION('',(0.,0.,-1.));
#65940=DIRECTION('center_axis',(1.,0.,0.));
#65941=DIRECTION('ref_axis',(0.,-1.,0.));
#65942=DIRECTION('',(0.,-1.,0.));
#65943=DIRECTION('',(0.,0.,-1.));
#65944=DIRECTION('',(0.,-1.,0.));
#65945=DIRECTION('center_axis',(0.,1.,0.));
#65946=DIRECTION('ref_axis',(1.,0.,0.));
#65947=DIRECTION('',(1.,0.,0.));
#65948=DIRECTION('',(0.,0.,-1.));
#65949=DIRECTION('',(1.,0.,0.));
#65950=DIRECTION('center_axis',(-1.,0.,0.));
#65951=DIRECTION('ref_axis',(0.,1.,0.));
#65952=DIRECTION('',(0.,1.,0.));
#65953=DIRECTION('',(0.,1.,0.));
#65954=DIRECTION('center_axis',(0.,0.,-1.));
#65955=DIRECTION('ref_axis',(-1.,0.,0.));
#65956=DIRECTION('center_axis',(0.,-1.,0.));
#65957=DIRECTION('ref_axis',(-1.,0.,0.));
#65958=DIRECTION('',(-1.,0.,0.));
#65959=DIRECTION('',(0.,0.,-1.));
#65960=DIRECTION('',(-1.,0.,0.));
#65961=DIRECTION('',(0.,0.,-1.));
#65962=DIRECTION('center_axis',(1.,0.,0.));
#65963=DIRECTION('ref_axis',(0.,-1.,0.));
#65964=DIRECTION('',(0.,-1.,0.));
#65965=DIRECTION('',(0.,0.,-1.));
#65966=DIRECTION('',(0.,-1.,0.));
#65967=DIRECTION('center_axis',(0.,1.,0.));
#65968=DIRECTION('ref_axis',(1.,0.,0.));
#65969=DIRECTION('',(1.,0.,0.));
#65970=DIRECTION('',(0.,0.,-1.));
#65971=DIRECTION('',(1.,0.,0.));
#65972=DIRECTION('center_axis',(-1.,0.,0.));
#65973=DIRECTION('ref_axis',(0.,1.,0.));
#65974=DIRECTION('',(0.,1.,0.));
#65975=DIRECTION('',(0.,1.,0.));
#65976=DIRECTION('center_axis',(0.,0.,-1.));
#65977=DIRECTION('ref_axis',(-1.,0.,0.));
#65978=DIRECTION('center_axis',(0.,-1.,0.));
#65979=DIRECTION('ref_axis',(-1.,0.,0.));
#65980=DIRECTION('',(-1.,0.,0.));
#65981=DIRECTION('',(0.,0.,-1.));
#65982=DIRECTION('',(-1.,0.,0.));
#65983=DIRECTION('',(0.,0.,-1.));
#65984=DIRECTION('center_axis',(1.,0.,0.));
#65985=DIRECTION('ref_axis',(0.,-1.,0.));
#65986=DIRECTION('',(0.,-1.,0.));
#65987=DIRECTION('',(0.,0.,-1.));
#65988=DIRECTION('',(0.,-1.,0.));
#65989=DIRECTION('center_axis',(0.,1.,0.));
#65990=DIRECTION('ref_axis',(1.,0.,0.));
#65991=DIRECTION('',(1.,0.,0.));
#65992=DIRECTION('',(0.,0.,-1.));
#65993=DIRECTION('',(1.,0.,0.));
#65994=DIRECTION('center_axis',(-1.,0.,0.));
#65995=DIRECTION('ref_axis',(0.,1.,0.));
#65996=DIRECTION('',(0.,1.,0.));
#65997=DIRECTION('',(0.,1.,0.));
#65998=DIRECTION('center_axis',(0.,0.,-1.));
#65999=DIRECTION('ref_axis',(-1.,0.,0.));
#66000=DIRECTION('center_axis',(0.,-1.,0.));
#66001=DIRECTION('ref_axis',(-1.,0.,0.));
#66002=DIRECTION('',(-1.,0.,0.));
#66003=DIRECTION('',(0.,0.,-1.));
#66004=DIRECTION('',(-1.,0.,0.));
#66005=DIRECTION('',(0.,0.,-1.));
#66006=DIRECTION('center_axis',(1.,0.,0.));
#66007=DIRECTION('ref_axis',(0.,-1.,0.));
#66008=DIRECTION('',(0.,-1.,0.));
#66009=DIRECTION('',(0.,0.,-1.));
#66010=DIRECTION('',(0.,-1.,0.));
#66011=DIRECTION('center_axis',(0.,1.,0.));
#66012=DIRECTION('ref_axis',(1.,0.,0.));
#66013=DIRECTION('',(1.,0.,0.));
#66014=DIRECTION('',(0.,0.,-1.));
#66015=DIRECTION('',(1.,0.,0.));
#66016=DIRECTION('center_axis',(-1.,0.,0.));
#66017=DIRECTION('ref_axis',(0.,1.,0.));
#66018=DIRECTION('',(0.,1.,0.));
#66019=DIRECTION('',(0.,1.,0.));
#66020=DIRECTION('center_axis',(0.,0.,-1.));
#66021=DIRECTION('ref_axis',(-1.,0.,0.));
#66022=DIRECTION('center_axis',(0.,-1.,0.));
#66023=DIRECTION('ref_axis',(-1.,0.,0.));
#66024=DIRECTION('',(-1.,0.,0.));
#66025=DIRECTION('',(0.,0.,-1.));
#66026=DIRECTION('',(-1.,0.,0.));
#66027=DIRECTION('',(0.,0.,-1.));
#66028=DIRECTION('center_axis',(1.,0.,0.));
#66029=DIRECTION('ref_axis',(0.,-1.,0.));
#66030=DIRECTION('',(0.,-1.,0.));
#66031=DIRECTION('',(0.,0.,-1.));
#66032=DIRECTION('',(0.,-1.,0.));
#66033=DIRECTION('center_axis',(0.,1.,0.));
#66034=DIRECTION('ref_axis',(1.,0.,0.));
#66035=DIRECTION('',(1.,0.,0.));
#66036=DIRECTION('',(0.,0.,-1.));
#66037=DIRECTION('',(1.,0.,0.));
#66038=DIRECTION('center_axis',(-1.,0.,0.));
#66039=DIRECTION('ref_axis',(0.,1.,0.));
#66040=DIRECTION('',(0.,1.,0.));
#66041=DIRECTION('',(0.,1.,0.));
#66042=DIRECTION('center_axis',(0.,0.,-1.));
#66043=DIRECTION('ref_axis',(-1.,0.,0.));
#66044=DIRECTION('center_axis',(0.,-1.,0.));
#66045=DIRECTION('ref_axis',(-1.,0.,0.));
#66046=DIRECTION('',(-1.,0.,0.));
#66047=DIRECTION('',(0.,0.,-1.));
#66048=DIRECTION('',(-1.,0.,0.));
#66049=DIRECTION('',(0.,0.,-1.));
#66050=DIRECTION('center_axis',(1.,0.,0.));
#66051=DIRECTION('ref_axis',(0.,-1.,0.));
#66052=DIRECTION('',(0.,-1.,0.));
#66053=DIRECTION('',(0.,0.,-1.));
#66054=DIRECTION('',(0.,-1.,0.));
#66055=DIRECTION('center_axis',(0.,1.,0.));
#66056=DIRECTION('ref_axis',(1.,0.,0.));
#66057=DIRECTION('',(1.,0.,0.));
#66058=DIRECTION('',(0.,0.,-1.));
#66059=DIRECTION('',(1.,0.,0.));
#66060=DIRECTION('center_axis',(-1.,0.,0.));
#66061=DIRECTION('ref_axis',(0.,1.,0.));
#66062=DIRECTION('',(0.,1.,0.));
#66063=DIRECTION('',(0.,1.,0.));
#66064=DIRECTION('center_axis',(0.,0.,-1.));
#66065=DIRECTION('ref_axis',(-1.,0.,0.));
#66066=DIRECTION('center_axis',(0.,-1.,0.));
#66067=DIRECTION('ref_axis',(-1.,0.,0.));
#66068=DIRECTION('',(-1.,0.,0.));
#66069=DIRECTION('',(0.,0.,-1.));
#66070=DIRECTION('',(-1.,0.,0.));
#66071=DIRECTION('',(0.,0.,-1.));
#66072=DIRECTION('center_axis',(1.,0.,0.));
#66073=DIRECTION('ref_axis',(0.,-1.,0.));
#66074=DIRECTION('',(0.,-1.,0.));
#66075=DIRECTION('',(0.,0.,-1.));
#66076=DIRECTION('',(0.,-1.,0.));
#66077=DIRECTION('center_axis',(0.,1.,0.));
#66078=DIRECTION('ref_axis',(1.,0.,0.));
#66079=DIRECTION('',(1.,0.,0.));
#66080=DIRECTION('',(0.,0.,-1.));
#66081=DIRECTION('',(1.,0.,0.));
#66082=DIRECTION('center_axis',(-1.,0.,0.));
#66083=DIRECTION('ref_axis',(0.,1.,0.));
#66084=DIRECTION('',(0.,1.,0.));
#66085=DIRECTION('',(0.,1.,0.));
#66086=DIRECTION('center_axis',(0.,0.,-1.));
#66087=DIRECTION('ref_axis',(-1.,0.,0.));
#66088=DIRECTION('center_axis',(0.,-1.,0.));
#66089=DIRECTION('ref_axis',(-1.,0.,0.));
#66090=DIRECTION('',(-1.,0.,0.));
#66091=DIRECTION('',(0.,0.,-1.));
#66092=DIRECTION('',(-1.,0.,0.));
#66093=DIRECTION('',(0.,0.,-1.));
#66094=DIRECTION('center_axis',(1.,0.,0.));
#66095=DIRECTION('ref_axis',(0.,-1.,0.));
#66096=DIRECTION('',(0.,-1.,0.));
#66097=DIRECTION('',(0.,0.,-1.));
#66098=DIRECTION('',(0.,-1.,0.));
#66099=DIRECTION('center_axis',(0.,1.,0.));
#66100=DIRECTION('ref_axis',(1.,0.,0.));
#66101=DIRECTION('',(1.,0.,0.));
#66102=DIRECTION('',(0.,0.,-1.));
#66103=DIRECTION('',(1.,0.,0.));
#66104=DIRECTION('center_axis',(-1.,0.,0.));
#66105=DIRECTION('ref_axis',(0.,1.,0.));
#66106=DIRECTION('',(0.,1.,0.));
#66107=DIRECTION('',(0.,1.,0.));
#66108=DIRECTION('center_axis',(0.,0.,-1.));
#66109=DIRECTION('ref_axis',(-1.,0.,0.));
#66110=DIRECTION('center_axis',(0.,-1.,0.));
#66111=DIRECTION('ref_axis',(-1.,0.,0.));
#66112=DIRECTION('',(-1.,0.,0.));
#66113=DIRECTION('',(0.,0.,-1.));
#66114=DIRECTION('',(-1.,0.,0.));
#66115=DIRECTION('',(0.,0.,-1.));
#66116=DIRECTION('center_axis',(1.,0.,0.));
#66117=DIRECTION('ref_axis',(0.,-1.,0.));
#66118=DIRECTION('',(0.,-1.,0.));
#66119=DIRECTION('',(0.,0.,-1.));
#66120=DIRECTION('',(0.,-1.,0.));
#66121=DIRECTION('center_axis',(0.,1.,0.));
#66122=DIRECTION('ref_axis',(1.,0.,0.));
#66123=DIRECTION('',(1.,0.,0.));
#66124=DIRECTION('',(0.,0.,-1.));
#66125=DIRECTION('',(1.,0.,0.));
#66126=DIRECTION('center_axis',(-1.,0.,0.));
#66127=DIRECTION('ref_axis',(0.,1.,0.));
#66128=DIRECTION('',(0.,1.,0.));
#66129=DIRECTION('',(0.,1.,0.));
#66130=DIRECTION('center_axis',(0.,0.,-1.));
#66131=DIRECTION('ref_axis',(-1.,0.,0.));
#66132=DIRECTION('center_axis',(0.,-1.,0.));
#66133=DIRECTION('ref_axis',(-1.,0.,0.));
#66134=DIRECTION('',(-1.,0.,0.));
#66135=DIRECTION('',(0.,0.,-1.));
#66136=DIRECTION('',(-1.,0.,0.));
#66137=DIRECTION('',(0.,0.,-1.));
#66138=DIRECTION('center_axis',(1.,0.,0.));
#66139=DIRECTION('ref_axis',(0.,-1.,0.));
#66140=DIRECTION('',(0.,-1.,0.));
#66141=DIRECTION('',(0.,0.,-1.));
#66142=DIRECTION('',(0.,-1.,0.));
#66143=DIRECTION('center_axis',(0.,1.,0.));
#66144=DIRECTION('ref_axis',(1.,0.,0.));
#66145=DIRECTION('',(1.,0.,0.));
#66146=DIRECTION('',(0.,0.,-1.));
#66147=DIRECTION('',(1.,0.,0.));
#66148=DIRECTION('center_axis',(-1.,0.,0.));
#66149=DIRECTION('ref_axis',(0.,1.,0.));
#66150=DIRECTION('',(0.,1.,0.));
#66151=DIRECTION('',(0.,1.,0.));
#66152=DIRECTION('center_axis',(0.,0.,-1.));
#66153=DIRECTION('ref_axis',(-1.,0.,0.));
#66154=DIRECTION('center_axis',(0.,-1.,0.));
#66155=DIRECTION('ref_axis',(-1.,0.,0.));
#66156=DIRECTION('',(-1.,0.,0.));
#66157=DIRECTION('',(0.,0.,-1.));
#66158=DIRECTION('',(-1.,0.,0.));
#66159=DIRECTION('',(0.,0.,-1.));
#66160=DIRECTION('center_axis',(1.,0.,0.));
#66161=DIRECTION('ref_axis',(0.,-1.,0.));
#66162=DIRECTION('',(0.,-1.,0.));
#66163=DIRECTION('',(0.,0.,-1.));
#66164=DIRECTION('',(0.,-1.,0.));
#66165=DIRECTION('center_axis',(0.,1.,0.));
#66166=DIRECTION('ref_axis',(1.,0.,0.));
#66167=DIRECTION('',(1.,0.,0.));
#66168=DIRECTION('',(0.,0.,-1.));
#66169=DIRECTION('',(1.,0.,0.));
#66170=DIRECTION('center_axis',(-1.,0.,0.));
#66171=DIRECTION('ref_axis',(0.,1.,0.));
#66172=DIRECTION('',(0.,1.,0.));
#66173=DIRECTION('',(0.,1.,0.));
#66174=DIRECTION('center_axis',(0.,0.,-1.));
#66175=DIRECTION('ref_axis',(-1.,0.,0.));
#66176=DIRECTION('center_axis',(0.,-1.,0.));
#66177=DIRECTION('ref_axis',(-1.,0.,0.));
#66178=DIRECTION('',(-1.,0.,0.));
#66179=DIRECTION('',(0.,0.,-1.));
#66180=DIRECTION('',(-1.,0.,0.));
#66181=DIRECTION('',(0.,0.,-1.));
#66182=DIRECTION('center_axis',(1.,0.,0.));
#66183=DIRECTION('ref_axis',(0.,-1.,0.));
#66184=DIRECTION('',(0.,-1.,0.));
#66185=DIRECTION('',(0.,0.,-1.));
#66186=DIRECTION('',(0.,-1.,0.));
#66187=DIRECTION('center_axis',(0.,1.,0.));
#66188=DIRECTION('ref_axis',(1.,0.,0.));
#66189=DIRECTION('',(1.,0.,0.));
#66190=DIRECTION('',(0.,0.,-1.));
#66191=DIRECTION('',(1.,0.,0.));
#66192=DIRECTION('center_axis',(-1.,0.,0.));
#66193=DIRECTION('ref_axis',(0.,1.,0.));
#66194=DIRECTION('',(0.,1.,0.));
#66195=DIRECTION('',(0.,1.,0.));
#66196=DIRECTION('center_axis',(0.,0.,-1.));
#66197=DIRECTION('ref_axis',(-1.,0.,0.));
#66198=DIRECTION('center_axis',(0.,-1.,0.));
#66199=DIRECTION('ref_axis',(-1.,0.,0.));
#66200=DIRECTION('',(-1.,0.,0.));
#66201=DIRECTION('',(0.,0.,-1.));
#66202=DIRECTION('',(-1.,0.,0.));
#66203=DIRECTION('',(0.,0.,-1.));
#66204=DIRECTION('center_axis',(1.,0.,0.));
#66205=DIRECTION('ref_axis',(0.,-1.,0.));
#66206=DIRECTION('',(0.,-1.,0.));
#66207=DIRECTION('',(0.,0.,-1.));
#66208=DIRECTION('',(0.,-1.,0.));
#66209=DIRECTION('center_axis',(0.,1.,0.));
#66210=DIRECTION('ref_axis',(1.,0.,0.));
#66211=DIRECTION('',(1.,0.,0.));
#66212=DIRECTION('',(0.,0.,-1.));
#66213=DIRECTION('',(1.,0.,0.));
#66214=DIRECTION('center_axis',(-1.,0.,0.));
#66215=DIRECTION('ref_axis',(0.,1.,0.));
#66216=DIRECTION('',(0.,1.,0.));
#66217=DIRECTION('',(0.,1.,0.));
#66218=DIRECTION('center_axis',(0.,0.,-1.));
#66219=DIRECTION('ref_axis',(-1.,0.,0.));
#66220=DIRECTION('center_axis',(0.,-1.,0.));
#66221=DIRECTION('ref_axis',(-1.,0.,0.));
#66222=DIRECTION('',(-1.,0.,0.));
#66223=DIRECTION('',(0.,0.,-1.));
#66224=DIRECTION('',(-1.,0.,0.));
#66225=DIRECTION('',(0.,0.,-1.));
#66226=DIRECTION('center_axis',(1.,0.,0.));
#66227=DIRECTION('ref_axis',(0.,-1.,0.));
#66228=DIRECTION('',(0.,-1.,0.));
#66229=DIRECTION('',(0.,0.,-1.));
#66230=DIRECTION('',(0.,-1.,0.));
#66231=DIRECTION('center_axis',(0.,1.,0.));
#66232=DIRECTION('ref_axis',(1.,0.,0.));
#66233=DIRECTION('',(1.,0.,0.));
#66234=DIRECTION('',(0.,0.,-1.));
#66235=DIRECTION('',(1.,0.,0.));
#66236=DIRECTION('center_axis',(-1.,0.,0.));
#66237=DIRECTION('ref_axis',(0.,1.,0.));
#66238=DIRECTION('',(0.,1.,0.));
#66239=DIRECTION('',(0.,1.,0.));
#66240=DIRECTION('center_axis',(0.,0.,-1.));
#66241=DIRECTION('ref_axis',(-1.,0.,0.));
#66242=DIRECTION('center_axis',(0.,-1.,0.));
#66243=DIRECTION('ref_axis',(-1.,0.,0.));
#66244=DIRECTION('',(-1.,0.,0.));
#66245=DIRECTION('',(0.,0.,-1.));
#66246=DIRECTION('',(-1.,0.,0.));
#66247=DIRECTION('',(0.,0.,-1.));
#66248=DIRECTION('center_axis',(1.,0.,0.));
#66249=DIRECTION('ref_axis',(0.,-1.,0.));
#66250=DIRECTION('',(0.,-1.,0.));
#66251=DIRECTION('',(0.,0.,-1.));
#66252=DIRECTION('',(0.,-1.,0.));
#66253=DIRECTION('center_axis',(0.,1.,0.));
#66254=DIRECTION('ref_axis',(1.,0.,0.));
#66255=DIRECTION('',(1.,0.,0.));
#66256=DIRECTION('',(0.,0.,-1.));
#66257=DIRECTION('',(1.,0.,0.));
#66258=DIRECTION('center_axis',(-1.,0.,0.));
#66259=DIRECTION('ref_axis',(0.,1.,0.));
#66260=DIRECTION('',(0.,1.,0.));
#66261=DIRECTION('',(0.,1.,0.));
#66262=DIRECTION('center_axis',(0.,0.,-1.));
#66263=DIRECTION('ref_axis',(-1.,0.,0.));
#66264=DIRECTION('center_axis',(0.,-1.,0.));
#66265=DIRECTION('ref_axis',(-1.,0.,0.));
#66266=DIRECTION('',(-1.,0.,0.));
#66267=DIRECTION('',(0.,0.,-1.));
#66268=DIRECTION('',(-1.,0.,0.));
#66269=DIRECTION('',(0.,0.,-1.));
#66270=DIRECTION('center_axis',(1.,0.,0.));
#66271=DIRECTION('ref_axis',(0.,-1.,0.));
#66272=DIRECTION('',(0.,-1.,0.));
#66273=DIRECTION('',(0.,0.,-1.));
#66274=DIRECTION('',(0.,-1.,0.));
#66275=DIRECTION('center_axis',(0.,1.,0.));
#66276=DIRECTION('ref_axis',(1.,0.,0.));
#66277=DIRECTION('',(1.,0.,0.));
#66278=DIRECTION('',(0.,0.,-1.));
#66279=DIRECTION('',(1.,0.,0.));
#66280=DIRECTION('center_axis',(-1.,0.,0.));
#66281=DIRECTION('ref_axis',(0.,1.,0.));
#66282=DIRECTION('',(0.,1.,0.));
#66283=DIRECTION('',(0.,1.,0.));
#66284=DIRECTION('center_axis',(0.,0.,-1.));
#66285=DIRECTION('ref_axis',(-1.,0.,0.));
#66286=DIRECTION('center_axis',(0.,-1.,0.));
#66287=DIRECTION('ref_axis',(-1.,0.,0.));
#66288=DIRECTION('',(-1.,0.,0.));
#66289=DIRECTION('',(0.,0.,-1.));
#66290=DIRECTION('',(-1.,0.,0.));
#66291=DIRECTION('',(0.,0.,-1.));
#66292=DIRECTION('center_axis',(1.,0.,0.));
#66293=DIRECTION('ref_axis',(0.,-1.,0.));
#66294=DIRECTION('',(0.,-1.,0.));
#66295=DIRECTION('',(0.,0.,-1.));
#66296=DIRECTION('',(0.,-1.,0.));
#66297=DIRECTION('center_axis',(0.,1.,0.));
#66298=DIRECTION('ref_axis',(1.,0.,0.));
#66299=DIRECTION('',(1.,0.,0.));
#66300=DIRECTION('',(0.,0.,-1.));
#66301=DIRECTION('',(1.,0.,0.));
#66302=DIRECTION('center_axis',(-1.,0.,0.));
#66303=DIRECTION('ref_axis',(0.,1.,0.));
#66304=DIRECTION('',(0.,1.,0.));
#66305=DIRECTION('',(0.,1.,0.));
#66306=DIRECTION('center_axis',(0.,0.,-1.));
#66307=DIRECTION('ref_axis',(-1.,0.,0.));
#66308=DIRECTION('center_axis',(0.,-1.,0.));
#66309=DIRECTION('ref_axis',(-1.,0.,0.));
#66310=DIRECTION('',(-1.,0.,0.));
#66311=DIRECTION('',(0.,0.,-1.));
#66312=DIRECTION('',(-1.,0.,0.));
#66313=DIRECTION('',(0.,0.,-1.));
#66314=DIRECTION('center_axis',(1.,0.,0.));
#66315=DIRECTION('ref_axis',(0.,-1.,0.));
#66316=DIRECTION('',(0.,-1.,0.));
#66317=DIRECTION('',(0.,0.,-1.));
#66318=DIRECTION('',(0.,-1.,0.));
#66319=DIRECTION('center_axis',(0.,1.,0.));
#66320=DIRECTION('ref_axis',(1.,0.,0.));
#66321=DIRECTION('',(1.,0.,0.));
#66322=DIRECTION('',(0.,0.,-1.));
#66323=DIRECTION('',(1.,0.,0.));
#66324=DIRECTION('center_axis',(-1.,0.,0.));
#66325=DIRECTION('ref_axis',(0.,1.,0.));
#66326=DIRECTION('',(0.,1.,0.));
#66327=DIRECTION('',(0.,1.,0.));
#66328=DIRECTION('center_axis',(0.,0.,-1.));
#66329=DIRECTION('ref_axis',(-1.,0.,0.));
#66330=DIRECTION('center_axis',(0.,-1.,0.));
#66331=DIRECTION('ref_axis',(-1.,0.,0.));
#66332=DIRECTION('',(-1.,0.,0.));
#66333=DIRECTION('',(0.,0.,-1.));
#66334=DIRECTION('',(-1.,0.,0.));
#66335=DIRECTION('',(0.,0.,-1.));
#66336=DIRECTION('center_axis',(1.,0.,0.));
#66337=DIRECTION('ref_axis',(0.,-1.,0.));
#66338=DIRECTION('',(0.,-1.,0.));
#66339=DIRECTION('',(0.,0.,-1.));
#66340=DIRECTION('',(0.,-1.,0.));
#66341=DIRECTION('center_axis',(0.,1.,0.));
#66342=DIRECTION('ref_axis',(1.,0.,0.));
#66343=DIRECTION('',(1.,0.,0.));
#66344=DIRECTION('',(0.,0.,-1.));
#66345=DIRECTION('',(1.,0.,0.));
#66346=DIRECTION('center_axis',(-1.,0.,0.));
#66347=DIRECTION('ref_axis',(0.,1.,0.));
#66348=DIRECTION('',(0.,1.,0.));
#66349=DIRECTION('',(0.,1.,0.));
#66350=DIRECTION('center_axis',(0.,0.,-1.));
#66351=DIRECTION('ref_axis',(-1.,0.,0.));
#66352=DIRECTION('center_axis',(0.,-1.,0.));
#66353=DIRECTION('ref_axis',(-1.,0.,0.));
#66354=DIRECTION('',(-1.,0.,0.));
#66355=DIRECTION('',(0.,0.,-1.));
#66356=DIRECTION('',(-1.,0.,0.));
#66357=DIRECTION('',(0.,0.,-1.));
#66358=DIRECTION('center_axis',(1.,0.,0.));
#66359=DIRECTION('ref_axis',(0.,-1.,0.));
#66360=DIRECTION('',(0.,-1.,0.));
#66361=DIRECTION('',(0.,0.,-1.));
#66362=DIRECTION('',(0.,-1.,0.));
#66363=DIRECTION('center_axis',(0.,1.,0.));
#66364=DIRECTION('ref_axis',(1.,0.,0.));
#66365=DIRECTION('',(1.,0.,0.));
#66366=DIRECTION('',(0.,0.,-1.));
#66367=DIRECTION('',(1.,0.,0.));
#66368=DIRECTION('center_axis',(-1.,0.,0.));
#66369=DIRECTION('ref_axis',(0.,1.,0.));
#66370=DIRECTION('',(0.,1.,0.));
#66371=DIRECTION('',(0.,1.,0.));
#66372=DIRECTION('center_axis',(0.,0.,-1.));
#66373=DIRECTION('ref_axis',(-1.,0.,0.));
#66374=DIRECTION('center_axis',(0.,-1.,0.));
#66375=DIRECTION('ref_axis',(-1.,0.,0.));
#66376=DIRECTION('',(-1.,0.,0.));
#66377=DIRECTION('',(0.,0.,-1.));
#66378=DIRECTION('',(-1.,0.,0.));
#66379=DIRECTION('',(0.,0.,-1.));
#66380=DIRECTION('center_axis',(1.,0.,0.));
#66381=DIRECTION('ref_axis',(0.,-1.,0.));
#66382=DIRECTION('',(0.,-1.,0.));
#66383=DIRECTION('',(0.,0.,-1.));
#66384=DIRECTION('',(0.,-1.,0.));
#66385=DIRECTION('center_axis',(0.,1.,0.));
#66386=DIRECTION('ref_axis',(1.,0.,0.));
#66387=DIRECTION('',(1.,0.,0.));
#66388=DIRECTION('',(0.,0.,-1.));
#66389=DIRECTION('',(1.,0.,0.));
#66390=DIRECTION('center_axis',(-1.,0.,0.));
#66391=DIRECTION('ref_axis',(0.,1.,0.));
#66392=DIRECTION('',(0.,1.,0.));
#66393=DIRECTION('',(0.,1.,0.));
#66394=DIRECTION('center_axis',(0.,0.,-1.));
#66395=DIRECTION('ref_axis',(-1.,0.,0.));
#66396=DIRECTION('center_axis',(0.,-1.,0.));
#66397=DIRECTION('ref_axis',(-1.,0.,0.));
#66398=DIRECTION('',(-1.,0.,0.));
#66399=DIRECTION('',(0.,0.,-1.));
#66400=DIRECTION('',(-1.,0.,0.));
#66401=DIRECTION('',(0.,0.,-1.));
#66402=DIRECTION('center_axis',(1.,0.,0.));
#66403=DIRECTION('ref_axis',(0.,-1.,0.));
#66404=DIRECTION('',(0.,-1.,0.));
#66405=DIRECTION('',(0.,0.,-1.));
#66406=DIRECTION('',(0.,-1.,0.));
#66407=DIRECTION('center_axis',(0.,1.,0.));
#66408=DIRECTION('ref_axis',(1.,0.,0.));
#66409=DIRECTION('',(1.,0.,0.));
#66410=DIRECTION('',(0.,0.,-1.));
#66411=DIRECTION('',(1.,0.,0.));
#66412=DIRECTION('center_axis',(-1.,0.,0.));
#66413=DIRECTION('ref_axis',(0.,1.,0.));
#66414=DIRECTION('',(0.,1.,0.));
#66415=DIRECTION('',(0.,1.,0.));
#66416=DIRECTION('center_axis',(0.,0.,-1.));
#66417=DIRECTION('ref_axis',(-1.,0.,0.));
#66418=DIRECTION('center_axis',(0.,-1.,0.));
#66419=DIRECTION('ref_axis',(-1.,0.,0.));
#66420=DIRECTION('',(-1.,0.,0.));
#66421=DIRECTION('',(0.,0.,-1.));
#66422=DIRECTION('',(-1.,0.,0.));
#66423=DIRECTION('',(0.,0.,-1.));
#66424=DIRECTION('center_axis',(1.,0.,0.));
#66425=DIRECTION('ref_axis',(0.,-1.,0.));
#66426=DIRECTION('',(0.,-1.,0.));
#66427=DIRECTION('',(0.,0.,-1.));
#66428=DIRECTION('',(0.,-1.,0.));
#66429=DIRECTION('center_axis',(0.,1.,0.));
#66430=DIRECTION('ref_axis',(1.,0.,0.));
#66431=DIRECTION('',(1.,0.,0.));
#66432=DIRECTION('',(0.,0.,-1.));
#66433=DIRECTION('',(1.,0.,0.));
#66434=DIRECTION('center_axis',(-1.,0.,0.));
#66435=DIRECTION('ref_axis',(0.,1.,0.));
#66436=DIRECTION('',(0.,1.,0.));
#66437=DIRECTION('',(0.,1.,0.));
#66438=DIRECTION('center_axis',(0.,0.,-1.));
#66439=DIRECTION('ref_axis',(-1.,0.,0.));
#66440=DIRECTION('center_axis',(0.,-1.,0.));
#66441=DIRECTION('ref_axis',(-1.,0.,0.));
#66442=DIRECTION('',(-1.,0.,0.));
#66443=DIRECTION('',(0.,0.,-1.));
#66444=DIRECTION('',(-1.,0.,0.));
#66445=DIRECTION('',(0.,0.,-1.));
#66446=DIRECTION('center_axis',(1.,0.,0.));
#66447=DIRECTION('ref_axis',(0.,-1.,0.));
#66448=DIRECTION('',(0.,-1.,0.));
#66449=DIRECTION('',(0.,0.,-1.));
#66450=DIRECTION('',(0.,-1.,0.));
#66451=DIRECTION('center_axis',(0.,1.,0.));
#66452=DIRECTION('ref_axis',(1.,0.,0.));
#66453=DIRECTION('',(1.,0.,0.));
#66454=DIRECTION('',(0.,0.,-1.));
#66455=DIRECTION('',(1.,0.,0.));
#66456=DIRECTION('center_axis',(-1.,0.,0.));
#66457=DIRECTION('ref_axis',(0.,1.,0.));
#66458=DIRECTION('',(0.,1.,0.));
#66459=DIRECTION('',(0.,1.,0.));
#66460=DIRECTION('center_axis',(0.,0.,-1.));
#66461=DIRECTION('ref_axis',(-1.,0.,0.));
#66462=DIRECTION('center_axis',(0.,-1.,0.));
#66463=DIRECTION('ref_axis',(-1.,0.,0.));
#66464=DIRECTION('',(-1.,0.,0.));
#66465=DIRECTION('',(0.,0.,-1.));
#66466=DIRECTION('',(-1.,0.,0.));
#66467=DIRECTION('',(0.,0.,-1.));
#66468=DIRECTION('center_axis',(1.,0.,0.));
#66469=DIRECTION('ref_axis',(0.,-1.,0.));
#66470=DIRECTION('',(0.,-1.,0.));
#66471=DIRECTION('',(0.,0.,-1.));
#66472=DIRECTION('',(0.,-1.,0.));
#66473=DIRECTION('center_axis',(0.,1.,0.));
#66474=DIRECTION('ref_axis',(1.,0.,0.));
#66475=DIRECTION('',(1.,0.,0.));
#66476=DIRECTION('',(0.,0.,-1.));
#66477=DIRECTION('',(1.,0.,0.));
#66478=DIRECTION('center_axis',(-1.,0.,0.));
#66479=DIRECTION('ref_axis',(0.,1.,0.));
#66480=DIRECTION('',(0.,1.,0.));
#66481=DIRECTION('',(0.,1.,0.));
#66482=DIRECTION('center_axis',(0.,0.,-1.));
#66483=DIRECTION('ref_axis',(-1.,0.,0.));
#66484=DIRECTION('center_axis',(0.,-1.,0.));
#66485=DIRECTION('ref_axis',(-1.,0.,0.));
#66486=DIRECTION('',(-1.,0.,0.));
#66487=DIRECTION('',(0.,0.,-1.));
#66488=DIRECTION('',(-1.,0.,0.));
#66489=DIRECTION('',(0.,0.,-1.));
#66490=DIRECTION('center_axis',(1.,0.,0.));
#66491=DIRECTION('ref_axis',(0.,-1.,0.));
#66492=DIRECTION('',(0.,-1.,0.));
#66493=DIRECTION('',(0.,0.,-1.));
#66494=DIRECTION('',(0.,-1.,0.));
#66495=DIRECTION('center_axis',(0.,1.,0.));
#66496=DIRECTION('ref_axis',(1.,0.,0.));
#66497=DIRECTION('',(1.,0.,0.));
#66498=DIRECTION('',(0.,0.,-1.));
#66499=DIRECTION('',(1.,0.,0.));
#66500=DIRECTION('center_axis',(-1.,0.,0.));
#66501=DIRECTION('ref_axis',(0.,1.,0.));
#66502=DIRECTION('',(0.,1.,0.));
#66503=DIRECTION('',(0.,1.,0.));
#66504=DIRECTION('center_axis',(0.,0.,-1.));
#66505=DIRECTION('ref_axis',(-1.,0.,0.));
#66506=DIRECTION('center_axis',(0.,-1.,0.));
#66507=DIRECTION('ref_axis',(-1.,0.,0.));
#66508=DIRECTION('',(-1.,0.,0.));
#66509=DIRECTION('',(0.,0.,-1.));
#66510=DIRECTION('',(-1.,0.,0.));
#66511=DIRECTION('',(0.,0.,-1.));
#66512=DIRECTION('center_axis',(1.,0.,0.));
#66513=DIRECTION('ref_axis',(0.,-1.,0.));
#66514=DIRECTION('',(0.,-1.,0.));
#66515=DIRECTION('',(0.,0.,-1.));
#66516=DIRECTION('',(0.,-1.,0.));
#66517=DIRECTION('center_axis',(0.,1.,0.));
#66518=DIRECTION('ref_axis',(1.,0.,0.));
#66519=DIRECTION('',(1.,0.,0.));
#66520=DIRECTION('',(0.,0.,-1.));
#66521=DIRECTION('',(1.,0.,0.));
#66522=DIRECTION('center_axis',(-1.,0.,0.));
#66523=DIRECTION('ref_axis',(0.,1.,0.));
#66524=DIRECTION('',(0.,1.,0.));
#66525=DIRECTION('',(0.,1.,0.));
#66526=DIRECTION('center_axis',(0.,0.,-1.));
#66527=DIRECTION('ref_axis',(-1.,0.,0.));
#66528=DIRECTION('center_axis',(0.,-1.,0.));
#66529=DIRECTION('ref_axis',(-1.,0.,0.));
#66530=DIRECTION('',(-1.,0.,0.));
#66531=DIRECTION('',(0.,0.,-1.));
#66532=DIRECTION('',(-1.,0.,0.));
#66533=DIRECTION('',(0.,0.,-1.));
#66534=DIRECTION('center_axis',(1.,0.,0.));
#66535=DIRECTION('ref_axis',(0.,-1.,0.));
#66536=DIRECTION('',(0.,-1.,0.));
#66537=DIRECTION('',(0.,0.,-1.));
#66538=DIRECTION('',(0.,-1.,0.));
#66539=DIRECTION('center_axis',(0.,1.,0.));
#66540=DIRECTION('ref_axis',(1.,0.,0.));
#66541=DIRECTION('',(1.,0.,0.));
#66542=DIRECTION('',(0.,0.,-1.));
#66543=DIRECTION('',(1.,0.,0.));
#66544=DIRECTION('center_axis',(-1.,0.,0.));
#66545=DIRECTION('ref_axis',(0.,1.,0.));
#66546=DIRECTION('',(0.,1.,0.));
#66547=DIRECTION('',(0.,1.,0.));
#66548=DIRECTION('center_axis',(0.,0.,-1.));
#66549=DIRECTION('ref_axis',(-1.,0.,0.));
#66550=DIRECTION('center_axis',(0.,-1.,0.));
#66551=DIRECTION('ref_axis',(-1.,0.,0.));
#66552=DIRECTION('',(-1.,0.,0.));
#66553=DIRECTION('',(0.,0.,-1.));
#66554=DIRECTION('',(-1.,0.,0.));
#66555=DIRECTION('',(0.,0.,-1.));
#66556=DIRECTION('center_axis',(1.,0.,0.));
#66557=DIRECTION('ref_axis',(0.,-1.,0.));
#66558=DIRECTION('',(0.,-1.,0.));
#66559=DIRECTION('',(0.,0.,-1.));
#66560=DIRECTION('',(0.,-1.,0.));
#66561=DIRECTION('center_axis',(0.,1.,0.));
#66562=DIRECTION('ref_axis',(1.,0.,0.));
#66563=DIRECTION('',(1.,0.,0.));
#66564=DIRECTION('',(0.,0.,-1.));
#66565=DIRECTION('',(1.,0.,0.));
#66566=DIRECTION('center_axis',(-1.,0.,0.));
#66567=DIRECTION('ref_axis',(0.,1.,0.));
#66568=DIRECTION('',(0.,1.,0.));
#66569=DIRECTION('',(0.,1.,0.));
#66570=DIRECTION('center_axis',(0.,0.,-1.));
#66571=DIRECTION('ref_axis',(-1.,0.,0.));
#66572=DIRECTION('center_axis',(0.,-1.,0.));
#66573=DIRECTION('ref_axis',(-1.,0.,0.));
#66574=DIRECTION('',(-1.,0.,0.));
#66575=DIRECTION('',(0.,0.,-1.));
#66576=DIRECTION('',(-1.,0.,0.));
#66577=DIRECTION('',(0.,0.,-1.));
#66578=DIRECTION('center_axis',(1.,0.,0.));
#66579=DIRECTION('ref_axis',(0.,-1.,0.));
#66580=DIRECTION('',(0.,-1.,0.));
#66581=DIRECTION('',(0.,0.,-1.));
#66582=DIRECTION('',(0.,-1.,0.));
#66583=DIRECTION('center_axis',(0.,1.,0.));
#66584=DIRECTION('ref_axis',(1.,0.,0.));
#66585=DIRECTION('',(1.,0.,0.));
#66586=DIRECTION('',(0.,0.,-1.));
#66587=DIRECTION('',(1.,0.,0.));
#66588=DIRECTION('center_axis',(-1.,0.,0.));
#66589=DIRECTION('ref_axis',(0.,1.,0.));
#66590=DIRECTION('',(0.,1.,0.));
#66591=DIRECTION('',(0.,1.,0.));
#66592=DIRECTION('center_axis',(0.,0.,-1.));
#66593=DIRECTION('ref_axis',(-1.,0.,0.));
#66594=DIRECTION('center_axis',(0.,-1.,0.));
#66595=DIRECTION('ref_axis',(-1.,0.,0.));
#66596=DIRECTION('',(-1.,0.,0.));
#66597=DIRECTION('',(0.,0.,-1.));
#66598=DIRECTION('',(-1.,0.,0.));
#66599=DIRECTION('',(0.,0.,-1.));
#66600=DIRECTION('center_axis',(1.,0.,0.));
#66601=DIRECTION('ref_axis',(0.,-1.,0.));
#66602=DIRECTION('',(0.,-1.,0.));
#66603=DIRECTION('',(0.,0.,-1.));
#66604=DIRECTION('',(0.,-1.,0.));
#66605=DIRECTION('center_axis',(0.,1.,0.));
#66606=DIRECTION('ref_axis',(1.,0.,0.));
#66607=DIRECTION('',(1.,0.,0.));
#66608=DIRECTION('',(0.,0.,-1.));
#66609=DIRECTION('',(1.,0.,0.));
#66610=DIRECTION('center_axis',(-1.,0.,0.));
#66611=DIRECTION('ref_axis',(0.,1.,0.));
#66612=DIRECTION('',(0.,1.,0.));
#66613=DIRECTION('',(0.,1.,0.));
#66614=DIRECTION('center_axis',(0.,0.,-1.));
#66615=DIRECTION('ref_axis',(-1.,0.,0.));
#66616=DIRECTION('center_axis',(0.,-1.,0.));
#66617=DIRECTION('ref_axis',(-1.,0.,0.));
#66618=DIRECTION('',(-1.,0.,0.));
#66619=DIRECTION('',(0.,0.,-1.));
#66620=DIRECTION('',(-1.,0.,0.));
#66621=DIRECTION('',(0.,0.,-1.));
#66622=DIRECTION('center_axis',(1.,0.,0.));
#66623=DIRECTION('ref_axis',(0.,-1.,0.));
#66624=DIRECTION('',(0.,-1.,0.));
#66625=DIRECTION('',(0.,0.,-1.));
#66626=DIRECTION('',(0.,-1.,0.));
#66627=DIRECTION('center_axis',(0.,1.,0.));
#66628=DIRECTION('ref_axis',(1.,0.,0.));
#66629=DIRECTION('',(1.,0.,0.));
#66630=DIRECTION('',(0.,0.,-1.));
#66631=DIRECTION('',(1.,0.,0.));
#66632=DIRECTION('center_axis',(-1.,0.,0.));
#66633=DIRECTION('ref_axis',(0.,1.,0.));
#66634=DIRECTION('',(0.,1.,0.));
#66635=DIRECTION('',(0.,1.,0.));
#66636=DIRECTION('center_axis',(0.,0.,-1.));
#66637=DIRECTION('ref_axis',(-1.,0.,0.));
#66638=DIRECTION('center_axis',(0.,-1.,0.));
#66639=DIRECTION('ref_axis',(-1.,0.,0.));
#66640=DIRECTION('',(-1.,0.,0.));
#66641=DIRECTION('',(0.,0.,-1.));
#66642=DIRECTION('',(-1.,0.,0.));
#66643=DIRECTION('',(0.,0.,-1.));
#66644=DIRECTION('center_axis',(1.,0.,0.));
#66645=DIRECTION('ref_axis',(0.,-1.,0.));
#66646=DIRECTION('',(0.,-1.,0.));
#66647=DIRECTION('',(0.,0.,-1.));
#66648=DIRECTION('',(0.,-1.,0.));
#66649=DIRECTION('center_axis',(0.,1.,0.));
#66650=DIRECTION('ref_axis',(1.,0.,0.));
#66651=DIRECTION('',(1.,0.,0.));
#66652=DIRECTION('',(0.,0.,-1.));
#66653=DIRECTION('',(1.,0.,0.));
#66654=DIRECTION('center_axis',(-1.,0.,0.));
#66655=DIRECTION('ref_axis',(0.,1.,0.));
#66656=DIRECTION('',(0.,1.,0.));
#66657=DIRECTION('',(0.,1.,0.));
#66658=DIRECTION('center_axis',(0.,0.,-1.));
#66659=DIRECTION('ref_axis',(-1.,0.,0.));
#66660=DIRECTION('center_axis',(0.,-1.,0.));
#66661=DIRECTION('ref_axis',(-1.,0.,0.));
#66662=DIRECTION('',(-1.,0.,0.));
#66663=DIRECTION('',(0.,0.,-1.));
#66664=DIRECTION('',(-1.,0.,0.));
#66665=DIRECTION('',(0.,0.,-1.));
#66666=DIRECTION('center_axis',(1.,0.,0.));
#66667=DIRECTION('ref_axis',(0.,-1.,0.));
#66668=DIRECTION('',(0.,-1.,0.));
#66669=DIRECTION('',(0.,0.,-1.));
#66670=DIRECTION('',(0.,-1.,0.));
#66671=DIRECTION('center_axis',(0.,1.,0.));
#66672=DIRECTION('ref_axis',(1.,0.,0.));
#66673=DIRECTION('',(1.,0.,0.));
#66674=DIRECTION('',(0.,0.,-1.));
#66675=DIRECTION('',(1.,0.,0.));
#66676=DIRECTION('center_axis',(-1.,0.,0.));
#66677=DIRECTION('ref_axis',(0.,1.,0.));
#66678=DIRECTION('',(0.,1.,0.));
#66679=DIRECTION('',(0.,1.,0.));
#66680=DIRECTION('center_axis',(0.,0.,-1.));
#66681=DIRECTION('ref_axis',(-1.,0.,0.));
#66682=DIRECTION('center_axis',(0.,-1.,0.));
#66683=DIRECTION('ref_axis',(-1.,0.,0.));
#66684=DIRECTION('',(-1.,0.,0.));
#66685=DIRECTION('',(0.,0.,-1.));
#66686=DIRECTION('',(-1.,0.,0.));
#66687=DIRECTION('',(0.,0.,-1.));
#66688=DIRECTION('center_axis',(1.,0.,0.));
#66689=DIRECTION('ref_axis',(0.,-1.,0.));
#66690=DIRECTION('',(0.,-1.,0.));
#66691=DIRECTION('',(0.,0.,-1.));
#66692=DIRECTION('',(0.,-1.,0.));
#66693=DIRECTION('center_axis',(0.,1.,0.));
#66694=DIRECTION('ref_axis',(1.,0.,0.));
#66695=DIRECTION('',(1.,0.,0.));
#66696=DIRECTION('',(0.,0.,-1.));
#66697=DIRECTION('',(1.,0.,0.));
#66698=DIRECTION('center_axis',(-1.,0.,0.));
#66699=DIRECTION('ref_axis',(0.,1.,0.));
#66700=DIRECTION('',(0.,1.,0.));
#66701=DIRECTION('',(0.,1.,0.));
#66702=DIRECTION('center_axis',(0.,0.,-1.));
#66703=DIRECTION('ref_axis',(-1.,0.,0.));
#66704=DIRECTION('center_axis',(0.,-1.,0.));
#66705=DIRECTION('ref_axis',(-1.,0.,0.));
#66706=DIRECTION('',(-1.,0.,0.));
#66707=DIRECTION('',(0.,0.,-1.));
#66708=DIRECTION('',(-1.,0.,0.));
#66709=DIRECTION('',(0.,0.,-1.));
#66710=DIRECTION('center_axis',(1.,0.,0.));
#66711=DIRECTION('ref_axis',(0.,-1.,0.));
#66712=DIRECTION('',(0.,-1.,0.));
#66713=DIRECTION('',(0.,0.,-1.));
#66714=DIRECTION('',(0.,-1.,0.));
#66715=DIRECTION('center_axis',(0.,1.,0.));
#66716=DIRECTION('ref_axis',(1.,0.,0.));
#66717=DIRECTION('',(1.,0.,0.));
#66718=DIRECTION('',(0.,0.,-1.));
#66719=DIRECTION('',(1.,0.,0.));
#66720=DIRECTION('center_axis',(-1.,0.,0.));
#66721=DIRECTION('ref_axis',(0.,1.,0.));
#66722=DIRECTION('',(0.,1.,0.));
#66723=DIRECTION('',(0.,1.,0.));
#66724=DIRECTION('center_axis',(0.,0.,-1.));
#66725=DIRECTION('ref_axis',(-1.,0.,0.));
#66726=DIRECTION('center_axis',(0.,-1.,0.));
#66727=DIRECTION('ref_axis',(-1.,0.,0.));
#66728=DIRECTION('',(-1.,0.,0.));
#66729=DIRECTION('',(0.,0.,-1.));
#66730=DIRECTION('',(-1.,0.,0.));
#66731=DIRECTION('',(0.,0.,-1.));
#66732=DIRECTION('center_axis',(1.,0.,0.));
#66733=DIRECTION('ref_axis',(0.,-1.,0.));
#66734=DIRECTION('',(0.,-1.,0.));
#66735=DIRECTION('',(0.,0.,-1.));
#66736=DIRECTION('',(0.,-1.,0.));
#66737=DIRECTION('center_axis',(0.,1.,0.));
#66738=DIRECTION('ref_axis',(1.,0.,0.));
#66739=DIRECTION('',(1.,0.,0.));
#66740=DIRECTION('',(0.,0.,-1.));
#66741=DIRECTION('',(1.,0.,0.));
#66742=DIRECTION('center_axis',(-1.,0.,0.));
#66743=DIRECTION('ref_axis',(0.,1.,0.));
#66744=DIRECTION('',(0.,1.,0.));
#66745=DIRECTION('',(0.,1.,0.));
#66746=DIRECTION('center_axis',(0.,0.,-1.));
#66747=DIRECTION('ref_axis',(-1.,0.,0.));
#66748=DIRECTION('center_axis',(0.,-1.,0.));
#66749=DIRECTION('ref_axis',(-1.,0.,0.));
#66750=DIRECTION('',(-1.,0.,0.));
#66751=DIRECTION('',(0.,0.,-1.));
#66752=DIRECTION('',(-1.,0.,0.));
#66753=DIRECTION('',(0.,0.,-1.));
#66754=DIRECTION('center_axis',(1.,0.,0.));
#66755=DIRECTION('ref_axis',(0.,-1.,0.));
#66756=DIRECTION('',(0.,-1.,0.));
#66757=DIRECTION('',(0.,0.,-1.));
#66758=DIRECTION('',(0.,-1.,0.));
#66759=DIRECTION('center_axis',(0.,1.,0.));
#66760=DIRECTION('ref_axis',(1.,0.,0.));
#66761=DIRECTION('',(1.,0.,0.));
#66762=DIRECTION('',(0.,0.,-1.));
#66763=DIRECTION('',(1.,0.,0.));
#66764=DIRECTION('center_axis',(-1.,0.,0.));
#66765=DIRECTION('ref_axis',(0.,1.,0.));
#66766=DIRECTION('',(0.,1.,0.));
#66767=DIRECTION('',(0.,1.,0.));
#66768=DIRECTION('center_axis',(0.,0.,-1.));
#66769=DIRECTION('ref_axis',(-1.,0.,0.));
#66770=DIRECTION('center_axis',(0.,-1.,0.));
#66771=DIRECTION('ref_axis',(-1.,0.,0.));
#66772=DIRECTION('',(-1.,0.,0.));
#66773=DIRECTION('',(0.,0.,-1.));
#66774=DIRECTION('',(-1.,0.,0.));
#66775=DIRECTION('',(0.,0.,-1.));
#66776=DIRECTION('center_axis',(1.,0.,0.));
#66777=DIRECTION('ref_axis',(0.,-1.,0.));
#66778=DIRECTION('',(0.,-1.,0.));
#66779=DIRECTION('',(0.,0.,-1.));
#66780=DIRECTION('',(0.,-1.,0.));
#66781=DIRECTION('center_axis',(0.,1.,0.));
#66782=DIRECTION('ref_axis',(1.,0.,0.));
#66783=DIRECTION('',(1.,0.,0.));
#66784=DIRECTION('',(0.,0.,-1.));
#66785=DIRECTION('',(1.,0.,0.));
#66786=DIRECTION('center_axis',(-1.,0.,0.));
#66787=DIRECTION('ref_axis',(0.,1.,0.));
#66788=DIRECTION('',(0.,1.,0.));
#66789=DIRECTION('',(0.,1.,0.));
#66790=DIRECTION('center_axis',(0.,0.,-1.));
#66791=DIRECTION('ref_axis',(-1.,0.,0.));
#66792=DIRECTION('center_axis',(0.,-1.,0.));
#66793=DIRECTION('ref_axis',(-1.,0.,0.));
#66794=DIRECTION('',(-1.,0.,0.));
#66795=DIRECTION('',(0.,0.,-1.));
#66796=DIRECTION('',(-1.,0.,0.));
#66797=DIRECTION('',(0.,0.,-1.));
#66798=DIRECTION('center_axis',(1.,0.,0.));
#66799=DIRECTION('ref_axis',(0.,-1.,0.));
#66800=DIRECTION('',(0.,-1.,0.));
#66801=DIRECTION('',(0.,0.,-1.));
#66802=DIRECTION('',(0.,-1.,0.));
#66803=DIRECTION('center_axis',(0.,1.,0.));
#66804=DIRECTION('ref_axis',(1.,0.,0.));
#66805=DIRECTION('',(1.,0.,0.));
#66806=DIRECTION('',(0.,0.,-1.));
#66807=DIRECTION('',(1.,0.,0.));
#66808=DIRECTION('center_axis',(-1.,0.,0.));
#66809=DIRECTION('ref_axis',(0.,1.,0.));
#66810=DIRECTION('',(0.,1.,0.));
#66811=DIRECTION('',(0.,1.,0.));
#66812=DIRECTION('center_axis',(0.,0.,-1.));
#66813=DIRECTION('ref_axis',(-1.,0.,0.));
#66814=DIRECTION('center_axis',(0.,-1.,0.));
#66815=DIRECTION('ref_axis',(-1.,0.,0.));
#66816=DIRECTION('',(-1.,0.,0.));
#66817=DIRECTION('',(0.,0.,-1.));
#66818=DIRECTION('',(-1.,0.,0.));
#66819=DIRECTION('',(0.,0.,-1.));
#66820=DIRECTION('center_axis',(1.,0.,0.));
#66821=DIRECTION('ref_axis',(0.,-1.,0.));
#66822=DIRECTION('',(0.,-1.,0.));
#66823=DIRECTION('',(0.,0.,-1.));
#66824=DIRECTION('',(0.,-1.,0.));
#66825=DIRECTION('center_axis',(0.,1.,0.));
#66826=DIRECTION('ref_axis',(1.,0.,0.));
#66827=DIRECTION('',(1.,0.,0.));
#66828=DIRECTION('',(0.,0.,-1.));
#66829=DIRECTION('',(1.,0.,0.));
#66830=DIRECTION('center_axis',(-1.,0.,0.));
#66831=DIRECTION('ref_axis',(0.,1.,0.));
#66832=DIRECTION('',(0.,1.,0.));
#66833=DIRECTION('',(0.,1.,0.));
#66834=DIRECTION('center_axis',(0.,0.,-1.));
#66835=DIRECTION('ref_axis',(-1.,0.,0.));
#66836=DIRECTION('center_axis',(0.,-1.,0.));
#66837=DIRECTION('ref_axis',(-1.,0.,0.));
#66838=DIRECTION('',(-1.,0.,0.));
#66839=DIRECTION('',(0.,0.,-1.));
#66840=DIRECTION('',(-1.,0.,0.));
#66841=DIRECTION('',(0.,0.,-1.));
#66842=DIRECTION('center_axis',(1.,0.,0.));
#66843=DIRECTION('ref_axis',(0.,-1.,0.));
#66844=DIRECTION('',(0.,-1.,0.));
#66845=DIRECTION('',(0.,0.,-1.));
#66846=DIRECTION('',(0.,-1.,0.));
#66847=DIRECTION('center_axis',(0.,1.,0.));
#66848=DIRECTION('ref_axis',(1.,0.,0.));
#66849=DIRECTION('',(1.,0.,0.));
#66850=DIRECTION('',(0.,0.,-1.));
#66851=DIRECTION('',(1.,0.,0.));
#66852=DIRECTION('center_axis',(-1.,0.,0.));
#66853=DIRECTION('ref_axis',(0.,1.,0.));
#66854=DIRECTION('',(0.,1.,0.));
#66855=DIRECTION('',(0.,1.,0.));
#66856=DIRECTION('center_axis',(0.,0.,-1.));
#66857=DIRECTION('ref_axis',(-1.,0.,0.));
#66858=DIRECTION('center_axis',(0.,-1.,0.));
#66859=DIRECTION('ref_axis',(-1.,0.,0.));
#66860=DIRECTION('',(-1.,0.,0.));
#66861=DIRECTION('',(0.,0.,-1.));
#66862=DIRECTION('',(-1.,0.,0.));
#66863=DIRECTION('',(0.,0.,-1.));
#66864=DIRECTION('center_axis',(1.,0.,0.));
#66865=DIRECTION('ref_axis',(0.,-1.,0.));
#66866=DIRECTION('',(0.,-1.,0.));
#66867=DIRECTION('',(0.,0.,-1.));
#66868=DIRECTION('',(0.,-1.,0.));
#66869=DIRECTION('center_axis',(0.,1.,0.));
#66870=DIRECTION('ref_axis',(1.,0.,0.));
#66871=DIRECTION('',(1.,0.,0.));
#66872=DIRECTION('',(0.,0.,-1.));
#66873=DIRECTION('',(1.,0.,0.));
#66874=DIRECTION('center_axis',(-1.,0.,0.));
#66875=DIRECTION('ref_axis',(0.,1.,0.));
#66876=DIRECTION('',(0.,1.,0.));
#66877=DIRECTION('',(0.,1.,0.));
#66878=DIRECTION('center_axis',(0.,0.,-1.));
#66879=DIRECTION('ref_axis',(-1.,0.,0.));
#66880=DIRECTION('center_axis',(0.,-1.,0.));
#66881=DIRECTION('ref_axis',(-1.,0.,0.));
#66882=DIRECTION('',(-1.,0.,0.));
#66883=DIRECTION('',(0.,0.,-1.));
#66884=DIRECTION('',(-1.,0.,0.));
#66885=DIRECTION('',(0.,0.,-1.));
#66886=DIRECTION('center_axis',(1.,0.,0.));
#66887=DIRECTION('ref_axis',(0.,-1.,0.));
#66888=DIRECTION('',(0.,-1.,0.));
#66889=DIRECTION('',(0.,0.,-1.));
#66890=DIRECTION('',(0.,-1.,0.));
#66891=DIRECTION('center_axis',(0.,1.,0.));
#66892=DIRECTION('ref_axis',(1.,0.,0.));
#66893=DIRECTION('',(1.,0.,0.));
#66894=DIRECTION('',(0.,0.,-1.));
#66895=DIRECTION('',(1.,0.,0.));
#66896=DIRECTION('center_axis',(-1.,0.,0.));
#66897=DIRECTION('ref_axis',(0.,1.,0.));
#66898=DIRECTION('',(0.,1.,0.));
#66899=DIRECTION('',(0.,1.,0.));
#66900=DIRECTION('center_axis',(0.,0.,-1.));
#66901=DIRECTION('ref_axis',(-1.,0.,0.));
#66902=DIRECTION('center_axis',(0.,-1.,0.));
#66903=DIRECTION('ref_axis',(-1.,0.,0.));
#66904=DIRECTION('',(-1.,0.,0.));
#66905=DIRECTION('',(0.,0.,-1.));
#66906=DIRECTION('',(-1.,0.,0.));
#66907=DIRECTION('',(0.,0.,-1.));
#66908=DIRECTION('center_axis',(1.,0.,0.));
#66909=DIRECTION('ref_axis',(0.,-1.,0.));
#66910=DIRECTION('',(0.,-1.,0.));
#66911=DIRECTION('',(0.,0.,-1.));
#66912=DIRECTION('',(0.,-1.,0.));
#66913=DIRECTION('center_axis',(0.,1.,0.));
#66914=DIRECTION('ref_axis',(1.,0.,0.));
#66915=DIRECTION('',(1.,0.,0.));
#66916=DIRECTION('',(0.,0.,-1.));
#66917=DIRECTION('',(1.,0.,0.));
#66918=DIRECTION('center_axis',(-1.,0.,0.));
#66919=DIRECTION('ref_axis',(0.,1.,0.));
#66920=DIRECTION('',(0.,1.,0.));
#66921=DIRECTION('',(0.,1.,0.));
#66922=DIRECTION('center_axis',(0.,0.,-1.));
#66923=DIRECTION('ref_axis',(-1.,0.,0.));
#66924=DIRECTION('center_axis',(0.,-1.,0.));
#66925=DIRECTION('ref_axis',(-1.,0.,0.));
#66926=DIRECTION('',(-1.,0.,0.));
#66927=DIRECTION('',(0.,0.,-1.));
#66928=DIRECTION('',(-1.,0.,0.));
#66929=DIRECTION('',(0.,0.,-1.));
#66930=DIRECTION('center_axis',(1.,0.,0.));
#66931=DIRECTION('ref_axis',(0.,-1.,0.));
#66932=DIRECTION('',(0.,-1.,0.));
#66933=DIRECTION('',(0.,0.,-1.));
#66934=DIRECTION('',(0.,-1.,0.));
#66935=DIRECTION('center_axis',(0.,1.,0.));
#66936=DIRECTION('ref_axis',(1.,0.,0.));
#66937=DIRECTION('',(1.,0.,0.));
#66938=DIRECTION('',(0.,0.,-1.));
#66939=DIRECTION('',(1.,0.,0.));
#66940=DIRECTION('center_axis',(-1.,0.,0.));
#66941=DIRECTION('ref_axis',(0.,1.,0.));
#66942=DIRECTION('',(0.,1.,0.));
#66943=DIRECTION('',(0.,1.,0.));
#66944=DIRECTION('center_axis',(0.,0.,-1.));
#66945=DIRECTION('ref_axis',(-1.,0.,0.));
#66946=DIRECTION('center_axis',(0.,-1.,0.));
#66947=DIRECTION('ref_axis',(-1.,0.,0.));
#66948=DIRECTION('',(-1.,0.,0.));
#66949=DIRECTION('',(0.,0.,-1.));
#66950=DIRECTION('',(-1.,0.,0.));
#66951=DIRECTION('',(0.,0.,-1.));
#66952=DIRECTION('center_axis',(1.,0.,0.));
#66953=DIRECTION('ref_axis',(0.,-1.,0.));
#66954=DIRECTION('',(0.,-1.,0.));
#66955=DIRECTION('',(0.,0.,-1.));
#66956=DIRECTION('',(0.,-1.,0.));
#66957=DIRECTION('center_axis',(0.,1.,0.));
#66958=DIRECTION('ref_axis',(1.,0.,0.));
#66959=DIRECTION('',(1.,0.,0.));
#66960=DIRECTION('',(0.,0.,-1.));
#66961=DIRECTION('',(1.,0.,0.));
#66962=DIRECTION('center_axis',(-1.,0.,0.));
#66963=DIRECTION('ref_axis',(0.,1.,0.));
#66964=DIRECTION('',(0.,1.,0.));
#66965=DIRECTION('',(0.,1.,0.));
#66966=DIRECTION('center_axis',(0.,0.,-1.));
#66967=DIRECTION('ref_axis',(-1.,0.,0.));
#66968=DIRECTION('center_axis',(0.,-1.,0.));
#66969=DIRECTION('ref_axis',(-1.,0.,0.));
#66970=DIRECTION('',(-1.,0.,0.));
#66971=DIRECTION('',(0.,0.,-1.));
#66972=DIRECTION('',(-1.,0.,0.));
#66973=DIRECTION('',(0.,0.,-1.));
#66974=DIRECTION('center_axis',(1.,0.,0.));
#66975=DIRECTION('ref_axis',(0.,-1.,0.));
#66976=DIRECTION('',(0.,-1.,0.));
#66977=DIRECTION('',(0.,0.,-1.));
#66978=DIRECTION('',(0.,-1.,0.));
#66979=DIRECTION('center_axis',(0.,1.,0.));
#66980=DIRECTION('ref_axis',(1.,0.,0.));
#66981=DIRECTION('',(1.,0.,0.));
#66982=DIRECTION('',(0.,0.,-1.));
#66983=DIRECTION('',(1.,0.,0.));
#66984=DIRECTION('center_axis',(-1.,0.,0.));
#66985=DIRECTION('ref_axis',(0.,1.,0.));
#66986=DIRECTION('',(0.,1.,0.));
#66987=DIRECTION('',(0.,1.,0.));
#66988=DIRECTION('center_axis',(0.,0.,-1.));
#66989=DIRECTION('ref_axis',(-1.,0.,0.));
#66990=DIRECTION('center_axis',(0.,-1.,0.));
#66991=DIRECTION('ref_axis',(-1.,0.,0.));
#66992=DIRECTION('',(-1.,0.,0.));
#66993=DIRECTION('',(0.,0.,-1.));
#66994=DIRECTION('',(-1.,0.,0.));
#66995=DIRECTION('',(0.,0.,-1.));
#66996=DIRECTION('center_axis',(1.,0.,0.));
#66997=DIRECTION('ref_axis',(0.,-1.,0.));
#66998=DIRECTION('',(0.,-1.,0.));
#66999=DIRECTION('',(0.,0.,-1.));
#67000=DIRECTION('',(0.,-1.,0.));
#67001=DIRECTION('center_axis',(0.,1.,0.));
#67002=DIRECTION('ref_axis',(1.,0.,0.));
#67003=DIRECTION('',(1.,0.,0.));
#67004=DIRECTION('',(0.,0.,-1.));
#67005=DIRECTION('',(1.,0.,0.));
#67006=DIRECTION('center_axis',(-1.,0.,0.));
#67007=DIRECTION('ref_axis',(0.,1.,0.));
#67008=DIRECTION('',(0.,1.,0.));
#67009=DIRECTION('',(0.,1.,0.));
#67010=DIRECTION('center_axis',(0.,0.,-1.));
#67011=DIRECTION('ref_axis',(-1.,0.,0.));
#67012=DIRECTION('center_axis',(0.,-1.,0.));
#67013=DIRECTION('ref_axis',(-1.,0.,0.));
#67014=DIRECTION('',(-1.,0.,0.));
#67015=DIRECTION('',(0.,0.,-1.));
#67016=DIRECTION('',(-1.,0.,0.));
#67017=DIRECTION('',(0.,0.,-1.));
#67018=DIRECTION('center_axis',(1.,0.,0.));
#67019=DIRECTION('ref_axis',(0.,-1.,0.));
#67020=DIRECTION('',(0.,-1.,0.));
#67021=DIRECTION('',(0.,0.,-1.));
#67022=DIRECTION('',(0.,-1.,0.));
#67023=DIRECTION('center_axis',(0.,1.,0.));
#67024=DIRECTION('ref_axis',(1.,0.,0.));
#67025=DIRECTION('',(1.,0.,0.));
#67026=DIRECTION('',(0.,0.,-1.));
#67027=DIRECTION('',(1.,0.,0.));
#67028=DIRECTION('center_axis',(-1.,0.,0.));
#67029=DIRECTION('ref_axis',(0.,1.,0.));
#67030=DIRECTION('',(0.,1.,0.));
#67031=DIRECTION('',(0.,1.,0.));
#67032=DIRECTION('center_axis',(0.,0.,-1.));
#67033=DIRECTION('ref_axis',(-1.,0.,0.));
#67034=DIRECTION('center_axis',(0.,-1.,0.));
#67035=DIRECTION('ref_axis',(-1.,0.,0.));
#67036=DIRECTION('',(-1.,0.,0.));
#67037=DIRECTION('',(0.,0.,-1.));
#67038=DIRECTION('',(-1.,0.,0.));
#67039=DIRECTION('',(0.,0.,-1.));
#67040=DIRECTION('center_axis',(1.,0.,0.));
#67041=DIRECTION('ref_axis',(0.,-1.,0.));
#67042=DIRECTION('',(0.,-1.,0.));
#67043=DIRECTION('',(0.,0.,-1.));
#67044=DIRECTION('',(0.,-1.,0.));
#67045=DIRECTION('center_axis',(0.,1.,0.));
#67046=DIRECTION('ref_axis',(1.,0.,0.));
#67047=DIRECTION('',(1.,0.,0.));
#67048=DIRECTION('',(0.,0.,-1.));
#67049=DIRECTION('',(1.,0.,0.));
#67050=DIRECTION('center_axis',(-1.,0.,0.));
#67051=DIRECTION('ref_axis',(0.,1.,0.));
#67052=DIRECTION('',(0.,1.,0.));
#67053=DIRECTION('',(0.,1.,0.));
#67054=DIRECTION('center_axis',(0.,0.,-1.));
#67055=DIRECTION('ref_axis',(-1.,0.,0.));
#67056=DIRECTION('center_axis',(0.,-1.,0.));
#67057=DIRECTION('ref_axis',(-1.,0.,0.));
#67058=DIRECTION('',(-1.,0.,0.));
#67059=DIRECTION('',(0.,0.,-1.));
#67060=DIRECTION('',(-1.,0.,0.));
#67061=DIRECTION('',(0.,0.,-1.));
#67062=DIRECTION('center_axis',(1.,0.,0.));
#67063=DIRECTION('ref_axis',(0.,-1.,0.));
#67064=DIRECTION('',(0.,-1.,0.));
#67065=DIRECTION('',(0.,0.,-1.));
#67066=DIRECTION('',(0.,-1.,0.));
#67067=DIRECTION('center_axis',(0.,1.,0.));
#67068=DIRECTION('ref_axis',(1.,0.,0.));
#67069=DIRECTION('',(1.,0.,0.));
#67070=DIRECTION('',(0.,0.,-1.));
#67071=DIRECTION('',(1.,0.,0.));
#67072=DIRECTION('center_axis',(-1.,0.,0.));
#67073=DIRECTION('ref_axis',(0.,1.,0.));
#67074=DIRECTION('',(0.,1.,0.));
#67075=DIRECTION('',(0.,1.,0.));
#67076=DIRECTION('center_axis',(0.,0.,-1.));
#67077=DIRECTION('ref_axis',(-1.,0.,0.));
#67078=DIRECTION('center_axis',(0.,-1.,0.));
#67079=DIRECTION('ref_axis',(-1.,0.,0.));
#67080=DIRECTION('',(-1.,0.,0.));
#67081=DIRECTION('',(0.,0.,-1.));
#67082=DIRECTION('',(-1.,0.,0.));
#67083=DIRECTION('',(0.,0.,-1.));
#67084=DIRECTION('center_axis',(1.,0.,0.));
#67085=DIRECTION('ref_axis',(0.,-1.,0.));
#67086=DIRECTION('',(0.,-1.,0.));
#67087=DIRECTION('',(0.,0.,-1.));
#67088=DIRECTION('',(0.,-1.,0.));
#67089=DIRECTION('center_axis',(0.,1.,0.));
#67090=DIRECTION('ref_axis',(1.,0.,0.));
#67091=DIRECTION('',(1.,0.,0.));
#67092=DIRECTION('',(0.,0.,-1.));
#67093=DIRECTION('',(1.,0.,0.));
#67094=DIRECTION('center_axis',(-1.,0.,0.));
#67095=DIRECTION('ref_axis',(0.,1.,0.));
#67096=DIRECTION('',(0.,1.,0.));
#67097=DIRECTION('',(0.,1.,0.));
#67098=DIRECTION('center_axis',(0.,0.,-1.));
#67099=DIRECTION('ref_axis',(-1.,0.,0.));
#67100=DIRECTION('center_axis',(0.,-1.,0.));
#67101=DIRECTION('ref_axis',(-1.,0.,0.));
#67102=DIRECTION('',(-1.,0.,0.));
#67103=DIRECTION('',(0.,0.,-1.));
#67104=DIRECTION('',(-1.,0.,0.));
#67105=DIRECTION('',(0.,0.,-1.));
#67106=DIRECTION('center_axis',(1.,0.,0.));
#67107=DIRECTION('ref_axis',(0.,-1.,0.));
#67108=DIRECTION('',(0.,-1.,0.));
#67109=DIRECTION('',(0.,0.,-1.));
#67110=DIRECTION('',(0.,-1.,0.));
#67111=DIRECTION('center_axis',(0.,1.,0.));
#67112=DIRECTION('ref_axis',(1.,0.,0.));
#67113=DIRECTION('',(1.,0.,0.));
#67114=DIRECTION('',(0.,0.,-1.));
#67115=DIRECTION('',(1.,0.,0.));
#67116=DIRECTION('center_axis',(-1.,0.,0.));
#67117=DIRECTION('ref_axis',(0.,1.,0.));
#67118=DIRECTION('',(0.,1.,0.));
#67119=DIRECTION('',(0.,1.,0.));
#67120=DIRECTION('center_axis',(0.,0.,-1.));
#67121=DIRECTION('ref_axis',(-1.,0.,0.));
#67122=DIRECTION('center_axis',(0.,-1.,0.));
#67123=DIRECTION('ref_axis',(-1.,0.,0.));
#67124=DIRECTION('',(-1.,0.,0.));
#67125=DIRECTION('',(0.,0.,-1.));
#67126=DIRECTION('',(-1.,0.,0.));
#67127=DIRECTION('',(0.,0.,-1.));
#67128=DIRECTION('center_axis',(1.,0.,0.));
#67129=DIRECTION('ref_axis',(0.,-1.,0.));
#67130=DIRECTION('',(0.,-1.,0.));
#67131=DIRECTION('',(0.,0.,-1.));
#67132=DIRECTION('',(0.,-1.,0.));
#67133=DIRECTION('center_axis',(0.,1.,0.));
#67134=DIRECTION('ref_axis',(1.,0.,0.));
#67135=DIRECTION('',(1.,0.,0.));
#67136=DIRECTION('',(0.,0.,-1.));
#67137=DIRECTION('',(1.,0.,0.));
#67138=DIRECTION('center_axis',(-1.,0.,0.));
#67139=DIRECTION('ref_axis',(0.,1.,0.));
#67140=DIRECTION('',(0.,1.,0.));
#67141=DIRECTION('',(0.,1.,0.));
#67142=DIRECTION('center_axis',(0.,0.,-1.));
#67143=DIRECTION('ref_axis',(-1.,0.,0.));
#67144=DIRECTION('center_axis',(0.,-1.,0.));
#67145=DIRECTION('ref_axis',(-1.,0.,0.));
#67146=DIRECTION('',(-1.,0.,0.));
#67147=DIRECTION('',(0.,0.,-1.));
#67148=DIRECTION('',(-1.,0.,0.));
#67149=DIRECTION('',(0.,0.,-1.));
#67150=DIRECTION('center_axis',(1.,0.,0.));
#67151=DIRECTION('ref_axis',(0.,-1.,0.));
#67152=DIRECTION('',(0.,-1.,0.));
#67153=DIRECTION('',(0.,0.,-1.));
#67154=DIRECTION('',(0.,-1.,0.));
#67155=DIRECTION('center_axis',(0.,1.,0.));
#67156=DIRECTION('ref_axis',(1.,0.,0.));
#67157=DIRECTION('',(1.,0.,0.));
#67158=DIRECTION('',(0.,0.,-1.));
#67159=DIRECTION('',(1.,0.,0.));
#67160=DIRECTION('center_axis',(-1.,0.,0.));
#67161=DIRECTION('ref_axis',(0.,1.,0.));
#67162=DIRECTION('',(0.,1.,0.));
#67163=DIRECTION('',(0.,1.,0.));
#67164=DIRECTION('center_axis',(0.,0.,-1.));
#67165=DIRECTION('ref_axis',(-1.,0.,0.));
#67166=DIRECTION('center_axis',(0.,-1.,0.));
#67167=DIRECTION('ref_axis',(-1.,0.,0.));
#67168=DIRECTION('',(-1.,0.,0.));
#67169=DIRECTION('',(0.,0.,-1.));
#67170=DIRECTION('',(-1.,0.,0.));
#67171=DIRECTION('',(0.,0.,-1.));
#67172=DIRECTION('center_axis',(1.,0.,0.));
#67173=DIRECTION('ref_axis',(0.,-1.,0.));
#67174=DIRECTION('',(0.,-1.,0.));
#67175=DIRECTION('',(0.,0.,-1.));
#67176=DIRECTION('',(0.,-1.,0.));
#67177=DIRECTION('center_axis',(0.,1.,0.));
#67178=DIRECTION('ref_axis',(1.,0.,0.));
#67179=DIRECTION('',(1.,0.,0.));
#67180=DIRECTION('',(0.,0.,-1.));
#67181=DIRECTION('',(1.,0.,0.));
#67182=DIRECTION('center_axis',(-1.,0.,0.));
#67183=DIRECTION('ref_axis',(0.,1.,0.));
#67184=DIRECTION('',(0.,1.,0.));
#67185=DIRECTION('',(0.,1.,0.));
#67186=DIRECTION('center_axis',(0.,0.,-1.));
#67187=DIRECTION('ref_axis',(-1.,0.,0.));
#67188=DIRECTION('center_axis',(0.,-1.,0.));
#67189=DIRECTION('ref_axis',(-1.,0.,0.));
#67190=DIRECTION('',(-1.,0.,0.));
#67191=DIRECTION('',(0.,0.,-1.));
#67192=DIRECTION('',(-1.,0.,0.));
#67193=DIRECTION('',(0.,0.,-1.));
#67194=DIRECTION('center_axis',(1.,0.,0.));
#67195=DIRECTION('ref_axis',(0.,-1.,0.));
#67196=DIRECTION('',(0.,-1.,0.));
#67197=DIRECTION('',(0.,0.,-1.));
#67198=DIRECTION('',(0.,-1.,0.));
#67199=DIRECTION('center_axis',(0.,1.,0.));
#67200=DIRECTION('ref_axis',(1.,0.,0.));
#67201=DIRECTION('',(1.,0.,0.));
#67202=DIRECTION('',(0.,0.,-1.));
#67203=DIRECTION('',(1.,0.,0.));
#67204=DIRECTION('center_axis',(-1.,0.,0.));
#67205=DIRECTION('ref_axis',(0.,1.,0.));
#67206=DIRECTION('',(0.,1.,0.));
#67207=DIRECTION('',(0.,1.,0.));
#67208=DIRECTION('center_axis',(0.,0.,-1.));
#67209=DIRECTION('ref_axis',(-1.,0.,0.));
#67210=DIRECTION('center_axis',(0.,-1.,0.));
#67211=DIRECTION('ref_axis',(-1.,0.,0.));
#67212=DIRECTION('',(-1.,0.,0.));
#67213=DIRECTION('',(0.,0.,-1.));
#67214=DIRECTION('',(-1.,0.,0.));
#67215=DIRECTION('',(0.,0.,-1.));
#67216=DIRECTION('center_axis',(1.,0.,0.));
#67217=DIRECTION('ref_axis',(0.,-1.,0.));
#67218=DIRECTION('',(0.,-1.,0.));
#67219=DIRECTION('',(0.,0.,-1.));
#67220=DIRECTION('',(0.,-1.,0.));
#67221=DIRECTION('center_axis',(0.,1.,0.));
#67222=DIRECTION('ref_axis',(1.,0.,0.));
#67223=DIRECTION('',(1.,0.,0.));
#67224=DIRECTION('',(0.,0.,-1.));
#67225=DIRECTION('',(1.,0.,0.));
#67226=DIRECTION('center_axis',(-1.,0.,0.));
#67227=DIRECTION('ref_axis',(0.,1.,0.));
#67228=DIRECTION('',(0.,1.,0.));
#67229=DIRECTION('',(0.,1.,0.));
#67230=DIRECTION('center_axis',(0.,0.,-1.));
#67231=DIRECTION('ref_axis',(-1.,0.,0.));
#67232=DIRECTION('center_axis',(0.,-1.,0.));
#67233=DIRECTION('ref_axis',(-1.,0.,0.));
#67234=DIRECTION('',(-1.,0.,0.));
#67235=DIRECTION('',(0.,0.,-1.));
#67236=DIRECTION('',(-1.,0.,0.));
#67237=DIRECTION('',(0.,0.,-1.));
#67238=DIRECTION('center_axis',(1.,0.,0.));
#67239=DIRECTION('ref_axis',(0.,-1.,0.));
#67240=DIRECTION('',(0.,-1.,0.));
#67241=DIRECTION('',(0.,0.,-1.));
#67242=DIRECTION('',(0.,-1.,0.));
#67243=DIRECTION('center_axis',(0.,1.,0.));
#67244=DIRECTION('ref_axis',(1.,0.,0.));
#67245=DIRECTION('',(1.,0.,0.));
#67246=DIRECTION('',(0.,0.,-1.));
#67247=DIRECTION('',(1.,0.,0.));
#67248=DIRECTION('center_axis',(-1.,0.,0.));
#67249=DIRECTION('ref_axis',(0.,1.,0.));
#67250=DIRECTION('',(0.,1.,0.));
#67251=DIRECTION('',(0.,1.,0.));
#67252=DIRECTION('center_axis',(0.,0.,-1.));
#67253=DIRECTION('ref_axis',(-1.,0.,0.));
#67254=DIRECTION('center_axis',(0.,-1.,0.));
#67255=DIRECTION('ref_axis',(-1.,0.,0.));
#67256=DIRECTION('',(-1.,0.,0.));
#67257=DIRECTION('',(0.,0.,-1.));
#67258=DIRECTION('',(-1.,0.,0.));
#67259=DIRECTION('',(0.,0.,-1.));
#67260=DIRECTION('center_axis',(1.,0.,0.));
#67261=DIRECTION('ref_axis',(0.,-1.,0.));
#67262=DIRECTION('',(0.,-1.,0.));
#67263=DIRECTION('',(0.,0.,-1.));
#67264=DIRECTION('',(0.,-1.,0.));
#67265=DIRECTION('center_axis',(0.,1.,0.));
#67266=DIRECTION('ref_axis',(1.,0.,0.));
#67267=DIRECTION('',(1.,0.,0.));
#67268=DIRECTION('',(0.,0.,-1.));
#67269=DIRECTION('',(1.,0.,0.));
#67270=DIRECTION('center_axis',(-1.,0.,0.));
#67271=DIRECTION('ref_axis',(0.,1.,0.));
#67272=DIRECTION('',(0.,1.,0.));
#67273=DIRECTION('',(0.,1.,0.));
#67274=DIRECTION('center_axis',(0.,0.,-1.));
#67275=DIRECTION('ref_axis',(-1.,0.,0.));
#67276=DIRECTION('center_axis',(0.,-1.,0.));
#67277=DIRECTION('ref_axis',(-1.,0.,0.));
#67278=DIRECTION('',(-1.,0.,0.));
#67279=DIRECTION('',(0.,0.,-1.));
#67280=DIRECTION('',(-1.,0.,0.));
#67281=DIRECTION('',(0.,0.,-1.));
#67282=DIRECTION('center_axis',(1.,0.,0.));
#67283=DIRECTION('ref_axis',(0.,-1.,0.));
#67284=DIRECTION('',(0.,-1.,0.));
#67285=DIRECTION('',(0.,0.,-1.));
#67286=DIRECTION('',(0.,-1.,0.));
#67287=DIRECTION('center_axis',(0.,1.,0.));
#67288=DIRECTION('ref_axis',(1.,0.,0.));
#67289=DIRECTION('',(1.,0.,0.));
#67290=DIRECTION('',(0.,0.,-1.));
#67291=DIRECTION('',(1.,0.,0.));
#67292=DIRECTION('center_axis',(-1.,0.,0.));
#67293=DIRECTION('ref_axis',(0.,1.,0.));
#67294=DIRECTION('',(0.,1.,0.));
#67295=DIRECTION('',(0.,1.,0.));
#67296=DIRECTION('center_axis',(0.,0.,-1.));
#67297=DIRECTION('ref_axis',(-1.,0.,0.));
#67298=DIRECTION('center_axis',(0.,-1.,0.));
#67299=DIRECTION('ref_axis',(-1.,0.,0.));
#67300=DIRECTION('',(-1.,0.,0.));
#67301=DIRECTION('',(0.,0.,-1.));
#67302=DIRECTION('',(-1.,0.,0.));
#67303=DIRECTION('',(0.,0.,-1.));
#67304=DIRECTION('center_axis',(1.,0.,0.));
#67305=DIRECTION('ref_axis',(0.,-1.,0.));
#67306=DIRECTION('',(0.,-1.,0.));
#67307=DIRECTION('',(0.,0.,-1.));
#67308=DIRECTION('',(0.,-1.,0.));
#67309=DIRECTION('center_axis',(0.,1.,0.));
#67310=DIRECTION('ref_axis',(1.,0.,0.));
#67311=DIRECTION('',(1.,0.,0.));
#67312=DIRECTION('',(0.,0.,-1.));
#67313=DIRECTION('',(1.,0.,0.));
#67314=DIRECTION('center_axis',(-1.,0.,0.));
#67315=DIRECTION('ref_axis',(0.,1.,0.));
#67316=DIRECTION('',(0.,1.,0.));
#67317=DIRECTION('',(0.,1.,0.));
#67318=DIRECTION('center_axis',(0.,0.,-1.));
#67319=DIRECTION('ref_axis',(-1.,0.,0.));
#67320=DIRECTION('center_axis',(0.,-1.,0.));
#67321=DIRECTION('ref_axis',(-1.,0.,0.));
#67322=DIRECTION('',(-1.,0.,0.));
#67323=DIRECTION('',(0.,0.,-1.));
#67324=DIRECTION('',(-1.,0.,0.));
#67325=DIRECTION('',(0.,0.,-1.));
#67326=DIRECTION('center_axis',(1.,0.,0.));
#67327=DIRECTION('ref_axis',(0.,-1.,0.));
#67328=DIRECTION('',(0.,-1.,0.));
#67329=DIRECTION('',(0.,0.,-1.));
#67330=DIRECTION('',(0.,-1.,0.));
#67331=DIRECTION('center_axis',(0.,1.,0.));
#67332=DIRECTION('ref_axis',(1.,0.,0.));
#67333=DIRECTION('',(1.,0.,0.));
#67334=DIRECTION('',(0.,0.,-1.));
#67335=DIRECTION('',(1.,0.,0.));
#67336=DIRECTION('center_axis',(-1.,0.,0.));
#67337=DIRECTION('ref_axis',(0.,1.,0.));
#67338=DIRECTION('',(0.,1.,0.));
#67339=DIRECTION('',(0.,1.,0.));
#67340=DIRECTION('center_axis',(0.,0.,-1.));
#67341=DIRECTION('ref_axis',(-1.,0.,0.));
#67342=DIRECTION('center_axis',(0.,-1.,0.));
#67343=DIRECTION('ref_axis',(-1.,0.,0.));
#67344=DIRECTION('',(-1.,0.,0.));
#67345=DIRECTION('',(0.,0.,-1.));
#67346=DIRECTION('',(-1.,0.,0.));
#67347=DIRECTION('',(0.,0.,-1.));
#67348=DIRECTION('center_axis',(1.,0.,0.));
#67349=DIRECTION('ref_axis',(0.,-1.,0.));
#67350=DIRECTION('',(0.,-1.,0.));
#67351=DIRECTION('',(0.,0.,-1.));
#67352=DIRECTION('',(0.,-1.,0.));
#67353=DIRECTION('center_axis',(0.,1.,0.));
#67354=DIRECTION('ref_axis',(1.,0.,0.));
#67355=DIRECTION('',(1.,0.,0.));
#67356=DIRECTION('',(0.,0.,-1.));
#67357=DIRECTION('',(1.,0.,0.));
#67358=DIRECTION('center_axis',(-1.,0.,0.));
#67359=DIRECTION('ref_axis',(0.,1.,0.));
#67360=DIRECTION('',(0.,1.,0.));
#67361=DIRECTION('',(0.,1.,0.));
#67362=DIRECTION('center_axis',(0.,0.,-1.));
#67363=DIRECTION('ref_axis',(-1.,0.,0.));
#67364=DIRECTION('center_axis',(0.,-1.,0.));
#67365=DIRECTION('ref_axis',(-1.,0.,0.));
#67366=DIRECTION('',(-1.,0.,0.));
#67367=DIRECTION('',(0.,0.,-1.));
#67368=DIRECTION('',(-1.,0.,0.));
#67369=DIRECTION('',(0.,0.,-1.));
#67370=DIRECTION('center_axis',(1.,0.,0.));
#67371=DIRECTION('ref_axis',(0.,-1.,0.));
#67372=DIRECTION('',(0.,-1.,0.));
#67373=DIRECTION('',(0.,0.,-1.));
#67374=DIRECTION('',(0.,-1.,0.));
#67375=DIRECTION('center_axis',(0.,1.,0.));
#67376=DIRECTION('ref_axis',(1.,0.,0.));
#67377=DIRECTION('',(1.,0.,0.));
#67378=DIRECTION('',(0.,0.,-1.));
#67379=DIRECTION('',(1.,0.,0.));
#67380=DIRECTION('center_axis',(-1.,0.,0.));
#67381=DIRECTION('ref_axis',(0.,1.,0.));
#67382=DIRECTION('',(0.,1.,0.));
#67383=DIRECTION('',(0.,1.,0.));
#67384=DIRECTION('center_axis',(0.,0.,-1.));
#67385=DIRECTION('ref_axis',(-1.,0.,0.));
#67386=DIRECTION('center_axis',(0.,-1.,0.));
#67387=DIRECTION('ref_axis',(-1.,0.,0.));
#67388=DIRECTION('',(-1.,0.,0.));
#67389=DIRECTION('',(0.,0.,-1.));
#67390=DIRECTION('',(-1.,0.,0.));
#67391=DIRECTION('',(0.,0.,-1.));
#67392=DIRECTION('center_axis',(1.,0.,0.));
#67393=DIRECTION('ref_axis',(0.,-1.,0.));
#67394=DIRECTION('',(0.,-1.,0.));
#67395=DIRECTION('',(0.,0.,-1.));
#67396=DIRECTION('',(0.,-1.,0.));
#67397=DIRECTION('center_axis',(0.,1.,0.));
#67398=DIRECTION('ref_axis',(1.,0.,0.));
#67399=DIRECTION('',(1.,0.,0.));
#67400=DIRECTION('',(0.,0.,-1.));
#67401=DIRECTION('',(1.,0.,0.));
#67402=DIRECTION('center_axis',(-1.,0.,0.));
#67403=DIRECTION('ref_axis',(0.,1.,0.));
#67404=DIRECTION('',(0.,1.,0.));
#67405=DIRECTION('',(0.,1.,0.));
#67406=DIRECTION('center_axis',(0.,0.,-1.));
#67407=DIRECTION('ref_axis',(-1.,0.,0.));
#67408=DIRECTION('center_axis',(0.,-1.,0.));
#67409=DIRECTION('ref_axis',(-1.,0.,0.));
#67410=DIRECTION('',(-1.,0.,0.));
#67411=DIRECTION('',(0.,0.,-1.));
#67412=DIRECTION('',(-1.,0.,0.));
#67413=DIRECTION('',(0.,0.,-1.));
#67414=DIRECTION('center_axis',(1.,0.,0.));
#67415=DIRECTION('ref_axis',(0.,-1.,0.));
#67416=DIRECTION('',(0.,-1.,0.));
#67417=DIRECTION('',(0.,0.,-1.));
#67418=DIRECTION('',(0.,-1.,0.));
#67419=DIRECTION('center_axis',(0.,1.,0.));
#67420=DIRECTION('ref_axis',(1.,0.,0.));
#67421=DIRECTION('',(1.,0.,0.));
#67422=DIRECTION('',(0.,0.,-1.));
#67423=DIRECTION('',(1.,0.,0.));
#67424=DIRECTION('center_axis',(-1.,0.,0.));
#67425=DIRECTION('ref_axis',(0.,1.,0.));
#67426=DIRECTION('',(0.,1.,0.));
#67427=DIRECTION('',(0.,1.,0.));
#67428=DIRECTION('center_axis',(0.,0.,-1.));
#67429=DIRECTION('ref_axis',(-1.,0.,0.));
#67430=DIRECTION('center_axis',(0.,-1.,0.));
#67431=DIRECTION('ref_axis',(-1.,0.,0.));
#67432=DIRECTION('',(-1.,0.,0.));
#67433=DIRECTION('',(0.,0.,-1.));
#67434=DIRECTION('',(-1.,0.,0.));
#67435=DIRECTION('',(0.,0.,-1.));
#67436=DIRECTION('center_axis',(1.,0.,0.));
#67437=DIRECTION('ref_axis',(0.,-1.,0.));
#67438=DIRECTION('',(0.,-1.,0.));
#67439=DIRECTION('',(0.,0.,-1.));
#67440=DIRECTION('',(0.,-1.,0.));
#67441=DIRECTION('center_axis',(0.,1.,0.));
#67442=DIRECTION('ref_axis',(1.,0.,0.));
#67443=DIRECTION('',(1.,0.,0.));
#67444=DIRECTION('',(0.,0.,-1.));
#67445=DIRECTION('',(1.,0.,0.));
#67446=DIRECTION('center_axis',(-1.,0.,0.));
#67447=DIRECTION('ref_axis',(0.,1.,0.));
#67448=DIRECTION('',(0.,1.,0.));
#67449=DIRECTION('',(0.,1.,0.));
#67450=DIRECTION('center_axis',(0.,0.,-1.));
#67451=DIRECTION('ref_axis',(-1.,0.,0.));
#67452=DIRECTION('center_axis',(0.,-1.,0.));
#67453=DIRECTION('ref_axis',(-1.,0.,0.));
#67454=DIRECTION('',(-1.,0.,0.));
#67455=DIRECTION('',(0.,0.,-1.));
#67456=DIRECTION('',(-1.,0.,0.));
#67457=DIRECTION('',(0.,0.,-1.));
#67458=DIRECTION('center_axis',(1.,0.,0.));
#67459=DIRECTION('ref_axis',(0.,-1.,0.));
#67460=DIRECTION('',(0.,-1.,0.));
#67461=DIRECTION('',(0.,0.,-1.));
#67462=DIRECTION('',(0.,-1.,0.));
#67463=DIRECTION('center_axis',(0.,1.,0.));
#67464=DIRECTION('ref_axis',(1.,0.,0.));
#67465=DIRECTION('',(1.,0.,0.));
#67466=DIRECTION('',(0.,0.,-1.));
#67467=DIRECTION('',(1.,0.,0.));
#67468=DIRECTION('center_axis',(-1.,0.,0.));
#67469=DIRECTION('ref_axis',(0.,1.,0.));
#67470=DIRECTION('',(0.,1.,0.));
#67471=DIRECTION('',(0.,1.,0.));
#67472=DIRECTION('center_axis',(0.,0.,-1.));
#67473=DIRECTION('ref_axis',(-1.,0.,0.));
#67474=DIRECTION('center_axis',(0.,-1.,0.));
#67475=DIRECTION('ref_axis',(-1.,0.,0.));
#67476=DIRECTION('',(-1.,0.,0.));
#67477=DIRECTION('',(0.,0.,-1.));
#67478=DIRECTION('',(-1.,0.,0.));
#67479=DIRECTION('',(0.,0.,-1.));
#67480=DIRECTION('center_axis',(1.,0.,0.));
#67481=DIRECTION('ref_axis',(0.,-1.,0.));
#67482=DIRECTION('',(0.,-1.,0.));
#67483=DIRECTION('',(0.,0.,-1.));
#67484=DIRECTION('',(0.,-1.,0.));
#67485=DIRECTION('center_axis',(0.,1.,0.));
#67486=DIRECTION('ref_axis',(1.,0.,0.));
#67487=DIRECTION('',(1.,0.,0.));
#67488=DIRECTION('',(0.,0.,-1.));
#67489=DIRECTION('',(1.,0.,0.));
#67490=DIRECTION('center_axis',(-1.,0.,0.));
#67491=DIRECTION('ref_axis',(0.,1.,0.));
#67492=DIRECTION('',(0.,1.,0.));
#67493=DIRECTION('',(0.,1.,0.));
#67494=DIRECTION('center_axis',(0.,0.,-1.));
#67495=DIRECTION('ref_axis',(-1.,0.,0.));
#67496=DIRECTION('center_axis',(0.,-1.,0.));
#67497=DIRECTION('ref_axis',(-1.,0.,0.));
#67498=DIRECTION('',(-1.,0.,0.));
#67499=DIRECTION('',(0.,0.,-1.));
#67500=DIRECTION('',(-1.,0.,0.));
#67501=DIRECTION('',(0.,0.,-1.));
#67502=DIRECTION('center_axis',(1.,0.,0.));
#67503=DIRECTION('ref_axis',(0.,-1.,0.));
#67504=DIRECTION('',(0.,-1.,0.));
#67505=DIRECTION('',(0.,0.,-1.));
#67506=DIRECTION('',(0.,-1.,0.));
#67507=DIRECTION('center_axis',(0.,1.,0.));
#67508=DIRECTION('ref_axis',(1.,0.,0.));
#67509=DIRECTION('',(1.,0.,0.));
#67510=DIRECTION('',(0.,0.,-1.));
#67511=DIRECTION('',(1.,0.,0.));
#67512=DIRECTION('center_axis',(-1.,0.,0.));
#67513=DIRECTION('ref_axis',(0.,1.,0.));
#67514=DIRECTION('',(0.,1.,0.));
#67515=DIRECTION('',(0.,1.,0.));
#67516=DIRECTION('center_axis',(0.,0.,-1.));
#67517=DIRECTION('ref_axis',(-1.,0.,0.));
#67518=DIRECTION('center_axis',(0.,-1.,0.));
#67519=DIRECTION('ref_axis',(-1.,0.,0.));
#67520=DIRECTION('',(-1.,0.,0.));
#67521=DIRECTION('',(0.,0.,-1.));
#67522=DIRECTION('',(-1.,0.,0.));
#67523=DIRECTION('',(0.,0.,-1.));
#67524=DIRECTION('center_axis',(1.,0.,0.));
#67525=DIRECTION('ref_axis',(0.,-1.,0.));
#67526=DIRECTION('',(0.,-1.,0.));
#67527=DIRECTION('',(0.,0.,-1.));
#67528=DIRECTION('',(0.,-1.,0.));
#67529=DIRECTION('center_axis',(0.,1.,0.));
#67530=DIRECTION('ref_axis',(1.,0.,0.));
#67531=DIRECTION('',(1.,0.,0.));
#67532=DIRECTION('',(0.,0.,-1.));
#67533=DIRECTION('',(1.,0.,0.));
#67534=DIRECTION('center_axis',(-1.,0.,0.));
#67535=DIRECTION('ref_axis',(0.,1.,0.));
#67536=DIRECTION('',(0.,1.,0.));
#67537=DIRECTION('',(0.,1.,0.));
#67538=DIRECTION('center_axis',(0.,0.,-1.));
#67539=DIRECTION('ref_axis',(-1.,0.,0.));
#67540=DIRECTION('center_axis',(0.,-1.,0.));
#67541=DIRECTION('ref_axis',(-1.,0.,0.));
#67542=DIRECTION('',(-1.,0.,0.));
#67543=DIRECTION('',(0.,0.,-1.));
#67544=DIRECTION('',(-1.,0.,0.));
#67545=DIRECTION('',(0.,0.,-1.));
#67546=DIRECTION('center_axis',(1.,0.,0.));
#67547=DIRECTION('ref_axis',(0.,-1.,0.));
#67548=DIRECTION('',(0.,-1.,0.));
#67549=DIRECTION('',(0.,0.,-1.));
#67550=DIRECTION('',(0.,-1.,0.));
#67551=DIRECTION('center_axis',(0.,1.,0.));
#67552=DIRECTION('ref_axis',(1.,0.,0.));
#67553=DIRECTION('',(1.,0.,0.));
#67554=DIRECTION('',(0.,0.,-1.));
#67555=DIRECTION('',(1.,0.,0.));
#67556=DIRECTION('center_axis',(-1.,0.,0.));
#67557=DIRECTION('ref_axis',(0.,1.,0.));
#67558=DIRECTION('',(0.,1.,0.));
#67559=DIRECTION('',(0.,1.,0.));
#67560=DIRECTION('center_axis',(0.,0.,-1.));
#67561=DIRECTION('ref_axis',(-1.,0.,0.));
#67562=DIRECTION('center_axis',(0.,-1.,0.));
#67563=DIRECTION('ref_axis',(-1.,0.,0.));
#67564=DIRECTION('',(-1.,0.,0.));
#67565=DIRECTION('',(0.,0.,-1.));
#67566=DIRECTION('',(-1.,0.,0.));
#67567=DIRECTION('',(0.,0.,-1.));
#67568=DIRECTION('center_axis',(1.,0.,0.));
#67569=DIRECTION('ref_axis',(0.,-1.,0.));
#67570=DIRECTION('',(0.,-1.,0.));
#67571=DIRECTION('',(0.,0.,-1.));
#67572=DIRECTION('',(0.,-1.,0.));
#67573=DIRECTION('center_axis',(0.,1.,0.));
#67574=DIRECTION('ref_axis',(1.,0.,0.));
#67575=DIRECTION('',(1.,0.,0.));
#67576=DIRECTION('',(0.,0.,-1.));
#67577=DIRECTION('',(1.,0.,0.));
#67578=DIRECTION('center_axis',(-1.,0.,0.));
#67579=DIRECTION('ref_axis',(0.,1.,0.));
#67580=DIRECTION('',(0.,1.,0.));
#67581=DIRECTION('',(0.,1.,0.));
#67582=DIRECTION('center_axis',(0.,0.,-1.));
#67583=DIRECTION('ref_axis',(-1.,0.,0.));
#67584=DIRECTION('center_axis',(0.,-1.,0.));
#67585=DIRECTION('ref_axis',(-1.,0.,0.));
#67586=DIRECTION('',(-1.,0.,0.));
#67587=DIRECTION('',(0.,0.,-1.));
#67588=DIRECTION('',(-1.,0.,0.));
#67589=DIRECTION('',(0.,0.,-1.));
#67590=DIRECTION('center_axis',(1.,0.,0.));
#67591=DIRECTION('ref_axis',(0.,-1.,0.));
#67592=DIRECTION('',(0.,-1.,0.));
#67593=DIRECTION('',(0.,0.,-1.));
#67594=DIRECTION('',(0.,-1.,0.));
#67595=DIRECTION('center_axis',(0.,1.,0.));
#67596=DIRECTION('ref_axis',(1.,0.,0.));
#67597=DIRECTION('',(1.,0.,0.));
#67598=DIRECTION('',(0.,0.,-1.));
#67599=DIRECTION('',(1.,0.,0.));
#67600=DIRECTION('center_axis',(-1.,0.,0.));
#67601=DIRECTION('ref_axis',(0.,1.,0.));
#67602=DIRECTION('',(0.,1.,0.));
#67603=DIRECTION('',(0.,1.,0.));
#67604=DIRECTION('center_axis',(0.,0.,-1.));
#67605=DIRECTION('ref_axis',(-1.,0.,0.));
#67606=DIRECTION('center_axis',(0.,-1.,0.));
#67607=DIRECTION('ref_axis',(-1.,0.,0.));
#67608=DIRECTION('',(-1.,0.,0.));
#67609=DIRECTION('',(0.,0.,-1.));
#67610=DIRECTION('',(-1.,0.,0.));
#67611=DIRECTION('',(0.,0.,-1.));
#67612=DIRECTION('center_axis',(1.,0.,0.));
#67613=DIRECTION('ref_axis',(0.,-1.,0.));
#67614=DIRECTION('',(0.,-1.,0.));
#67615=DIRECTION('',(0.,0.,-1.));
#67616=DIRECTION('',(0.,-1.,0.));
#67617=DIRECTION('center_axis',(0.,1.,0.));
#67618=DIRECTION('ref_axis',(1.,0.,0.));
#67619=DIRECTION('',(1.,0.,0.));
#67620=DIRECTION('',(0.,0.,-1.));
#67621=DIRECTION('',(1.,0.,0.));
#67622=DIRECTION('center_axis',(-1.,0.,0.));
#67623=DIRECTION('ref_axis',(0.,1.,0.));
#67624=DIRECTION('',(0.,1.,0.));
#67625=DIRECTION('',(0.,1.,0.));
#67626=DIRECTION('center_axis',(0.,0.,-1.));
#67627=DIRECTION('ref_axis',(-1.,0.,0.));
#67628=DIRECTION('center_axis',(0.,-1.,0.));
#67629=DIRECTION('ref_axis',(-1.,0.,0.));
#67630=DIRECTION('',(-1.,0.,0.));
#67631=DIRECTION('',(0.,0.,-1.));
#67632=DIRECTION('',(-1.,0.,0.));
#67633=DIRECTION('',(0.,0.,-1.));
#67634=DIRECTION('center_axis',(1.,0.,0.));
#67635=DIRECTION('ref_axis',(0.,-1.,0.));
#67636=DIRECTION('',(0.,-1.,0.));
#67637=DIRECTION('',(0.,0.,-1.));
#67638=DIRECTION('',(0.,-1.,0.));
#67639=DIRECTION('center_axis',(0.,1.,0.));
#67640=DIRECTION('ref_axis',(1.,0.,0.));
#67641=DIRECTION('',(1.,0.,0.));
#67642=DIRECTION('',(0.,0.,-1.));
#67643=DIRECTION('',(1.,0.,0.));
#67644=DIRECTION('center_axis',(-1.,0.,0.));
#67645=DIRECTION('ref_axis',(0.,1.,0.));
#67646=DIRECTION('',(0.,1.,0.));
#67647=DIRECTION('',(0.,1.,0.));
#67648=DIRECTION('center_axis',(0.,0.,-1.));
#67649=DIRECTION('ref_axis',(-1.,0.,0.));
#67650=DIRECTION('center_axis',(0.,-1.,0.));
#67651=DIRECTION('ref_axis',(-1.,0.,0.));
#67652=DIRECTION('',(-1.,0.,0.));
#67653=DIRECTION('',(0.,0.,-1.));
#67654=DIRECTION('',(-1.,0.,0.));
#67655=DIRECTION('',(0.,0.,-1.));
#67656=DIRECTION('center_axis',(1.,0.,0.));
#67657=DIRECTION('ref_axis',(0.,-1.,0.));
#67658=DIRECTION('',(0.,-1.,0.));
#67659=DIRECTION('',(0.,0.,-1.));
#67660=DIRECTION('',(0.,-1.,0.));
#67661=DIRECTION('center_axis',(0.,1.,0.));
#67662=DIRECTION('ref_axis',(1.,0.,0.));
#67663=DIRECTION('',(1.,0.,0.));
#67664=DIRECTION('',(0.,0.,-1.));
#67665=DIRECTION('',(1.,0.,0.));
#67666=DIRECTION('center_axis',(-1.,0.,0.));
#67667=DIRECTION('ref_axis',(0.,1.,0.));
#67668=DIRECTION('',(0.,1.,0.));
#67669=DIRECTION('',(0.,1.,0.));
#67670=DIRECTION('center_axis',(0.,0.,-1.));
#67671=DIRECTION('ref_axis',(-1.,0.,0.));
#67672=DIRECTION('center_axis',(0.,-1.,0.));
#67673=DIRECTION('ref_axis',(-1.,0.,0.));
#67674=DIRECTION('',(-1.,0.,0.));
#67675=DIRECTION('',(0.,0.,-1.));
#67676=DIRECTION('',(-1.,0.,0.));
#67677=DIRECTION('',(0.,0.,-1.));
#67678=DIRECTION('center_axis',(1.,0.,0.));
#67679=DIRECTION('ref_axis',(0.,-1.,0.));
#67680=DIRECTION('',(0.,-1.,0.));
#67681=DIRECTION('',(0.,0.,-1.));
#67682=DIRECTION('',(0.,-1.,0.));
#67683=DIRECTION('center_axis',(0.,1.,0.));
#67684=DIRECTION('ref_axis',(1.,0.,0.));
#67685=DIRECTION('',(1.,0.,0.));
#67686=DIRECTION('',(0.,0.,-1.));
#67687=DIRECTION('',(1.,0.,0.));
#67688=DIRECTION('center_axis',(-1.,0.,0.));
#67689=DIRECTION('ref_axis',(0.,1.,0.));
#67690=DIRECTION('',(0.,1.,0.));
#67691=DIRECTION('',(0.,1.,0.));
#67692=DIRECTION('center_axis',(0.,0.,-1.));
#67693=DIRECTION('ref_axis',(-1.,0.,0.));
#67694=DIRECTION('center_axis',(0.,-1.,0.));
#67695=DIRECTION('ref_axis',(-1.,0.,0.));
#67696=DIRECTION('',(-1.,0.,0.));
#67697=DIRECTION('',(0.,0.,-1.));
#67698=DIRECTION('',(-1.,0.,0.));
#67699=DIRECTION('',(0.,0.,-1.));
#67700=DIRECTION('center_axis',(1.,0.,0.));
#67701=DIRECTION('ref_axis',(0.,-1.,0.));
#67702=DIRECTION('',(0.,-1.,0.));
#67703=DIRECTION('',(0.,0.,-1.));
#67704=DIRECTION('',(0.,-1.,0.));
#67705=DIRECTION('center_axis',(0.,1.,0.));
#67706=DIRECTION('ref_axis',(1.,0.,0.));
#67707=DIRECTION('',(1.,0.,0.));
#67708=DIRECTION('',(0.,0.,-1.));
#67709=DIRECTION('',(1.,0.,0.));
#67710=DIRECTION('center_axis',(-1.,0.,0.));
#67711=DIRECTION('ref_axis',(0.,1.,0.));
#67712=DIRECTION('',(0.,1.,0.));
#67713=DIRECTION('',(0.,1.,0.));
#67714=DIRECTION('center_axis',(0.,0.,-1.));
#67715=DIRECTION('ref_axis',(-1.,0.,0.));
#67716=DIRECTION('center_axis',(0.,-1.,0.));
#67717=DIRECTION('ref_axis',(-1.,0.,0.));
#67718=DIRECTION('',(-1.,0.,0.));
#67719=DIRECTION('',(0.,0.,-1.));
#67720=DIRECTION('',(-1.,0.,0.));
#67721=DIRECTION('',(0.,0.,-1.));
#67722=DIRECTION('center_axis',(1.,0.,0.));
#67723=DIRECTION('ref_axis',(0.,-1.,0.));
#67724=DIRECTION('',(0.,-1.,0.));
#67725=DIRECTION('',(0.,0.,-1.));
#67726=DIRECTION('',(0.,-1.,0.));
#67727=DIRECTION('center_axis',(0.,1.,0.));
#67728=DIRECTION('ref_axis',(1.,0.,0.));
#67729=DIRECTION('',(1.,0.,0.));
#67730=DIRECTION('',(0.,0.,-1.));
#67731=DIRECTION('',(1.,0.,0.));
#67732=DIRECTION('center_axis',(-1.,0.,0.));
#67733=DIRECTION('ref_axis',(0.,1.,0.));
#67734=DIRECTION('',(0.,1.,0.));
#67735=DIRECTION('',(0.,1.,0.));
#67736=DIRECTION('center_axis',(0.,0.,-1.));
#67737=DIRECTION('ref_axis',(-1.,0.,0.));
#67738=DIRECTION('center_axis',(0.,-1.,0.));
#67739=DIRECTION('ref_axis',(-1.,0.,0.));
#67740=DIRECTION('',(-1.,0.,0.));
#67741=DIRECTION('',(0.,0.,-1.));
#67742=DIRECTION('',(-1.,0.,0.));
#67743=DIRECTION('',(0.,0.,-1.));
#67744=DIRECTION('center_axis',(1.,0.,0.));
#67745=DIRECTION('ref_axis',(0.,-1.,0.));
#67746=DIRECTION('',(0.,-1.,0.));
#67747=DIRECTION('',(0.,0.,-1.));
#67748=DIRECTION('',(0.,-1.,0.));
#67749=DIRECTION('center_axis',(0.,1.,0.));
#67750=DIRECTION('ref_axis',(1.,0.,0.));
#67751=DIRECTION('',(1.,0.,0.));
#67752=DIRECTION('',(0.,0.,-1.));
#67753=DIRECTION('',(1.,0.,0.));
#67754=DIRECTION('center_axis',(-1.,0.,0.));
#67755=DIRECTION('ref_axis',(0.,1.,0.));
#67756=DIRECTION('',(0.,1.,0.));
#67757=DIRECTION('',(0.,1.,0.));
#67758=DIRECTION('center_axis',(0.,0.,-1.));
#67759=DIRECTION('ref_axis',(-1.,0.,0.));
#67760=DIRECTION('center_axis',(0.,-1.,0.));
#67761=DIRECTION('ref_axis',(-1.,0.,0.));
#67762=DIRECTION('',(-1.,0.,0.));
#67763=DIRECTION('',(0.,0.,-1.));
#67764=DIRECTION('',(-1.,0.,0.));
#67765=DIRECTION('',(0.,0.,-1.));
#67766=DIRECTION('center_axis',(1.,0.,0.));
#67767=DIRECTION('ref_axis',(0.,-1.,0.));
#67768=DIRECTION('',(0.,-1.,0.));
#67769=DIRECTION('',(0.,0.,-1.));
#67770=DIRECTION('',(0.,-1.,0.));
#67771=DIRECTION('center_axis',(0.,1.,0.));
#67772=DIRECTION('ref_axis',(1.,0.,0.));
#67773=DIRECTION('',(1.,0.,0.));
#67774=DIRECTION('',(0.,0.,-1.));
#67775=DIRECTION('',(1.,0.,0.));
#67776=DIRECTION('center_axis',(-1.,0.,0.));
#67777=DIRECTION('ref_axis',(0.,1.,0.));
#67778=DIRECTION('',(0.,1.,0.));
#67779=DIRECTION('',(0.,1.,0.));
#67780=DIRECTION('center_axis',(0.,0.,-1.));
#67781=DIRECTION('ref_axis',(-1.,0.,0.));
#67782=DIRECTION('center_axis',(0.,-1.,0.));
#67783=DIRECTION('ref_axis',(-1.,0.,0.));
#67784=DIRECTION('',(-1.,0.,0.));
#67785=DIRECTION('',(0.,0.,-1.));
#67786=DIRECTION('',(-1.,0.,0.));
#67787=DIRECTION('',(0.,0.,-1.));
#67788=DIRECTION('center_axis',(1.,0.,0.));
#67789=DIRECTION('ref_axis',(0.,-1.,0.));
#67790=DIRECTION('',(0.,-1.,0.));
#67791=DIRECTION('',(0.,0.,-1.));
#67792=DIRECTION('',(0.,-1.,0.));
#67793=DIRECTION('center_axis',(0.,1.,0.));
#67794=DIRECTION('ref_axis',(1.,0.,0.));
#67795=DIRECTION('',(1.,0.,0.));
#67796=DIRECTION('',(0.,0.,-1.));
#67797=DIRECTION('',(1.,0.,0.));
#67798=DIRECTION('center_axis',(-1.,0.,0.));
#67799=DIRECTION('ref_axis',(0.,1.,0.));
#67800=DIRECTION('',(0.,1.,0.));
#67801=DIRECTION('',(0.,1.,0.));
#67802=DIRECTION('center_axis',(0.,0.,-1.));
#67803=DIRECTION('ref_axis',(-1.,0.,0.));
#67804=DIRECTION('center_axis',(0.,-1.,0.));
#67805=DIRECTION('ref_axis',(-1.,0.,0.));
#67806=DIRECTION('',(-1.,0.,0.));
#67807=DIRECTION('',(0.,0.,-1.));
#67808=DIRECTION('',(-1.,0.,0.));
#67809=DIRECTION('',(0.,0.,-1.));
#67810=DIRECTION('center_axis',(1.,0.,0.));
#67811=DIRECTION('ref_axis',(0.,-1.,0.));
#67812=DIRECTION('',(0.,-1.,0.));
#67813=DIRECTION('',(0.,0.,-1.));
#67814=DIRECTION('',(0.,-1.,0.));
#67815=DIRECTION('center_axis',(0.,1.,0.));
#67816=DIRECTION('ref_axis',(1.,0.,0.));
#67817=DIRECTION('',(1.,0.,0.));
#67818=DIRECTION('',(0.,0.,-1.));
#67819=DIRECTION('',(1.,0.,0.));
#67820=DIRECTION('center_axis',(-1.,0.,0.));
#67821=DIRECTION('ref_axis',(0.,1.,0.));
#67822=DIRECTION('',(0.,1.,0.));
#67823=DIRECTION('',(0.,1.,0.));
#67824=DIRECTION('center_axis',(0.,0.,-1.));
#67825=DIRECTION('ref_axis',(-1.,0.,0.));
#67826=DIRECTION('center_axis',(0.,-1.,0.));
#67827=DIRECTION('ref_axis',(-1.,0.,0.));
#67828=DIRECTION('',(-1.,0.,0.));
#67829=DIRECTION('',(0.,0.,-1.));
#67830=DIRECTION('',(-1.,0.,0.));
#67831=DIRECTION('',(0.,0.,-1.));
#67832=DIRECTION('center_axis',(1.,0.,0.));
#67833=DIRECTION('ref_axis',(0.,-1.,0.));
#67834=DIRECTION('',(0.,-1.,0.));
#67835=DIRECTION('',(0.,0.,-1.));
#67836=DIRECTION('',(0.,-1.,0.));
#67837=DIRECTION('center_axis',(0.,1.,0.));
#67838=DIRECTION('ref_axis',(1.,0.,0.));
#67839=DIRECTION('',(1.,0.,0.));
#67840=DIRECTION('',(0.,0.,-1.));
#67841=DIRECTION('',(1.,0.,0.));
#67842=DIRECTION('center_axis',(-1.,0.,0.));
#67843=DIRECTION('ref_axis',(0.,1.,0.));
#67844=DIRECTION('',(0.,1.,0.));
#67845=DIRECTION('',(0.,1.,0.));
#67846=DIRECTION('center_axis',(0.,0.,-1.));
#67847=DIRECTION('ref_axis',(-1.,0.,0.));
#67848=DIRECTION('center_axis',(0.,-1.,0.));
#67849=DIRECTION('ref_axis',(-1.,0.,0.));
#67850=DIRECTION('',(-1.,0.,0.));
#67851=DIRECTION('',(0.,0.,-1.));
#67852=DIRECTION('',(-1.,0.,0.));
#67853=DIRECTION('',(0.,0.,-1.));
#67854=DIRECTION('center_axis',(1.,0.,0.));
#67855=DIRECTION('ref_axis',(0.,-1.,0.));
#67856=DIRECTION('',(0.,-1.,0.));
#67857=DIRECTION('',(0.,0.,-1.));
#67858=DIRECTION('',(0.,-1.,0.));
#67859=DIRECTION('center_axis',(0.,1.,0.));
#67860=DIRECTION('ref_axis',(1.,0.,0.));
#67861=DIRECTION('',(1.,0.,0.));
#67862=DIRECTION('',(0.,0.,-1.));
#67863=DIRECTION('',(1.,0.,0.));
#67864=DIRECTION('center_axis',(-1.,0.,0.));
#67865=DIRECTION('ref_axis',(0.,1.,0.));
#67866=DIRECTION('',(0.,1.,0.));
#67867=DIRECTION('',(0.,1.,0.));
#67868=DIRECTION('center_axis',(0.,0.,-1.));
#67869=DIRECTION('ref_axis',(-1.,0.,0.));
#67870=DIRECTION('center_axis',(0.,-1.,0.));
#67871=DIRECTION('ref_axis',(-1.,0.,0.));
#67872=DIRECTION('',(-1.,0.,0.));
#67873=DIRECTION('',(0.,0.,-1.));
#67874=DIRECTION('',(-1.,0.,0.));
#67875=DIRECTION('',(0.,0.,-1.));
#67876=DIRECTION('center_axis',(1.,0.,0.));
#67877=DIRECTION('ref_axis',(0.,-1.,0.));
#67878=DIRECTION('',(0.,-1.,0.));
#67879=DIRECTION('',(0.,0.,-1.));
#67880=DIRECTION('',(0.,-1.,0.));
#67881=DIRECTION('center_axis',(0.,1.,0.));
#67882=DIRECTION('ref_axis',(1.,0.,0.));
#67883=DIRECTION('',(1.,0.,0.));
#67884=DIRECTION('',(0.,0.,-1.));
#67885=DIRECTION('',(1.,0.,0.));
#67886=DIRECTION('center_axis',(-1.,0.,0.));
#67887=DIRECTION('ref_axis',(0.,1.,0.));
#67888=DIRECTION('',(0.,1.,0.));
#67889=DIRECTION('',(0.,1.,0.));
#67890=DIRECTION('center_axis',(0.,0.,-1.));
#67891=DIRECTION('ref_axis',(-1.,0.,0.));
#67892=DIRECTION('center_axis',(0.,-1.,0.));
#67893=DIRECTION('ref_axis',(-1.,0.,0.));
#67894=DIRECTION('',(-1.,0.,0.));
#67895=DIRECTION('',(0.,0.,-1.));
#67896=DIRECTION('',(-1.,0.,0.));
#67897=DIRECTION('',(0.,0.,-1.));
#67898=DIRECTION('center_axis',(1.,0.,0.));
#67899=DIRECTION('ref_axis',(0.,-1.,0.));
#67900=DIRECTION('',(0.,-1.,0.));
#67901=DIRECTION('',(0.,0.,-1.));
#67902=DIRECTION('',(0.,-1.,0.));
#67903=DIRECTION('center_axis',(0.,1.,0.));
#67904=DIRECTION('ref_axis',(1.,0.,0.));
#67905=DIRECTION('',(1.,0.,0.));
#67906=DIRECTION('',(0.,0.,-1.));
#67907=DIRECTION('',(1.,0.,0.));
#67908=DIRECTION('center_axis',(-1.,0.,0.));
#67909=DIRECTION('ref_axis',(0.,1.,0.));
#67910=DIRECTION('',(0.,1.,0.));
#67911=DIRECTION('',(0.,1.,0.));
#67912=DIRECTION('center_axis',(0.,0.,-1.));
#67913=DIRECTION('ref_axis',(-1.,0.,0.));
#67914=DIRECTION('center_axis',(0.,-1.,0.));
#67915=DIRECTION('ref_axis',(-1.,0.,0.));
#67916=DIRECTION('',(-1.,0.,0.));
#67917=DIRECTION('',(0.,0.,-1.));
#67918=DIRECTION('',(-1.,0.,0.));
#67919=DIRECTION('',(0.,0.,-1.));
#67920=DIRECTION('center_axis',(1.,0.,0.));
#67921=DIRECTION('ref_axis',(0.,-1.,0.));
#67922=DIRECTION('',(0.,-1.,0.));
#67923=DIRECTION('',(0.,0.,-1.));
#67924=DIRECTION('',(0.,-1.,0.));
#67925=DIRECTION('center_axis',(0.,1.,0.));
#67926=DIRECTION('ref_axis',(1.,0.,0.));
#67927=DIRECTION('',(1.,0.,0.));
#67928=DIRECTION('',(0.,0.,-1.));
#67929=DIRECTION('',(1.,0.,0.));
#67930=DIRECTION('center_axis',(-1.,0.,0.));
#67931=DIRECTION('ref_axis',(0.,1.,0.));
#67932=DIRECTION('',(0.,1.,0.));
#67933=DIRECTION('',(0.,1.,0.));
#67934=DIRECTION('center_axis',(0.,0.,-1.));
#67935=DIRECTION('ref_axis',(-1.,0.,0.));
#67936=DIRECTION('center_axis',(0.,-1.,0.));
#67937=DIRECTION('ref_axis',(-1.,0.,0.));
#67938=DIRECTION('',(-1.,0.,0.));
#67939=DIRECTION('',(0.,0.,-1.));
#67940=DIRECTION('',(-1.,0.,0.));
#67941=DIRECTION('',(0.,0.,-1.));
#67942=DIRECTION('center_axis',(1.,0.,0.));
#67943=DIRECTION('ref_axis',(0.,-1.,0.));
#67944=DIRECTION('',(0.,-1.,0.));
#67945=DIRECTION('',(0.,0.,-1.));
#67946=DIRECTION('',(0.,-1.,0.));
#67947=DIRECTION('center_axis',(0.,1.,0.));
#67948=DIRECTION('ref_axis',(1.,0.,0.));
#67949=DIRECTION('',(1.,0.,0.));
#67950=DIRECTION('',(0.,0.,-1.));
#67951=DIRECTION('',(1.,0.,0.));
#67952=DIRECTION('center_axis',(-1.,0.,0.));
#67953=DIRECTION('ref_axis',(0.,1.,0.));
#67954=DIRECTION('',(0.,1.,0.));
#67955=DIRECTION('',(0.,1.,0.));
#67956=DIRECTION('center_axis',(0.,0.,-1.));
#67957=DIRECTION('ref_axis',(-1.,0.,0.));
#67958=DIRECTION('center_axis',(0.,-1.,0.));
#67959=DIRECTION('ref_axis',(-1.,0.,0.));
#67960=DIRECTION('',(-1.,0.,0.));
#67961=DIRECTION('',(0.,0.,-1.));
#67962=DIRECTION('',(-1.,0.,0.));
#67963=DIRECTION('',(0.,0.,-1.));
#67964=DIRECTION('center_axis',(1.,0.,0.));
#67965=DIRECTION('ref_axis',(0.,-1.,0.));
#67966=DIRECTION('',(0.,-1.,0.));
#67967=DIRECTION('',(0.,0.,-1.));
#67968=DIRECTION('',(0.,-1.,0.));
#67969=DIRECTION('center_axis',(0.,1.,0.));
#67970=DIRECTION('ref_axis',(1.,0.,0.));
#67971=DIRECTION('',(1.,0.,0.));
#67972=DIRECTION('',(0.,0.,-1.));
#67973=DIRECTION('',(1.,0.,0.));
#67974=DIRECTION('center_axis',(-1.,0.,0.));
#67975=DIRECTION('ref_axis',(0.,1.,0.));
#67976=DIRECTION('',(0.,1.,0.));
#67977=DIRECTION('',(0.,1.,0.));
#67978=DIRECTION('center_axis',(0.,0.,-1.));
#67979=DIRECTION('ref_axis',(-1.,0.,0.));
#67980=DIRECTION('center_axis',(0.,-1.,0.));
#67981=DIRECTION('ref_axis',(-1.,0.,0.));
#67982=DIRECTION('',(-1.,0.,0.));
#67983=DIRECTION('',(0.,0.,-1.));
#67984=DIRECTION('',(-1.,0.,0.));
#67985=DIRECTION('',(0.,0.,-1.));
#67986=DIRECTION('center_axis',(1.,0.,0.));
#67987=DIRECTION('ref_axis',(0.,-1.,0.));
#67988=DIRECTION('',(0.,-1.,0.));
#67989=DIRECTION('',(0.,0.,-1.));
#67990=DIRECTION('',(0.,-1.,0.));
#67991=DIRECTION('center_axis',(0.,1.,0.));
#67992=DIRECTION('ref_axis',(1.,0.,0.));
#67993=DIRECTION('',(1.,0.,0.));
#67994=DIRECTION('',(0.,0.,-1.));
#67995=DIRECTION('',(1.,0.,0.));
#67996=DIRECTION('center_axis',(-1.,0.,0.));
#67997=DIRECTION('ref_axis',(0.,1.,0.));
#67998=DIRECTION('',(0.,1.,0.));
#67999=DIRECTION('',(0.,1.,0.));
#68000=DIRECTION('center_axis',(0.,0.,-1.));
#68001=DIRECTION('ref_axis',(-1.,0.,0.));
#68002=DIRECTION('center_axis',(0.,-1.,0.));
#68003=DIRECTION('ref_axis',(-1.,0.,0.));
#68004=DIRECTION('',(-1.,0.,0.));
#68005=DIRECTION('',(0.,0.,-1.));
#68006=DIRECTION('',(-1.,0.,0.));
#68007=DIRECTION('',(0.,0.,-1.));
#68008=DIRECTION('center_axis',(1.,0.,0.));
#68009=DIRECTION('ref_axis',(0.,-1.,0.));
#68010=DIRECTION('',(0.,-1.,0.));
#68011=DIRECTION('',(0.,0.,-1.));
#68012=DIRECTION('',(0.,-1.,0.));
#68013=DIRECTION('center_axis',(0.,1.,0.));
#68014=DIRECTION('ref_axis',(1.,0.,0.));
#68015=DIRECTION('',(1.,0.,0.));
#68016=DIRECTION('',(0.,0.,-1.));
#68017=DIRECTION('',(1.,0.,0.));
#68018=DIRECTION('center_axis',(-1.,0.,0.));
#68019=DIRECTION('ref_axis',(0.,1.,0.));
#68020=DIRECTION('',(0.,1.,0.));
#68021=DIRECTION('',(0.,1.,0.));
#68022=DIRECTION('center_axis',(0.,0.,-1.));
#68023=DIRECTION('ref_axis',(-1.,0.,0.));
#68024=DIRECTION('center_axis',(0.,-1.,0.));
#68025=DIRECTION('ref_axis',(-1.,0.,0.));
#68026=DIRECTION('',(-1.,0.,0.));
#68027=DIRECTION('',(0.,0.,-1.));
#68028=DIRECTION('',(-1.,0.,0.));
#68029=DIRECTION('',(0.,0.,-1.));
#68030=DIRECTION('center_axis',(1.,0.,0.));
#68031=DIRECTION('ref_axis',(0.,-1.,0.));
#68032=DIRECTION('',(0.,-1.,0.));
#68033=DIRECTION('',(0.,0.,-1.));
#68034=DIRECTION('',(0.,-1.,0.));
#68035=DIRECTION('center_axis',(0.,1.,0.));
#68036=DIRECTION('ref_axis',(1.,0.,0.));
#68037=DIRECTION('',(1.,0.,0.));
#68038=DIRECTION('',(0.,0.,-1.));
#68039=DIRECTION('',(1.,0.,0.));
#68040=DIRECTION('center_axis',(-1.,0.,0.));
#68041=DIRECTION('ref_axis',(0.,1.,0.));
#68042=DIRECTION('',(0.,1.,0.));
#68043=DIRECTION('',(0.,1.,0.));
#68044=DIRECTION('center_axis',(0.,0.,-1.));
#68045=DIRECTION('ref_axis',(-1.,0.,0.));
#68046=DIRECTION('center_axis',(0.,-1.,0.));
#68047=DIRECTION('ref_axis',(-1.,0.,0.));
#68048=DIRECTION('',(-1.,0.,0.));
#68049=DIRECTION('',(0.,0.,-1.));
#68050=DIRECTION('',(-1.,0.,0.));
#68051=DIRECTION('',(0.,0.,-1.));
#68052=DIRECTION('center_axis',(1.,0.,0.));
#68053=DIRECTION('ref_axis',(0.,-1.,0.));
#68054=DIRECTION('',(0.,-1.,0.));
#68055=DIRECTION('',(0.,0.,-1.));
#68056=DIRECTION('',(0.,-1.,0.));
#68057=DIRECTION('center_axis',(0.,1.,0.));
#68058=DIRECTION('ref_axis',(1.,0.,0.));
#68059=DIRECTION('',(1.,0.,0.));
#68060=DIRECTION('',(0.,0.,-1.));
#68061=DIRECTION('',(1.,0.,0.));
#68062=DIRECTION('center_axis',(-1.,0.,0.));
#68063=DIRECTION('ref_axis',(0.,1.,0.));
#68064=DIRECTION('',(0.,1.,0.));
#68065=DIRECTION('',(0.,1.,0.));
#68066=DIRECTION('center_axis',(0.,0.,-1.));
#68067=DIRECTION('ref_axis',(-1.,0.,0.));
#68068=DIRECTION('center_axis',(0.,-1.,0.));
#68069=DIRECTION('ref_axis',(-1.,0.,0.));
#68070=DIRECTION('',(-1.,0.,0.));
#68071=DIRECTION('',(0.,0.,-1.));
#68072=DIRECTION('',(-1.,0.,0.));
#68073=DIRECTION('',(0.,0.,-1.));
#68074=DIRECTION('center_axis',(1.,0.,0.));
#68075=DIRECTION('ref_axis',(0.,-1.,0.));
#68076=DIRECTION('',(0.,-1.,0.));
#68077=DIRECTION('',(0.,0.,-1.));
#68078=DIRECTION('',(0.,-1.,0.));
#68079=DIRECTION('center_axis',(0.,1.,0.));
#68080=DIRECTION('ref_axis',(1.,0.,0.));
#68081=DIRECTION('',(1.,0.,0.));
#68082=DIRECTION('',(0.,0.,-1.));
#68083=DIRECTION('',(1.,0.,0.));
#68084=DIRECTION('center_axis',(-1.,0.,0.));
#68085=DIRECTION('ref_axis',(0.,1.,0.));
#68086=DIRECTION('',(0.,1.,0.));
#68087=DIRECTION('',(0.,1.,0.));
#68088=DIRECTION('center_axis',(0.,0.,-1.));
#68089=DIRECTION('ref_axis',(-1.,0.,0.));
#68090=DIRECTION('center_axis',(0.,-1.,0.));
#68091=DIRECTION('ref_axis',(-1.,0.,0.));
#68092=DIRECTION('',(-1.,0.,0.));
#68093=DIRECTION('',(0.,0.,-1.));
#68094=DIRECTION('',(-1.,0.,0.));
#68095=DIRECTION('',(0.,0.,-1.));
#68096=DIRECTION('center_axis',(1.,0.,0.));
#68097=DIRECTION('ref_axis',(0.,-1.,0.));
#68098=DIRECTION('',(0.,-1.,0.));
#68099=DIRECTION('',(0.,0.,-1.));
#68100=DIRECTION('',(0.,-1.,0.));
#68101=DIRECTION('center_axis',(0.,1.,0.));
#68102=DIRECTION('ref_axis',(1.,0.,0.));
#68103=DIRECTION('',(1.,0.,0.));
#68104=DIRECTION('',(0.,0.,-1.));
#68105=DIRECTION('',(1.,0.,0.));
#68106=DIRECTION('center_axis',(-1.,0.,0.));
#68107=DIRECTION('ref_axis',(0.,1.,0.));
#68108=DIRECTION('',(0.,1.,0.));
#68109=DIRECTION('',(0.,1.,0.));
#68110=DIRECTION('center_axis',(0.,0.,-1.));
#68111=DIRECTION('ref_axis',(-1.,0.,0.));
#68112=DIRECTION('center_axis',(0.,-1.,0.));
#68113=DIRECTION('ref_axis',(-1.,0.,0.));
#68114=DIRECTION('',(-1.,0.,0.));
#68115=DIRECTION('',(0.,0.,-1.));
#68116=DIRECTION('',(-1.,0.,0.));
#68117=DIRECTION('',(0.,0.,-1.));
#68118=DIRECTION('center_axis',(1.,0.,0.));
#68119=DIRECTION('ref_axis',(0.,-1.,0.));
#68120=DIRECTION('',(0.,-1.,0.));
#68121=DIRECTION('',(0.,0.,-1.));
#68122=DIRECTION('',(0.,-1.,0.));
#68123=DIRECTION('center_axis',(0.,1.,0.));
#68124=DIRECTION('ref_axis',(1.,0.,0.));
#68125=DIRECTION('',(1.,0.,0.));
#68126=DIRECTION('',(0.,0.,-1.));
#68127=DIRECTION('',(1.,0.,0.));
#68128=DIRECTION('center_axis',(-1.,0.,0.));
#68129=DIRECTION('ref_axis',(0.,1.,0.));
#68130=DIRECTION('',(0.,1.,0.));
#68131=DIRECTION('',(0.,1.,0.));
#68132=DIRECTION('center_axis',(0.,0.,-1.));
#68133=DIRECTION('ref_axis',(-1.,0.,0.));
#68134=DIRECTION('center_axis',(0.,-1.,0.));
#68135=DIRECTION('ref_axis',(-1.,0.,0.));
#68136=DIRECTION('',(-1.,0.,0.));
#68137=DIRECTION('',(0.,0.,-1.));
#68138=DIRECTION('',(-1.,0.,0.));
#68139=DIRECTION('',(0.,0.,-1.));
#68140=DIRECTION('center_axis',(1.,0.,0.));
#68141=DIRECTION('ref_axis',(0.,-1.,0.));
#68142=DIRECTION('',(0.,-1.,0.));
#68143=DIRECTION('',(0.,0.,-1.));
#68144=DIRECTION('',(0.,-1.,0.));
#68145=DIRECTION('center_axis',(0.,1.,0.));
#68146=DIRECTION('ref_axis',(1.,0.,0.));
#68147=DIRECTION('',(1.,0.,0.));
#68148=DIRECTION('',(0.,0.,-1.));
#68149=DIRECTION('',(1.,0.,0.));
#68150=DIRECTION('center_axis',(-1.,0.,0.));
#68151=DIRECTION('ref_axis',(0.,1.,0.));
#68152=DIRECTION('',(0.,1.,0.));
#68153=DIRECTION('',(0.,1.,0.));
#68154=DIRECTION('center_axis',(0.,0.,-1.));
#68155=DIRECTION('ref_axis',(-1.,0.,0.));
#68156=DIRECTION('center_axis',(0.,-1.,0.));
#68157=DIRECTION('ref_axis',(-1.,0.,0.));
#68158=DIRECTION('',(-1.,0.,0.));
#68159=DIRECTION('',(0.,0.,-1.));
#68160=DIRECTION('',(-1.,0.,0.));
#68161=DIRECTION('',(0.,0.,-1.));
#68162=DIRECTION('center_axis',(1.,0.,0.));
#68163=DIRECTION('ref_axis',(0.,-1.,0.));
#68164=DIRECTION('',(0.,-1.,0.));
#68165=DIRECTION('',(0.,0.,-1.));
#68166=DIRECTION('',(0.,-1.,0.));
#68167=DIRECTION('center_axis',(0.,1.,0.));
#68168=DIRECTION('ref_axis',(1.,0.,0.));
#68169=DIRECTION('',(1.,0.,0.));
#68170=DIRECTION('',(0.,0.,-1.));
#68171=DIRECTION('',(1.,0.,0.));
#68172=DIRECTION('center_axis',(-1.,0.,0.));
#68173=DIRECTION('ref_axis',(0.,1.,0.));
#68174=DIRECTION('',(0.,1.,0.));
#68175=DIRECTION('',(0.,1.,0.));
#68176=DIRECTION('center_axis',(0.,0.,-1.));
#68177=DIRECTION('ref_axis',(-1.,0.,0.));
#68178=DIRECTION('center_axis',(0.,-1.,0.));
#68179=DIRECTION('ref_axis',(-1.,0.,0.));
#68180=DIRECTION('',(-1.,0.,0.));
#68181=DIRECTION('',(0.,0.,-1.));
#68182=DIRECTION('',(-1.,0.,0.));
#68183=DIRECTION('',(0.,0.,-1.));
#68184=DIRECTION('center_axis',(1.,0.,0.));
#68185=DIRECTION('ref_axis',(0.,-1.,0.));
#68186=DIRECTION('',(0.,-1.,0.));
#68187=DIRECTION('',(0.,0.,-1.));
#68188=DIRECTION('',(0.,-1.,0.));
#68189=DIRECTION('center_axis',(0.,1.,0.));
#68190=DIRECTION('ref_axis',(1.,0.,0.));
#68191=DIRECTION('',(1.,0.,0.));
#68192=DIRECTION('',(0.,0.,-1.));
#68193=DIRECTION('',(1.,0.,0.));
#68194=DIRECTION('center_axis',(-1.,0.,0.));
#68195=DIRECTION('ref_axis',(0.,1.,0.));
#68196=DIRECTION('',(0.,1.,0.));
#68197=DIRECTION('',(0.,1.,0.));
#68198=DIRECTION('center_axis',(0.,0.,-1.));
#68199=DIRECTION('ref_axis',(-1.,0.,0.));
#68200=DIRECTION('center_axis',(0.,-1.,0.));
#68201=DIRECTION('ref_axis',(-1.,0.,0.));
#68202=DIRECTION('',(-1.,0.,0.));
#68203=DIRECTION('',(0.,0.,-1.));
#68204=DIRECTION('',(-1.,0.,0.));
#68205=DIRECTION('',(0.,0.,-1.));
#68206=DIRECTION('center_axis',(1.,0.,0.));
#68207=DIRECTION('ref_axis',(0.,-1.,0.));
#68208=DIRECTION('',(0.,-1.,0.));
#68209=DIRECTION('',(0.,0.,-1.));
#68210=DIRECTION('',(0.,-1.,0.));
#68211=DIRECTION('center_axis',(0.,1.,0.));
#68212=DIRECTION('ref_axis',(1.,0.,0.));
#68213=DIRECTION('',(1.,0.,0.));
#68214=DIRECTION('',(0.,0.,-1.));
#68215=DIRECTION('',(1.,0.,0.));
#68216=DIRECTION('center_axis',(-1.,0.,0.));
#68217=DIRECTION('ref_axis',(0.,1.,0.));
#68218=DIRECTION('',(0.,1.,0.));
#68219=DIRECTION('',(0.,1.,0.));
#68220=DIRECTION('center_axis',(0.,0.,-1.));
#68221=DIRECTION('ref_axis',(-1.,0.,0.));
#68222=DIRECTION('center_axis',(0.,-1.,0.));
#68223=DIRECTION('ref_axis',(-1.,0.,0.));
#68224=DIRECTION('',(-1.,0.,0.));
#68225=DIRECTION('',(0.,0.,-1.));
#68226=DIRECTION('',(-1.,0.,0.));
#68227=DIRECTION('',(0.,0.,-1.));
#68228=DIRECTION('center_axis',(1.,0.,0.));
#68229=DIRECTION('ref_axis',(0.,-1.,0.));
#68230=DIRECTION('',(0.,-1.,0.));
#68231=DIRECTION('',(0.,0.,-1.));
#68232=DIRECTION('',(0.,-1.,0.));
#68233=DIRECTION('center_axis',(0.,1.,0.));
#68234=DIRECTION('ref_axis',(1.,0.,0.));
#68235=DIRECTION('',(1.,0.,0.));
#68236=DIRECTION('',(0.,0.,-1.));
#68237=DIRECTION('',(1.,0.,0.));
#68238=DIRECTION('center_axis',(-1.,0.,0.));
#68239=DIRECTION('ref_axis',(0.,1.,0.));
#68240=DIRECTION('',(0.,1.,0.));
#68241=DIRECTION('',(0.,1.,0.));
#68242=DIRECTION('center_axis',(0.,0.,-1.));
#68243=DIRECTION('ref_axis',(-1.,0.,0.));
#68244=DIRECTION('center_axis',(0.,-1.,0.));
#68245=DIRECTION('ref_axis',(-1.,0.,0.));
#68246=DIRECTION('',(-1.,0.,0.));
#68247=DIRECTION('',(0.,0.,-1.));
#68248=DIRECTION('',(-1.,0.,0.));
#68249=DIRECTION('',(0.,0.,-1.));
#68250=DIRECTION('center_axis',(1.,0.,0.));
#68251=DIRECTION('ref_axis',(0.,-1.,0.));
#68252=DIRECTION('',(0.,-1.,0.));
#68253=DIRECTION('',(0.,0.,-1.));
#68254=DIRECTION('',(0.,-1.,0.));
#68255=DIRECTION('center_axis',(0.,1.,0.));
#68256=DIRECTION('ref_axis',(1.,0.,0.));
#68257=DIRECTION('',(1.,0.,0.));
#68258=DIRECTION('',(0.,0.,-1.));
#68259=DIRECTION('',(1.,0.,0.));
#68260=DIRECTION('center_axis',(-1.,0.,0.));
#68261=DIRECTION('ref_axis',(0.,1.,0.));
#68262=DIRECTION('',(0.,1.,0.));
#68263=DIRECTION('',(0.,1.,0.));
#68264=DIRECTION('center_axis',(0.,0.,-1.));
#68265=DIRECTION('ref_axis',(-1.,0.,0.));
#68266=DIRECTION('center_axis',(0.,-1.,0.));
#68267=DIRECTION('ref_axis',(-1.,0.,0.));
#68268=DIRECTION('',(-1.,0.,0.));
#68269=DIRECTION('',(0.,0.,-1.));
#68270=DIRECTION('',(-1.,0.,0.));
#68271=DIRECTION('',(0.,0.,-1.));
#68272=DIRECTION('center_axis',(1.,0.,0.));
#68273=DIRECTION('ref_axis',(0.,-1.,0.));
#68274=DIRECTION('',(0.,-1.,0.));
#68275=DIRECTION('',(0.,0.,-1.));
#68276=DIRECTION('',(0.,-1.,0.));
#68277=DIRECTION('center_axis',(0.,1.,0.));
#68278=DIRECTION('ref_axis',(1.,0.,0.));
#68279=DIRECTION('',(1.,0.,0.));
#68280=DIRECTION('',(0.,0.,-1.));
#68281=DIRECTION('',(1.,0.,0.));
#68282=DIRECTION('center_axis',(-1.,0.,0.));
#68283=DIRECTION('ref_axis',(0.,1.,0.));
#68284=DIRECTION('',(0.,1.,0.));
#68285=DIRECTION('',(0.,1.,0.));
#68286=DIRECTION('center_axis',(0.,0.,-1.));
#68287=DIRECTION('ref_axis',(-1.,0.,0.));
#68288=DIRECTION('center_axis',(0.,-1.,0.));
#68289=DIRECTION('ref_axis',(-1.,0.,0.));
#68290=DIRECTION('',(-1.,0.,0.));
#68291=DIRECTION('',(0.,0.,-1.));
#68292=DIRECTION('',(-1.,0.,0.));
#68293=DIRECTION('',(0.,0.,-1.));
#68294=DIRECTION('center_axis',(1.,0.,0.));
#68295=DIRECTION('ref_axis',(0.,-1.,0.));
#68296=DIRECTION('',(0.,-1.,0.));
#68297=DIRECTION('',(0.,0.,-1.));
#68298=DIRECTION('',(0.,-1.,0.));
#68299=DIRECTION('center_axis',(0.,1.,0.));
#68300=DIRECTION('ref_axis',(1.,0.,0.));
#68301=DIRECTION('',(1.,0.,0.));
#68302=DIRECTION('',(0.,0.,-1.));
#68303=DIRECTION('',(1.,0.,0.));
#68304=DIRECTION('center_axis',(-1.,0.,0.));
#68305=DIRECTION('ref_axis',(0.,1.,0.));
#68306=DIRECTION('',(0.,1.,0.));
#68307=DIRECTION('',(0.,1.,0.));
#68308=DIRECTION('center_axis',(0.,0.,-1.));
#68309=DIRECTION('ref_axis',(-1.,0.,0.));
#68310=DIRECTION('center_axis',(0.,-1.,0.));
#68311=DIRECTION('ref_axis',(-1.,0.,0.));
#68312=DIRECTION('',(-1.,0.,0.));
#68313=DIRECTION('',(0.,0.,-1.));
#68314=DIRECTION('',(-1.,0.,0.));
#68315=DIRECTION('',(0.,0.,-1.));
#68316=DIRECTION('center_axis',(1.,0.,0.));
#68317=DIRECTION('ref_axis',(0.,-1.,0.));
#68318=DIRECTION('',(0.,-1.,0.));
#68319=DIRECTION('',(0.,0.,-1.));
#68320=DIRECTION('',(0.,-1.,0.));
#68321=DIRECTION('center_axis',(0.,1.,0.));
#68322=DIRECTION('ref_axis',(1.,0.,0.));
#68323=DIRECTION('',(1.,0.,0.));
#68324=DIRECTION('',(0.,0.,-1.));
#68325=DIRECTION('',(1.,0.,0.));
#68326=DIRECTION('center_axis',(-1.,0.,0.));
#68327=DIRECTION('ref_axis',(0.,1.,0.));
#68328=DIRECTION('',(0.,1.,0.));
#68329=DIRECTION('',(0.,1.,0.));
#68330=DIRECTION('center_axis',(0.,0.,-1.));
#68331=DIRECTION('ref_axis',(-1.,0.,0.));
#68332=DIRECTION('center_axis',(0.,-1.,0.));
#68333=DIRECTION('ref_axis',(-1.,0.,0.));
#68334=DIRECTION('',(-1.,0.,0.));
#68335=DIRECTION('',(0.,0.,-1.));
#68336=DIRECTION('',(-1.,0.,0.));
#68337=DIRECTION('',(0.,0.,-1.));
#68338=DIRECTION('center_axis',(1.,0.,0.));
#68339=DIRECTION('ref_axis',(0.,-1.,0.));
#68340=DIRECTION('',(0.,-1.,0.));
#68341=DIRECTION('',(0.,0.,-1.));
#68342=DIRECTION('',(0.,-1.,0.));
#68343=DIRECTION('center_axis',(0.,1.,0.));
#68344=DIRECTION('ref_axis',(1.,0.,0.));
#68345=DIRECTION('',(1.,0.,0.));
#68346=DIRECTION('',(0.,0.,-1.));
#68347=DIRECTION('',(1.,0.,0.));
#68348=DIRECTION('center_axis',(-1.,0.,0.));
#68349=DIRECTION('ref_axis',(0.,1.,0.));
#68350=DIRECTION('',(0.,1.,0.));
#68351=DIRECTION('',(0.,1.,0.));
#68352=DIRECTION('center_axis',(0.,0.,-1.));
#68353=DIRECTION('ref_axis',(-1.,0.,0.));
#68354=DIRECTION('center_axis',(0.,-1.,0.));
#68355=DIRECTION('ref_axis',(-1.,0.,0.));
#68356=DIRECTION('',(-1.,0.,0.));
#68357=DIRECTION('',(0.,0.,-1.));
#68358=DIRECTION('',(-1.,0.,0.));
#68359=DIRECTION('',(0.,0.,-1.));
#68360=DIRECTION('center_axis',(1.,0.,0.));
#68361=DIRECTION('ref_axis',(0.,-1.,0.));
#68362=DIRECTION('',(0.,-1.,0.));
#68363=DIRECTION('',(0.,0.,-1.));
#68364=DIRECTION('',(0.,-1.,0.));
#68365=DIRECTION('center_axis',(0.,1.,0.));
#68366=DIRECTION('ref_axis',(1.,0.,0.));
#68367=DIRECTION('',(1.,0.,0.));
#68368=DIRECTION('',(0.,0.,-1.));
#68369=DIRECTION('',(1.,0.,0.));
#68370=DIRECTION('center_axis',(-1.,0.,0.));
#68371=DIRECTION('ref_axis',(0.,1.,0.));
#68372=DIRECTION('',(0.,1.,0.));
#68373=DIRECTION('',(0.,1.,0.));
#68374=DIRECTION('center_axis',(0.,0.,-1.));
#68375=DIRECTION('ref_axis',(-1.,0.,0.));
#68376=DIRECTION('center_axis',(0.,-1.,0.));
#68377=DIRECTION('ref_axis',(-1.,0.,0.));
#68378=DIRECTION('',(-1.,0.,0.));
#68379=DIRECTION('',(0.,0.,-1.));
#68380=DIRECTION('',(-1.,0.,0.));
#68381=DIRECTION('',(0.,0.,-1.));
#68382=DIRECTION('center_axis',(1.,0.,0.));
#68383=DIRECTION('ref_axis',(0.,-1.,0.));
#68384=DIRECTION('',(0.,-1.,0.));
#68385=DIRECTION('',(0.,0.,-1.));
#68386=DIRECTION('',(0.,-1.,0.));
#68387=DIRECTION('center_axis',(0.,1.,0.));
#68388=DIRECTION('ref_axis',(1.,0.,0.));
#68389=DIRECTION('',(1.,0.,0.));
#68390=DIRECTION('',(0.,0.,-1.));
#68391=DIRECTION('',(1.,0.,0.));
#68392=DIRECTION('center_axis',(-1.,0.,0.));
#68393=DIRECTION('ref_axis',(0.,1.,0.));
#68394=DIRECTION('',(0.,1.,0.));
#68395=DIRECTION('',(0.,1.,0.));
#68396=DIRECTION('center_axis',(0.,0.,-1.));
#68397=DIRECTION('ref_axis',(-1.,0.,0.));
#68398=DIRECTION('center_axis',(0.,-1.,0.));
#68399=DIRECTION('ref_axis',(-1.,0.,0.));
#68400=DIRECTION('',(-1.,0.,0.));
#68401=DIRECTION('',(0.,0.,-1.));
#68402=DIRECTION('',(-1.,0.,0.));
#68403=DIRECTION('',(0.,0.,-1.));
#68404=DIRECTION('center_axis',(1.,0.,0.));
#68405=DIRECTION('ref_axis',(0.,-1.,0.));
#68406=DIRECTION('',(0.,-1.,0.));
#68407=DIRECTION('',(0.,0.,-1.));
#68408=DIRECTION('',(0.,-1.,0.));
#68409=DIRECTION('center_axis',(0.,1.,0.));
#68410=DIRECTION('ref_axis',(1.,0.,0.));
#68411=DIRECTION('',(1.,0.,0.));
#68412=DIRECTION('',(0.,0.,-1.));
#68413=DIRECTION('',(1.,0.,0.));
#68414=DIRECTION('center_axis',(-1.,0.,0.));
#68415=DIRECTION('ref_axis',(0.,1.,0.));
#68416=DIRECTION('',(0.,1.,0.));
#68417=DIRECTION('',(0.,1.,0.));
#68418=DIRECTION('center_axis',(0.,0.,-1.));
#68419=DIRECTION('ref_axis',(-1.,0.,0.));
#68420=DIRECTION('center_axis',(0.,-1.,0.));
#68421=DIRECTION('ref_axis',(-1.,0.,0.));
#68422=DIRECTION('',(-1.,0.,0.));
#68423=DIRECTION('',(0.,0.,-1.));
#68424=DIRECTION('',(-1.,0.,0.));
#68425=DIRECTION('',(0.,0.,-1.));
#68426=DIRECTION('center_axis',(1.,0.,0.));
#68427=DIRECTION('ref_axis',(0.,-1.,0.));
#68428=DIRECTION('',(0.,-1.,0.));
#68429=DIRECTION('',(0.,0.,-1.));
#68430=DIRECTION('',(0.,-1.,0.));
#68431=DIRECTION('center_axis',(0.,1.,0.));
#68432=DIRECTION('ref_axis',(1.,0.,0.));
#68433=DIRECTION('',(1.,0.,0.));
#68434=DIRECTION('',(0.,0.,-1.));
#68435=DIRECTION('',(1.,0.,0.));
#68436=DIRECTION('center_axis',(-1.,0.,0.));
#68437=DIRECTION('ref_axis',(0.,1.,0.));
#68438=DIRECTION('',(0.,1.,0.));
#68439=DIRECTION('',(0.,1.,0.));
#68440=DIRECTION('center_axis',(0.,0.,-1.));
#68441=DIRECTION('ref_axis',(-1.,0.,0.));
#68442=DIRECTION('center_axis',(0.,-1.,0.));
#68443=DIRECTION('ref_axis',(-1.,0.,0.));
#68444=DIRECTION('',(-1.,0.,0.));
#68445=DIRECTION('',(0.,0.,-1.));
#68446=DIRECTION('',(-1.,0.,0.));
#68447=DIRECTION('',(0.,0.,-1.));
#68448=DIRECTION('center_axis',(1.,0.,0.));
#68449=DIRECTION('ref_axis',(0.,-1.,0.));
#68450=DIRECTION('',(0.,-1.,0.));
#68451=DIRECTION('',(0.,0.,-1.));
#68452=DIRECTION('',(0.,-1.,0.));
#68453=DIRECTION('center_axis',(0.,1.,0.));
#68454=DIRECTION('ref_axis',(1.,0.,0.));
#68455=DIRECTION('',(1.,0.,0.));
#68456=DIRECTION('',(0.,0.,-1.));
#68457=DIRECTION('',(1.,0.,0.));
#68458=DIRECTION('center_axis',(-1.,0.,0.));
#68459=DIRECTION('ref_axis',(0.,1.,0.));
#68460=DIRECTION('',(0.,1.,0.));
#68461=DIRECTION('',(0.,1.,0.));
#68462=DIRECTION('center_axis',(0.,0.,-1.));
#68463=DIRECTION('ref_axis',(-1.,0.,0.));
#68464=DIRECTION('center_axis',(0.,-1.,0.));
#68465=DIRECTION('ref_axis',(-1.,0.,0.));
#68466=DIRECTION('',(-1.,0.,0.));
#68467=DIRECTION('',(0.,0.,-1.));
#68468=DIRECTION('',(-1.,0.,0.));
#68469=DIRECTION('',(0.,0.,-1.));
#68470=DIRECTION('center_axis',(1.,0.,0.));
#68471=DIRECTION('ref_axis',(0.,-1.,0.));
#68472=DIRECTION('',(0.,-1.,0.));
#68473=DIRECTION('',(0.,0.,-1.));
#68474=DIRECTION('',(0.,-1.,0.));
#68475=DIRECTION('center_axis',(0.,1.,0.));
#68476=DIRECTION('ref_axis',(1.,0.,0.));
#68477=DIRECTION('',(1.,0.,0.));
#68478=DIRECTION('',(0.,0.,-1.));
#68479=DIRECTION('',(1.,0.,0.));
#68480=DIRECTION('center_axis',(-1.,0.,0.));
#68481=DIRECTION('ref_axis',(0.,1.,0.));
#68482=DIRECTION('',(0.,1.,0.));
#68483=DIRECTION('',(0.,1.,0.));
#68484=DIRECTION('center_axis',(0.,0.,-1.));
#68485=DIRECTION('ref_axis',(-1.,0.,0.));
#68486=DIRECTION('center_axis',(0.,-1.,0.));
#68487=DIRECTION('ref_axis',(-1.,0.,0.));
#68488=DIRECTION('',(-1.,0.,0.));
#68489=DIRECTION('',(0.,0.,-1.));
#68490=DIRECTION('',(-1.,0.,0.));
#68491=DIRECTION('',(0.,0.,-1.));
#68492=DIRECTION('center_axis',(1.,0.,0.));
#68493=DIRECTION('ref_axis',(0.,-1.,0.));
#68494=DIRECTION('',(0.,-1.,0.));
#68495=DIRECTION('',(0.,0.,-1.));
#68496=DIRECTION('',(0.,-1.,0.));
#68497=DIRECTION('center_axis',(0.,1.,0.));
#68498=DIRECTION('ref_axis',(1.,0.,0.));
#68499=DIRECTION('',(1.,0.,0.));
#68500=DIRECTION('',(0.,0.,-1.));
#68501=DIRECTION('',(1.,0.,0.));
#68502=DIRECTION('center_axis',(-1.,0.,0.));
#68503=DIRECTION('ref_axis',(0.,1.,0.));
#68504=DIRECTION('',(0.,1.,0.));
#68505=DIRECTION('',(0.,1.,0.));
#68506=DIRECTION('center_axis',(0.,0.,-1.));
#68507=DIRECTION('ref_axis',(-1.,0.,0.));
#68508=DIRECTION('center_axis',(0.,-1.,0.));
#68509=DIRECTION('ref_axis',(-1.,0.,0.));
#68510=DIRECTION('',(-1.,0.,0.));
#68511=DIRECTION('',(0.,0.,-1.));
#68512=DIRECTION('',(-1.,0.,0.));
#68513=DIRECTION('',(0.,0.,-1.));
#68514=DIRECTION('center_axis',(1.,0.,0.));
#68515=DIRECTION('ref_axis',(0.,-1.,0.));
#68516=DIRECTION('',(0.,-1.,0.));
#68517=DIRECTION('',(0.,0.,-1.));
#68518=DIRECTION('',(0.,-1.,0.));
#68519=DIRECTION('center_axis',(0.,1.,0.));
#68520=DIRECTION('ref_axis',(1.,0.,0.));
#68521=DIRECTION('',(1.,0.,0.));
#68522=DIRECTION('',(0.,0.,-1.));
#68523=DIRECTION('',(1.,0.,0.));
#68524=DIRECTION('center_axis',(-1.,0.,0.));
#68525=DIRECTION('ref_axis',(0.,1.,0.));
#68526=DIRECTION('',(0.,1.,0.));
#68527=DIRECTION('',(0.,1.,0.));
#68528=DIRECTION('center_axis',(0.,0.,-1.));
#68529=DIRECTION('ref_axis',(-1.,0.,0.));
#68530=DIRECTION('center_axis',(0.,-1.,0.));
#68531=DIRECTION('ref_axis',(-1.,0.,0.));
#68532=DIRECTION('',(-1.,0.,0.));
#68533=DIRECTION('',(0.,0.,-1.));
#68534=DIRECTION('',(-1.,0.,0.));
#68535=DIRECTION('',(0.,0.,-1.));
#68536=DIRECTION('center_axis',(1.,0.,0.));
#68537=DIRECTION('ref_axis',(0.,-1.,0.));
#68538=DIRECTION('',(0.,-1.,0.));
#68539=DIRECTION('',(0.,0.,-1.));
#68540=DIRECTION('',(0.,-1.,0.));
#68541=DIRECTION('center_axis',(0.,1.,0.));
#68542=DIRECTION('ref_axis',(1.,0.,0.));
#68543=DIRECTION('',(1.,0.,0.));
#68544=DIRECTION('',(0.,0.,-1.));
#68545=DIRECTION('',(1.,0.,0.));
#68546=DIRECTION('center_axis',(-1.,0.,0.));
#68547=DIRECTION('ref_axis',(0.,1.,0.));
#68548=DIRECTION('',(0.,1.,0.));
#68549=DIRECTION('',(0.,1.,0.));
#68550=DIRECTION('center_axis',(0.,0.,-1.));
#68551=DIRECTION('ref_axis',(-1.,0.,0.));
#68552=DIRECTION('center_axis',(0.,-1.,0.));
#68553=DIRECTION('ref_axis',(-1.,0.,0.));
#68554=DIRECTION('',(-1.,0.,0.));
#68555=DIRECTION('',(0.,0.,-1.));
#68556=DIRECTION('',(-1.,0.,0.));
#68557=DIRECTION('',(0.,0.,-1.));
#68558=DIRECTION('center_axis',(1.,0.,0.));
#68559=DIRECTION('ref_axis',(0.,-1.,0.));
#68560=DIRECTION('',(0.,-1.,0.));
#68561=DIRECTION('',(0.,0.,-1.));
#68562=DIRECTION('',(0.,-1.,0.));
#68563=DIRECTION('center_axis',(0.,1.,0.));
#68564=DIRECTION('ref_axis',(1.,0.,0.));
#68565=DIRECTION('',(1.,0.,0.));
#68566=DIRECTION('',(0.,0.,-1.));
#68567=DIRECTION('',(1.,0.,0.));
#68568=DIRECTION('center_axis',(-1.,0.,0.));
#68569=DIRECTION('ref_axis',(0.,1.,0.));
#68570=DIRECTION('',(0.,1.,0.));
#68571=DIRECTION('',(0.,1.,0.));
#68572=DIRECTION('center_axis',(0.,0.,-1.));
#68573=DIRECTION('ref_axis',(-1.,0.,0.));
#68574=DIRECTION('center_axis',(0.,-1.,0.));
#68575=DIRECTION('ref_axis',(-1.,0.,0.));
#68576=DIRECTION('',(-1.,0.,0.));
#68577=DIRECTION('',(0.,0.,-1.));
#68578=DIRECTION('',(-1.,0.,0.));
#68579=DIRECTION('',(0.,0.,-1.));
#68580=DIRECTION('center_axis',(1.,0.,0.));
#68581=DIRECTION('ref_axis',(0.,-1.,0.));
#68582=DIRECTION('',(0.,-1.,0.));
#68583=DIRECTION('',(0.,0.,-1.));
#68584=DIRECTION('',(0.,-1.,0.));
#68585=DIRECTION('center_axis',(0.,1.,0.));
#68586=DIRECTION('ref_axis',(1.,0.,0.));
#68587=DIRECTION('',(1.,0.,0.));
#68588=DIRECTION('',(0.,0.,-1.));
#68589=DIRECTION('',(1.,0.,0.));
#68590=DIRECTION('center_axis',(-1.,0.,0.));
#68591=DIRECTION('ref_axis',(0.,1.,0.));
#68592=DIRECTION('',(0.,1.,0.));
#68593=DIRECTION('',(0.,1.,0.));
#68594=DIRECTION('center_axis',(0.,0.,-1.));
#68595=DIRECTION('ref_axis',(-1.,0.,0.));
#68596=DIRECTION('center_axis',(0.,-1.,0.));
#68597=DIRECTION('ref_axis',(-1.,0.,0.));
#68598=DIRECTION('',(-1.,0.,0.));
#68599=DIRECTION('',(0.,0.,-1.));
#68600=DIRECTION('',(-1.,0.,0.));
#68601=DIRECTION('',(0.,0.,-1.));
#68602=DIRECTION('center_axis',(1.,0.,0.));
#68603=DIRECTION('ref_axis',(0.,-1.,0.));
#68604=DIRECTION('',(0.,-1.,0.));
#68605=DIRECTION('',(0.,0.,-1.));
#68606=DIRECTION('',(0.,-1.,0.));
#68607=DIRECTION('center_axis',(0.,1.,0.));
#68608=DIRECTION('ref_axis',(1.,0.,0.));
#68609=DIRECTION('',(1.,0.,0.));
#68610=DIRECTION('',(0.,0.,-1.));
#68611=DIRECTION('',(1.,0.,0.));
#68612=DIRECTION('center_axis',(-1.,0.,0.));
#68613=DIRECTION('ref_axis',(0.,1.,0.));
#68614=DIRECTION('',(0.,1.,0.));
#68615=DIRECTION('',(0.,1.,0.));
#68616=DIRECTION('center_axis',(0.,0.,-1.));
#68617=DIRECTION('ref_axis',(-1.,0.,0.));
#68618=DIRECTION('center_axis',(0.,-1.,0.));
#68619=DIRECTION('ref_axis',(-1.,0.,0.));
#68620=DIRECTION('',(-1.,0.,0.));
#68621=DIRECTION('',(0.,0.,-1.));
#68622=DIRECTION('',(-1.,0.,0.));
#68623=DIRECTION('',(0.,0.,-1.));
#68624=DIRECTION('center_axis',(1.,0.,0.));
#68625=DIRECTION('ref_axis',(0.,-1.,0.));
#68626=DIRECTION('',(0.,-1.,0.));
#68627=DIRECTION('',(0.,0.,-1.));
#68628=DIRECTION('',(0.,-1.,0.));
#68629=DIRECTION('center_axis',(0.,1.,0.));
#68630=DIRECTION('ref_axis',(1.,0.,0.));
#68631=DIRECTION('',(1.,0.,0.));
#68632=DIRECTION('',(0.,0.,-1.));
#68633=DIRECTION('',(1.,0.,0.));
#68634=DIRECTION('center_axis',(-1.,0.,0.));
#68635=DIRECTION('ref_axis',(0.,1.,0.));
#68636=DIRECTION('',(0.,1.,0.));
#68637=DIRECTION('',(0.,1.,0.));
#68638=DIRECTION('center_axis',(0.,0.,-1.));
#68639=DIRECTION('ref_axis',(-1.,0.,0.));
#68640=DIRECTION('center_axis',(0.,-1.,0.));
#68641=DIRECTION('ref_axis',(-1.,0.,0.));
#68642=DIRECTION('',(-1.,0.,0.));
#68643=DIRECTION('',(0.,0.,-1.));
#68644=DIRECTION('',(-1.,0.,0.));
#68645=DIRECTION('',(0.,0.,-1.));
#68646=DIRECTION('center_axis',(1.,0.,0.));
#68647=DIRECTION('ref_axis',(0.,-1.,0.));
#68648=DIRECTION('',(0.,-1.,0.));
#68649=DIRECTION('',(0.,0.,-1.));
#68650=DIRECTION('',(0.,-1.,0.));
#68651=DIRECTION('center_axis',(0.,1.,0.));
#68652=DIRECTION('ref_axis',(1.,0.,0.));
#68653=DIRECTION('',(1.,0.,0.));
#68654=DIRECTION('',(0.,0.,-1.));
#68655=DIRECTION('',(1.,0.,0.));
#68656=DIRECTION('center_axis',(-1.,0.,0.));
#68657=DIRECTION('ref_axis',(0.,1.,0.));
#68658=DIRECTION('',(0.,1.,0.));
#68659=DIRECTION('',(0.,1.,0.));
#68660=DIRECTION('center_axis',(0.,0.,-1.));
#68661=DIRECTION('ref_axis',(-1.,0.,0.));
#68662=DIRECTION('center_axis',(0.,-1.,0.));
#68663=DIRECTION('ref_axis',(-1.,0.,0.));
#68664=DIRECTION('',(-1.,0.,0.));
#68665=DIRECTION('',(0.,0.,-1.));
#68666=DIRECTION('',(-1.,0.,0.));
#68667=DIRECTION('',(0.,0.,-1.));
#68668=DIRECTION('center_axis',(1.,0.,0.));
#68669=DIRECTION('ref_axis',(0.,-1.,0.));
#68670=DIRECTION('',(0.,-1.,0.));
#68671=DIRECTION('',(0.,0.,-1.));
#68672=DIRECTION('',(0.,-1.,0.));
#68673=DIRECTION('center_axis',(0.,1.,0.));
#68674=DIRECTION('ref_axis',(1.,0.,0.));
#68675=DIRECTION('',(1.,0.,0.));
#68676=DIRECTION('',(0.,0.,-1.));
#68677=DIRECTION('',(1.,0.,0.));
#68678=DIRECTION('center_axis',(-1.,0.,0.));
#68679=DIRECTION('ref_axis',(0.,1.,0.));
#68680=DIRECTION('',(0.,1.,0.));
#68681=DIRECTION('',(0.,1.,0.));
#68682=DIRECTION('center_axis',(0.,0.,-1.));
#68683=DIRECTION('ref_axis',(-1.,0.,0.));
#68684=DIRECTION('center_axis',(0.,-1.,0.));
#68685=DIRECTION('ref_axis',(-1.,0.,0.));
#68686=DIRECTION('',(-1.,0.,0.));
#68687=DIRECTION('',(0.,0.,-1.));
#68688=DIRECTION('',(-1.,0.,0.));
#68689=DIRECTION('',(0.,0.,-1.));
#68690=DIRECTION('center_axis',(1.,0.,0.));
#68691=DIRECTION('ref_axis',(0.,-1.,0.));
#68692=DIRECTION('',(0.,-1.,0.));
#68693=DIRECTION('',(0.,0.,-1.));
#68694=DIRECTION('',(0.,-1.,0.));
#68695=DIRECTION('center_axis',(0.,1.,0.));
#68696=DIRECTION('ref_axis',(1.,0.,0.));
#68697=DIRECTION('',(1.,0.,0.));
#68698=DIRECTION('',(0.,0.,-1.));
#68699=DIRECTION('',(1.,0.,0.));
#68700=DIRECTION('center_axis',(-1.,0.,0.));
#68701=DIRECTION('ref_axis',(0.,1.,0.));
#68702=DIRECTION('',(0.,1.,0.));
#68703=DIRECTION('',(0.,1.,0.));
#68704=DIRECTION('center_axis',(0.,0.,-1.));
#68705=DIRECTION('ref_axis',(-1.,0.,0.));
#68706=DIRECTION('center_axis',(0.,-1.,0.));
#68707=DIRECTION('ref_axis',(-1.,0.,0.));
#68708=DIRECTION('',(-1.,0.,0.));
#68709=DIRECTION('',(0.,0.,-1.));
#68710=DIRECTION('',(-1.,0.,0.));
#68711=DIRECTION('',(0.,0.,-1.));
#68712=DIRECTION('center_axis',(1.,0.,0.));
#68713=DIRECTION('ref_axis',(0.,-1.,0.));
#68714=DIRECTION('',(0.,-1.,0.));
#68715=DIRECTION('',(0.,0.,-1.));
#68716=DIRECTION('',(0.,-1.,0.));
#68717=DIRECTION('center_axis',(0.,1.,0.));
#68718=DIRECTION('ref_axis',(1.,0.,0.));
#68719=DIRECTION('',(1.,0.,0.));
#68720=DIRECTION('',(0.,0.,-1.));
#68721=DIRECTION('',(1.,0.,0.));
#68722=DIRECTION('center_axis',(-1.,0.,0.));
#68723=DIRECTION('ref_axis',(0.,1.,0.));
#68724=DIRECTION('',(0.,1.,0.));
#68725=DIRECTION('',(0.,1.,0.));
#68726=DIRECTION('center_axis',(0.,0.,-1.));
#68727=DIRECTION('ref_axis',(-1.,0.,0.));
#68728=DIRECTION('center_axis',(0.,-1.,0.));
#68729=DIRECTION('ref_axis',(-1.,0.,0.));
#68730=DIRECTION('',(-1.,0.,0.));
#68731=DIRECTION('',(0.,0.,-1.));
#68732=DIRECTION('',(-1.,0.,0.));
#68733=DIRECTION('',(0.,0.,-1.));
#68734=DIRECTION('center_axis',(1.,0.,0.));
#68735=DIRECTION('ref_axis',(0.,-1.,0.));
#68736=DIRECTION('',(0.,-1.,0.));
#68737=DIRECTION('',(0.,0.,-1.));
#68738=DIRECTION('',(0.,-1.,0.));
#68739=DIRECTION('center_axis',(0.,1.,0.));
#68740=DIRECTION('ref_axis',(1.,0.,0.));
#68741=DIRECTION('',(1.,0.,0.));
#68742=DIRECTION('',(0.,0.,-1.));
#68743=DIRECTION('',(1.,0.,0.));
#68744=DIRECTION('center_axis',(-1.,0.,0.));
#68745=DIRECTION('ref_axis',(0.,1.,0.));
#68746=DIRECTION('',(0.,1.,0.));
#68747=DIRECTION('',(0.,1.,0.));
#68748=DIRECTION('center_axis',(0.,0.,-1.));
#68749=DIRECTION('ref_axis',(-1.,0.,0.));
#68750=DIRECTION('center_axis',(0.,-1.,0.));
#68751=DIRECTION('ref_axis',(-1.,0.,0.));
#68752=DIRECTION('',(-1.,0.,0.));
#68753=DIRECTION('',(0.,0.,-1.));
#68754=DIRECTION('',(-1.,0.,0.));
#68755=DIRECTION('',(0.,0.,-1.));
#68756=DIRECTION('center_axis',(1.,0.,0.));
#68757=DIRECTION('ref_axis',(0.,-1.,0.));
#68758=DIRECTION('',(0.,-1.,0.));
#68759=DIRECTION('',(0.,0.,-1.));
#68760=DIRECTION('',(0.,-1.,0.));
#68761=DIRECTION('center_axis',(0.,1.,0.));
#68762=DIRECTION('ref_axis',(1.,0.,0.));
#68763=DIRECTION('',(1.,0.,0.));
#68764=DIRECTION('',(0.,0.,-1.));
#68765=DIRECTION('',(1.,0.,0.));
#68766=DIRECTION('center_axis',(-1.,0.,0.));
#68767=DIRECTION('ref_axis',(0.,1.,0.));
#68768=DIRECTION('',(0.,1.,0.));
#68769=DIRECTION('',(0.,1.,0.));
#68770=DIRECTION('center_axis',(0.,0.,-1.));
#68771=DIRECTION('ref_axis',(-1.,0.,0.));
#68772=DIRECTION('center_axis',(0.,-1.,0.));
#68773=DIRECTION('ref_axis',(-1.,0.,0.));
#68774=DIRECTION('',(-1.,0.,0.));
#68775=DIRECTION('',(0.,0.,-1.));
#68776=DIRECTION('',(-1.,0.,0.));
#68777=DIRECTION('',(0.,0.,-1.));
#68778=DIRECTION('center_axis',(1.,0.,0.));
#68779=DIRECTION('ref_axis',(0.,-1.,0.));
#68780=DIRECTION('',(0.,-1.,0.));
#68781=DIRECTION('',(0.,0.,-1.));
#68782=DIRECTION('',(0.,-1.,0.));
#68783=DIRECTION('center_axis',(0.,1.,0.));
#68784=DIRECTION('ref_axis',(1.,0.,0.));
#68785=DIRECTION('',(1.,0.,0.));
#68786=DIRECTION('',(0.,0.,-1.));
#68787=DIRECTION('',(1.,0.,0.));
#68788=DIRECTION('center_axis',(-1.,0.,0.));
#68789=DIRECTION('ref_axis',(0.,1.,0.));
#68790=DIRECTION('',(0.,1.,0.));
#68791=DIRECTION('',(0.,1.,0.));
#68792=DIRECTION('center_axis',(0.,0.,-1.));
#68793=DIRECTION('ref_axis',(-1.,0.,0.));
#68794=DIRECTION('center_axis',(0.,-1.,0.));
#68795=DIRECTION('ref_axis',(-1.,0.,0.));
#68796=DIRECTION('',(-1.,0.,0.));
#68797=DIRECTION('',(0.,0.,-1.));
#68798=DIRECTION('',(-1.,0.,0.));
#68799=DIRECTION('',(0.,0.,-1.));
#68800=DIRECTION('center_axis',(1.,0.,0.));
#68801=DIRECTION('ref_axis',(0.,-1.,0.));
#68802=DIRECTION('',(0.,-1.,0.));
#68803=DIRECTION('',(0.,0.,-1.));
#68804=DIRECTION('',(0.,-1.,0.));
#68805=DIRECTION('center_axis',(0.,1.,0.));
#68806=DIRECTION('ref_axis',(1.,0.,0.));
#68807=DIRECTION('',(1.,0.,0.));
#68808=DIRECTION('',(0.,0.,-1.));
#68809=DIRECTION('',(1.,0.,0.));
#68810=DIRECTION('center_axis',(-1.,0.,0.));
#68811=DIRECTION('ref_axis',(0.,1.,0.));
#68812=DIRECTION('',(0.,1.,0.));
#68813=DIRECTION('',(0.,1.,0.));
#68814=DIRECTION('center_axis',(0.,0.,-1.));
#68815=DIRECTION('ref_axis',(-1.,0.,0.));
#68816=DIRECTION('center_axis',(0.,-1.,0.));
#68817=DIRECTION('ref_axis',(-1.,0.,0.));
#68818=DIRECTION('',(-1.,0.,0.));
#68819=DIRECTION('',(0.,0.,-1.));
#68820=DIRECTION('',(-1.,0.,0.));
#68821=DIRECTION('',(0.,0.,-1.));
#68822=DIRECTION('center_axis',(1.,0.,0.));
#68823=DIRECTION('ref_axis',(0.,-1.,0.));
#68824=DIRECTION('',(0.,-1.,0.));
#68825=DIRECTION('',(0.,0.,-1.));
#68826=DIRECTION('',(0.,-1.,0.));
#68827=DIRECTION('center_axis',(0.,1.,0.));
#68828=DIRECTION('ref_axis',(1.,0.,0.));
#68829=DIRECTION('',(1.,0.,0.));
#68830=DIRECTION('',(0.,0.,-1.));
#68831=DIRECTION('',(1.,0.,0.));
#68832=DIRECTION('center_axis',(-1.,0.,0.));
#68833=DIRECTION('ref_axis',(0.,1.,0.));
#68834=DIRECTION('',(0.,1.,0.));
#68835=DIRECTION('',(0.,1.,0.));
#68836=DIRECTION('center_axis',(0.,0.,-1.));
#68837=DIRECTION('ref_axis',(-1.,0.,0.));
#68838=DIRECTION('center_axis',(0.,-1.,0.));
#68839=DIRECTION('ref_axis',(-1.,0.,0.));
#68840=DIRECTION('',(-1.,0.,0.));
#68841=DIRECTION('',(0.,0.,-1.));
#68842=DIRECTION('',(-1.,0.,0.));
#68843=DIRECTION('',(0.,0.,-1.));
#68844=DIRECTION('center_axis',(1.,0.,0.));
#68845=DIRECTION('ref_axis',(0.,-1.,0.));
#68846=DIRECTION('',(0.,-1.,0.));
#68847=DIRECTION('',(0.,0.,-1.));
#68848=DIRECTION('',(0.,-1.,0.));
#68849=DIRECTION('center_axis',(0.,1.,0.));
#68850=DIRECTION('ref_axis',(1.,0.,0.));
#68851=DIRECTION('',(1.,0.,0.));
#68852=DIRECTION('',(0.,0.,-1.));
#68853=DIRECTION('',(1.,0.,0.));
#68854=DIRECTION('center_axis',(-1.,0.,0.));
#68855=DIRECTION('ref_axis',(0.,1.,0.));
#68856=DIRECTION('',(0.,1.,0.));
#68857=DIRECTION('',(0.,1.,0.));
#68858=DIRECTION('center_axis',(0.,0.,-1.));
#68859=DIRECTION('ref_axis',(-1.,0.,0.));
#68860=DIRECTION('center_axis',(0.,-1.,0.));
#68861=DIRECTION('ref_axis',(-1.,0.,0.));
#68862=DIRECTION('',(-1.,0.,0.));
#68863=DIRECTION('',(0.,0.,-1.));
#68864=DIRECTION('',(-1.,0.,0.));
#68865=DIRECTION('',(0.,0.,-1.));
#68866=DIRECTION('center_axis',(1.,0.,0.));
#68867=DIRECTION('ref_axis',(0.,-1.,0.));
#68868=DIRECTION('',(0.,-1.,0.));
#68869=DIRECTION('',(0.,0.,-1.));
#68870=DIRECTION('',(0.,-1.,0.));
#68871=DIRECTION('center_axis',(0.,1.,0.));
#68872=DIRECTION('ref_axis',(1.,0.,0.));
#68873=DIRECTION('',(1.,0.,0.));
#68874=DIRECTION('',(0.,0.,-1.));
#68875=DIRECTION('',(1.,0.,0.));
#68876=DIRECTION('center_axis',(-1.,0.,0.));
#68877=DIRECTION('ref_axis',(0.,1.,0.));
#68878=DIRECTION('',(0.,1.,0.));
#68879=DIRECTION('',(0.,1.,0.));
#68880=DIRECTION('center_axis',(0.,0.,-1.));
#68881=DIRECTION('ref_axis',(-1.,0.,0.));
#68882=DIRECTION('center_axis',(0.,-1.,0.));
#68883=DIRECTION('ref_axis',(-1.,0.,0.));
#68884=DIRECTION('',(-1.,0.,0.));
#68885=DIRECTION('',(0.,0.,-1.));
#68886=DIRECTION('',(-1.,0.,0.));
#68887=DIRECTION('',(0.,0.,-1.));
#68888=DIRECTION('center_axis',(1.,0.,0.));
#68889=DIRECTION('ref_axis',(0.,-1.,0.));
#68890=DIRECTION('',(0.,-1.,0.));
#68891=DIRECTION('',(0.,0.,-1.));
#68892=DIRECTION('',(0.,-1.,0.));
#68893=DIRECTION('center_axis',(0.,1.,0.));
#68894=DIRECTION('ref_axis',(1.,0.,0.));
#68895=DIRECTION('',(1.,0.,0.));
#68896=DIRECTION('',(0.,0.,-1.));
#68897=DIRECTION('',(1.,0.,0.));
#68898=DIRECTION('center_axis',(-1.,0.,0.));
#68899=DIRECTION('ref_axis',(0.,1.,0.));
#68900=DIRECTION('',(0.,1.,0.));
#68901=DIRECTION('',(0.,1.,0.));
#68902=DIRECTION('center_axis',(0.,0.,-1.));
#68903=DIRECTION('ref_axis',(-1.,0.,0.));
#68904=DIRECTION('center_axis',(0.,-1.,0.));
#68905=DIRECTION('ref_axis',(-1.,0.,0.));
#68906=DIRECTION('',(-1.,0.,0.));
#68907=DIRECTION('',(0.,0.,-1.));
#68908=DIRECTION('',(-1.,0.,0.));
#68909=DIRECTION('',(0.,0.,-1.));
#68910=DIRECTION('center_axis',(1.,0.,0.));
#68911=DIRECTION('ref_axis',(0.,-1.,0.));
#68912=DIRECTION('',(0.,-1.,0.));
#68913=DIRECTION('',(0.,0.,-1.));
#68914=DIRECTION('',(0.,-1.,0.));
#68915=DIRECTION('center_axis',(0.,1.,0.));
#68916=DIRECTION('ref_axis',(1.,0.,0.));
#68917=DIRECTION('',(1.,0.,0.));
#68918=DIRECTION('',(0.,0.,-1.));
#68919=DIRECTION('',(1.,0.,0.));
#68920=DIRECTION('center_axis',(-1.,0.,0.));
#68921=DIRECTION('ref_axis',(0.,1.,0.));
#68922=DIRECTION('',(0.,1.,0.));
#68923=DIRECTION('',(0.,1.,0.));
#68924=DIRECTION('center_axis',(0.,0.,-1.));
#68925=DIRECTION('ref_axis',(-1.,0.,0.));
#68926=DIRECTION('center_axis',(0.,-1.,0.));
#68927=DIRECTION('ref_axis',(-1.,0.,0.));
#68928=DIRECTION('',(-1.,0.,0.));
#68929=DIRECTION('',(0.,0.,-1.));
#68930=DIRECTION('',(-1.,0.,0.));
#68931=DIRECTION('',(0.,0.,-1.));
#68932=DIRECTION('center_axis',(1.,0.,0.));
#68933=DIRECTION('ref_axis',(0.,-1.,0.));
#68934=DIRECTION('',(0.,-1.,0.));
#68935=DIRECTION('',(0.,0.,-1.));
#68936=DIRECTION('',(0.,-1.,0.));
#68937=DIRECTION('center_axis',(0.,1.,0.));
#68938=DIRECTION('ref_axis',(1.,0.,0.));
#68939=DIRECTION('',(1.,0.,0.));
#68940=DIRECTION('',(0.,0.,-1.));
#68941=DIRECTION('',(1.,0.,0.));
#68942=DIRECTION('center_axis',(-1.,0.,0.));
#68943=DIRECTION('ref_axis',(0.,1.,0.));
#68944=DIRECTION('',(0.,1.,0.));
#68945=DIRECTION('',(0.,1.,0.));
#68946=DIRECTION('center_axis',(0.,0.,-1.));
#68947=DIRECTION('ref_axis',(-1.,0.,0.));
#68948=DIRECTION('center_axis',(0.,-1.,0.));
#68949=DIRECTION('ref_axis',(-1.,0.,0.));
#68950=DIRECTION('',(-1.,0.,0.));
#68951=DIRECTION('',(0.,0.,-1.));
#68952=DIRECTION('',(-1.,0.,0.));
#68953=DIRECTION('',(0.,0.,-1.));
#68954=DIRECTION('center_axis',(1.,0.,0.));
#68955=DIRECTION('ref_axis',(0.,-1.,0.));
#68956=DIRECTION('',(0.,-1.,0.));
#68957=DIRECTION('',(0.,0.,-1.));
#68958=DIRECTION('',(0.,-1.,0.));
#68959=DIRECTION('center_axis',(0.,1.,0.));
#68960=DIRECTION('ref_axis',(1.,0.,0.));
#68961=DIRECTION('',(1.,0.,0.));
#68962=DIRECTION('',(0.,0.,-1.));
#68963=DIRECTION('',(1.,0.,0.));
#68964=DIRECTION('center_axis',(-1.,0.,0.));
#68965=DIRECTION('ref_axis',(0.,1.,0.));
#68966=DIRECTION('',(0.,1.,0.));
#68967=DIRECTION('',(0.,1.,0.));
#68968=DIRECTION('center_axis',(0.,0.,-1.));
#68969=DIRECTION('ref_axis',(-1.,0.,0.));
#68970=DIRECTION('center_axis',(0.,-1.,0.));
#68971=DIRECTION('ref_axis',(-1.,0.,0.));
#68972=DIRECTION('',(-1.,0.,0.));
#68973=DIRECTION('',(0.,0.,-1.));
#68974=DIRECTION('',(-1.,0.,0.));
#68975=DIRECTION('',(0.,0.,-1.));
#68976=DIRECTION('center_axis',(1.,0.,0.));
#68977=DIRECTION('ref_axis',(0.,-1.,0.));
#68978=DIRECTION('',(0.,-1.,0.));
#68979=DIRECTION('',(0.,0.,-1.));
#68980=DIRECTION('',(0.,-1.,0.));
#68981=DIRECTION('center_axis',(0.,1.,0.));
#68982=DIRECTION('ref_axis',(1.,0.,0.));
#68983=DIRECTION('',(1.,0.,0.));
#68984=DIRECTION('',(0.,0.,-1.));
#68985=DIRECTION('',(1.,0.,0.));
#68986=DIRECTION('center_axis',(-1.,0.,0.));
#68987=DIRECTION('ref_axis',(0.,1.,0.));
#68988=DIRECTION('',(0.,1.,0.));
#68989=DIRECTION('',(0.,1.,0.));
#68990=DIRECTION('center_axis',(0.,0.,-1.));
#68991=DIRECTION('ref_axis',(-1.,0.,0.));
#68992=DIRECTION('center_axis',(0.,0.,-1.));
#68993=DIRECTION('ref_axis',(-1.,0.,0.));
#68994=DIRECTION('',(-0.707106781186561,-0.707106781186534,0.));
#68995=DIRECTION('',(0.,-1.,0.));
#68996=DIRECTION('',(-1.,0.,0.));
#68997=DIRECTION('',(0.,1.,0.));
#68998=DIRECTION('',(-0.707106781186548,0.707106781186548,0.));
#68999=DIRECTION('',(-1.,0.,0.));
#69000=DIRECTION('center_axis',(0.,0.,1.));
#69001=DIRECTION('ref_axis',(1.,0.,0.));
#69002=DIRECTION('',(0.707106781186561,0.707106781186534,0.));
#69003=DIRECTION('',(1.,0.,0.));
#69004=DIRECTION('',(0.707106781186548,-0.707106781186548,0.));
#69005=DIRECTION('',(0.,-1.,0.));
#69006=DIRECTION('',(1.,0.,0.));
#69007=DIRECTION('',(0.,1.,0.));
#69008=DIRECTION('center_axis',(0.,1.,0.));
#69009=DIRECTION('ref_axis',(0.,0.,1.));
#69010=DIRECTION('',(0.,0.,1.));
#69011=DIRECTION('',(0.,0.,-1.));
#69012=DIRECTION('center_axis',(1.,0.,0.));
#69013=DIRECTION('ref_axis',(0.,0.,-1.));
#69014=DIRECTION('',(0.,0.,-1.));
#69015=DIRECTION('',(0.,-0.707106781186542,-0.707106781186553));
#69016=DIRECTION('',(0.,-1.,0.));
#69017=DIRECTION('',(0.,-0.707106781186549,0.707106781186546));
#69018=DIRECTION('',(0.,0.,1.));
#69019=DIRECTION('center_axis',(1.,0.,0.));
#69020=DIRECTION('ref_axis',(0.,0.,-1.));
#69021=DIRECTION('',(0.,-0.866025403784439,-0.499999999999999));
#69022=DIRECTION('',(0.,-0.866025403784432,0.500000000000012));
#69023=DIRECTION('',(0.,0.,1.));
#69024=DIRECTION('',(0.,1.,0.));
#69025=DIRECTION('',(0.,0.,1.));
#69026=DIRECTION('',(0.,-1.,0.));
#69027=DIRECTION('',(0.,0.,1.));
#69028=DIRECTION('',(0.,0.86602540378444,0.499999999999997));
#69029=DIRECTION('',(0.,0.866025403784439,-0.5));
#69030=DIRECTION('center_axis',(1.,0.,0.));
#69031=DIRECTION('ref_axis',(0.,0.,-1.));
#69032=DIRECTION('',(0.,0.,1.));
#69033=DIRECTION('',(0.,0.707106781186548,0.707106781186547));
#69034=DIRECTION('',(0.,1.,0.));
#69035=DIRECTION('',(0.,0.707106781186548,-0.707106781186547));
#69036=DIRECTION('',(0.,0.,-1.));
#69037=DIRECTION('center_axis',(0.707106781186534,-0.707106781186561,0.));
#69038=DIRECTION('ref_axis',(0.,0.,-1.));
#69039=DIRECTION('',(0.,0.,1.));
#69040=DIRECTION('',(-0.678598344545862,-0.678598344545838,0.281084637714804));
#69041=DIRECTION('',(0.,0.,-1.));
#69042=DIRECTION('center_axis',(0.707106781186534,-0.707106781186561,0.));
#69043=DIRECTION('ref_axis',(0.,0.,-1.));
#69044=DIRECTION('',(0.,0.,-1.));
#69045=DIRECTION('',(-0.678598344545863,-0.678598344545837,-0.281084637714805));
#69046=DIRECTION('',(0.,0.,1.));
#69047=DIRECTION('center_axis',(-0.707106781186548,-0.707106781186548,0.));
#69048=DIRECTION('ref_axis',(0.,0.,1.));
#69049=DIRECTION('',(0.,0.,1.));
#69050=DIRECTION('',(0.678598344545849,-0.678598344545849,0.28108463771481));
#69051=DIRECTION('center_axis',(0.,-1.,0.));
#69052=DIRECTION('ref_axis',(0.,0.,-1.));
#69053=DIRECTION('',(1.,0.,0.));
#69054=DIRECTION('center_axis',(0.,-1.,0.));
#69055=DIRECTION('ref_axis',(1.,0.,0.));
#69056=DIRECTION('center_axis',(0.,-1.,0.));
#69057=DIRECTION('ref_axis',(1.,0.,0.));
#69058=DIRECTION('center_axis',(0.,-1.,0.));
#69059=DIRECTION('ref_axis',(1.,0.,0.));
#69060=DIRECTION('center_axis',(0.,1.,0.));
#69061=DIRECTION('ref_axis',(1.,0.,0.));
#69062=DIRECTION('center_axis',(0.,-1.,0.));
#69063=DIRECTION('ref_axis',(1.,0.,0.));
#69064=DIRECTION('',(0.857167300702107,-0.515038074910062,1.04972719113861E-16));
#69065=DIRECTION('center_axis',(0.,1.,0.));
#69066=DIRECTION('ref_axis',(1.,0.,0.));
#69067=DIRECTION('center_axis',(0.,-1.,0.));
#69068=DIRECTION('ref_axis',(1.,0.,0.));
#69069=DIRECTION('',(0.857167300702112,-0.515038074910054,1.04972719113862E-16));
#69070=DIRECTION('center_axis',(0.,-1.,0.));
#69071=DIRECTION('ref_axis',(1.,0.,0.));
#69072=DIRECTION('center_axis',(0.,-1.,0.));
#69073=DIRECTION('ref_axis',(1.,0.,0.));
#69074=DIRECTION('',(0.,-1.,0.));
#69075=DIRECTION('center_axis',(0.,-1.,0.));
#69076=DIRECTION('ref_axis',(1.,0.,0.));
#69077=DIRECTION('center_axis',(0.,-1.,0.));
#69078=DIRECTION('ref_axis',(1.,0.,0.));
#69079=DIRECTION('',(0.,-1.,0.));
#69080=DIRECTION('center_axis',(0.,1.,0.));
#69081=DIRECTION('ref_axis',(1.,0.,0.));
#69082=DIRECTION('center_axis',(0.,1.,0.));
#69083=DIRECTION('ref_axis',(1.,0.,0.));
#69084=DIRECTION('',(0.70710678118654,-0.707106781186555,-8.65956056235483E-17));
#69085=DIRECTION('center_axis',(0.,-1.,0.));
#69086=DIRECTION('ref_axis',(1.,0.,0.));
#69087=DIRECTION('center_axis',(0.,-1.,0.));
#69088=DIRECTION('ref_axis',(1.,0.,0.));
#69089=DIRECTION('',(0.,-1.,0.));
#69090=DIRECTION('center_axis',(0.,-1.,0.));
#69091=DIRECTION('ref_axis',(1.,0.,0.));
#69092=DIRECTION('center_axis',(0.,-1.,0.));
#69093=DIRECTION('ref_axis',(0.,0.,-1.));
#69094=DIRECTION('',(0.,0.,1.));
#69095=DIRECTION('',(1.,0.,0.));
#69096=DIRECTION('',(0.,0.,-1.));
#69097=DIRECTION('',(1.,0.,0.));
#69098=DIRECTION('center_axis',(0.,1.,0.));
#69099=DIRECTION('ref_axis',(1.,0.,0.));
#69100=DIRECTION('center_axis',(0.,1.,0.));
#69101=DIRECTION('ref_axis',(1.,0.,0.));
#69102=DIRECTION('',(0.857167300702117,-0.515038074910047,1.04972719113862E-16));
#69103=DIRECTION('center_axis',(0.,1.,0.));
#69104=DIRECTION('ref_axis',(1.,0.,0.));
#69105=DIRECTION('',(0.707106781186547,-0.707106781186547,-8.65956056235493E-17));
#69106=DIRECTION('center_axis',(0.,-1.,0.));
#69107=DIRECTION('ref_axis',(1.,0.,0.));
#69108=DIRECTION('center_axis',(0.,-1.,0.));
#69109=DIRECTION('ref_axis',(1.,0.,0.));
#69110=DIRECTION('',(0.,-1.,0.));
#69111=DIRECTION('center_axis',(0.,-1.,0.));
#69112=DIRECTION('ref_axis',(1.,0.,0.));
#69113=DIRECTION('center_axis',(0.,1.,0.));
#69114=DIRECTION('ref_axis',(1.,0.,0.));
#69115=DIRECTION('',(0.857167300702112,-0.515038074910054,1.04972719113862E-16));
#69116=DIRECTION('center_axis',(0.,-1.,0.));
#69117=DIRECTION('ref_axis',(1.,0.,0.));
#69118=DIRECTION('center_axis',(0.,-1.,0.));
#69119=DIRECTION('ref_axis',(1.,0.,0.));
#69120=DIRECTION('',(0.,-1.,0.));
#69121=DIRECTION('center_axis',(0.,-1.,0.));
#69122=DIRECTION('ref_axis',(1.,0.,0.));
#69123=DIRECTION('center_axis',(0.,1.,0.));
#69124=DIRECTION('ref_axis',(1.,0.,0.));
#69125=DIRECTION('center_axis',(0.,1.,0.));
#69126=DIRECTION('ref_axis',(1.,0.,0.));
#69127=DIRECTION('center_axis',(0.,-1.,0.));
#69128=DIRECTION('ref_axis',(1.,0.,0.));
#69129=DIRECTION('center_axis',(0.,-1.,0.));
#69130=DIRECTION('ref_axis',(1.,0.,0.));
#69131=DIRECTION('',(0.,-1.,0.));
#69132=DIRECTION('center_axis',(0.,-1.,0.));
#69133=DIRECTION('ref_axis',(1.,0.,0.));
#69134=DIRECTION('center_axis',(0.,1.,0.));
#69135=DIRECTION('ref_axis',(1.,0.,0.));
#69136=DIRECTION('center_axis',(0.,1.,0.));
#69137=DIRECTION('ref_axis',(1.,0.,0.));
#69138=DIRECTION('center_axis',(0.,-1.,0.));
#69139=DIRECTION('ref_axis',(1.,0.,0.));
#69140=DIRECTION('center_axis',(0.,-1.,0.));
#69141=DIRECTION('ref_axis',(1.,0.,0.));
#69142=DIRECTION('',(0.,-1.,0.));
#69143=DIRECTION('center_axis',(0.,-1.,0.));
#69144=DIRECTION('ref_axis',(1.,0.,0.));
#69145=DIRECTION('center_axis',(0.,1.,0.));
#69146=DIRECTION('ref_axis',(1.,0.,0.));
#69147=DIRECTION('center_axis',(0.,1.,0.));
#69148=DIRECTION('ref_axis',(1.,0.,0.));
#69149=DIRECTION('center_axis',(0.,-1.,0.));
#69150=DIRECTION('ref_axis',(1.,0.,0.));
#69151=DIRECTION('center_axis',(0.,-1.,0.));
#69152=DIRECTION('ref_axis',(1.,0.,0.));
#69153=DIRECTION('',(0.,-1.,0.));
#69154=DIRECTION('center_axis',(0.,-1.,0.));
#69155=DIRECTION('ref_axis',(1.,0.,0.));
#69156=DIRECTION('center_axis',(0.,1.,0.));
#69157=DIRECTION('ref_axis',(1.,0.,0.));
#69158=DIRECTION('center_axis',(0.,1.,0.));
#69159=DIRECTION('ref_axis',(1.,0.,0.));
#69160=DIRECTION('center_axis',(0.,-1.,0.));
#69161=DIRECTION('ref_axis',(1.,0.,0.));
#69162=DIRECTION('center_axis',(0.,-1.,0.));
#69163=DIRECTION('ref_axis',(1.,0.,0.));
#69164=DIRECTION('',(0.,-1.,0.));
#69165=DIRECTION('center_axis',(0.,-1.,0.));
#69166=DIRECTION('ref_axis',(1.,0.,0.));
#69167=DIRECTION('center_axis',(0.,1.,0.));
#69168=DIRECTION('ref_axis',(1.,0.,0.));
#69169=DIRECTION('center_axis',(0.,1.,0.));
#69170=DIRECTION('ref_axis',(1.,0.,0.));
#69171=DIRECTION('center_axis',(0.,-1.,0.));
#69172=DIRECTION('ref_axis',(1.,0.,0.));
#69173=DIRECTION('center_axis',(0.,-1.,0.));
#69174=DIRECTION('ref_axis',(1.,0.,0.));
#69175=DIRECTION('',(0.,-1.,0.));
#69176=DIRECTION('center_axis',(0.,-1.,0.));
#69177=DIRECTION('ref_axis',(1.,0.,0.));
#69178=DIRECTION('center_axis',(0.,1.,0.));
#69179=DIRECTION('ref_axis',(1.,0.,0.));
#69180=DIRECTION('center_axis',(0.,1.,0.));
#69181=DIRECTION('ref_axis',(1.,0.,0.));
#69182=DIRECTION('center_axis',(0.,-1.,0.));
#69183=DIRECTION('ref_axis',(1.,0.,0.));
#69184=DIRECTION('',(0.707106781186561,0.707106781186534,8.6595605623551E-17));
#69185=DIRECTION('center_axis',(0.,1.,0.));
#69186=DIRECTION('ref_axis',(1.,0.,0.));
#69187=DIRECTION('center_axis',(0.,-1.,0.));
#69188=DIRECTION('ref_axis',(0.,0.,-1.));
#69189=DIRECTION('',(0.,0.,1.));
#69190=DIRECTION('',(-1.,0.,0.));
#69191=DIRECTION('center_axis',(0.,-1.,0.));
#69192=DIRECTION('ref_axis',(1.,0.,0.));
#69193=DIRECTION('center_axis',(0.,-1.,0.));
#69194=DIRECTION('ref_axis',(1.,0.,0.));
#69195=DIRECTION('center_axis',(0.,-1.,0.));
#69196=DIRECTION('ref_axis',(1.,0.,0.));
#69197=DIRECTION('center_axis',(0.,1.,0.));
#69198=DIRECTION('ref_axis',(1.,0.,0.));
#69199=DIRECTION('',(0.,1.,0.));
#69200=DIRECTION('center_axis',(0.,-1.,0.));
#69201=DIRECTION('ref_axis',(1.,0.,0.));
#69202=DIRECTION('',(0.70710678118654,0.707106781186555,8.65956056235484E-17));
#69203=DIRECTION('center_axis',(0.,1.,0.));
#69204=DIRECTION('ref_axis',(1.,0.,0.));
#69205=DIRECTION('center_axis',(0.,1.,0.));
#69206=DIRECTION('ref_axis',(1.,0.,0.));
#69207=DIRECTION('',(0.,1.,0.));
#69208=DIRECTION('center_axis',(0.,-1.,0.));
#69209=DIRECTION('ref_axis',(1.,0.,0.));
#69210=DIRECTION('',(0.70710678118654,0.707106781186555,8.65956056235484E-17));
#69211=DIRECTION('center_axis',(0.,1.,0.));
#69212=DIRECTION('ref_axis',(1.,0.,0.));
#69213=DIRECTION('center_axis',(0.,1.,0.));
#69214=DIRECTION('ref_axis',(1.,0.,0.));
#69215=DIRECTION('',(0.,1.,0.));
#69216=DIRECTION('center_axis',(0.,-1.,0.));
#69217=DIRECTION('ref_axis',(1.,0.,0.));
#69218=DIRECTION('',(0.707106781186545,0.70710678118655,8.6595605623549E-17));
#69219=DIRECTION('center_axis',(0.,1.,0.));
#69220=DIRECTION('ref_axis',(1.,0.,0.));
#69221=DIRECTION('center_axis',(0.,1.,0.));
#69222=DIRECTION('ref_axis',(1.,0.,0.));
#69223=DIRECTION('',(0.,1.,0.));
#69224=DIRECTION('center_axis',(0.,-1.,0.));
#69225=DIRECTION('ref_axis',(1.,0.,0.));
#69226=DIRECTION('',(0.707106781186545,0.70710678118655,8.6595605623549E-17));
#69227=DIRECTION('center_axis',(0.,1.,0.));
#69228=DIRECTION('ref_axis',(1.,0.,0.));
#69229=DIRECTION('center_axis',(0.,1.,0.));
#69230=DIRECTION('ref_axis',(1.,0.,0.));
#69231=DIRECTION('',(0.,1.,0.));
#69232=DIRECTION('center_axis',(0.,-1.,0.));
#69233=DIRECTION('ref_axis',(1.,0.,0.));
#69234=DIRECTION('',(0.707106781186561,0.707106781186534,8.6595605623551E-17));
#69235=DIRECTION('center_axis',(0.,1.,0.));
#69236=DIRECTION('ref_axis',(1.,0.,0.));
#69237=DIRECTION('center_axis',(0.,1.,0.));
#69238=DIRECTION('ref_axis',(1.,0.,0.));
#69239=DIRECTION('',(0.,1.,0.));
#69240=DIRECTION('center_axis',(0.70710678118653,-0.353553390593282,0.61237243569581));
#69241=DIRECTION('ref_axis',(0.654653670707996,0.,-0.755928946018439));
#69242=DIRECTION('',(0.,-0.866025403784439,-0.499999999999999));
#69243=DIRECTION('center_axis',(-0.70710678118653,0.353553390593282,-0.61237243569581));
#69244=DIRECTION('ref_axis',(0.707106781186565,0.353553390593265,-0.61237243569578));
#69245=DIRECTION('',(0.,0.866025403784439,0.499999999999999));
#69246=DIRECTION('',(-0.654653670707999,-1.45362315675074E-14,0.755928946018435));
#69247=DIRECTION('center_axis',(0.707106781186532,0.35355339059329,0.612372435695804));
#69248=DIRECTION('ref_axis',(0.654653670707991,0.,-0.755928946018442));
#69249=DIRECTION('',(0.,0.866025403784432,-0.500000000000012));
#69250=DIRECTION('',(-0.654653670708,0.654653670707976,0.377964473009189));
#69251=DIRECTION('',(0.,-0.866025403784432,0.500000000000012));
#69252=DIRECTION('center_axis',(0.707106781186534,0.707106781186561,0.));
#69253=DIRECTION('ref_axis',(0.,0.,-1.));
#69254=DIRECTION('',(0.,0.,-1.));
#69255=DIRECTION('',(-0.577350269189639,0.577350269189617,-0.577350269189622));
#69256=DIRECTION('',(0.,0.,1.));
#69257=DIRECTION('center_axis',(0.707106781186532,0.,0.707106781186563));
#69258=DIRECTION('ref_axis',(0.707106781186563,0.,-0.707106781186532));
#69259=DIRECTION('',(0.,1.,0.));
#69260=DIRECTION('',(-0.577350269189641,0.57735026918962,0.577350269189616));
#69261=DIRECTION('',(0.,-1.,0.));
#69262=DIRECTION('',(0.577350269189641,-0.57735026918962,-0.577350269189616));
#69263=DIRECTION('center_axis',(0.707106781186534,0.707106781186561,0.));
#69264=DIRECTION('ref_axis',(0.,0.,-1.));
#69265=DIRECTION('',(0.,0.,-1.));
#69266=DIRECTION('',(-0.654653670707992,0.654653670707968,-0.377964473009218));
#69267=DIRECTION('',(0.,0.,1.));
#69268=DIRECTION('center_axis',(0.707106781186533,0.353553390593279,-0.612372435695809));
#69269=DIRECTION('ref_axis',(-0.654653670707994,0.,-0.75592894601844));
#69270=DIRECTION('',(0.,-0.86602540378444,-0.499999999999997));
#69271=DIRECTION('',(-0.654653670707994,-4.84541052250242E-15,-0.75592894601844));
#69272=DIRECTION('',(0.,0.86602540378444,0.499999999999997));
#69273=DIRECTION('center_axis',(0.707106781186535,-0.35355339059328,-0.612372435695805));
#69274=DIRECTION('ref_axis',(-0.65465367070799,0.,-0.755928946018443));
#69275=DIRECTION('',(0.,-0.866025403784439,0.5));
#69276=DIRECTION('center_axis',(-0.707106781186535,0.35355339059328,0.612372435695805));
#69277=DIRECTION('ref_axis',(-0.70710678118656,-0.353553390593267,-0.612372435695784));
#69278=DIRECTION('',(0.,0.866025403784439,-0.5));
#69279=DIRECTION('center_axis',(0.707106781186534,0.707106781186561,0.));
#69280=DIRECTION('ref_axis',(0.,0.,-1.));
#69281=DIRECTION('',(0.,0.,-1.));
#69282=DIRECTION('',(0.577350269189639,-0.577350269189617,0.577350269189622));
#69283=DIRECTION('center_axis',(0.707106781186537,0.,-0.707106781186558));
#69284=DIRECTION('ref_axis',(-0.707106781186558,0.,-0.707106781186537));
#69285=DIRECTION('',(0.,-1.,0.));
#69286=DIRECTION('',(0.,1.,0.));
#69287=DIRECTION('center_axis',(1.,0.,0.));
#69288=DIRECTION('ref_axis',(0.,0.,-1.));
#69289=DIRECTION('',(1.,0.,0.));
#69290=DIRECTION('center_axis',(0.707106781186544,0.353553390593275,-0.612372435695798));
#69291=DIRECTION('ref_axis',(-0.707106781186551,0.353553390593271,-0.612372435695791));
#69292=DIRECTION('center_axis',(0.707106781186548,-0.707106781186547,0.));
#69293=DIRECTION('ref_axis',(0.707106781186547,0.707106781186548,0.));
#69294=DIRECTION('',(-1.,0.,0.));
#69295=DIRECTION('center_axis',(-0.707106781186534,-0.707106781186561,0.));
#69296=DIRECTION('ref_axis',(-0.707106781186561,0.707106781186534,0.));
#69297=DIRECTION('center_axis',(-1.,0.,0.));
#69298=DIRECTION('ref_axis',(0.,0.,-1.));
#69299=DIRECTION('center_axis',(0.,-0.499999999999999,0.866025403784439));
#69300=DIRECTION('ref_axis',(0.,-0.866025403784439,-0.499999999999999));
#69301=DIRECTION('',(1.,0.,0.));
#69302=DIRECTION('',(0.,0.866025403784439,0.499999999999999));
#69303=DIRECTION('center_axis',(0.,0.500000000000012,0.866025403784432));
#69304=DIRECTION('ref_axis',(1.,0.,0.));
#69305=DIRECTION('',(-1.,0.,0.));
#69306=DIRECTION('',(0.,0.866025403784432,-0.500000000000012));
#69307=DIRECTION('center_axis',(0.,1.,0.));
#69308=DIRECTION('ref_axis',(0.,0.,1.));
#69309=DIRECTION('',(-1.,0.,0.));
#69310=DIRECTION('',(0.,0.,-1.));
#69311=DIRECTION('center_axis',(0.,0.,1.));
#69312=DIRECTION('ref_axis',(0.,-1.,0.));
#69313=DIRECTION('',(0.,-1.,0.));
#69314=DIRECTION('center_axis',(0.,0.,-1.));
#69315=DIRECTION('ref_axis',(0.,1.,0.));
#69316=DIRECTION('',(1.,0.,0.));
#69317=DIRECTION('',(0.,1.,0.));
#69318=DIRECTION('center_axis',(0.707106781186534,0.707106781186561,0.));
#69319=DIRECTION('ref_axis',(0.,0.,-1.));
#69320=DIRECTION('',(0.,0.,1.));
#69321=DIRECTION('center_axis',(-0.707106781186534,-0.707106781186561,0.));
#69322=DIRECTION('ref_axis',(-0.707106781186561,0.707106781186534,0.));
#69323=DIRECTION('',(0.,0.,-1.));
#69324=DIRECTION('',(-0.678598344545864,0.678598344545836,-0.281084637714807));
#69325=DIRECTION('center_axis',(0.707106781186528,0.500000000000013,-0.500000000000014));
#69326=DIRECTION('ref_axis',(-0.577350269189647,0.,-0.816496580927711));
#69327=DIRECTION('',(0.,-0.707106781186548,-0.707106781186547));
#69328=DIRECTION('',(-0.678598344545863,0.281084637714805,-0.678598344545838));
#69329=DIRECTION('',(0.,0.707106781186548,0.707106781186547));
#69330=DIRECTION('center_axis',(0.707106781186534,0.,-0.707106781186561));
#69331=DIRECTION('ref_axis',(-0.707106781186561,0.,-0.707106781186534));
#69332=DIRECTION('',(0.,-1.,0.));
#69333=DIRECTION('',(-0.678598344545862,-0.281084637714807,-0.678598344545837));
#69334=DIRECTION('',(0.,1.,0.));
#69335=DIRECTION('center_axis',(0.707106781186531,-0.500000000000011,-0.500000000000012));
#69336=DIRECTION('ref_axis',(-0.577350269189644,0.,-0.816496580927713));
#69337=DIRECTION('',(0.,-0.707106781186548,0.707106781186547));
#69338=DIRECTION('',(0.,0.707106781186548,-0.707106781186547));
#69339=DIRECTION('center_axis',(0.70710678118653,-0.500000000000016,0.500000000000009));
#69340=DIRECTION('ref_axis',(0.577350269189642,0.,-0.816496580927714));
#69341=DIRECTION('',(0.,0.707106781186542,0.707106781186553));
#69342=DIRECTION('',(-0.678598344545859,-0.281084637714809,0.678598344545839));
#69343=DIRECTION('',(0.,-0.707106781186542,-0.707106781186553));
#69344=DIRECTION('center_axis',(0.707106781186537,0.,0.707106781186558));
#69345=DIRECTION('ref_axis',(0.707106781186558,0.,-0.707106781186537));
#69346=DIRECTION('',(0.,1.,0.));
#69347=DIRECTION('',(-0.678598344545856,0.281084637714825,0.678598344545836));
#69348=DIRECTION('',(0.,-1.,0.));
#69349=DIRECTION('center_axis',(0.707106781186538,0.500000000000006,0.500000000000008));
#69350=DIRECTION('ref_axis',(0.577350269189637,0.,-0.816496580927718));
#69351=DIRECTION('',(0.,0.707106781186549,-0.707106781186546));
#69352=DIRECTION('',(-0.678598344545859,0.678598344545834,0.281084637714823));
#69353=DIRECTION('',(0.,-0.707106781186549,0.707106781186546));
#69354=DIRECTION('center_axis',(0.707106781186534,0.707106781186561,0.));
#69355=DIRECTION('ref_axis',(0.,0.,-1.));
#69356=DIRECTION('',(0.,0.,-1.));
#69357=DIRECTION('',(0.,0.,1.));
#69358=DIRECTION('center_axis',(0.,1.,0.));
#69359=DIRECTION('ref_axis',(0.,0.,1.));
#69360=DIRECTION('',(1.,0.,0.));
#69361=DIRECTION('',(0.,0.,-1.));
#69362=DIRECTION('',(1.,0.,0.));
#69363=DIRECTION('center_axis',(0.,0.707106781186547,-0.707106781186548));
#69364=DIRECTION('ref_axis',(-1.,0.,0.));
#69365=DIRECTION('',(-1.,0.,0.));
#69366=DIRECTION('',(0.,-0.707106781186548,-0.707106781186547));
#69367=DIRECTION('center_axis',(0.,0.,-1.));
#69368=DIRECTION('ref_axis',(0.,1.,0.));
#69369=DIRECTION('',(1.,0.,0.));
#69370=DIRECTION('',(0.,-1.,0.));
#69371=DIRECTION('center_axis',(0.,-0.707106781186547,-0.707106781186548));
#69372=DIRECTION('ref_axis',(-1.,0.,0.));
#69373=DIRECTION('',(0.,-0.707106781186548,0.707106781186547));
#69374=DIRECTION('center_axis',(0.,-0.707106781186553,0.707106781186542));
#69375=DIRECTION('ref_axis',(1.,0.,0.));
#69376=DIRECTION('',(-1.,0.,0.));
#69377=DIRECTION('',(0.,0.707106781186542,0.707106781186553));
#69378=DIRECTION('center_axis',(0.,0.,1.));
#69379=DIRECTION('ref_axis',(0.,-1.,0.));
#69380=DIRECTION('',(1.,0.,0.));
#69381=DIRECTION('',(0.,1.,0.));
#69382=DIRECTION('center_axis',(0.,0.707106781186546,0.707106781186549));
#69383=DIRECTION('ref_axis',(1.,0.,0.));
#69384=DIRECTION('',(-1.,0.,0.));
#69385=DIRECTION('',(0.,0.707106781186549,-0.707106781186546));
#69386=DIRECTION('center_axis',(0.,1.,0.));
#69387=DIRECTION('ref_axis',(0.,0.,1.));
#69388=DIRECTION('',(0.,0.,-1.));
#69389=DIRECTION('center_axis',(-0.707106781186549,-0.353553390593273,-0.612372435695794));
#69390=DIRECTION('ref_axis',(-0.654653670707976,0.,0.755928946018455));
#69391=DIRECTION('',(0.,-0.866025403784439,0.5));
#69392=DIRECTION('center_axis',(0.707106781186549,0.353553390593273,0.612372435695794));
#69393=DIRECTION('ref_axis',(0.707106781186546,-0.353553390593274,-0.612372435695796));
#69394=DIRECTION('',(0.65465367070798,-4.8454105225025E-15,-0.755928946018452));
#69395=DIRECTION('center_axis',(-0.707106781186546,0.353553390593272,-0.612372435695797));
#69396=DIRECTION('ref_axis',(-0.65465367070798,0.,0.755928946018452));
#69397=DIRECTION('',(0.654653670707978,0.654653670707978,-0.377964473009224));
#69398=DIRECTION('',(0.,-0.86602540378444,-0.499999999999997));
#69399=DIRECTION('center_axis',(-0.707106781186548,0.707106781186547,0.));
#69400=DIRECTION('ref_axis',(0.,0.,1.));
#69401=DIRECTION('',(0.577350269189627,0.577350269189627,0.577350269189623));
#69402=DIRECTION('',(0.,0.,-1.));
#69403=DIRECTION('center_axis',(-0.707106781186545,0.,0.70710678118655));
#69404=DIRECTION('ref_axis',(0.70710678118655,0.,0.707106781186545));
#69405=DIRECTION('',(0.577350269189627,0.577350269189627,0.577350269189623));
#69406=DIRECTION('center_axis',(-0.707106781186548,0.707106781186547,0.));
#69407=DIRECTION('ref_axis',(0.,0.,1.));
#69408=DIRECTION('',(0.577350269189624,0.577350269189625,-0.577350269189629));
#69409=DIRECTION('center_axis',(-0.70710678118655,0.,-0.707106781186545));
#69410=DIRECTION('ref_axis',(-0.707106781186545,0.,0.70710678118655));
#69411=DIRECTION('',(0.577350269189624,0.577350269189625,-0.577350269189629));
#69412=DIRECTION('center_axis',(-0.707106781186548,0.707106781186547,0.));
#69413=DIRECTION('ref_axis',(0.,0.,1.));
#69414=DIRECTION('',(0.654653670707986,0.654653670707987,0.377964473009195));
#69415=DIRECTION('center_axis',(-0.707106781186545,0.353553390593283,0.612372435695792));
#69416=DIRECTION('ref_axis',(0.654653670707977,0.,0.755928946018455));
#69417=DIRECTION('',(0.654653670707985,-1.45362315675076E-14,0.755928946018448));
#69418=DIRECTION('center_axis',(-0.707106781186544,-0.353553390593275,0.612372435695798));
#69419=DIRECTION('ref_axis',(0.654653670707981,0.,0.755928946018451));
#69420=DIRECTION('center_axis',(-0.707106781186548,0.707106781186547,0.));
#69421=DIRECTION('ref_axis',(0.,0.,1.));
#69422=DIRECTION('',(0.678598344545843,0.678598344545848,0.281084637714827));
#69423=DIRECTION('center_axis',(-0.707106781186551,0.499999999999997,0.499999999999999));
#69424=DIRECTION('ref_axis',(0.577350269189623,0.,0.816496580927728));
#69425=DIRECTION('',(0.678598344545843,0.281084637714827,0.678598344545848));
#69426=DIRECTION('center_axis',(-0.70710678118655,0.,0.707106781186545));
#69427=DIRECTION('ref_axis',(0.707106781186545,0.,0.70710678118655));
#69428=DIRECTION('',(0.678598344545845,-0.281084637714814,0.678598344545851));
#69429=DIRECTION('center_axis',(-0.707106781186543,-0.500000000000007,0.5));
#69430=DIRECTION('ref_axis',(0.577350269189628,0.,0.816496580927724));
#69431=DIRECTION('center_axis',(-0.707106781186548,-0.707106781186548,0.));
#69432=DIRECTION('ref_axis',(0.,0.,1.));
#69433=DIRECTION('',(0.678598344545846,-0.678598344545855,-0.281084637714803));
#69434=DIRECTION('center_axis',(-0.707106781186544,-0.500000000000002,-0.500000000000003));
#69435=DIRECTION('ref_axis',(-0.57735026918963,0.,0.816496580927723));
#69436=DIRECTION('',(0.678598344545849,-0.281084637714812,-0.678598344545849));
#69437=DIRECTION('center_axis',(-0.707106781186548,0.,-0.707106781186547));
#69438=DIRECTION('ref_axis',(-0.707106781186547,0.,0.707106781186548));
#69439=DIRECTION('',(0.678598344545848,0.281084637714809,-0.678598344545851));
#69440=DIRECTION('center_axis',(-0.707106781186542,0.500000000000004,-0.500000000000005));
#69441=DIRECTION('ref_axis',(-0.577350269189633,0.,0.816496580927721));
#69442=DIRECTION('',(0.678598344545849,0.67859834454585,-0.28108463771481));
#69443=DIRECTION('center_axis',(-0.707106781186548,0.707106781186547,0.));
#69444=DIRECTION('ref_axis',(0.,0.,1.));
#69445=DIRECTION('center_axis',(0.707106781186548,-0.707106781186547,0.));
#69446=DIRECTION('ref_axis',(0.707106781186547,0.707106781186548,0.));
#69447=DIRECTION('center_axis',(1.,0.,0.));
#69448=DIRECTION('ref_axis',(0.,0.,-1.));
#69449=DIRECTION('center_axis',(-1.,0.,0.));
#69450=DIRECTION('ref_axis',(0.,0.,-1.));
#69451=DIRECTION('center_axis',(0.,1.,0.));
#69452=DIRECTION('ref_axis',(0.,0.,1.));
#69453=DIRECTION('',(1.,0.,0.));
#69454=DIRECTION('center_axis',(1.,0.,0.));
#69455=DIRECTION('ref_axis',(0.,-0.500000000000001,0.866025403784438));
#69456=DIRECTION('',(-1.,0.,0.));
#69457=DIRECTION('center_axis',(0.,0.499999999999997,-0.86602540378444));
#69458=DIRECTION('ref_axis',(-1.,0.,0.));
#69459=DIRECTION('',(-1.,0.,0.));
#69460=DIRECTION('center_axis',(0.,-0.5,-0.866025403784439));
#69461=DIRECTION('ref_axis',(0.,0.866025403784439,-0.5));
#76145=CARTESIAN_POINT('',(0.,0.,0.));
#76146=CARTESIAN_POINT('Ctrl Pts',(200.85163737461,3.38540250062943,48.5));
#76147=CARTESIAN_POINT('Ctrl Pts',(200.85163737461,3.38540250062943,48.35));
#76148=CARTESIAN_POINT('Ctrl Pts',(200.665552567691,3.38540250062943,48.5));
#76149=CARTESIAN_POINT('Ctrl Pts',(200.665552567691,3.38540250062943,48.35));
#76150=CARTESIAN_POINT('Ctrl Pts',(200.55450225994,3.22783091664314,48.5));
#76151=CARTESIAN_POINT('Ctrl Pts',(200.55450225994,3.22783091664314,48.35));
#76152=CARTESIAN_POINT('',(200.85163737461,3.38540250062943,48.5));
#76153=CARTESIAN_POINT('',(200.55450225994,3.22783091664314,48.5));
#76154=CARTESIAN_POINT('Ctrl Pts',(200.85163737461,3.38540250062943,48.5));
#76155=CARTESIAN_POINT('Ctrl Pts',(200.665552567691,3.38540250062943,48.5));
#76156=CARTESIAN_POINT('Ctrl Pts',(200.55450225994,3.22783091664314,48.5));
#76157=CARTESIAN_POINT('',(200.85163737461,3.38540250062943,48.35));
#76158=CARTESIAN_POINT('',(200.85163737461,3.38540250062943,48.5));
#76159=CARTESIAN_POINT('',(200.55450225994,3.22783091664314,48.35));
#76160=CARTESIAN_POINT('Ctrl Pts',(200.85163737461,3.38540250062943,48.35));
#76161=CARTESIAN_POINT('Ctrl Pts',(200.665552567691,3.38540250062943,48.35));
#76162=CARTESIAN_POINT('Ctrl Pts',(200.55450225994,3.22783091664314,48.35));
#76163=CARTESIAN_POINT('',(200.55450225994,3.22783091664314,48.5));
#76164=CARTESIAN_POINT('Ctrl Pts',(201.167530667037,3.2068213224411,48.5));
#76165=CARTESIAN_POINT('Ctrl Pts',(201.167530667037,3.2068213224411,48.35));
#76166=CARTESIAN_POINT('Ctrl Pts',(201.04072297737,3.38540250062943,48.5));
#76167=CARTESIAN_POINT('Ctrl Pts',(201.04072297737,3.38540250062943,48.35));
#76168=CARTESIAN_POINT('Ctrl Pts',(200.85163737461,3.38540250062943,48.5));
#76169=CARTESIAN_POINT('Ctrl Pts',(200.85163737461,3.38540250062943,48.35));
#76170=CARTESIAN_POINT('',(201.167530667037,3.2068213224411,48.5));
#76171=CARTESIAN_POINT('Ctrl Pts',(201.167530667037,3.2068213224411,48.5));
#76172=CARTESIAN_POINT('Ctrl Pts',(201.04072297737,3.38540250062943,48.5));
#76173=CARTESIAN_POINT('Ctrl Pts',(200.85163737461,3.38540250062943,48.5));
#76174=CARTESIAN_POINT('',(201.167530667037,3.2068213224411,48.35));
#76175=CARTESIAN_POINT('',(201.167530667037,3.2068213224411,48.5));
#76176=CARTESIAN_POINT('Ctrl Pts',(201.167530667037,3.2068213224411,48.35));
#76177=CARTESIAN_POINT('Ctrl Pts',(201.04072297737,3.38540250062943,48.35));
#76178=CARTESIAN_POINT('Ctrl Pts',(200.85163737461,3.38540250062943,48.35));
#76179=CARTESIAN_POINT('Ctrl Pts',(201.294338356704,2.48499327898026,48.5));
#76180=CARTESIAN_POINT('Ctrl Pts',(201.294338356704,2.48499327898026,48.35));
#76181=CARTESIAN_POINT('Ctrl Pts',(201.294338356704,3.02824014425278,48.5));
#76182=CARTESIAN_POINT('Ctrl Pts',(201.294338356704,3.02824014425278,48.35));
#76183=CARTESIAN_POINT('Ctrl Pts',(201.167530667037,3.2068213224411,48.5));
#76184=CARTESIAN_POINT('Ctrl Pts',(201.167530667037,3.2068213224411,48.35));
#76185=CARTESIAN_POINT('',(201.294338356704,2.48499327898026,48.5));
#76186=CARTESIAN_POINT('Ctrl Pts',(201.294338356704,2.48499327898026,48.5));
#76187=CARTESIAN_POINT('Ctrl Pts',(201.294338356704,3.02824014425278,48.5));
#76188=CARTESIAN_POINT('Ctrl Pts',(201.167530667037,3.2068213224411,48.5));
#76189=CARTESIAN_POINT('',(201.294338356704,2.48499327898026,48.35));
#76190=CARTESIAN_POINT('',(201.294338356704,2.48499327898026,48.5));
#76191=CARTESIAN_POINT('Ctrl Pts',(201.294338356704,2.48499327898026,48.35));
#76192=CARTESIAN_POINT('Ctrl Pts',(201.294338356704,3.02824014425278,48.35));
#76193=CARTESIAN_POINT('Ctrl Pts',(201.167530667037,3.2068213224411,48.35));
#76194=CARTESIAN_POINT('Ctrl Pts',(201.167530667037,1.76466578245163,48.5));
#76195=CARTESIAN_POINT('Ctrl Pts',(201.167530667037,1.76466578245163,48.35));
#76196=CARTESIAN_POINT('Ctrl Pts',(201.294338356704,1.9447478055954,48.5));
#76197=CARTESIAN_POINT('Ctrl Pts',(201.294338356704,1.9447478055954,48.35));
#76198=CARTESIAN_POINT('Ctrl Pts',(201.294338356704,2.48499327898026,48.5));
#76199=CARTESIAN_POINT('Ctrl Pts',(201.294338356704,2.48499327898026,48.35));
#76200=CARTESIAN_POINT('',(201.167530667037,1.76466578245163,48.5));
#76201=CARTESIAN_POINT('Ctrl Pts',(201.167530667037,1.76466578245163,48.5));
#76202=CARTESIAN_POINT('Ctrl Pts',(201.294338356704,1.9447478055954,48.5));
#76203=CARTESIAN_POINT('Ctrl Pts',(201.294338356704,2.48499327898026,48.5));
#76204=CARTESIAN_POINT('',(201.167530667037,1.76466578245163,48.35));
#76205=CARTESIAN_POINT('',(201.167530667037,1.76466578245163,48.5));
#76206=CARTESIAN_POINT('Ctrl Pts',(201.167530667037,1.76466578245163,48.35));
#76207=CARTESIAN_POINT('Ctrl Pts',(201.294338356704,1.9447478055954,48.35));
#76208=CARTESIAN_POINT('Ctrl Pts',(201.294338356704,2.48499327898026,48.35));
#76209=CARTESIAN_POINT('Ctrl Pts',(200.854638468474,1.58458405733109,48.5));
#76210=CARTESIAN_POINT('Ctrl Pts',(200.854638468474,1.58458405733109,48.35));
#76211=CARTESIAN_POINT('Ctrl Pts',(201.04072297737,1.58458405733109,48.5));
#76212=CARTESIAN_POINT('Ctrl Pts',(201.04072297737,1.58458405733109,48.35));
#76213=CARTESIAN_POINT('Ctrl Pts',(201.167530667037,1.76466578245163,48.5));
#76214=CARTESIAN_POINT('Ctrl Pts',(201.167530667037,1.76466578245163,48.35));
#76215=CARTESIAN_POINT('',(200.854638468474,1.58458405733109,48.5));
#76216=CARTESIAN_POINT('Ctrl Pts',(200.854638468474,1.58458405733109,48.5));
#76217=CARTESIAN_POINT('Ctrl Pts',(201.04072297737,1.58458405733109,48.5));
#76218=CARTESIAN_POINT('Ctrl Pts',(201.167530667037,1.76466578245163,48.5));
#76219=CARTESIAN_POINT('',(200.854638468474,1.58458405733109,48.35));
#76220=CARTESIAN_POINT('',(200.854638468474,1.58458405733109,48.5));
#76221=CARTESIAN_POINT('Ctrl Pts',(200.854638468474,1.58458405733109,48.35));
#76222=CARTESIAN_POINT('Ctrl Pts',(201.04072297737,1.58458405733109,48.35));
#76223=CARTESIAN_POINT('Ctrl Pts',(201.167530667037,1.76466578245163,48.35));
#76224=CARTESIAN_POINT('Ctrl Pts',(200.541746269912,1.76391565799713,48.5));
#76225=CARTESIAN_POINT('Ctrl Pts',(200.541746269912,1.76391565799713,48.35));
#76226=CARTESIAN_POINT('Ctrl Pts',(200.668553959578,1.58458405733109,48.5));
#76227=CARTESIAN_POINT('Ctrl Pts',(200.668553959578,1.58458405733109,48.35));
#76228=CARTESIAN_POINT('Ctrl Pts',(200.854638468474,1.58458405733109,48.5));
#76229=CARTESIAN_POINT('Ctrl Pts',(200.854638468474,1.58458405733109,48.35));
#76230=CARTESIAN_POINT('',(200.541746269912,1.76391565799713,48.5));
#76231=CARTESIAN_POINT('Ctrl Pts',(200.541746269912,1.76391565799713,48.5));
#76232=CARTESIAN_POINT('Ctrl Pts',(200.668553959578,1.58458405733109,48.5));
#76233=CARTESIAN_POINT('Ctrl Pts',(200.854638468474,1.58458405733109,48.5));
#76234=CARTESIAN_POINT('',(200.541746269912,1.76391565799713,48.35));
#76235=CARTESIAN_POINT('',(200.541746269912,1.76391565799713,48.5));
#76236=CARTESIAN_POINT('Ctrl Pts',(200.541746269912,1.76391565799713,48.35));
#76237=CARTESIAN_POINT('Ctrl Pts',(200.668553959578,1.58458405733109,48.35));
#76238=CARTESIAN_POINT('Ctrl Pts',(200.854638468474,1.58458405733109,48.35));
#76239=CARTESIAN_POINT('Ctrl Pts',(200.414938580245,2.48499327898026,48.5));
#76240=CARTESIAN_POINT('Ctrl Pts',(200.414938580245,2.48499327898026,48.35));
#76241=CARTESIAN_POINT('Ctrl Pts',(200.414938580245,1.94324696063995,48.5));
#76242=CARTESIAN_POINT('Ctrl Pts',(200.414938580245,1.94324696063995,48.35));
#76243=CARTESIAN_POINT('Ctrl Pts',(200.541746269912,1.76391565799713,48.5));
#76244=CARTESIAN_POINT('Ctrl Pts',(200.541746269912,1.76391565799713,48.35));
#76245=CARTESIAN_POINT('',(200.414938580245,2.48499327898026,48.5));
#76246=CARTESIAN_POINT('Ctrl Pts',(200.414938580245,2.48499327898026,48.5));
#76247=CARTESIAN_POINT('Ctrl Pts',(200.414938580245,1.94324696063995,48.5));
#76248=CARTESIAN_POINT('Ctrl Pts',(200.541746269912,1.76391565799713,48.5));
#76249=CARTESIAN_POINT('',(200.414938580245,2.48499327898026,48.35));
#76250=CARTESIAN_POINT('',(200.414938580245,2.48499327898026,48.5));
#76251=CARTESIAN_POINT('Ctrl Pts',(200.414938580245,2.48499327898026,48.35));
#76252=CARTESIAN_POINT('Ctrl Pts',(200.414938580245,1.94324696063995,48.35));
#76253=CARTESIAN_POINT('Ctrl Pts',(200.541746269912,1.76391565799713,48.35));
#76254=CARTESIAN_POINT('Ctrl Pts',(200.55450225994,3.22783091664314,48.5));
#76255=CARTESIAN_POINT('Ctrl Pts',(200.55450225994,3.22783091664314,48.35));
#76256=CARTESIAN_POINT('Ctrl Pts',(200.414938580245,3.02673944830894,48.5));
#76257=CARTESIAN_POINT('Ctrl Pts',(200.414938580245,3.02673944830894,48.35));
#76258=CARTESIAN_POINT('Ctrl Pts',(200.414938580245,2.48499327898026,48.5));
#76259=CARTESIAN_POINT('Ctrl Pts',(200.414938580245,2.48499327898026,48.35));
#76260=CARTESIAN_POINT('Ctrl Pts',(200.55450225994,3.22783091664314,48.5));
#76261=CARTESIAN_POINT('Ctrl Pts',(200.414938580245,3.02673944830894,48.5));
#76262=CARTESIAN_POINT('Ctrl Pts',(200.414938580245,2.48499327898026,48.5));
#76263=CARTESIAN_POINT('Ctrl Pts',(200.55450225994,3.22783091664314,48.35));
#76264=CARTESIAN_POINT('Ctrl Pts',(200.414938580245,3.02673944830894,48.35));
#76265=CARTESIAN_POINT('Ctrl Pts',(200.414938580245,2.48499327898026,48.35));
#76266=CARTESIAN_POINT('Ctrl Pts',(200.854638468474,1.36248314380646,48.5));
#76267=CARTESIAN_POINT('Ctrl Pts',(200.854638468474,1.36248314380646,48.35));
#76268=CARTESIAN_POINT('Ctrl Pts',(200.536493908614,1.36248314380646,48.5));
#76269=CARTESIAN_POINT('Ctrl Pts',(200.536493908614,1.36248314380646,48.35));
#76270=CARTESIAN_POINT('Ctrl Pts',(200.354911338538,1.59058684110642,48.5));
#76271=CARTESIAN_POINT('Ctrl Pts',(200.354911338538,1.59058684110642,48.35));
#76272=CARTESIAN_POINT('',(200.854638468474,1.36248314380646,48.5));
#76273=CARTESIAN_POINT('',(200.354911338538,1.59058684110642,48.5));
#76274=CARTESIAN_POINT('Ctrl Pts',(200.854638468474,1.36248314380646,48.5));
#76275=CARTESIAN_POINT('Ctrl Pts',(200.536493908614,1.36248314380646,48.5));
#76276=CARTESIAN_POINT('Ctrl Pts',(200.354911338538,1.59058684110642,48.5));
#76277=CARTESIAN_POINT('',(200.854638468474,1.36248314380646,48.35));
#76278=CARTESIAN_POINT('',(200.854638468474,1.36248314380646,48.5));
#76279=CARTESIAN_POINT('',(200.354911338538,1.59058684110642,48.35));
#76280=CARTESIAN_POINT('Ctrl Pts',(200.854638468474,1.36248314380646,48.35));
#76281=CARTESIAN_POINT('Ctrl Pts',(200.536493908614,1.36248314380646,48.35));
#76282=CARTESIAN_POINT('Ctrl Pts',(200.354911338538,1.59058684110642,48.35));
#76283=CARTESIAN_POINT('',(200.354911338538,1.59058684110642,48.5));
#76284=CARTESIAN_POINT('Ctrl Pts',(201.254570137709,1.49229192733765,48.5));
#76285=CARTESIAN_POINT('Ctrl Pts',(201.254570137709,1.49229192733765,48.35));
#76286=CARTESIAN_POINT('Ctrl Pts',(201.096248280257,1.36248314380646,48.5));
#76287=CARTESIAN_POINT('Ctrl Pts',(201.096248280257,1.36248314380646,48.35));
#76288=CARTESIAN_POINT('Ctrl Pts',(200.854638468474,1.36248314380646,48.5));
#76289=CARTESIAN_POINT('Ctrl Pts',(200.854638468474,1.36248314380646,48.35));
#76290=CARTESIAN_POINT('',(201.254570137709,1.49229192733765,48.5));
#76291=CARTESIAN_POINT('Ctrl Pts',(201.254570137709,1.49229192733765,48.5));
#76292=CARTESIAN_POINT('Ctrl Pts',(201.096248280257,1.36248314380646,48.5));
#76293=CARTESIAN_POINT('Ctrl Pts',(200.854638468474,1.36248314380646,48.5));
#76294=CARTESIAN_POINT('',(201.254570137709,1.49229192733765,48.35));
#76295=CARTESIAN_POINT('',(201.254570137709,1.49229192733765,48.5));
#76296=CARTESIAN_POINT('Ctrl Pts',(201.254570137709,1.49229192733765,48.35));
#76297=CARTESIAN_POINT('Ctrl Pts',(201.096248280257,1.36248314380646,48.35));
#76298=CARTESIAN_POINT('Ctrl Pts',(200.854638468474,1.36248314380646,48.35));
#76299=CARTESIAN_POINT('Ctrl Pts',(201.49242843315,1.85995900630951,48.5));
#76300=CARTESIAN_POINT('Ctrl Pts',(201.49242843315,1.85995900630951,48.35));
#76301=CARTESIAN_POINT('Ctrl Pts',(201.412891995162,1.62210100889206,48.5));
#76302=CARTESIAN_POINT('Ctrl Pts',(201.412891995162,1.62210100889206,48.35));
#76303=CARTESIAN_POINT('Ctrl Pts',(201.254570137709,1.49229192733765,48.5));
#76304=CARTESIAN_POINT('Ctrl Pts',(201.254570137709,1.49229192733765,48.35));
#76305=CARTESIAN_POINT('',(201.49242843315,1.85995900630951,48.5));
#76306=CARTESIAN_POINT('Ctrl Pts',(201.49242843315,1.85995900630951,48.5));
#76307=CARTESIAN_POINT('Ctrl Pts',(201.412891995162,1.62210100889206,48.5));
#76308=CARTESIAN_POINT('Ctrl Pts',(201.254570137709,1.49229192733765,48.5));
#76309=CARTESIAN_POINT('',(201.49242843315,1.85995900630951,48.35));
#76310=CARTESIAN_POINT('',(201.49242843315,1.85995900630951,48.5));
#76311=CARTESIAN_POINT('Ctrl Pts',(201.49242843315,1.85995900630951,48.35));
#76312=CARTESIAN_POINT('Ctrl Pts',(201.412891995162,1.62210100889206,48.35));
#76313=CARTESIAN_POINT('Ctrl Pts',(201.254570137709,1.49229192733765,48.35));
#76314=CARTESIAN_POINT('Ctrl Pts',(201.571964275092,2.48499327898026,48.5));
#76315=CARTESIAN_POINT('Ctrl Pts',(201.571964275092,2.48499327898026,48.35));
#76316=CARTESIAN_POINT('Ctrl Pts',(201.571964275092,2.09781730175018,48.5));
#76317=CARTESIAN_POINT('Ctrl Pts',(201.571964275092,2.09781730175018,48.35));
#76318=CARTESIAN_POINT('Ctrl Pts',(201.49242843315,1.85995900630951,48.5));
#76319=CARTESIAN_POINT('Ctrl Pts',(201.49242843315,1.85995900630951,48.35));
#76320=CARTESIAN_POINT('',(201.571964275092,2.48499327898026,48.5));
#76321=CARTESIAN_POINT('Ctrl Pts',(201.571964275092,2.48499327898026,48.5));
#76322=CARTESIAN_POINT('Ctrl Pts',(201.571964275092,2.09781730175018,48.5));
#76323=CARTESIAN_POINT('Ctrl Pts',(201.49242843315,1.85995900630951,48.5));
#76324=CARTESIAN_POINT('',(201.571964275092,2.48499327898026,48.35));
#76325=CARTESIAN_POINT('',(201.571964275092,2.48499327898026,48.5));
#76326=CARTESIAN_POINT('Ctrl Pts',(201.571964275092,2.48499327898026,48.35));
#76327=CARTESIAN_POINT('Ctrl Pts',(201.571964275092,2.09781730175018,48.35));
#76328=CARTESIAN_POINT('Ctrl Pts',(201.49242843315,1.85995900630951,48.35));
#76329=CARTESIAN_POINT('Ctrl Pts',(201.52244175598,3.00497958064079,48.5));
#76330=CARTESIAN_POINT('Ctrl Pts',(201.52244175598,3.00497958064079,48.35));
#76331=CARTESIAN_POINT('Ctrl Pts',(201.571964275092,2.81214186549187,48.5));
#76332=CARTESIAN_POINT('Ctrl Pts',(201.571964275092,2.81214186549187,48.35));
#76333=CARTESIAN_POINT('Ctrl Pts',(201.571964275092,2.48499327898026,48.5));
#76334=CARTESIAN_POINT('Ctrl Pts',(201.571964275092,2.48499327898026,48.35));
#76335=CARTESIAN_POINT('',(201.52244175598,3.00497958064079,48.5));
#76336=CARTESIAN_POINT('Ctrl Pts',(201.52244175598,3.00497958064079,48.5));
#76337=CARTESIAN_POINT('Ctrl Pts',(201.571964275092,2.81214186549187,48.5));
#76338=CARTESIAN_POINT('Ctrl Pts',(201.571964275092,2.48499327898026,48.5));
#76339=CARTESIAN_POINT('',(201.52244175598,3.00497958064079,48.35));
#76340=CARTESIAN_POINT('',(201.52244175598,3.00497958064079,48.5));
#76341=CARTESIAN_POINT('Ctrl Pts',(201.52244175598,3.00497958064079,48.35));
#76342=CARTESIAN_POINT('Ctrl Pts',(201.571964275092,2.81214186549187,48.35));
#76343=CARTESIAN_POINT('Ctrl Pts',(201.571964275092,2.48499327898026,48.35));
#76344=CARTESIAN_POINT('Ctrl Pts',(201.385879766196,3.33212831616402,48.5));
#76345=CARTESIAN_POINT('Ctrl Pts',(201.385879766196,3.33212831616402,48.35));
#76346=CARTESIAN_POINT('Ctrl Pts',(201.472919236869,3.19781729578972,48.5));
#76347=CARTESIAN_POINT('Ctrl Pts',(201.472919236869,3.19781729578972,48.35));
#76348=CARTESIAN_POINT('Ctrl Pts',(201.52244175598,3.00497958064079,48.5));
#76349=CARTESIAN_POINT('Ctrl Pts',(201.52244175598,3.00497958064079,48.35));
#76350=CARTESIAN_POINT('',(201.385879766196,3.33212831616402,48.5));
#76351=CARTESIAN_POINT('Ctrl Pts',(201.385879766196,3.33212831616402,48.5));
#76352=CARTESIAN_POINT('Ctrl Pts',(201.472919236869,3.19781729578972,48.5));
#76353=CARTESIAN_POINT('Ctrl Pts',(201.52244175598,3.00497958064079,48.5));
#76354=CARTESIAN_POINT('',(201.385879766196,3.33212831616402,48.35));
#76355=CARTESIAN_POINT('',(201.385879766196,3.33212831616402,48.5));
#76356=CARTESIAN_POINT('Ctrl Pts',(201.385879766196,3.33212831616402,48.35));
#76357=CARTESIAN_POINT('Ctrl Pts',(201.472919236869,3.19781729578972,48.35));
#76358=CARTESIAN_POINT('Ctrl Pts',(201.52244175598,3.00497958064079,48.35));
#76359=CARTESIAN_POINT('Ctrl Pts',(201.16527999565,3.5377217233181,48.5));
#76360=CARTESIAN_POINT('Ctrl Pts',(201.16527999565,3.5377217233181,48.35));
#76361=CARTESIAN_POINT('Ctrl Pts',(201.298840295523,3.46643933653831,48.5));
#76362=CARTESIAN_POINT('Ctrl Pts',(201.298840295523,3.46643933653831,48.35));
#76363=CARTESIAN_POINT('Ctrl Pts',(201.385879766196,3.33212831616402,48.5));
#76364=CARTESIAN_POINT('Ctrl Pts',(201.385879766196,3.33212831616402,48.35));
#76365=CARTESIAN_POINT('',(201.16527999565,3.5377217233181,48.5));
#76366=CARTESIAN_POINT('Ctrl Pts',(201.16527999565,3.5377217233181,48.5));
#76367=CARTESIAN_POINT('Ctrl Pts',(201.298840295523,3.46643933653831,48.5));
#76368=CARTESIAN_POINT('Ctrl Pts',(201.385879766196,3.33212831616402,48.5));
#76369=CARTESIAN_POINT('',(201.16527999565,3.5377217233181,48.35));
#76370=CARTESIAN_POINT('',(201.16527999565,3.5377217233181,48.5));
#76371=CARTESIAN_POINT('Ctrl Pts',(201.16527999565,3.5377217233181,48.35));
#76372=CARTESIAN_POINT('Ctrl Pts',(201.298840295523,3.46643933653831,48.35));
#76373=CARTESIAN_POINT('Ctrl Pts',(201.385879766196,3.33212831616402,48.35));
#76374=CARTESIAN_POINT('Ctrl Pts',(200.854638468474,3.60900411009789,48.5));
#76375=CARTESIAN_POINT('Ctrl Pts',(200.854638468474,3.60900411009789,48.35));
#76376=CARTESIAN_POINT('Ctrl Pts',(201.03171909973,3.60900411009789,48.5));
#76377=CARTESIAN_POINT('Ctrl Pts',(201.03171909973,3.60900411009789,48.35));
#76378=CARTESIAN_POINT('Ctrl Pts',(201.16527999565,3.5377217233181,48.5));
#76379=CARTESIAN_POINT('Ctrl Pts',(201.16527999565,3.5377217233181,48.35));
#76380=CARTESIAN_POINT('',(200.854638468474,3.60900411009789,48.5));
#76381=CARTESIAN_POINT('Ctrl Pts',(200.854638468474,3.60900411009789,48.5));
#76382=CARTESIAN_POINT('Ctrl Pts',(201.03171909973,3.60900411009789,48.5));
#76383=CARTESIAN_POINT('Ctrl Pts',(201.16527999565,3.5377217233181,48.5));
#76384=CARTESIAN_POINT('',(200.854638468474,3.60900411009789,48.35));
#76385=CARTESIAN_POINT('',(200.854638468474,3.60900411009789,48.5));
#76386=CARTESIAN_POINT('Ctrl Pts',(200.854638468474,3.60900411009789,48.35));
#76387=CARTESIAN_POINT('Ctrl Pts',(201.03171909973,3.60900411009789,48.35));
#76388=CARTESIAN_POINT('Ctrl Pts',(201.16527999565,3.5377217233181,48.35));
#76389=CARTESIAN_POINT('Ctrl Pts',(200.456207644194,3.47994545102119,48.5));
#76390=CARTESIAN_POINT('Ctrl Pts',(200.456207644194,3.47994545102119,48.35));
#76391=CARTESIAN_POINT('Ctrl Pts',(200.614529501647,3.60900411009789,48.5));
#76392=CARTESIAN_POINT('Ctrl Pts',(200.614529501647,3.60900411009789,48.35));
#76393=CARTESIAN_POINT('Ctrl Pts',(200.854638468474,3.60900411009789,48.5));
#76394=CARTESIAN_POINT('Ctrl Pts',(200.854638468474,3.60900411009789,48.35));
#76395=CARTESIAN_POINT('',(200.456207644194,3.47994545102119,48.5));
#76396=CARTESIAN_POINT('Ctrl Pts',(200.456207644194,3.47994545102119,48.5));
#76397=CARTESIAN_POINT('Ctrl Pts',(200.614529501647,3.60900411009789,48.5));
#76398=CARTESIAN_POINT('Ctrl Pts',(200.854638468474,3.60900411009789,48.5));
#76399=CARTESIAN_POINT('',(200.456207644194,3.47994545102119,48.35));
#76400=CARTESIAN_POINT('',(200.456207644194,3.47994545102119,48.5));
#76401=CARTESIAN_POINT('Ctrl Pts',(200.456207644194,3.47994545102119,48.35));
#76402=CARTESIAN_POINT('Ctrl Pts',(200.614529501647,3.60900411009789,48.35));
#76403=CARTESIAN_POINT('Ctrl Pts',(200.854638468474,3.60900411009789,48.35));
#76404=CARTESIAN_POINT('Ctrl Pts',(200.217598926276,3.11302864551544,48.5));
#76405=CARTESIAN_POINT('Ctrl Pts',(200.217598926276,3.11302864551544,48.35));
#76406=CARTESIAN_POINT('Ctrl Pts',(200.297885488719,3.3508867919445,48.5));
#76407=CARTESIAN_POINT('Ctrl Pts',(200.297885488719,3.3508867919445,48.35));
#76408=CARTESIAN_POINT('Ctrl Pts',(200.456207644194,3.47994545102119,48.5));
#76409=CARTESIAN_POINT('Ctrl Pts',(200.456207644194,3.47994545102119,48.35));
#76410=CARTESIAN_POINT('',(200.217598926276,3.11302864551544,48.5));
#76411=CARTESIAN_POINT('Ctrl Pts',(200.217598926276,3.11302864551544,48.5));
#76412=CARTESIAN_POINT('Ctrl Pts',(200.297885488719,3.3508867919445,48.5));
#76413=CARTESIAN_POINT('Ctrl Pts',(200.456207644194,3.47994545102119,48.5));
#76414=CARTESIAN_POINT('',(200.217598926276,3.11302864551544,48.35));
#76415=CARTESIAN_POINT('',(200.217598926276,3.11302864551544,48.5));
#76416=CARTESIAN_POINT('Ctrl Pts',(200.217598926276,3.11302864551544,48.35));
#76417=CARTESIAN_POINT('Ctrl Pts',(200.297885488719,3.3508867919445,48.35));
#76418=CARTESIAN_POINT('Ctrl Pts',(200.456207644194,3.47994545102119,48.35));
#76419=CARTESIAN_POINT('Ctrl Pts',(200.137312661856,2.48499327898026,48.5));
#76420=CARTESIAN_POINT('Ctrl Pts',(200.137312661856,2.48499327898026,48.35));
#76421=CARTESIAN_POINT('Ctrl Pts',(200.137312661856,2.87517049908638,48.5));
#76422=CARTESIAN_POINT('Ctrl Pts',(200.137312661856,2.87517049908638,48.35));
#76423=CARTESIAN_POINT('Ctrl Pts',(200.217598926276,3.11302864551544,48.5));
#76424=CARTESIAN_POINT('Ctrl Pts',(200.217598926276,3.11302864551544,48.35));
#76425=CARTESIAN_POINT('',(200.137312661856,2.48499327898026,48.5));
#76426=CARTESIAN_POINT('Ctrl Pts',(200.137312661856,2.48499327898026,48.5));
#76427=CARTESIAN_POINT('Ctrl Pts',(200.137312661856,2.87517049908638,48.5));
#76428=CARTESIAN_POINT('Ctrl Pts',(200.217598926276,3.11302864551544,48.5));
#76429=CARTESIAN_POINT('',(200.137312661856,2.48499327898026,48.35));
#76430=CARTESIAN_POINT('',(200.137312661856,2.48499327898026,48.5));
#76431=CARTESIAN_POINT('Ctrl Pts',(200.137312661856,2.48499327898026,48.35));
#76432=CARTESIAN_POINT('Ctrl Pts',(200.137312661856,2.87517049908638,48.35));
#76433=CARTESIAN_POINT('Ctrl Pts',(200.217598926276,3.11302864551544,48.35));
#76434=CARTESIAN_POINT('Ctrl Pts',(200.354911338538,1.59058684110642,48.5));
#76435=CARTESIAN_POINT('Ctrl Pts',(200.354911338538,1.59058684110642,48.35));
#76436=CARTESIAN_POINT('Ctrl Pts',(200.137312661856,1.86521166563034,48.5));
#76437=CARTESIAN_POINT('Ctrl Pts',(200.137312661856,1.86521166563034,48.35));
#76438=CARTESIAN_POINT('Ctrl Pts',(200.137312661856,2.48499327898026,48.5));
#76439=CARTESIAN_POINT('Ctrl Pts',(200.137312661856,2.48499327898026,48.35));
#76440=CARTESIAN_POINT('Ctrl Pts',(200.354911338538,1.59058684110642,48.5));
#76441=CARTESIAN_POINT('Ctrl Pts',(200.137312661856,1.86521166563034,48.5));
#76442=CARTESIAN_POINT('Ctrl Pts',(200.137312661856,2.48499327898026,48.5));
#76443=CARTESIAN_POINT('Ctrl Pts',(200.354911338538,1.59058684110642,48.35));
#76444=CARTESIAN_POINT('Ctrl Pts',(200.137312661856,1.86521166563034,48.35));
#76445=CARTESIAN_POINT('Ctrl Pts',(200.137312661856,2.48499327898026,48.35));
#76446=CARTESIAN_POINT('Origin',(199.999999951571,2.48574362695217,48.35));
#76447=CARTESIAN_POINT('Ctrl Pts',(199.145361732692,2.38444769382477,48.5));
#76448=CARTESIAN_POINT('Ctrl Pts',(199.145361732692,2.38444769382477,48.35));
#76449=CARTESIAN_POINT('Ctrl Pts',(199.332946937531,2.38444769382477,48.5));
#76450=CARTESIAN_POINT('Ctrl Pts',(199.332946937531,2.38444769382477,48.35));
#76451=CARTESIAN_POINT('Ctrl Pts',(199.453751694411,2.5157573223114,48.5));
#76452=CARTESIAN_POINT('Ctrl Pts',(199.453751694411,2.5157573223114,48.35));
#76453=CARTESIAN_POINT('',(199.145361732692,2.38444769382477,48.5));
#76454=CARTESIAN_POINT('',(199.453751694411,2.5157573223114,48.5));
#76455=CARTESIAN_POINT('Ctrl Pts',(199.145361732692,2.38444769382477,48.5));
#76456=CARTESIAN_POINT('Ctrl Pts',(199.332946937531,2.38444769382477,48.5));
#76457=CARTESIAN_POINT('Ctrl Pts',(199.453751694411,2.5157573223114,48.5));
#76458=CARTESIAN_POINT('',(199.145361732692,2.38444769382477,48.35));
#76459=CARTESIAN_POINT('',(199.145361732692,2.38444769382477,48.5));
#76460=CARTESIAN_POINT('',(199.453751694411,2.5157573223114,48.35));
#76461=CARTESIAN_POINT('Ctrl Pts',(199.145361732692,2.38444769382477,48.35));
#76462=CARTESIAN_POINT('Ctrl Pts',(199.332946937531,2.38444769382477,48.35));
#76463=CARTESIAN_POINT('Ctrl Pts',(199.453751694411,2.5157573223114,48.35));
#76464=CARTESIAN_POINT('',(199.453751694411,2.5157573223114,48.5));
#76465=CARTESIAN_POINT('Ctrl Pts',(198.832469534129,2.5157573223114,48.5));
#76466=CARTESIAN_POINT('Ctrl Pts',(198.832469534129,2.5157573223114,48.35));
#76467=CARTESIAN_POINT('Ctrl Pts',(198.959277223796,2.38444769382477,48.5));
#76468=CARTESIAN_POINT('Ctrl Pts',(198.959277223796,2.38444769382477,48.35));
#76469=CARTESIAN_POINT('Ctrl Pts',(199.145361732692,2.38444769382477,48.5));
#76470=CARTESIAN_POINT('Ctrl Pts',(199.145361732692,2.38444769382477,48.35));
#76471=CARTESIAN_POINT('',(198.832469534129,2.5157573223114,48.5));
#76472=CARTESIAN_POINT('Ctrl Pts',(198.832469534129,2.5157573223114,48.5));
#76473=CARTESIAN_POINT('Ctrl Pts',(198.959277223796,2.38444769382477,48.5));
#76474=CARTESIAN_POINT('Ctrl Pts',(199.145361732692,2.38444769382477,48.5));
#76475=CARTESIAN_POINT('',(198.832469534129,2.5157573223114,48.35));
#76476=CARTESIAN_POINT('',(198.832469534129,2.5157573223114,48.5));
#76477=CARTESIAN_POINT('Ctrl Pts',(198.832469534129,2.5157573223114,48.35));
#76478=CARTESIAN_POINT('Ctrl Pts',(198.959277223796,2.38444769382477,48.35));
#76479=CARTESIAN_POINT('Ctrl Pts',(199.145361732692,2.38444769382477,48.35));
#76480=CARTESIAN_POINT('Ctrl Pts',(198.705661844462,2.85716244578362,48.5));
#76481=CARTESIAN_POINT('Ctrl Pts',(198.705661844462,2.85716244578362,48.35));
#76482=CARTESIAN_POINT('Ctrl Pts',(198.705661844462,2.64706695079803,48.5));
#76483=CARTESIAN_POINT('Ctrl Pts',(198.705661844462,2.64706695079803,48.35));
#76484=CARTESIAN_POINT('Ctrl Pts',(198.832469534129,2.5157573223114,48.5));
#76485=CARTESIAN_POINT('Ctrl Pts',(198.832469534129,2.5157573223114,48.35));
#76486=CARTESIAN_POINT('',(198.705661844462,2.85716244578362,48.5));
#76487=CARTESIAN_POINT('Ctrl Pts',(198.705661844462,2.85716244578362,48.5));
#76488=CARTESIAN_POINT('Ctrl Pts',(198.705661844462,2.64706695079803,48.5));
#76489=CARTESIAN_POINT('Ctrl Pts',(198.832469534129,2.5157573223114,48.5));
#76490=CARTESIAN_POINT('',(198.705661844462,2.85716244578362,48.35));
#76491=CARTESIAN_POINT('',(198.705661844462,2.85716244578362,48.5));
#76492=CARTESIAN_POINT('Ctrl Pts',(198.705661844462,2.85716244578362,48.35));
#76493=CARTESIAN_POINT('Ctrl Pts',(198.705661844462,2.64706695079803,48.35));
#76494=CARTESIAN_POINT('Ctrl Pts',(198.832469534129,2.5157573223114,48.35));
#76495=CARTESIAN_POINT('Ctrl Pts',(198.839222442359,3.23833563923836,48.5));
#76496=CARTESIAN_POINT('Ctrl Pts',(198.839222442359,3.23833563923836,48.35));
#76497=CARTESIAN_POINT('Ctrl Pts',(198.705661844462,3.09126877784729,48.5));
#76498=CARTESIAN_POINT('Ctrl Pts',(198.705661844462,3.09126877784729,48.35));
#76499=CARTESIAN_POINT('Ctrl Pts',(198.705661844462,2.85716244578362,48.5));
#76500=CARTESIAN_POINT('Ctrl Pts',(198.705661844462,2.85716244578362,48.35));
#76501=CARTESIAN_POINT('',(198.839222442359,3.23833563923836,48.5));
#76502=CARTESIAN_POINT('Ctrl Pts',(198.839222442359,3.23833563923836,48.5));
#76503=CARTESIAN_POINT('Ctrl Pts',(198.705661844462,3.09126877784729,48.5));
#76504=CARTESIAN_POINT('Ctrl Pts',(198.705661844462,2.85716244578362,48.5));
#76505=CARTESIAN_POINT('',(198.839222442359,3.23833563923836,48.35));
#76506=CARTESIAN_POINT('',(198.839222442359,3.23833563923836,48.5));
#76507=CARTESIAN_POINT('Ctrl Pts',(198.839222442359,3.23833563923836,48.35));
#76508=CARTESIAN_POINT('Ctrl Pts',(198.705661844462,3.09126877784729,48.35));
#76509=CARTESIAN_POINT('Ctrl Pts',(198.705661844462,2.85716244578362,48.35));
#76510=CARTESIAN_POINT('Ctrl Pts',(199.152865063399,3.38540250062943,48.5));
#76511=CARTESIAN_POINT('Ctrl Pts',(199.152865063399,3.38540250062943,48.35));
#76512=CARTESIAN_POINT('Ctrl Pts',(198.972783338279,3.38540250062943,48.5));
#76513=CARTESIAN_POINT('Ctrl Pts',(198.972783338279,3.38540250062943,48.35));
#76514=CARTESIAN_POINT('Ctrl Pts',(198.839222442359,3.23833563923836,48.5));
#76515=CARTESIAN_POINT('Ctrl Pts',(198.839222442359,3.23833563923836,48.35));
#76516=CARTESIAN_POINT('',(199.152865063399,3.38540250062943,48.5));
#76517=CARTESIAN_POINT('Ctrl Pts',(199.152865063399,3.38540250062943,48.5));
#76518=CARTESIAN_POINT('Ctrl Pts',(198.972783338279,3.38540250062943,48.5));
#76519=CARTESIAN_POINT('Ctrl Pts',(198.839222442359,3.23833563923836,48.5));
#76520=CARTESIAN_POINT('',(199.152865063399,3.38540250062943,48.35));
#76521=CARTESIAN_POINT('',(199.152865063399,3.38540250062943,48.5));
#76522=CARTESIAN_POINT('Ctrl Pts',(199.152865063399,3.38540250062943,48.35));
#76523=CARTESIAN_POINT('Ctrl Pts',(198.972783338279,3.38540250062943,48.35));
#76524=CARTESIAN_POINT('Ctrl Pts',(198.839222442359,3.23833563923836,48.35));
#76525=CARTESIAN_POINT('Ctrl Pts',(199.450750600547,3.24884036183357,48.5));
#76526=CARTESIAN_POINT('Ctrl Pts',(199.450750600547,3.24884036183357,48.35));
#76527=CARTESIAN_POINT('Ctrl Pts',(199.326944302768,3.38540250062943,48.5));
#76528=CARTESIAN_POINT('Ctrl Pts',(199.326944302768,3.38540250062943,48.35));
#76529=CARTESIAN_POINT('Ctrl Pts',(199.152865063399,3.38540250062943,48.5));
#76530=CARTESIAN_POINT('Ctrl Pts',(199.152865063399,3.38540250062943,48.35));
#76531=CARTESIAN_POINT('',(199.450750600547,3.24884036183357,48.5));
#76532=CARTESIAN_POINT('Ctrl Pts',(199.450750600547,3.24884036183357,48.5));
#76533=CARTESIAN_POINT('Ctrl Pts',(199.326944302768,3.38540250062943,48.5));
#76534=CARTESIAN_POINT('Ctrl Pts',(199.152865063399,3.38540250062943,48.5));
#76535=CARTESIAN_POINT('',(199.450750600547,3.24884036183357,48.35));
#76536=CARTESIAN_POINT('',(199.450750600547,3.24884036183357,48.5));
#76537=CARTESIAN_POINT('Ctrl Pts',(199.450750600547,3.24884036183357,48.35));
#76538=CARTESIAN_POINT('Ctrl Pts',(199.326944302768,3.38540250062943,48.35));
#76539=CARTESIAN_POINT('Ctrl Pts',(199.152865063399,3.38540250062943,48.35));
#76540=CARTESIAN_POINT('Ctrl Pts',(199.574556600302,2.87967258691788,48.5));
#76541=CARTESIAN_POINT('Ctrl Pts',(199.574556600302,2.87967258691788,48.35));
#76542=CARTESIAN_POINT('Ctrl Pts',(199.574556600302,3.11227837204933,48.5));
#76543=CARTESIAN_POINT('Ctrl Pts',(199.574556600302,3.11227837204933,48.35));
#76544=CARTESIAN_POINT('Ctrl Pts',(199.450750600547,3.24884036183357,48.5));
#76545=CARTESIAN_POINT('Ctrl Pts',(199.450750600547,3.24884036183357,48.35));
#76546=CARTESIAN_POINT('',(199.574556600302,2.87967258691788,48.5));
#76547=CARTESIAN_POINT('Ctrl Pts',(199.574556600302,2.87967258691788,48.5));
#76548=CARTESIAN_POINT('Ctrl Pts',(199.574556600302,3.11227837204933,48.5));
#76549=CARTESIAN_POINT('Ctrl Pts',(199.450750600547,3.24884036183357,48.5));
#76550=CARTESIAN_POINT('',(199.574556600302,2.87967258691788,48.35));
#76551=CARTESIAN_POINT('',(199.574556600302,2.87967258691788,48.5));
#76552=CARTESIAN_POINT('Ctrl Pts',(199.574556600302,2.87967258691788,48.35));
#76553=CARTESIAN_POINT('Ctrl Pts',(199.574556600302,3.11227837204933,48.35));
#76554=CARTESIAN_POINT('Ctrl Pts',(199.450750600547,3.24884036183357,48.35));
#76555=CARTESIAN_POINT('Ctrl Pts',(199.453751694411,2.5157573223114,48.5));
#76556=CARTESIAN_POINT('Ctrl Pts',(199.453751694411,2.5157573223114,48.35));
#76557=CARTESIAN_POINT('Ctrl Pts',(199.574556600302,2.64706695079803,48.5));
#76558=CARTESIAN_POINT('Ctrl Pts',(199.574556600302,2.64706695079803,48.35));
#76559=CARTESIAN_POINT('Ctrl Pts',(199.574556600302,2.87967258691788,48.5));
#76560=CARTESIAN_POINT('Ctrl Pts',(199.574556600302,2.87967258691788,48.35));
#76561=CARTESIAN_POINT('Ctrl Pts',(199.453751694411,2.5157573223114,48.5));
#76562=CARTESIAN_POINT('Ctrl Pts',(199.574556600302,2.64706695079803,48.5));
#76563=CARTESIAN_POINT('Ctrl Pts',(199.574556600302,2.87967258691788,48.5));
#76564=CARTESIAN_POINT('Ctrl Pts',(199.453751694411,2.5157573223114,48.35));
#76565=CARTESIAN_POINT('Ctrl Pts',(199.574556600302,2.64706695079803,48.35));
#76566=CARTESIAN_POINT('Ctrl Pts',(199.574556600302,2.87967258691788,48.35));
#76567=CARTESIAN_POINT('Ctrl Pts',(199.086835037917,1.36248314380646,48.5));
#76568=CARTESIAN_POINT('Ctrl Pts',(199.086835037917,1.36248314380646,48.35));
#76569=CARTESIAN_POINT('Ctrl Pts',(198.828717719764,1.36248314380646,48.5));
#76570=CARTESIAN_POINT('Ctrl Pts',(198.828717719764,1.36248314380646,48.35));
#76571=CARTESIAN_POINT('Ctrl Pts',(198.665143501014,1.50579804182053,48.5));
#76572=CARTESIAN_POINT('Ctrl Pts',(198.665143501014,1.50579804182053,48.35));
#76573=CARTESIAN_POINT('',(199.086835037917,1.36248314380646,48.5));
#76574=CARTESIAN_POINT('',(198.665143501014,1.50579804182053,48.5));
#76575=CARTESIAN_POINT('Ctrl Pts',(199.086835037917,1.36248314380646,48.5));
#76576=CARTESIAN_POINT('Ctrl Pts',(198.828717719764,1.36248314380646,48.5));
#76577=CARTESIAN_POINT('Ctrl Pts',(198.665143501014,1.50579804182053,48.5));
#76578=CARTESIAN_POINT('',(199.086835037917,1.36248314380646,48.35));
#76579=CARTESIAN_POINT('',(199.086835037917,1.36248314380646,48.5));
#76580=CARTESIAN_POINT('',(198.665143501014,1.50579804182053,48.35));
#76581=CARTESIAN_POINT('Ctrl Pts',(199.086835037917,1.36248314380646,48.35));
#76582=CARTESIAN_POINT('Ctrl Pts',(198.828717719764,1.36248314380646,48.35));
#76583=CARTESIAN_POINT('Ctrl Pts',(198.665143501014,1.50579804182053,48.35));
#76584=CARTESIAN_POINT('',(198.665143501014,1.50579804182053,48.5));
#76585=CARTESIAN_POINT('Ctrl Pts',(199.510777842253,1.49304234981537,48.5));
#76586=CARTESIAN_POINT('Ctrl Pts',(199.510777842253,1.49304234981537,48.35));
#76587=CARTESIAN_POINT('Ctrl Pts',(199.329945545644,1.36248314380646,48.5));
#76588=CARTESIAN_POINT('Ctrl Pts',(199.329945545644,1.36248314380646,48.35));
#76589=CARTESIAN_POINT('Ctrl Pts',(199.086835037917,1.36248314380646,48.5));
#76590=CARTESIAN_POINT('Ctrl Pts',(199.086835037917,1.36248314380646,48.35));
#76591=CARTESIAN_POINT('',(199.510777842253,1.49304234981537,48.5));
#76592=CARTESIAN_POINT('Ctrl Pts',(199.510777842253,1.49304234981537,48.5));
#76593=CARTESIAN_POINT('Ctrl Pts',(199.329945545644,1.36248314380646,48.5));
#76594=CARTESIAN_POINT('Ctrl Pts',(199.086835037917,1.36248314380646,48.5));
#76595=CARTESIAN_POINT('',(199.510777842253,1.49304234981537,48.35));
#76596=CARTESIAN_POINT('',(199.510777842253,1.49304234981537,48.5));
#76597=CARTESIAN_POINT('Ctrl Pts',(199.510777842253,1.49304234981537,48.35));
#76598=CARTESIAN_POINT('Ctrl Pts',(199.329945545644,1.36248314380646,48.35));
#76599=CARTESIAN_POINT('Ctrl Pts',(199.086835037917,1.36248314380646,48.35));
#76600=CARTESIAN_POINT('Ctrl Pts',(199.783151399344,1.87346541881561,48.5));
#76601=CARTESIAN_POINT('Ctrl Pts',(199.783151399344,1.87346541881561,48.35));
#76602=CARTESIAN_POINT('Ctrl Pts',(199.691609989852,1.6236018538475,48.5));
#76603=CARTESIAN_POINT('Ctrl Pts',(199.691609989852,1.6236018538475,48.35));
#76604=CARTESIAN_POINT('Ctrl Pts',(199.510777842253,1.49304234981537,48.5));
#76605=CARTESIAN_POINT('Ctrl Pts',(199.510777842253,1.49304234981537,48.35));
#76606=CARTESIAN_POINT('',(199.783151399344,1.87346541881561,48.5));
#76607=CARTESIAN_POINT('Ctrl Pts',(199.783151399344,1.87346541881561,48.5));
#76608=CARTESIAN_POINT('Ctrl Pts',(199.691609989852,1.6236018538475,48.5));
#76609=CARTESIAN_POINT('Ctrl Pts',(199.510777842253,1.49304234981537,48.5));
#76610=CARTESIAN_POINT('',(199.783151399344,1.87346541881561,48.35));
#76611=CARTESIAN_POINT('',(199.783151399344,1.87346541881561,48.5));
#76612=CARTESIAN_POINT('Ctrl Pts',(199.783151399344,1.87346541881561,48.35));
#76613=CARTESIAN_POINT('Ctrl Pts',(199.691609989852,1.6236018538475,48.35));
#76614=CARTESIAN_POINT('Ctrl Pts',(199.510777842253,1.49304234981537,48.35));
#76615=CARTESIAN_POINT('Ctrl Pts',(199.874693404883,2.5450205206871,48.5));
#76616=CARTESIAN_POINT('Ctrl Pts',(199.874693404883,2.5450205206871,48.35));
#76617=CARTESIAN_POINT('Ctrl Pts',(199.874693404883,2.12332898378372,48.5));
#76618=CARTESIAN_POINT('Ctrl Pts',(199.874693404883,2.12332898378372,48.35));
#76619=CARTESIAN_POINT('Ctrl Pts',(199.783151399344,1.87346541881561,48.5));
#76620=CARTESIAN_POINT('Ctrl Pts',(199.783151399344,1.87346541881561,48.35));
#76621=CARTESIAN_POINT('',(199.874693404883,2.5450205206871,48.5));
#76622=CARTESIAN_POINT('Ctrl Pts',(199.874693404883,2.5450205206871,48.5));
#76623=CARTESIAN_POINT('Ctrl Pts',(199.874693404883,2.12332898378372,48.5));
#76624=CARTESIAN_POINT('Ctrl Pts',(199.783151399344,1.87346541881561,48.5));
#76625=CARTESIAN_POINT('',(199.874693404883,2.5450205206871,48.35));
#76626=CARTESIAN_POINT('',(199.874693404883,2.5450205206871,48.5));
#76627=CARTESIAN_POINT('Ctrl Pts',(199.874693404883,2.5450205206871,48.35));
#76628=CARTESIAN_POINT('Ctrl Pts',(199.874693404883,2.12332898378372,48.35));
#76629=CARTESIAN_POINT('Ctrl Pts',(199.783151399344,1.87346541881561,48.35));
#76630=CARTESIAN_POINT('Ctrl Pts',(199.78240127489,3.16405186057091,48.5));
#76631=CARTESIAN_POINT('Ctrl Pts',(199.78240127489,3.16405186057091,48.35));
#76632=CARTESIAN_POINT('Ctrl Pts',(199.874693404883,2.95020470023155,48.5));
#76633=CARTESIAN_POINT('Ctrl Pts',(199.874693404883,2.95020470023155,48.35));
#76634=CARTESIAN_POINT('Ctrl Pts',(199.874693404883,2.5450205206871,48.5));
#76635=CARTESIAN_POINT('Ctrl Pts',(199.874693404883,2.5450205206871,48.35));
#76636=CARTESIAN_POINT('',(199.78240127489,3.16405186057091,48.5));
#76637=CARTESIAN_POINT('Ctrl Pts',(199.78240127489,3.16405186057091,48.5));
#76638=CARTESIAN_POINT('Ctrl Pts',(199.874693404883,2.95020470023155,48.5));
#76639=CARTESIAN_POINT('Ctrl Pts',(199.874693404883,2.5450205206871,48.5));
#76640=CARTESIAN_POINT('',(199.78240127489,3.16405186057091,48.35));
#76641=CARTESIAN_POINT('',(199.78240127489,3.16405186057091,48.5));
#76642=CARTESIAN_POINT('Ctrl Pts',(199.78240127489,3.16405186057091,48.35));
#76643=CARTESIAN_POINT('Ctrl Pts',(199.874693404883,2.95020470023155,48.35));
#76644=CARTESIAN_POINT('Ctrl Pts',(199.874693404883,2.5450205206871,48.35));
#76645=CARTESIAN_POINT('Ctrl Pts',(199.512278389186,3.49345156550407,48.5));
#76646=CARTESIAN_POINT('Ctrl Pts',(199.512278389186,3.49345156550407,48.35));
#76647=CARTESIAN_POINT('Ctrl Pts',(199.690109144896,3.37789902091026,48.5));
#76648=CARTESIAN_POINT('Ctrl Pts',(199.690109144896,3.37789902091026,48.35));
#76649=CARTESIAN_POINT('Ctrl Pts',(199.78240127489,3.16405186057091,48.5));
#76650=CARTESIAN_POINT('Ctrl Pts',(199.78240127489,3.16405186057091,48.35));
#76651=CARTESIAN_POINT('',(199.512278389186,3.49345156550407,48.5));
#76652=CARTESIAN_POINT('Ctrl Pts',(199.512278389186,3.49345156550407,48.5));
#76653=CARTESIAN_POINT('Ctrl Pts',(199.690109144896,3.37789902091026,48.5));
#76654=CARTESIAN_POINT('Ctrl Pts',(199.78240127489,3.16405186057091,48.5));
#76655=CARTESIAN_POINT('',(199.512278389186,3.49345156550407,48.35));
#76656=CARTESIAN_POINT('',(199.512278389186,3.49345156550407,48.5));
#76657=CARTESIAN_POINT('Ctrl Pts',(199.512278389186,3.49345156550407,48.35));
#76658=CARTESIAN_POINT('Ctrl Pts',(199.690109144896,3.37789902091026,48.35));
#76659=CARTESIAN_POINT('Ctrl Pts',(199.78240127489,3.16405186057091,48.35));
#76660=CARTESIAN_POINT('Ctrl Pts',(199.119850050658,3.60900411009789,48.5));
#76661=CARTESIAN_POINT('Ctrl Pts',(199.119850050658,3.60900411009789,48.35));
#76662=CARTESIAN_POINT('Ctrl Pts',(199.334447633475,3.60900411009789,48.5));
#76663=CARTESIAN_POINT('Ctrl Pts',(199.334447633475,3.60900411009789,48.35));
#76664=CARTESIAN_POINT('Ctrl Pts',(199.512278389186,3.49345156550407,48.5));
#76665=CARTESIAN_POINT('Ctrl Pts',(199.512278389186,3.49345156550407,48.35));
#76666=CARTESIAN_POINT('',(199.119850050658,3.60900411009789,48.5));
#76667=CARTESIAN_POINT('Ctrl Pts',(199.119850050658,3.60900411009789,48.5));
#76668=CARTESIAN_POINT('Ctrl Pts',(199.334447633475,3.60900411009789,48.5));
#76669=CARTESIAN_POINT('Ctrl Pts',(199.512278389186,3.49345156550407,48.5));
#76670=CARTESIAN_POINT('',(199.119850050658,3.60900411009789,48.35));
#76671=CARTESIAN_POINT('',(199.119850050658,3.60900411009789,48.5));
#76672=CARTESIAN_POINT('Ctrl Pts',(199.119850050658,3.60900411009789,48.35));
#76673=CARTESIAN_POINT('Ctrl Pts',(199.334447633475,3.60900411009789,48.35));
#76674=CARTESIAN_POINT('Ctrl Pts',(199.512278389186,3.49345156550407,48.35));
#76675=CARTESIAN_POINT('Ctrl Pts',(198.625375282019,3.40491139888763,48.5));
#76676=CARTESIAN_POINT('Ctrl Pts',(198.625375282019,3.40491139888763,48.35));
#76677=CARTESIAN_POINT('Ctrl Pts',(198.822714935988,3.60900411009789,48.5));
#76678=CARTESIAN_POINT('Ctrl Pts',(198.822714935988,3.60900411009789,48.35));
#76679=CARTESIAN_POINT('Ctrl Pts',(199.119850050658,3.60900411009789,48.5));
#76680=CARTESIAN_POINT('Ctrl Pts',(199.119850050658,3.60900411009789,48.35));
#76681=CARTESIAN_POINT('',(198.625375282019,3.40491139888763,48.5));
#76682=CARTESIAN_POINT('Ctrl Pts',(198.625375282019,3.40491139888763,48.5));
#76683=CARTESIAN_POINT('Ctrl Pts',(198.822714935988,3.60900411009789,48.5));
#76684=CARTESIAN_POINT('Ctrl Pts',(199.119850050658,3.60900411009789,48.5));
#76685=CARTESIAN_POINT('',(198.625375282019,3.40491139888763,48.35));
#76686=CARTESIAN_POINT('',(198.625375282019,3.40491139888763,48.5));
#76687=CARTESIAN_POINT('Ctrl Pts',(198.625375282019,3.40491139888763,48.35));
#76688=CARTESIAN_POINT('Ctrl Pts',(198.822714935988,3.60900411009789,48.35));
#76689=CARTESIAN_POINT('Ctrl Pts',(199.119850050658,3.60900411009789,48.35));
#76690=CARTESIAN_POINT('Ctrl Pts',(198.428035628051,2.866166472435,48.5));
#76691=CARTESIAN_POINT('Ctrl Pts',(198.428035628051,2.866166472435,48.35));
#76692=CARTESIAN_POINT('Ctrl Pts',(198.428035628051,3.20081853866577,48.5));
#76693=CARTESIAN_POINT('Ctrl Pts',(198.428035628051,3.20081853866577,48.35));
#76694=CARTESIAN_POINT('Ctrl Pts',(198.625375282019,3.40491139888763,48.5));
#76695=CARTESIAN_POINT('Ctrl Pts',(198.625375282019,3.40491139888763,48.35));
#76696=CARTESIAN_POINT('',(198.428035628051,2.866166472435,48.5));
#76697=CARTESIAN_POINT('Ctrl Pts',(198.428035628051,2.866166472435,48.5));
#76698=CARTESIAN_POINT('Ctrl Pts',(198.428035628051,3.20081853866577,48.5));
#76699=CARTESIAN_POINT('Ctrl Pts',(198.625375282019,3.40491139888763,48.5));
#76700=CARTESIAN_POINT('',(198.428035628051,2.866166472435,48.35));
#76701=CARTESIAN_POINT('',(198.428035628051,2.866166472435,48.5));
#76702=CARTESIAN_POINT('Ctrl Pts',(198.428035628051,2.866166472435,48.35));
#76703=CARTESIAN_POINT('Ctrl Pts',(198.428035628051,3.20081853866577,48.35));
#76704=CARTESIAN_POINT('Ctrl Pts',(198.625375282019,3.40491139888763,48.35));
#76705=CARTESIAN_POINT('Ctrl Pts',(198.617121528834,2.34392920136452,48.5));
#76706=CARTESIAN_POINT('Ctrl Pts',(198.617121528834,2.34392920136452,48.35));
#76707=CARTESIAN_POINT('Ctrl Pts',(198.428035628051,2.54201912879944,48.5));
#76708=CARTESIAN_POINT('Ctrl Pts',(198.428035628051,2.54201912879944,48.35));
#76709=CARTESIAN_POINT('Ctrl Pts',(198.428035628051,2.866166472435,48.5));
#76710=CARTESIAN_POINT('Ctrl Pts',(198.428035628051,2.866166472435,48.35));
#76711=CARTESIAN_POINT('',(198.617121528834,2.34392920136452,48.5));
#76712=CARTESIAN_POINT('Ctrl Pts',(198.617121528834,2.34392920136452,48.5));
#76713=CARTESIAN_POINT('Ctrl Pts',(198.428035628051,2.54201912879944,48.5));
#76714=CARTESIAN_POINT('Ctrl Pts',(198.428035628051,2.866166472435,48.5));
#76715=CARTESIAN_POINT('',(198.617121528834,2.34392920136452,48.35));
#76716=CARTESIAN_POINT('',(198.617121528834,2.34392920136452,48.5));
#76717=CARTESIAN_POINT('Ctrl Pts',(198.617121528834,2.34392920136452,48.35));
#76718=CARTESIAN_POINT('Ctrl Pts',(198.428035628051,2.54201912879944,48.35));
#76719=CARTESIAN_POINT('Ctrl Pts',(198.428035628051,2.866166472435,48.35));
#76720=CARTESIAN_POINT('Ctrl Pts',(199.079331707209,2.14583912491798,48.5));
#76721=CARTESIAN_POINT('Ctrl Pts',(199.079331707209,2.14583912491798,48.35));
#76722=CARTESIAN_POINT('Ctrl Pts',(198.806207429618,2.14583912491798,48.5));
#76723=CARTESIAN_POINT('Ctrl Pts',(198.806207429618,2.14583912491798,48.35));
#76724=CARTESIAN_POINT('Ctrl Pts',(198.617121528834,2.34392920136452,48.5));
#76725=CARTESIAN_POINT('Ctrl Pts',(198.617121528834,2.34392920136452,48.35));
#76726=CARTESIAN_POINT('',(199.079331707209,2.14583912491798,48.5));
#76727=CARTESIAN_POINT('Ctrl Pts',(199.079331707209,2.14583912491798,48.5));
#76728=CARTESIAN_POINT('Ctrl Pts',(198.806207429618,2.14583912491798,48.5));
#76729=CARTESIAN_POINT('Ctrl Pts',(198.617121528834,2.34392920136452,48.5));
#76730=CARTESIAN_POINT('',(199.079331707209,2.14583912491798,48.35));
#76731=CARTESIAN_POINT('',(199.079331707209,2.14583912491798,48.5));
#76732=CARTESIAN_POINT('Ctrl Pts',(199.079331707209,2.14583912491798,48.35));
#76733=CARTESIAN_POINT('Ctrl Pts',(198.806207429618,2.14583912491798,48.35));
#76734=CARTESIAN_POINT('Ctrl Pts',(198.617121528834,2.34392920136452,48.35));
#76735=CARTESIAN_POINT('Ctrl Pts',(199.383219730109,2.22612553834915,48.5));
#76736=CARTESIAN_POINT('Ctrl Pts',(199.383219730109,2.22612553834915,48.35));
#76737=CARTESIAN_POINT('Ctrl Pts',(199.242905925959,2.14583912491798,48.5));
#76738=CARTESIAN_POINT('Ctrl Pts',(199.242905925959,2.14583912491798,48.35));
#76739=CARTESIAN_POINT('Ctrl Pts',(199.079331707209,2.14583912491798,48.5));
#76740=CARTESIAN_POINT('Ctrl Pts',(199.079331707209,2.14583912491798,48.35));
#76741=CARTESIAN_POINT('',(199.383219730109,2.22612553834915,48.5));
#76742=CARTESIAN_POINT('Ctrl Pts',(199.383219730109,2.22612553834915,48.5));
#76743=CARTESIAN_POINT('Ctrl Pts',(199.242905925959,2.14583912491798,48.5));
#76744=CARTESIAN_POINT('Ctrl Pts',(199.079331707209,2.14583912491798,48.5));
#76745=CARTESIAN_POINT('',(199.383219730109,2.22612553834915,48.35));
#76746=CARTESIAN_POINT('',(199.383219730109,2.22612553834915,48.5));
#76747=CARTESIAN_POINT('Ctrl Pts',(199.383219730109,2.22612553834915,48.35));
#76748=CARTESIAN_POINT('Ctrl Pts',(199.242905925959,2.14583912491798,48.35));
#76749=CARTESIAN_POINT('Ctrl Pts',(199.079331707209,2.14583912491798,48.35));
#76750=CARTESIAN_POINT('Ctrl Pts',(199.604570519179,2.43547075986862,48.5));
#76751=CARTESIAN_POINT('Ctrl Pts',(199.604570519179,2.43547075986862,48.35));
#76752=CARTESIAN_POINT('Ctrl Pts',(199.523533534259,2.30641210079193,48.5));
#76753=CARTESIAN_POINT('Ctrl Pts',(199.523533534259,2.30641210079193,48.35));
#76754=CARTESIAN_POINT('Ctrl Pts',(199.383219730109,2.22612553834915,48.5));
#76755=CARTESIAN_POINT('Ctrl Pts',(199.383219730109,2.22612553834915,48.35));
#76756=CARTESIAN_POINT('',(199.604570519179,2.43547075986862,48.5));
#76757=CARTESIAN_POINT('Ctrl Pts',(199.604570519179,2.43547075986862,48.5));
#76758=CARTESIAN_POINT('Ctrl Pts',(199.523533534259,2.30641210079193,48.5));
#76759=CARTESIAN_POINT('Ctrl Pts',(199.383219730109,2.22612553834915,48.5));
#76760=CARTESIAN_POINT('',(199.604570519179,2.43547075986862,48.35));
#76761=CARTESIAN_POINT('',(199.604570519179,2.43547075986862,48.5));
#76762=CARTESIAN_POINT('Ctrl Pts',(199.604570519179,2.43547075986862,48.35));
#76763=CARTESIAN_POINT('Ctrl Pts',(199.523533534259,2.30641210079193,48.35));
#76764=CARTESIAN_POINT('Ctrl Pts',(199.383219730109,2.22612553834915,48.35));
#76765=CARTESIAN_POINT('Ctrl Pts',(199.606071066111,2.3814463019371,48.5));
#76766=CARTESIAN_POINT('Ctrl Pts',(199.606071066111,2.3814463019371,48.35));
#76767=CARTESIAN_POINT('Ctrl Pts',(199.606071066111,2.39945435523987,48.5));
#76768=CARTESIAN_POINT('Ctrl Pts',(199.606071066111,2.39945435523987,48.35));
#76769=CARTESIAN_POINT('Ctrl Pts',(199.604570519179,2.43547075986862,48.5));
#76770=CARTESIAN_POINT('Ctrl Pts',(199.604570519179,2.43547075986862,48.35));
#76771=CARTESIAN_POINT('',(199.606071066111,2.3814463019371,48.5));
#76772=CARTESIAN_POINT('Ctrl Pts',(199.606071066111,2.3814463019371,48.5));
#76773=CARTESIAN_POINT('Ctrl Pts',(199.606071066111,2.39945435523987,48.5));
#76774=CARTESIAN_POINT('Ctrl Pts',(199.604570519179,2.43547075986862,48.5));
#76775=CARTESIAN_POINT('',(199.606071066111,2.3814463019371,48.35));
#76776=CARTESIAN_POINT('',(199.606071066111,2.3814463019371,48.5));
#76777=CARTESIAN_POINT('Ctrl Pts',(199.606071066111,2.3814463019371,48.35));
#76778=CARTESIAN_POINT('Ctrl Pts',(199.606071066111,2.39945435523987,48.35));
#76779=CARTESIAN_POINT('Ctrl Pts',(199.604570519179,2.43547075986862,48.35));
#76780=CARTESIAN_POINT('Ctrl Pts',(199.565552722663,2.05129617452621,48.5));
#76781=CARTESIAN_POINT('Ctrl Pts',(199.565552722663,2.05129617452621,48.35));
#76782=CARTESIAN_POINT('Ctrl Pts',(199.606071066111,2.21336984634399,48.5));
#76783=CARTESIAN_POINT('Ctrl Pts',(199.606071066111,2.21336984634399,48.35));
#76784=CARTESIAN_POINT('Ctrl Pts',(199.606071066111,2.3814463019371,48.5));
#76785=CARTESIAN_POINT('Ctrl Pts',(199.606071066111,2.3814463019371,48.35));
#76786=CARTESIAN_POINT('',(199.565552722663,2.05129617452621,48.5));
#76787=CARTESIAN_POINT('Ctrl Pts',(199.565552722663,2.05129617452621,48.5));
#76788=CARTESIAN_POINT('Ctrl Pts',(199.606071066111,2.21336984634399,48.5));
#76789=CARTESIAN_POINT('Ctrl Pts',(199.606071066111,2.3814463019371,48.5));
#76790=CARTESIAN_POINT('',(199.565552722663,2.05129617452621,48.35));
#76791=CARTESIAN_POINT('',(199.565552722663,2.05129617452621,48.5));
#76792=CARTESIAN_POINT('Ctrl Pts',(199.565552722663,2.05129617452621,48.35));
#76793=CARTESIAN_POINT('Ctrl Pts',(199.606071066111,2.21336984634399,48.35));
#76794=CARTESIAN_POINT('Ctrl Pts',(199.606071066111,2.3814463019371,48.35));
#76795=CARTESIAN_POINT('Ctrl Pts',(199.465006839484,1.79392898082733,48.5));
#76796=CARTESIAN_POINT('Ctrl Pts',(199.465006839484,1.79392898082733,48.35));
#76797=CARTESIAN_POINT('Ctrl Pts',(199.525034081191,1.88922250270844,48.5));
#76798=CARTESIAN_POINT('Ctrl Pts',(199.525034081191,1.88922250270844,48.35));
#76799=CARTESIAN_POINT('Ctrl Pts',(199.565552722663,2.05129617452621,48.5));
#76800=CARTESIAN_POINT('Ctrl Pts',(199.565552722663,2.05129617452621,48.35));
#76801=CARTESIAN_POINT('',(199.465006839484,1.79392898082733,48.5));
#76802=CARTESIAN_POINT('Ctrl Pts',(199.465006839484,1.79392898082733,48.5));
#76803=CARTESIAN_POINT('Ctrl Pts',(199.525034081191,1.88922250270844,48.5));
#76804=CARTESIAN_POINT('Ctrl Pts',(199.565552722663,2.05129617452621,48.5));
#76805=CARTESIAN_POINT('',(199.465006839484,1.79392898082733,48.35));
#76806=CARTESIAN_POINT('',(199.465006839484,1.79392898082733,48.5));
#76807=CARTESIAN_POINT('Ctrl Pts',(199.465006839484,1.79392898082733,48.35));
#76808=CARTESIAN_POINT('Ctrl Pts',(199.525034081191,1.88922250270844,48.35));
#76809=CARTESIAN_POINT('Ctrl Pts',(199.565552722663,2.05129617452621,48.35));
#76810=CARTESIAN_POINT('Ctrl Pts',(199.311187069863,1.64160990715027,48.5));
#76811=CARTESIAN_POINT('Ctrl Pts',(199.311187069863,1.64160990715027,48.35));
#76812=CARTESIAN_POINT('Ctrl Pts',(199.404979597777,1.69863575696945,48.5));
#76813=CARTESIAN_POINT('Ctrl Pts',(199.404979597777,1.69863575696945,48.35));
#76814=CARTESIAN_POINT('Ctrl Pts',(199.465006839484,1.79392898082733,48.5));
#76815=CARTESIAN_POINT('Ctrl Pts',(199.465006839484,1.79392898082733,48.35));
#76816=CARTESIAN_POINT('',(199.311187069863,1.64160990715027,48.5));
#76817=CARTESIAN_POINT('Ctrl Pts',(199.311187069863,1.64160990715027,48.5));
#76818=CARTESIAN_POINT('Ctrl Pts',(199.404979597777,1.69863575696945,48.5));
#76819=CARTESIAN_POINT('Ctrl Pts',(199.465006839484,1.79392898082733,48.5));
#76820=CARTESIAN_POINT('',(199.311187069863,1.64160990715027,48.35));
#76821=CARTESIAN_POINT('',(199.311187069863,1.64160990715027,48.5));
#76822=CARTESIAN_POINT('Ctrl Pts',(199.311187069863,1.64160990715027,48.35));
#76823=CARTESIAN_POINT('Ctrl Pts',(199.404979597777,1.69863575696945,48.35));
#76824=CARTESIAN_POINT('Ctrl Pts',(199.465006839484,1.79392898082733,48.35));
#76825=CARTESIAN_POINT('Ctrl Pts',(199.092837821692,1.58458405733109,48.5));
#76826=CARTESIAN_POINT('Ctrl Pts',(199.092837821692,1.58458405733109,48.35));
#76827=CARTESIAN_POINT('Ctrl Pts',(199.217394392937,1.58458405733109,48.5));
#76828=CARTESIAN_POINT('Ctrl Pts',(199.217394392937,1.58458405733109,48.35));
#76829=CARTESIAN_POINT('Ctrl Pts',(199.311187069863,1.64160990715027,48.5));
#76830=CARTESIAN_POINT('Ctrl Pts',(199.311187069863,1.64160990715027,48.35));
#76831=CARTESIAN_POINT('',(199.092837821692,1.58458405733109,48.5));
#76832=CARTESIAN_POINT('Ctrl Pts',(199.092837821692,1.58458405733109,48.5));
#76833=CARTESIAN_POINT('Ctrl Pts',(199.217394392937,1.58458405733109,48.5));
#76834=CARTESIAN_POINT('Ctrl Pts',(199.311187069863,1.64160990715027,48.5));
#76835=CARTESIAN_POINT('',(199.092837821692,1.58458405733109,48.35));
#76836=CARTESIAN_POINT('',(199.092837821692,1.58458405733109,48.5));
#76837=CARTESIAN_POINT('Ctrl Pts',(199.092837821692,1.58458405733109,48.35));
#76838=CARTESIAN_POINT('Ctrl Pts',(199.217394392937,1.58458405733109,48.35));
#76839=CARTESIAN_POINT('Ctrl Pts',(199.311187069863,1.64160990715027,48.35));
#76840=CARTESIAN_POINT('Ctrl Pts',(198.854229401797,1.66712158918381,48.5));
#76841=CARTESIAN_POINT('Ctrl Pts',(198.854229401797,1.66712158918381,48.35));
#76842=CARTESIAN_POINT('Ctrl Pts',(198.947271656245,1.58458405733109,48.5));
#76843=CARTESIAN_POINT('Ctrl Pts',(198.947271656245,1.58458405733109,48.35));
#76844=CARTESIAN_POINT('Ctrl Pts',(199.092837821692,1.58458405733109,48.5));
#76845=CARTESIAN_POINT('Ctrl Pts',(199.092837821692,1.58458405733109,48.35));
#76846=CARTESIAN_POINT('',(198.854229401797,1.66712158918381,48.5));
#76847=CARTESIAN_POINT('Ctrl Pts',(198.854229401797,1.66712158918381,48.5));
#76848=CARTESIAN_POINT('Ctrl Pts',(198.947271656245,1.58458405733109,48.5));
#76849=CARTESIAN_POINT('Ctrl Pts',(199.092837821692,1.58458405733109,48.5));
#76850=CARTESIAN_POINT('',(198.854229401797,1.66712158918381,48.35));
#76851=CARTESIAN_POINT('',(198.854229401797,1.66712158918381,48.5));
#76852=CARTESIAN_POINT('Ctrl Pts',(198.854229401797,1.66712158918381,48.35));
#76853=CARTESIAN_POINT('Ctrl Pts',(198.947271656245,1.58458405733109,48.35));
#76854=CARTESIAN_POINT('Ctrl Pts',(199.092837821692,1.58458405733109,48.35));
#76855=CARTESIAN_POINT('Ctrl Pts',(198.728172134608,1.93274223804474,48.5));
#76856=CARTESIAN_POINT('Ctrl Pts',(198.728172134608,1.93274223804474,48.35));
#76857=CARTESIAN_POINT('Ctrl Pts',(198.761187147349,1.74965912103653,48.5));
#76858=CARTESIAN_POINT('Ctrl Pts',(198.761187147349,1.74965912103653,48.35));
#76859=CARTESIAN_POINT('Ctrl Pts',(198.854229401797,1.66712158918381,48.5));
#76860=CARTESIAN_POINT('Ctrl Pts',(198.854229401797,1.66712158918381,48.35));
#76861=CARTESIAN_POINT('',(198.728172134608,1.93274223804474,48.5));
#76862=CARTESIAN_POINT('Ctrl Pts',(198.728172134608,1.93274223804474,48.5));
#76863=CARTESIAN_POINT('Ctrl Pts',(198.761187147349,1.74965912103653,48.5));
#76864=CARTESIAN_POINT('Ctrl Pts',(198.854229401797,1.66712158918381,48.5));
#76865=CARTESIAN_POINT('',(198.728172134608,1.93274223804474,48.35));
#76866=CARTESIAN_POINT('',(198.728172134608,1.93274223804474,48.5));
#76867=CARTESIAN_POINT('Ctrl Pts',(198.728172134608,1.93274223804474,48.35));
#76868=CARTESIAN_POINT('Ctrl Pts',(198.761187147349,1.74965912103653,48.35));
#76869=CARTESIAN_POINT('Ctrl Pts',(198.854229401797,1.66712158918381,48.35));
#76870=CARTESIAN_POINT('Origin',(198.468554120511,1.90873140096664,48.5));
#76871=CARTESIAN_POINT('',(198.468554120511,1.90873140096664,48.5));
#76872=CARTESIAN_POINT('',(100.355168273367,-7.16530967028919,48.5));
#76873=CARTESIAN_POINT('',(198.468554120511,1.90873140096664,48.35));
#76874=CARTESIAN_POINT('',(198.468554120511,1.90873140096664,48.5));
#76875=CARTESIAN_POINT('',(198.468554120511,1.90873140096664,48.35));
#76876=CARTESIAN_POINT('Ctrl Pts',(198.665143501014,1.50579804182053,48.5));
#76877=CARTESIAN_POINT('Ctrl Pts',(198.665143501014,1.50579804182053,48.35));
#76878=CARTESIAN_POINT('Ctrl Pts',(198.501569133252,1.64911323785782,48.5));
#76879=CARTESIAN_POINT('Ctrl Pts',(198.501569133252,1.64911323785782,48.35));
#76880=CARTESIAN_POINT('Ctrl Pts',(198.468554120511,1.90873140096664,48.5));
#76881=CARTESIAN_POINT('Ctrl Pts',(198.468554120511,1.90873140096664,48.35));
#76882=CARTESIAN_POINT('Ctrl Pts',(198.665143501014,1.50579804182053,48.5));
#76883=CARTESIAN_POINT('Ctrl Pts',(198.501569133252,1.64911323785782,48.5));
#76884=CARTESIAN_POINT('Ctrl Pts',(198.468554120511,1.90873140096664,48.5));
#76885=CARTESIAN_POINT('Ctrl Pts',(198.665143501014,1.50579804182053,48.35));
#76886=CARTESIAN_POINT('Ctrl Pts',(198.501569133252,1.64911323785782,48.35));
#76887=CARTESIAN_POINT('Ctrl Pts',(198.468554120511,1.90873140096664,48.35));
#76888=CARTESIAN_POINT('Origin',(199.999999951571,2.48574362695217,48.35));
#76889=CARTESIAN_POINT('Origin',(0.,8.,48.5));
#76890=CARTESIAN_POINT('Origin',(0.,8.,48.5));
#76891=CARTESIAN_POINT('Ctrl Pts',(190.853137893602,3.38540250062943,48.5));
#76892=CARTESIAN_POINT('Ctrl Pts',(190.853137893602,3.38540250062943,48.35));
#76893=CARTESIAN_POINT('Ctrl Pts',(190.667053086683,3.38540250062943,48.5));
#76894=CARTESIAN_POINT('Ctrl Pts',(190.667053086683,3.38540250062943,48.35));
#76895=CARTESIAN_POINT('Ctrl Pts',(190.556002778932,3.22783091664314,48.5));
#76896=CARTESIAN_POINT('Ctrl Pts',(190.556002778932,3.22783091664314,48.35));
#76897=CARTESIAN_POINT('',(190.853137893602,3.38540250062943,48.5));
#76898=CARTESIAN_POINT('',(190.556002778932,3.22783091664314,48.5));
#76899=CARTESIAN_POINT('Ctrl Pts',(190.853137893602,3.38540250062943,48.5));
#76900=CARTESIAN_POINT('Ctrl Pts',(190.667053086683,3.38540250062943,48.5));
#76901=CARTESIAN_POINT('Ctrl Pts',(190.556002778932,3.22783091664314,48.5));
#76902=CARTESIAN_POINT('',(190.853137893602,3.38540250062943,48.35));
#76903=CARTESIAN_POINT('',(190.853137893602,3.38540250062943,48.5));
#76904=CARTESIAN_POINT('',(190.556002778932,3.22783091664314,48.35));
#76905=CARTESIAN_POINT('Ctrl Pts',(190.853137893602,3.38540250062943,48.35));
#76906=CARTESIAN_POINT('Ctrl Pts',(190.667053086683,3.38540250062943,48.35));
#76907=CARTESIAN_POINT('Ctrl Pts',(190.556002778932,3.22783091664314,48.35));
#76908=CARTESIAN_POINT('',(190.556002778932,3.22783091664314,48.5));
#76909=CARTESIAN_POINT('Ctrl Pts',(191.169031186029,3.2068213224411,48.5));
#76910=CARTESIAN_POINT('Ctrl Pts',(191.169031186029,3.2068213224411,48.35));
#76911=CARTESIAN_POINT('Ctrl Pts',(191.042223496363,3.38540250062943,48.5));
#76912=CARTESIAN_POINT('Ctrl Pts',(191.042223496363,3.38540250062943,48.35));
#76913=CARTESIAN_POINT('Ctrl Pts',(190.853137893602,3.38540250062943,48.5));
#76914=CARTESIAN_POINT('Ctrl Pts',(190.853137893602,3.38540250062943,48.35));
#76915=CARTESIAN_POINT('',(191.169031186029,3.2068213224411,48.5));
#76916=CARTESIAN_POINT('Ctrl Pts',(191.169031186029,3.2068213224411,48.5));
#76917=CARTESIAN_POINT('Ctrl Pts',(191.042223496363,3.38540250062943,48.5));
#76918=CARTESIAN_POINT('Ctrl Pts',(190.853137893602,3.38540250062943,48.5));
#76919=CARTESIAN_POINT('',(191.169031186029,3.2068213224411,48.35));
#76920=CARTESIAN_POINT('',(191.169031186029,3.2068213224411,48.5));
#76921=CARTESIAN_POINT('Ctrl Pts',(191.169031186029,3.2068213224411,48.35));
#76922=CARTESIAN_POINT('Ctrl Pts',(191.042223496363,3.38540250062943,48.35));
#76923=CARTESIAN_POINT('Ctrl Pts',(190.853137893602,3.38540250062943,48.35));
#76924=CARTESIAN_POINT('Ctrl Pts',(191.295838875696,2.48499327898026,48.5));
#76925=CARTESIAN_POINT('Ctrl Pts',(191.295838875696,2.48499327898026,48.35));
#76926=CARTESIAN_POINT('Ctrl Pts',(191.295838875696,3.02824014425278,48.5));
#76927=CARTESIAN_POINT('Ctrl Pts',(191.295838875696,3.02824014425278,48.35));
#76928=CARTESIAN_POINT('Ctrl Pts',(191.169031186029,3.2068213224411,48.5));
#76929=CARTESIAN_POINT('Ctrl Pts',(191.169031186029,3.2068213224411,48.35));
#76930=CARTESIAN_POINT('',(191.295838875696,2.48499327898026,48.5));
#76931=CARTESIAN_POINT('Ctrl Pts',(191.295838875696,2.48499327898026,48.5));
#76932=CARTESIAN_POINT('Ctrl Pts',(191.295838875696,3.02824014425278,48.5));
#76933=CARTESIAN_POINT('Ctrl Pts',(191.169031186029,3.2068213224411,48.5));
#76934=CARTESIAN_POINT('',(191.295838875696,2.48499327898026,48.35));
#76935=CARTESIAN_POINT('',(191.295838875696,2.48499327898026,48.5));
#76936=CARTESIAN_POINT('Ctrl Pts',(191.295838875696,2.48499327898026,48.35));
#76937=CARTESIAN_POINT('Ctrl Pts',(191.295838875696,3.02824014425278,48.35));
#76938=CARTESIAN_POINT('Ctrl Pts',(191.169031186029,3.2068213224411,48.35));
#76939=CARTESIAN_POINT('Ctrl Pts',(191.169031186029,1.76466578245163,48.5));
#76940=CARTESIAN_POINT('Ctrl Pts',(191.169031186029,1.76466578245163,48.35));
#76941=CARTESIAN_POINT('Ctrl Pts',(191.295838875696,1.9447478055954,48.5));
#76942=CARTESIAN_POINT('Ctrl Pts',(191.295838875696,1.9447478055954,48.35));
#76943=CARTESIAN_POINT('Ctrl Pts',(191.295838875696,2.48499327898026,48.5));
#76944=CARTESIAN_POINT('Ctrl Pts',(191.295838875696,2.48499327898026,48.35));
#76945=CARTESIAN_POINT('',(191.169031186029,1.76466578245163,48.5));
#76946=CARTESIAN_POINT('Ctrl Pts',(191.169031186029,1.76466578245163,48.5));
#76947=CARTESIAN_POINT('Ctrl Pts',(191.295838875696,1.9447478055954,48.5));
#76948=CARTESIAN_POINT('Ctrl Pts',(191.295838875696,2.48499327898026,48.5));
#76949=CARTESIAN_POINT('',(191.169031186029,1.76466578245163,48.35));
#76950=CARTESIAN_POINT('',(191.169031186029,1.76466578245163,48.5));
#76951=CARTESIAN_POINT('Ctrl Pts',(191.169031186029,1.76466578245163,48.35));
#76952=CARTESIAN_POINT('Ctrl Pts',(191.295838875696,1.9447478055954,48.35));
#76953=CARTESIAN_POINT('Ctrl Pts',(191.295838875696,2.48499327898026,48.35));
#76954=CARTESIAN_POINT('Ctrl Pts',(190.856138987467,1.58458405733109,48.5));
#76955=CARTESIAN_POINT('Ctrl Pts',(190.856138987467,1.58458405733109,48.35));
#76956=CARTESIAN_POINT('Ctrl Pts',(191.042223496363,1.58458405733109,48.5));
#76957=CARTESIAN_POINT('Ctrl Pts',(191.042223496363,1.58458405733109,48.35));
#76958=CARTESIAN_POINT('Ctrl Pts',(191.169031186029,1.76466578245163,48.5));
#76959=CARTESIAN_POINT('Ctrl Pts',(191.169031186029,1.76466578245163,48.35));
#76960=CARTESIAN_POINT('',(190.856138987467,1.58458405733109,48.5));
#76961=CARTESIAN_POINT('Ctrl Pts',(190.856138987467,1.58458405733109,48.5));
#76962=CARTESIAN_POINT('Ctrl Pts',(191.042223496363,1.58458405733109,48.5));
#76963=CARTESIAN_POINT('Ctrl Pts',(191.169031186029,1.76466578245163,48.5));
#76964=CARTESIAN_POINT('',(190.856138987467,1.58458405733109,48.35));
#76965=CARTESIAN_POINT('',(190.856138987467,1.58458405733109,48.5));
#76966=CARTESIAN_POINT('Ctrl Pts',(190.856138987467,1.58458405733109,48.35));
#76967=CARTESIAN_POINT('Ctrl Pts',(191.042223496363,1.58458405733109,48.35));
#76968=CARTESIAN_POINT('Ctrl Pts',(191.169031186029,1.76466578245163,48.35));
#76969=CARTESIAN_POINT('Ctrl Pts',(190.543246788904,1.76391565799713,48.5));
#76970=CARTESIAN_POINT('Ctrl Pts',(190.543246788904,1.76391565799713,48.35));
#76971=CARTESIAN_POINT('Ctrl Pts',(190.670054478571,1.58458405733109,48.5));
#76972=CARTESIAN_POINT('Ctrl Pts',(190.670054478571,1.58458405733109,48.35));
#76973=CARTESIAN_POINT('Ctrl Pts',(190.856138987467,1.58458405733109,48.5));
#76974=CARTESIAN_POINT('Ctrl Pts',(190.856138987467,1.58458405733109,48.35));
#76975=CARTESIAN_POINT('',(190.543246788904,1.76391565799713,48.5));
#76976=CARTESIAN_POINT('Ctrl Pts',(190.543246788904,1.76391565799713,48.5));
#76977=CARTESIAN_POINT('Ctrl Pts',(190.670054478571,1.58458405733109,48.5));
#76978=CARTESIAN_POINT('Ctrl Pts',(190.856138987467,1.58458405733109,48.5));
#76979=CARTESIAN_POINT('',(190.543246788904,1.76391565799713,48.35));
#76980=CARTESIAN_POINT('',(190.543246788904,1.76391565799713,48.5));
#76981=CARTESIAN_POINT('Ctrl Pts',(190.543246788904,1.76391565799713,48.35));
#76982=CARTESIAN_POINT('Ctrl Pts',(190.670054478571,1.58458405733109,48.35));
#76983=CARTESIAN_POINT('Ctrl Pts',(190.856138987467,1.58458405733109,48.35));
#76984=CARTESIAN_POINT('Ctrl Pts',(190.416439099237,2.48499327898026,48.5));
#76985=CARTESIAN_POINT('Ctrl Pts',(190.416439099237,2.48499327898026,48.35));
#76986=CARTESIAN_POINT('Ctrl Pts',(190.416439099237,1.94324696063995,48.5));
#76987=CARTESIAN_POINT('Ctrl Pts',(190.416439099237,1.94324696063995,48.35));
#76988=CARTESIAN_POINT('Ctrl Pts',(190.543246788904,1.76391565799713,48.5));
#76989=CARTESIAN_POINT('Ctrl Pts',(190.543246788904,1.76391565799713,48.35));
#76990=CARTESIAN_POINT('',(190.416439099237,2.48499327898026,48.5));
#76991=CARTESIAN_POINT('Ctrl Pts',(190.416439099237,2.48499327898026,48.5));
#76992=CARTESIAN_POINT('Ctrl Pts',(190.416439099237,1.94324696063995,48.5));
#76993=CARTESIAN_POINT('Ctrl Pts',(190.543246788904,1.76391565799713,48.5));
#76994=CARTESIAN_POINT('',(190.416439099237,2.48499327898026,48.35));
#76995=CARTESIAN_POINT('',(190.416439099237,2.48499327898026,48.5));
#76996=CARTESIAN_POINT('Ctrl Pts',(190.416439099237,2.48499327898026,48.35));
#76997=CARTESIAN_POINT('Ctrl Pts',(190.416439099237,1.94324696063995,48.35));
#76998=CARTESIAN_POINT('Ctrl Pts',(190.543246788904,1.76391565799713,48.35));
#76999=CARTESIAN_POINT('Ctrl Pts',(190.556002778932,3.22783091664314,48.5));
#77000=CARTESIAN_POINT('Ctrl Pts',(190.556002778932,3.22783091664314,48.35));
#77001=CARTESIAN_POINT('Ctrl Pts',(190.416439099237,3.02673944830894,48.5));
#77002=CARTESIAN_POINT('Ctrl Pts',(190.416439099237,3.02673944830894,48.35));
#77003=CARTESIAN_POINT('Ctrl Pts',(190.416439099237,2.48499327898026,48.5));
#77004=CARTESIAN_POINT('Ctrl Pts',(190.416439099237,2.48499327898026,48.35));
#77005=CARTESIAN_POINT('Ctrl Pts',(190.556002778932,3.22783091664314,48.5));
#77006=CARTESIAN_POINT('Ctrl Pts',(190.416439099237,3.02673944830894,48.5));
#77007=CARTESIAN_POINT('Ctrl Pts',(190.416439099237,2.48499327898026,48.5));
#77008=CARTESIAN_POINT('Ctrl Pts',(190.556002778932,3.22783091664314,48.35));
#77009=CARTESIAN_POINT('Ctrl Pts',(190.416439099237,3.02673944830894,48.35));
#77010=CARTESIAN_POINT('Ctrl Pts',(190.416439099237,2.48499327898026,48.35));
#77011=CARTESIAN_POINT('Ctrl Pts',(190.856138987467,1.36248314380646,48.5));
#77012=CARTESIAN_POINT('Ctrl Pts',(190.856138987467,1.36248314380646,48.35));
#77013=CARTESIAN_POINT('Ctrl Pts',(190.537994427606,1.36248314380646,48.5));
#77014=CARTESIAN_POINT('Ctrl Pts',(190.537994427606,1.36248314380646,48.35));
#77015=CARTESIAN_POINT('Ctrl Pts',(190.35641185753,1.59058684110642,48.5));
#77016=CARTESIAN_POINT('Ctrl Pts',(190.35641185753,1.59058684110642,48.35));
#77017=CARTESIAN_POINT('',(190.856138987467,1.36248314380646,48.5));
#77018=CARTESIAN_POINT('',(190.35641185753,1.59058684110642,48.5));
#77019=CARTESIAN_POINT('Ctrl Pts',(190.856138987467,1.36248314380646,48.5));
#77020=CARTESIAN_POINT('Ctrl Pts',(190.537994427606,1.36248314380646,48.5));
#77021=CARTESIAN_POINT('Ctrl Pts',(190.35641185753,1.59058684110642,48.5));
#77022=CARTESIAN_POINT('',(190.856138987467,1.36248314380646,48.35));
#77023=CARTESIAN_POINT('',(190.856138987467,1.36248314380646,48.5));
#77024=CARTESIAN_POINT('',(190.35641185753,1.59058684110642,48.35));
#77025=CARTESIAN_POINT('Ctrl Pts',(190.856138987467,1.36248314380646,48.35));
#77026=CARTESIAN_POINT('Ctrl Pts',(190.537994427606,1.36248314380646,48.35));
#77027=CARTESIAN_POINT('Ctrl Pts',(190.35641185753,1.59058684110642,48.35));
#77028=CARTESIAN_POINT('',(190.35641185753,1.59058684110642,48.5));
#77029=CARTESIAN_POINT('Ctrl Pts',(191.256070656702,1.49229192733765,48.5));
#77030=CARTESIAN_POINT('Ctrl Pts',(191.256070656702,1.49229192733765,48.35));
#77031=CARTESIAN_POINT('Ctrl Pts',(191.09774879925,1.36248314380646,48.5));
#77032=CARTESIAN_POINT('Ctrl Pts',(191.09774879925,1.36248314380646,48.35));
#77033=CARTESIAN_POINT('Ctrl Pts',(190.856138987467,1.36248314380646,48.5));
#77034=CARTESIAN_POINT('Ctrl Pts',(190.856138987467,1.36248314380646,48.35));
#77035=CARTESIAN_POINT('',(191.256070656702,1.49229192733765,48.5));
#77036=CARTESIAN_POINT('Ctrl Pts',(191.256070656702,1.49229192733765,48.5));
#77037=CARTESIAN_POINT('Ctrl Pts',(191.09774879925,1.36248314380646,48.5));
#77038=CARTESIAN_POINT('Ctrl Pts',(190.856138987467,1.36248314380646,48.5));
#77039=CARTESIAN_POINT('',(191.256070656702,1.49229192733765,48.35));
#77040=CARTESIAN_POINT('',(191.256070656702,1.49229192733765,48.5));
#77041=CARTESIAN_POINT('Ctrl Pts',(191.256070656702,1.49229192733765,48.35));
#77042=CARTESIAN_POINT('Ctrl Pts',(191.09774879925,1.36248314380646,48.35));
#77043=CARTESIAN_POINT('Ctrl Pts',(190.856138987467,1.36248314380646,48.35));
#77044=CARTESIAN_POINT('Ctrl Pts',(191.493928952143,1.85995900630951,48.5));
#77045=CARTESIAN_POINT('Ctrl Pts',(191.493928952143,1.85995900630951,48.35));
#77046=CARTESIAN_POINT('Ctrl Pts',(191.414392514154,1.62210100889206,48.5));
#77047=CARTESIAN_POINT('Ctrl Pts',(191.414392514154,1.62210100889206,48.35));
#77048=CARTESIAN_POINT('Ctrl Pts',(191.256070656702,1.49229192733765,48.5));
#77049=CARTESIAN_POINT('Ctrl Pts',(191.256070656702,1.49229192733765,48.35));
#77050=CARTESIAN_POINT('',(191.493928952143,1.85995900630951,48.5));
#77051=CARTESIAN_POINT('Ctrl Pts',(191.493928952143,1.85995900630951,48.5));
#77052=CARTESIAN_POINT('Ctrl Pts',(191.414392514154,1.62210100889206,48.5));
#77053=CARTESIAN_POINT('Ctrl Pts',(191.256070656702,1.49229192733765,48.5));
#77054=CARTESIAN_POINT('',(191.493928952143,1.85995900630951,48.35));
#77055=CARTESIAN_POINT('',(191.493928952143,1.85995900630951,48.5));
#77056=CARTESIAN_POINT('Ctrl Pts',(191.493928952143,1.85995900630951,48.35));
#77057=CARTESIAN_POINT('Ctrl Pts',(191.414392514154,1.62210100889206,48.35));
#77058=CARTESIAN_POINT('Ctrl Pts',(191.256070656702,1.49229192733765,48.35));
#77059=CARTESIAN_POINT('Ctrl Pts',(191.573464794084,2.48499327898026,48.5));
#77060=CARTESIAN_POINT('Ctrl Pts',(191.573464794084,2.48499327898026,48.35));
#77061=CARTESIAN_POINT('Ctrl Pts',(191.573464794084,2.09781730175018,48.5));
#77062=CARTESIAN_POINT('Ctrl Pts',(191.573464794084,2.09781730175018,48.35));
#77063=CARTESIAN_POINT('Ctrl Pts',(191.493928952143,1.85995900630951,48.5));
#77064=CARTESIAN_POINT('Ctrl Pts',(191.493928952143,1.85995900630951,48.35));
#77065=CARTESIAN_POINT('',(191.573464794084,2.48499327898026,48.5));
#77066=CARTESIAN_POINT('Ctrl Pts',(191.573464794084,2.48499327898026,48.5));
#77067=CARTESIAN_POINT('Ctrl Pts',(191.573464794084,2.09781730175018,48.5));
#77068=CARTESIAN_POINT('Ctrl Pts',(191.493928952143,1.85995900630951,48.5));
#77069=CARTESIAN_POINT('',(191.573464794084,2.48499327898026,48.35));
#77070=CARTESIAN_POINT('',(191.573464794084,2.48499327898026,48.5));
#77071=CARTESIAN_POINT('Ctrl Pts',(191.573464794084,2.48499327898026,48.35));
#77072=CARTESIAN_POINT('Ctrl Pts',(191.573464794084,2.09781730175018,48.35));
#77073=CARTESIAN_POINT('Ctrl Pts',(191.493928952143,1.85995900630951,48.35));
#77074=CARTESIAN_POINT('Ctrl Pts',(191.523942274973,3.00497958064079,48.5));
#77075=CARTESIAN_POINT('Ctrl Pts',(191.523942274973,3.00497958064079,48.35));
#77076=CARTESIAN_POINT('Ctrl Pts',(191.573464794084,2.81214186549187,48.5));
#77077=CARTESIAN_POINT('Ctrl Pts',(191.573464794084,2.81214186549187,48.35));
#77078=CARTESIAN_POINT('Ctrl Pts',(191.573464794084,2.48499327898026,48.5));
#77079=CARTESIAN_POINT('Ctrl Pts',(191.573464794084,2.48499327898026,48.35));
#77080=CARTESIAN_POINT('',(191.523942274973,3.00497958064079,48.5));
#77081=CARTESIAN_POINT('Ctrl Pts',(191.523942274973,3.00497958064079,48.5));
#77082=CARTESIAN_POINT('Ctrl Pts',(191.573464794084,2.81214186549187,48.5));
#77083=CARTESIAN_POINT('Ctrl Pts',(191.573464794084,2.48499327898026,48.5));
#77084=CARTESIAN_POINT('',(191.523942274973,3.00497958064079,48.35));
#77085=CARTESIAN_POINT('',(191.523942274973,3.00497958064079,48.5));
#77086=CARTESIAN_POINT('Ctrl Pts',(191.523942274973,3.00497958064079,48.35));
#77087=CARTESIAN_POINT('Ctrl Pts',(191.573464794084,2.81214186549187,48.35));
#77088=CARTESIAN_POINT('Ctrl Pts',(191.573464794084,2.48499327898026,48.35));
#77089=CARTESIAN_POINT('Ctrl Pts',(191.387380285189,3.33212831616402,48.5));
#77090=CARTESIAN_POINT('Ctrl Pts',(191.387380285189,3.33212831616402,48.35));
#77091=CARTESIAN_POINT('Ctrl Pts',(191.474419755861,3.19781729578972,48.5));
#77092=CARTESIAN_POINT('Ctrl Pts',(191.474419755861,3.19781729578972,48.35));
#77093=CARTESIAN_POINT('Ctrl Pts',(191.523942274973,3.00497958064079,48.5));
#77094=CARTESIAN_POINT('Ctrl Pts',(191.523942274973,3.00497958064079,48.35));
#77095=CARTESIAN_POINT('',(191.387380285189,3.33212831616402,48.5));
#77096=CARTESIAN_POINT('Ctrl Pts',(191.387380285189,3.33212831616402,48.5));
#77097=CARTESIAN_POINT('Ctrl Pts',(191.474419755861,3.19781729578972,48.5));
#77098=CARTESIAN_POINT('Ctrl Pts',(191.523942274973,3.00497958064079,48.5));
#77099=CARTESIAN_POINT('',(191.387380285189,3.33212831616402,48.35));
#77100=CARTESIAN_POINT('',(191.387380285189,3.33212831616402,48.5));
#77101=CARTESIAN_POINT('Ctrl Pts',(191.387380285189,3.33212831616402,48.35));
#77102=CARTESIAN_POINT('Ctrl Pts',(191.474419755861,3.19781729578972,48.35));
#77103=CARTESIAN_POINT('Ctrl Pts',(191.523942274973,3.00497958064079,48.35));
#77104=CARTESIAN_POINT('Ctrl Pts',(191.166780514643,3.5377217233181,48.5));
#77105=CARTESIAN_POINT('Ctrl Pts',(191.166780514643,3.5377217233181,48.35));
#77106=CARTESIAN_POINT('Ctrl Pts',(191.300340814516,3.46643933653831,48.5));
#77107=CARTESIAN_POINT('Ctrl Pts',(191.300340814516,3.46643933653831,48.35));
#77108=CARTESIAN_POINT('Ctrl Pts',(191.387380285189,3.33212831616402,48.5));
#77109=CARTESIAN_POINT('Ctrl Pts',(191.387380285189,3.33212831616402,48.35));
#77110=CARTESIAN_POINT('',(191.166780514643,3.5377217233181,48.5));
#77111=CARTESIAN_POINT('Ctrl Pts',(191.166780514643,3.5377217233181,48.5));
#77112=CARTESIAN_POINT('Ctrl Pts',(191.300340814516,3.46643933653831,48.5));
#77113=CARTESIAN_POINT('Ctrl Pts',(191.387380285189,3.33212831616402,48.5));
#77114=CARTESIAN_POINT('',(191.166780514643,3.5377217233181,48.35));
#77115=CARTESIAN_POINT('',(191.166780514643,3.5377217233181,48.5));
#77116=CARTESIAN_POINT('Ctrl Pts',(191.166780514643,3.5377217233181,48.35));
#77117=CARTESIAN_POINT('Ctrl Pts',(191.300340814516,3.46643933653831,48.35));
#77118=CARTESIAN_POINT('Ctrl Pts',(191.387380285189,3.33212831616402,48.35));
#77119=CARTESIAN_POINT('Ctrl Pts',(190.856138987467,3.60900411009789,48.5));
#77120=CARTESIAN_POINT('Ctrl Pts',(190.856138987467,3.60900411009789,48.35));
#77121=CARTESIAN_POINT('Ctrl Pts',(191.033219618723,3.60900411009789,48.5));
#77122=CARTESIAN_POINT('Ctrl Pts',(191.033219618723,3.60900411009789,48.35));
#77123=CARTESIAN_POINT('Ctrl Pts',(191.166780514643,3.5377217233181,48.5));
#77124=CARTESIAN_POINT('Ctrl Pts',(191.166780514643,3.5377217233181,48.35));
#77125=CARTESIAN_POINT('',(190.856138987467,3.60900411009789,48.5));
#77126=CARTESIAN_POINT('Ctrl Pts',(190.856138987467,3.60900411009789,48.5));
#77127=CARTESIAN_POINT('Ctrl Pts',(191.033219618723,3.60900411009789,48.5));
#77128=CARTESIAN_POINT('Ctrl Pts',(191.166780514643,3.5377217233181,48.5));
#77129=CARTESIAN_POINT('',(190.856138987467,3.60900411009789,48.35));
#77130=CARTESIAN_POINT('',(190.856138987467,3.60900411009789,48.5));
#77131=CARTESIAN_POINT('Ctrl Pts',(190.856138987467,3.60900411009789,48.35));
#77132=CARTESIAN_POINT('Ctrl Pts',(191.033219618723,3.60900411009789,48.35));
#77133=CARTESIAN_POINT('Ctrl Pts',(191.166780514643,3.5377217233181,48.35));
#77134=CARTESIAN_POINT('Ctrl Pts',(190.457708163187,3.47994545102119,48.5));
#77135=CARTESIAN_POINT('Ctrl Pts',(190.457708163187,3.47994545102119,48.35));
#77136=CARTESIAN_POINT('Ctrl Pts',(190.616030020639,3.60900411009789,48.5));
#77137=CARTESIAN_POINT('Ctrl Pts',(190.616030020639,3.60900411009789,48.35));
#77138=CARTESIAN_POINT('Ctrl Pts',(190.856138987467,3.60900411009789,48.5));
#77139=CARTESIAN_POINT('Ctrl Pts',(190.856138987467,3.60900411009789,48.35));
#77140=CARTESIAN_POINT('',(190.457708163187,3.47994545102119,48.5));
#77141=CARTESIAN_POINT('Ctrl Pts',(190.457708163187,3.47994545102119,48.5));
#77142=CARTESIAN_POINT('Ctrl Pts',(190.616030020639,3.60900411009789,48.5));
#77143=CARTESIAN_POINT('Ctrl Pts',(190.856138987467,3.60900411009789,48.5));
#77144=CARTESIAN_POINT('',(190.457708163187,3.47994545102119,48.35));
#77145=CARTESIAN_POINT('',(190.457708163187,3.47994545102119,48.5));
#77146=CARTESIAN_POINT('Ctrl Pts',(190.457708163187,3.47994545102119,48.35));
#77147=CARTESIAN_POINT('Ctrl Pts',(190.616030020639,3.60900411009789,48.35));
#77148=CARTESIAN_POINT('Ctrl Pts',(190.856138987467,3.60900411009789,48.35));
#77149=CARTESIAN_POINT('Ctrl Pts',(190.219099445269,3.11302864551544,48.5));
#77150=CARTESIAN_POINT('Ctrl Pts',(190.219099445269,3.11302864551544,48.35));
#77151=CARTESIAN_POINT('Ctrl Pts',(190.299386007711,3.3508867919445,48.5));
#77152=CARTESIAN_POINT('Ctrl Pts',(190.299386007711,3.3508867919445,48.35));
#77153=CARTESIAN_POINT('Ctrl Pts',(190.457708163187,3.47994545102119,48.5));
#77154=CARTESIAN_POINT('Ctrl Pts',(190.457708163187,3.47994545102119,48.35));
#77155=CARTESIAN_POINT('',(190.219099445269,3.11302864551544,48.5));
#77156=CARTESIAN_POINT('Ctrl Pts',(190.219099445269,3.11302864551544,48.5));
#77157=CARTESIAN_POINT('Ctrl Pts',(190.299386007711,3.3508867919445,48.5));
#77158=CARTESIAN_POINT('Ctrl Pts',(190.457708163187,3.47994545102119,48.5));
#77159=CARTESIAN_POINT('',(190.219099445269,3.11302864551544,48.35));
#77160=CARTESIAN_POINT('',(190.219099445269,3.11302864551544,48.5));
#77161=CARTESIAN_POINT('Ctrl Pts',(190.219099445269,3.11302864551544,48.35));
#77162=CARTESIAN_POINT('Ctrl Pts',(190.299386007711,3.3508867919445,48.35));
#77163=CARTESIAN_POINT('Ctrl Pts',(190.457708163187,3.47994545102119,48.35));
#77164=CARTESIAN_POINT('Ctrl Pts',(190.138813180849,2.48499327898026,48.5));
#77165=CARTESIAN_POINT('Ctrl Pts',(190.138813180849,2.48499327898026,48.35));
#77166=CARTESIAN_POINT('Ctrl Pts',(190.138813180849,2.87517049908638,48.5));
#77167=CARTESIAN_POINT('Ctrl Pts',(190.138813180849,2.87517049908638,48.35));
#77168=CARTESIAN_POINT('Ctrl Pts',(190.219099445269,3.11302864551544,48.5));
#77169=CARTESIAN_POINT('Ctrl Pts',(190.219099445269,3.11302864551544,48.35));
#77170=CARTESIAN_POINT('',(190.138813180849,2.48499327898026,48.5));
#77171=CARTESIAN_POINT('Ctrl Pts',(190.138813180849,2.48499327898026,48.5));
#77172=CARTESIAN_POINT('Ctrl Pts',(190.138813180849,2.87517049908638,48.5));
#77173=CARTESIAN_POINT('Ctrl Pts',(190.219099445269,3.11302864551544,48.5));
#77174=CARTESIAN_POINT('',(190.138813180849,2.48499327898026,48.35));
#77175=CARTESIAN_POINT('',(190.138813180849,2.48499327898026,48.5));
#77176=CARTESIAN_POINT('Ctrl Pts',(190.138813180849,2.48499327898026,48.35));
#77177=CARTESIAN_POINT('Ctrl Pts',(190.138813180849,2.87517049908638,48.35));
#77178=CARTESIAN_POINT('Ctrl Pts',(190.219099445269,3.11302864551544,48.35));
#77179=CARTESIAN_POINT('Ctrl Pts',(190.35641185753,1.59058684110642,48.5));
#77180=CARTESIAN_POINT('Ctrl Pts',(190.35641185753,1.59058684110642,48.35));
#77181=CARTESIAN_POINT('Ctrl Pts',(190.138813180849,1.86521166563034,48.5));
#77182=CARTESIAN_POINT('Ctrl Pts',(190.138813180849,1.86521166563034,48.35));
#77183=CARTESIAN_POINT('Ctrl Pts',(190.138813180849,2.48499327898026,48.5));
#77184=CARTESIAN_POINT('Ctrl Pts',(190.138813180849,2.48499327898026,48.35));
#77185=CARTESIAN_POINT('Ctrl Pts',(190.35641185753,1.59058684110642,48.5));
#77186=CARTESIAN_POINT('Ctrl Pts',(190.138813180849,1.86521166563034,48.5));
#77187=CARTESIAN_POINT('Ctrl Pts',(190.138813180849,2.48499327898026,48.5));
#77188=CARTESIAN_POINT('Ctrl Pts',(190.35641185753,1.59058684110642,48.35));
#77189=CARTESIAN_POINT('Ctrl Pts',(190.138813180849,1.86521166563034,48.35));
#77190=CARTESIAN_POINT('Ctrl Pts',(190.138813180849,2.48499327898026,48.35));
#77191=CARTESIAN_POINT('Origin',(189.99999977462,2.48574362695217,48.35));
#77192=CARTESIAN_POINT('Ctrl Pts',(189.149863643572,3.38690319657326,48.5));
#77193=CARTESIAN_POINT('Ctrl Pts',(189.149863643572,3.38690319657326,48.35));
#77194=CARTESIAN_POINT('Ctrl Pts',(188.995293302462,3.38690319657326,48.5));
#77195=CARTESIAN_POINT('Ctrl Pts',(188.995293302462,3.38690319657326,48.35));
#77196=CARTESIAN_POINT('Ctrl Pts',(188.893246872351,3.28785815834999,48.5));
#77197=CARTESIAN_POINT('Ctrl Pts',(188.893246872351,3.28785815834999,48.35));
#77198=CARTESIAN_POINT('',(189.149863643572,3.38690319657326,48.5));
#77199=CARTESIAN_POINT('',(188.893246872351,3.28785815834999,48.5));
#77200=CARTESIAN_POINT('Ctrl Pts',(189.149863643572,3.38690319657326,48.5));
#77201=CARTESIAN_POINT('Ctrl Pts',(188.995293302462,3.38690319657326,48.5));
#77202=CARTESIAN_POINT('Ctrl Pts',(188.893246872351,3.28785815834999,48.5));
#77203=CARTESIAN_POINT('',(189.149863643572,3.38690319657326,48.35));
#77204=CARTESIAN_POINT('',(189.149863643572,3.38690319657326,48.5));
#77205=CARTESIAN_POINT('',(188.893246872351,3.28785815834999,48.35));
#77206=CARTESIAN_POINT('Ctrl Pts',(189.149863643572,3.38690319657326,48.35));
#77207=CARTESIAN_POINT('Ctrl Pts',(188.995293302462,3.38690319657326,48.35));
#77208=CARTESIAN_POINT('Ctrl Pts',(188.893246872351,3.28785815834999,48.35));
#77209=CARTESIAN_POINT('',(188.893246872351,3.28785815834999,48.5));
#77210=CARTESIAN_POINT('Ctrl Pts',(189.405729992315,3.28560718894005,48.5));
#77211=CARTESIAN_POINT('Ctrl Pts',(189.405729992315,3.28560718894005,48.35));
#77212=CARTESIAN_POINT('Ctrl Pts',(189.302933139727,3.38690319657326,48.5));
#77213=CARTESIAN_POINT('Ctrl Pts',(189.302933139727,3.38690319657326,48.35));
#77214=CARTESIAN_POINT('Ctrl Pts',(189.149863643572,3.38690319657326,48.5));
#77215=CARTESIAN_POINT('Ctrl Pts',(189.149863643572,3.38690319657326,48.35));
#77216=CARTESIAN_POINT('',(189.405729992315,3.28560718894005,48.5));
#77217=CARTESIAN_POINT('Ctrl Pts',(189.405729992315,3.28560718894005,48.5));
#77218=CARTESIAN_POINT('Ctrl Pts',(189.302933139727,3.38690319657326,48.5));
#77219=CARTESIAN_POINT('Ctrl Pts',(189.149863643572,3.38690319657326,48.5));
#77220=CARTESIAN_POINT('',(189.405729992315,3.28560718894005,48.35));
#77221=CARTESIAN_POINT('',(189.405729992315,3.28560718894005,48.5));
#77222=CARTESIAN_POINT('Ctrl Pts',(189.405729992315,3.28560718894005,48.35));
#77223=CARTESIAN_POINT('Ctrl Pts',(189.302933139727,3.38690319657326,48.35));
#77224=CARTESIAN_POINT('Ctrl Pts',(189.149863643572,3.38690319657326,48.35));
#77225=CARTESIAN_POINT('Ctrl Pts',(189.508526546881,3.03574362397194,48.5));
#77226=CARTESIAN_POINT('Ctrl Pts',(189.508526546881,3.03574362397194,48.35));
#77227=CARTESIAN_POINT('Ctrl Pts',(189.508526546881,3.18431103229523,48.5));
#77228=CARTESIAN_POINT('Ctrl Pts',(189.508526546881,3.18431103229523,48.35));
#77229=CARTESIAN_POINT('Ctrl Pts',(189.405729992315,3.28560718894005,48.5));
#77230=CARTESIAN_POINT('Ctrl Pts',(189.405729992315,3.28560718894005,48.35));
#77231=CARTESIAN_POINT('',(189.508526546881,3.03574362397194,48.5));
#77232=CARTESIAN_POINT('Ctrl Pts',(189.508526546881,3.03574362397194,48.5));
#77233=CARTESIAN_POINT('Ctrl Pts',(189.508526546881,3.18431103229523,48.5));
#77234=CARTESIAN_POINT('Ctrl Pts',(189.405729992315,3.28560718894005,48.5));
#77235=CARTESIAN_POINT('',(189.508526546881,3.03574362397194,48.35));
#77236=CARTESIAN_POINT('',(189.508526546881,3.03574362397194,48.5));
#77237=CARTESIAN_POINT('Ctrl Pts',(189.508526546881,3.03574362397194,48.35));
#77238=CARTESIAN_POINT('Ctrl Pts',(189.508526546881,3.18431103229523,48.35));
#77239=CARTESIAN_POINT('Ctrl Pts',(189.405729992315,3.28560718894005,48.35));
#77240=CARTESIAN_POINT('Ctrl Pts',(189.408731384203,2.79488408565521,48.5));
#77241=CARTESIAN_POINT('Ctrl Pts',(189.408731384203,2.79488408565521,48.35));
#77242=CARTESIAN_POINT('Ctrl Pts',(189.508526546881,2.89317870140076,48.5));
#77243=CARTESIAN_POINT('Ctrl Pts',(189.508526546881,2.89317870140076,48.35));
#77244=CARTESIAN_POINT('Ctrl Pts',(189.508526546881,3.03574362397194,48.5));
#77245=CARTESIAN_POINT('Ctrl Pts',(189.508526546881,3.03574362397194,48.35));
#77246=CARTESIAN_POINT('',(189.408731384203,2.79488408565521,48.5));
#77247=CARTESIAN_POINT('Ctrl Pts',(189.408731384203,2.79488408565521,48.5));
#77248=CARTESIAN_POINT('Ctrl Pts',(189.508526546881,2.89317870140076,48.5));
#77249=CARTESIAN_POINT('Ctrl Pts',(189.508526546881,3.03574362397194,48.5));
#77250=CARTESIAN_POINT('',(189.408731384203,2.79488408565521,48.35));
#77251=CARTESIAN_POINT('',(189.408731384203,2.79488408565521,48.5));
#77252=CARTESIAN_POINT('Ctrl Pts',(189.408731384203,2.79488408565521,48.35));
#77253=CARTESIAN_POINT('Ctrl Pts',(189.508526546881,2.89317870140076,48.35));
#77254=CARTESIAN_POINT('Ctrl Pts',(189.508526546881,3.03574362397194,48.35));
#77255=CARTESIAN_POINT('Ctrl Pts',(189.152865035459,2.69658946990967,48.5));
#77256=CARTESIAN_POINT('Ctrl Pts',(189.152865035459,2.69658946990967,48.35));
#77257=CARTESIAN_POINT('Ctrl Pts',(189.308935923502,2.69658946990967,48.5));
#77258=CARTESIAN_POINT('Ctrl Pts',(189.308935923502,2.69658946990967,48.35));
#77259=CARTESIAN_POINT('Ctrl Pts',(189.408731384203,2.79488408565521,48.5));
#77260=CARTESIAN_POINT('Ctrl Pts',(189.408731384203,2.79488408565521,48.35));
#77261=CARTESIAN_POINT('',(189.152865035459,2.69658946990967,48.5));
#77262=CARTESIAN_POINT('Ctrl Pts',(189.152865035459,2.69658946990967,48.5));
#77263=CARTESIAN_POINT('Ctrl Pts',(189.308935923502,2.69658946990967,48.5));
#77264=CARTESIAN_POINT('Ctrl Pts',(189.408731384203,2.79488408565521,48.5));
#77265=CARTESIAN_POINT('',(189.152865035459,2.69658946990967,48.35));
#77266=CARTESIAN_POINT('',(189.152865035459,2.69658946990967,48.5));
#77267=CARTESIAN_POINT('Ctrl Pts',(189.152865035459,2.69658946990967,48.35));
#77268=CARTESIAN_POINT('Ctrl Pts',(189.308935923502,2.69658946990967,48.35));
#77269=CARTESIAN_POINT('Ctrl Pts',(189.408731384203,2.79488408565521,48.35));
#77270=CARTESIAN_POINT('Ctrl Pts',(188.891746325418,2.79563435912132,48.5));
#77271=CARTESIAN_POINT('Ctrl Pts',(188.891746325418,2.79563435912132,48.35));
#77272=CARTESIAN_POINT('Ctrl Pts',(188.992291910574,2.69658946990967,48.5));
#77273=CARTESIAN_POINT('Ctrl Pts',(188.992291910574,2.69658946990967,48.35));
#77274=CARTESIAN_POINT('Ctrl Pts',(189.152865035459,2.69658946990967,48.5));
#77275=CARTESIAN_POINT('Ctrl Pts',(189.152865035459,2.69658946990967,48.35));
#77276=CARTESIAN_POINT('',(188.891746325418,2.79563435912132,48.5));
#77277=CARTESIAN_POINT('Ctrl Pts',(188.891746325418,2.79563435912132,48.5));
#77278=CARTESIAN_POINT('Ctrl Pts',(188.992291910574,2.69658946990967,48.5));
#77279=CARTESIAN_POINT('Ctrl Pts',(189.152865035459,2.69658946990967,48.5));
#77280=CARTESIAN_POINT('',(188.891746325418,2.79563435912132,48.35));
#77281=CARTESIAN_POINT('',(188.891746325418,2.79563435912132,48.5));
#77282=CARTESIAN_POINT('Ctrl Pts',(188.891746325418,2.79563435912132,48.35));
#77283=CARTESIAN_POINT('Ctrl Pts',(188.992291910574,2.69658946990967,48.35));
#77284=CARTESIAN_POINT('Ctrl Pts',(189.152865035459,2.69658946990967,48.35));
#77285=CARTESIAN_POINT('Ctrl Pts',(188.791200591251,3.05075043439865,48.5));
#77286=CARTESIAN_POINT('Ctrl Pts',(188.791200591251,3.05075043439865,48.35));
#77287=CARTESIAN_POINT('Ctrl Pts',(188.791200591251,2.89467939734459,48.5));
#77288=CARTESIAN_POINT('Ctrl Pts',(188.791200591251,2.89467939734459,48.35));
#77289=CARTESIAN_POINT('Ctrl Pts',(188.891746325418,2.79563435912132,48.5));
#77290=CARTESIAN_POINT('Ctrl Pts',(188.891746325418,2.79563435912132,48.35));
#77291=CARTESIAN_POINT('',(188.791200591251,3.05075043439865,48.5));
#77292=CARTESIAN_POINT('Ctrl Pts',(188.791200591251,3.05075043439865,48.5));
#77293=CARTESIAN_POINT('Ctrl Pts',(188.791200591251,2.89467939734459,48.5));
#77294=CARTESIAN_POINT('Ctrl Pts',(188.891746325418,2.79563435912132,48.5));
#77295=CARTESIAN_POINT('',(188.791200591251,3.05075043439865,48.35));
#77296=CARTESIAN_POINT('',(188.791200591251,3.05075043439865,48.5));
#77297=CARTESIAN_POINT('Ctrl Pts',(188.791200591251,3.05075043439865,48.35));
#77298=CARTESIAN_POINT('Ctrl Pts',(188.791200591251,2.89467939734459,48.35));
#77299=CARTESIAN_POINT('Ctrl Pts',(188.891746325418,2.79563435912132,48.35));
#77300=CARTESIAN_POINT('Ctrl Pts',(188.893246872351,3.28785815834999,48.5));
#77301=CARTESIAN_POINT('Ctrl Pts',(188.893246872351,3.28785815834999,48.35));
#77302=CARTESIAN_POINT('Ctrl Pts',(188.791200591251,3.18881312012672,48.5));
#77303=CARTESIAN_POINT('Ctrl Pts',(188.791200591251,3.18881312012672,48.35));
#77304=CARTESIAN_POINT('Ctrl Pts',(188.791200591251,3.05075043439865,48.5));
#77305=CARTESIAN_POINT('Ctrl Pts',(188.791200591251,3.05075043439865,48.35));
#77306=CARTESIAN_POINT('Ctrl Pts',(188.893246872351,3.28785815834999,48.5));
#77307=CARTESIAN_POINT('Ctrl Pts',(188.791200591251,3.18881312012672,48.5));
#77308=CARTESIAN_POINT('Ctrl Pts',(188.791200591251,3.05075043439865,48.5));
#77309=CARTESIAN_POINT('Ctrl Pts',(188.893246872351,3.28785815834999,48.35));
#77310=CARTESIAN_POINT('Ctrl Pts',(188.791200591251,3.18881312012672,48.35));
#77311=CARTESIAN_POINT('Ctrl Pts',(188.791200591251,3.05075043439865,48.35));
#77312=CARTESIAN_POINT('Ctrl Pts',(189.14536155574,2.47598910331726,48.5));
#77313=CARTESIAN_POINT('Ctrl Pts',(189.14536155574,2.47598910331726,48.35));
#77314=CARTESIAN_POINT('Ctrl Pts',(188.954774959013,2.47598910331726,48.5));
#77315=CARTESIAN_POINT('Ctrl Pts',(188.954774959013,2.47598910331726,48.35));
#77316=CARTESIAN_POINT('Ctrl Pts',(188.82946796529,2.34993183612823,48.5));
#77317=CARTESIAN_POINT('Ctrl Pts',(188.82946796529,2.34993183612823,48.35));
#77318=CARTESIAN_POINT('',(189.14536155574,2.47598910331726,48.5));
#77319=CARTESIAN_POINT('',(188.82946796529,2.34993183612823,48.5));
#77320=CARTESIAN_POINT('Ctrl Pts',(189.14536155574,2.47598910331726,48.5));
#77321=CARTESIAN_POINT('Ctrl Pts',(188.954774959013,2.47598910331726,48.5));
#77322=CARTESIAN_POINT('Ctrl Pts',(188.82946796529,2.34993183612823,48.5));
#77323=CARTESIAN_POINT('',(189.14536155574,2.47598910331726,48.35));
#77324=CARTESIAN_POINT('',(189.14536155574,2.47598910331726,48.5));
#77325=CARTESIAN_POINT('',(188.82946796529,2.34993183612823,48.35));
#77326=CARTESIAN_POINT('Ctrl Pts',(189.14536155574,2.47598910331726,48.35));
#77327=CARTESIAN_POINT('Ctrl Pts',(188.954774959013,2.47598910331726,48.35));
#77328=CARTESIAN_POINT('Ctrl Pts',(188.82946796529,2.34993183612823,48.35));
#77329=CARTESIAN_POINT('',(188.82946796529,2.34993183612823,48.5));
#77330=CARTESIAN_POINT('Ctrl Pts',(189.470259172842,2.34843128919601,48.5));
#77331=CARTESIAN_POINT('Ctrl Pts',(189.470259172842,2.34843128919601,48.35));
#77332=CARTESIAN_POINT('Ctrl Pts',(189.340450240299,2.47598910331726,48.5));
#77333=CARTESIAN_POINT('Ctrl Pts',(189.340450240299,2.47598910331726,48.35));
#77334=CARTESIAN_POINT('Ctrl Pts',(189.14536155574,2.47598910331726,48.5));
#77335=CARTESIAN_POINT('Ctrl Pts',(189.14536155574,2.47598910331726,48.35));
#77336=CARTESIAN_POINT('',(189.470259172842,2.34843128919601,48.5));
#77337=CARTESIAN_POINT('Ctrl Pts',(189.470259172842,2.34843128919601,48.5));
#77338=CARTESIAN_POINT('Ctrl Pts',(189.340450240299,2.47598910331726,48.5));
#77339=CARTESIAN_POINT('Ctrl Pts',(189.14536155574,2.47598910331726,48.5));
#77340=CARTESIAN_POINT('',(189.470259172842,2.34843128919601,48.35));
#77341=CARTESIAN_POINT('',(189.470259172842,2.34843128919601,48.5));
#77342=CARTESIAN_POINT('Ctrl Pts',(189.470259172842,2.34843128919601,48.35));
#77343=CARTESIAN_POINT('Ctrl Pts',(189.340450240299,2.47598910331726,48.35));
#77344=CARTESIAN_POINT('Ctrl Pts',(189.14536155574,2.47598910331726,48.35));
#77345=CARTESIAN_POINT('Ctrl Pts',(189.600068254396,2.02578449249268,48.5));
#77346=CARTESIAN_POINT('Ctrl Pts',(189.600068254396,2.02578449249268,48.35));
#77347=CARTESIAN_POINT('Ctrl Pts',(189.600068254396,2.22087317705154,48.5));
#77348=CARTESIAN_POINT('Ctrl Pts',(189.600068254396,2.22087317705154,48.35));
#77349=CARTESIAN_POINT('Ctrl Pts',(189.470259172842,2.34843128919601,48.5));
#77350=CARTESIAN_POINT('Ctrl Pts',(189.470259172842,2.34843128919601,48.35));
#77351=CARTESIAN_POINT('',(189.600068254396,2.02578449249268,48.5));
#77352=CARTESIAN_POINT('Ctrl Pts',(189.600068254396,2.02578449249268,48.5));
#77353=CARTESIAN_POINT('Ctrl Pts',(189.600068254396,2.22087317705154,48.5));
#77354=CARTESIAN_POINT('Ctrl Pts',(189.470259172842,2.34843128919601,48.5));
#77355=CARTESIAN_POINT('',(189.600068254396,2.02578449249268,48.35));
#77356=CARTESIAN_POINT('',(189.600068254396,2.02578449249268,48.5));
#77357=CARTESIAN_POINT('Ctrl Pts',(189.600068254396,2.02578449249268,48.35));
#77358=CARTESIAN_POINT('Ctrl Pts',(189.600068254396,2.22087317705154,48.35));
#77359=CARTESIAN_POINT('Ctrl Pts',(189.470259172842,2.34843128919601,48.35));
#77360=CARTESIAN_POINT('Ctrl Pts',(189.474010987207,1.70914047956467,48.5));
#77361=CARTESIAN_POINT('Ctrl Pts',(189.474010987207,1.70914047956467,48.35));
#77362=CARTESIAN_POINT('Ctrl Pts',(189.600068254396,1.83369719982147,48.5));
#77363=CARTESIAN_POINT('Ctrl Pts',(189.600068254396,1.83369719982147,48.35));
#77364=CARTESIAN_POINT('Ctrl Pts',(189.600068254396,2.02578449249268,48.5));
#77365=CARTESIAN_POINT('Ctrl Pts',(189.600068254396,2.02578449249268,48.35));
#77366=CARTESIAN_POINT('',(189.474010987207,1.70914047956467,48.5));
#77367=CARTESIAN_POINT('Ctrl Pts',(189.474010987207,1.70914047956467,48.5));
#77368=CARTESIAN_POINT('Ctrl Pts',(189.600068254396,1.83369719982147,48.5));
#77369=CARTESIAN_POINT('Ctrl Pts',(189.600068254396,2.02578449249268,48.5));
#77370=CARTESIAN_POINT('',(189.474010987207,1.70914047956467,48.35));
#77371=CARTESIAN_POINT('',(189.474010987207,1.70914047956467,48.5));
#77372=CARTESIAN_POINT('Ctrl Pts',(189.474010987207,1.70914047956467,48.35));
#77373=CARTESIAN_POINT('Ctrl Pts',(189.600068254396,1.83369719982147,48.35));
#77374=CARTESIAN_POINT('Ctrl Pts',(189.600068254396,2.02578449249268,48.35));
#77375=CARTESIAN_POINT('Ctrl Pts',(189.154365582392,1.58458405733109,48.5));
#77376=CARTESIAN_POINT('Ctrl Pts',(189.154365582392,1.58458405733109,48.35));
#77377=CARTESIAN_POINT('Ctrl Pts',(189.347953720018,1.58458405733109,48.5));
#77378=CARTESIAN_POINT('Ctrl Pts',(189.347953720018,1.58458405733109,48.35));
#77379=CARTESIAN_POINT('Ctrl Pts',(189.474010987207,1.70914047956467,48.5));
#77380=CARTESIAN_POINT('Ctrl Pts',(189.474010987207,1.70914047956467,48.35));
#77381=CARTESIAN_POINT('',(189.154365582392,1.58458405733109,48.5));
#77382=CARTESIAN_POINT('Ctrl Pts',(189.154365582392,1.58458405733109,48.5));
#77383=CARTESIAN_POINT('Ctrl Pts',(189.347953720018,1.58458405733109,48.5));
#77384=CARTESIAN_POINT('Ctrl Pts',(189.474010987207,1.70914047956467,48.5));
#77385=CARTESIAN_POINT('',(189.154365582392,1.58458405733109,48.35));
#77386=CARTESIAN_POINT('',(189.154365582392,1.58458405733109,48.5));
#77387=CARTESIAN_POINT('Ctrl Pts',(189.154365582392,1.58458405733109,48.35));
#77388=CARTESIAN_POINT('Ctrl Pts',(189.347953720018,1.58458405733109,48.35));
#77389=CARTESIAN_POINT('Ctrl Pts',(189.474010987207,1.70914047956467,48.35));
#77390=CARTESIAN_POINT('Ctrl Pts',(188.921759946272,1.64386087656021,48.5));
#77391=CARTESIAN_POINT('Ctrl Pts',(188.921759946272,1.64386087656021,48.35));
#77392=CARTESIAN_POINT('Ctrl Pts',(189.029809011146,1.58458405733109,48.5));
#77393=CARTESIAN_POINT('Ctrl Pts',(189.029809011146,1.58458405733109,48.35));
#77394=CARTESIAN_POINT('Ctrl Pts',(189.154365582392,1.58458405733109,48.5));
#77395=CARTESIAN_POINT('Ctrl Pts',(189.154365582392,1.58458405733109,48.35));
#77396=CARTESIAN_POINT('',(188.921759946272,1.64386087656021,48.5));
#77397=CARTESIAN_POINT('Ctrl Pts',(188.921759946272,1.64386087656021,48.5));
#77398=CARTESIAN_POINT('Ctrl Pts',(189.029809011146,1.58458405733109,48.5));
#77399=CARTESIAN_POINT('Ctrl Pts',(189.154365582392,1.58458405733109,48.5));
#77400=CARTESIAN_POINT('',(188.921759946272,1.64386087656021,48.35));
#77401=CARTESIAN_POINT('',(188.921759946272,1.64386087656021,48.5));
#77402=CARTESIAN_POINT('Ctrl Pts',(188.921759946272,1.64386087656021,48.35));
#77403=CARTESIAN_POINT('Ctrl Pts',(189.029809011146,1.58458405733109,48.35));
#77404=CARTESIAN_POINT('Ctrl Pts',(189.154365582392,1.58458405733109,48.35));
#77405=CARTESIAN_POINT('Ctrl Pts',(188.758935851976,1.8111869096756,48.5));
#77406=CARTESIAN_POINT('Ctrl Pts',(188.758935851976,1.8111869096756,48.35));
#77407=CARTESIAN_POINT('Ctrl Pts',(188.813710732386,1.70313799381256,48.5));
#77408=CARTESIAN_POINT('Ctrl Pts',(188.813710732386,1.70313799381256,48.35));
#77409=CARTESIAN_POINT('Ctrl Pts',(188.921759946272,1.64386087656021,48.5));
#77410=CARTESIAN_POINT('Ctrl Pts',(188.921759946272,1.64386087656021,48.35));
#77411=CARTESIAN_POINT('',(188.758935851976,1.8111869096756,48.5));
#77412=CARTESIAN_POINT('Ctrl Pts',(188.758935851976,1.8111869096756,48.5));
#77413=CARTESIAN_POINT('Ctrl Pts',(188.813710732386,1.70313799381256,48.5));
#77414=CARTESIAN_POINT('Ctrl Pts',(188.921759946272,1.64386087656021,48.5));
#77415=CARTESIAN_POINT('',(188.758935851976,1.8111869096756,48.35));
#77416=CARTESIAN_POINT('',(188.758935851976,1.8111869096756,48.5));
#77417=CARTESIAN_POINT('Ctrl Pts',(188.758935851976,1.8111869096756,48.35));
#77418=CARTESIAN_POINT('Ctrl Pts',(188.813710732386,1.70313799381256,48.35));
#77419=CARTESIAN_POINT('Ctrl Pts',(188.921759946272,1.64386087656021,48.35));
#77420=CARTESIAN_POINT('Ctrl Pts',(188.704160971567,2.03478866815567,48.5));
#77421=CARTESIAN_POINT('Ctrl Pts',(188.704160971567,2.03478866815567,48.35));
#77422=CARTESIAN_POINT('Ctrl Pts',(188.704160971567,1.91923612356186,48.5));
#77423=CARTESIAN_POINT('Ctrl Pts',(188.704160971567,1.91923612356186,48.35));
#77424=CARTESIAN_POINT('Ctrl Pts',(188.758935851976,1.8111869096756,48.5));
#77425=CARTESIAN_POINT('Ctrl Pts',(188.758935851976,1.8111869096756,48.35));
#77426=CARTESIAN_POINT('',(188.704160971567,2.03478866815567,48.5));
#77427=CARTESIAN_POINT('Ctrl Pts',(188.704160971567,2.03478866815567,48.5));
#77428=CARTESIAN_POINT('Ctrl Pts',(188.704160971567,1.91923612356186,48.5));
#77429=CARTESIAN_POINT('Ctrl Pts',(188.758935851976,1.8111869096756,48.5));
#77430=CARTESIAN_POINT('',(188.704160971567,2.03478866815567,48.35));
#77431=CARTESIAN_POINT('',(188.704160971567,2.03478866815567,48.5));
#77432=CARTESIAN_POINT('Ctrl Pts',(188.704160971567,2.03478866815567,48.35));
#77433=CARTESIAN_POINT('Ctrl Pts',(188.704160971567,1.91923612356186,48.35));
#77434=CARTESIAN_POINT('Ctrl Pts',(188.758935851976,1.8111869096756,48.35));
#77435=CARTESIAN_POINT('Ctrl Pts',(188.82946796529,2.34993183612823,48.5));
#77436=CARTESIAN_POINT('Ctrl Pts',(188.82946796529,2.34993183612823,48.35));
#77437=CARTESIAN_POINT('Ctrl Pts',(188.704160971567,2.22387456893921,48.5));
#77438=CARTESIAN_POINT('Ctrl Pts',(188.704160971567,2.22387456893921,48.35));
#77439=CARTESIAN_POINT('Ctrl Pts',(188.704160971567,2.03478866815567,48.5));
#77440=CARTESIAN_POINT('Ctrl Pts',(188.704160971567,2.03478866815567,48.35));
#77441=CARTESIAN_POINT('Ctrl Pts',(188.82946796529,2.34993183612823,48.5));
#77442=CARTESIAN_POINT('Ctrl Pts',(188.704160971567,2.22387456893921,48.5));
#77443=CARTESIAN_POINT('Ctrl Pts',(188.704160971567,2.03478866815567,48.5));
#77444=CARTESIAN_POINT('Ctrl Pts',(188.82946796529,2.34993183612823,48.35));
#77445=CARTESIAN_POINT('Ctrl Pts',(188.704160971567,2.22387456893921,48.35));
#77446=CARTESIAN_POINT('Ctrl Pts',(188.704160971567,2.03478866815567,48.35));
#77447=CARTESIAN_POINT('Ctrl Pts',(188.426534755155,2.03628921508789,48.5));
#77448=CARTESIAN_POINT('Ctrl Pts',(188.426534755155,2.03628921508789,48.35));
#77449=CARTESIAN_POINT('Ctrl Pts',(188.426534755155,2.25088679790497,48.5));
#77450=CARTESIAN_POINT('Ctrl Pts',(188.426534755155,2.25088679790497,48.35));
#77451=CARTESIAN_POINT('Ctrl Pts',(188.535334242508,2.39570268988609,48.5));
#77452=CARTESIAN_POINT('Ctrl Pts',(188.535334242508,2.39570268988609,48.35));
#77453=CARTESIAN_POINT('',(188.426534755155,2.03628921508789,48.5));
#77454=CARTESIAN_POINT('',(188.535334242508,2.39570268988609,48.5));
#77455=CARTESIAN_POINT('Ctrl Pts',(188.426534755155,2.03628921508789,48.5));
#77456=CARTESIAN_POINT('Ctrl Pts',(188.426534755155,2.25088679790497,48.5));
#77457=CARTESIAN_POINT('Ctrl Pts',(188.535334242508,2.39570268988609,48.5));
#77458=CARTESIAN_POINT('',(188.426534755155,2.03628921508789,48.35));
#77459=CARTESIAN_POINT('',(188.426534755155,2.03628921508789,48.5));
#77460=CARTESIAN_POINT('',(188.535334242508,2.39570268988609,48.35));
#77461=CARTESIAN_POINT('Ctrl Pts',(188.426534755155,2.03628921508789,48.35));
#77462=CARTESIAN_POINT('Ctrl Pts',(188.426534755155,2.25088679790497,48.35));
#77463=CARTESIAN_POINT('Ctrl Pts',(188.535334242508,2.39570268988609,48.35));
#77464=CARTESIAN_POINT('',(188.535334242508,2.39570268988609,48.5));
#77465=CARTESIAN_POINT('Ctrl Pts',(188.626125527546,1.55532056093216,48.5));
#77466=CARTESIAN_POINT('Ctrl Pts',(188.626125527546,1.55532056093216,48.35));
#77467=CARTESIAN_POINT('Ctrl Pts',(188.426534755155,1.74815827608109,48.5));
#77468=CARTESIAN_POINT('Ctrl Pts',(188.426534755155,1.74815827608109,48.35));
#77469=CARTESIAN_POINT('Ctrl Pts',(188.426534755155,2.03628921508789,48.5));
#77470=CARTESIAN_POINT('Ctrl Pts',(188.426534755155,2.03628921508789,48.35));
#77471=CARTESIAN_POINT('',(188.626125527546,1.55532056093216,48.5));
#77472=CARTESIAN_POINT('Ctrl Pts',(188.626125527546,1.55532056093216,48.5));
#77473=CARTESIAN_POINT('Ctrl Pts',(188.426534755155,1.74815827608109,48.5));
#77474=CARTESIAN_POINT('Ctrl Pts',(188.426534755155,2.03628921508789,48.5));
#77475=CARTESIAN_POINT('',(188.626125527546,1.55532056093216,48.35));
#77476=CARTESIAN_POINT('',(188.626125527546,1.55532056093216,48.5));
#77477=CARTESIAN_POINT('Ctrl Pts',(188.626125527546,1.55532056093216,48.35));
#77478=CARTESIAN_POINT('Ctrl Pts',(188.426534755155,1.74815827608109,48.35));
#77479=CARTESIAN_POINT('Ctrl Pts',(188.426534755155,2.03628921508789,48.35));
#77480=CARTESIAN_POINT('Ctrl Pts',(189.151364190504,1.36248314380646,48.5));
#77481=CARTESIAN_POINT('Ctrl Pts',(189.151364190504,1.36248314380646,48.35));
#77482=CARTESIAN_POINT('Ctrl Pts',(188.825716299936,1.36248314380646,48.5));
#77483=CARTESIAN_POINT('Ctrl Pts',(188.825716299936,1.36248314380646,48.35));
#77484=CARTESIAN_POINT('Ctrl Pts',(188.626125527546,1.55532056093216,48.5));
#77485=CARTESIAN_POINT('Ctrl Pts',(188.626125527546,1.55532056093216,48.35));
#77486=CARTESIAN_POINT('',(189.151364190504,1.36248314380646,48.5));
#77487=CARTESIAN_POINT('Ctrl Pts',(189.151364190504,1.36248314380646,48.5));
#77488=CARTESIAN_POINT('Ctrl Pts',(188.825716299936,1.36248314380646,48.5));
#77489=CARTESIAN_POINT('Ctrl Pts',(188.626125527546,1.55532056093216,48.5));
#77490=CARTESIAN_POINT('',(189.151364190504,1.36248314380646,48.35));
#77491=CARTESIAN_POINT('',(189.151364190504,1.36248314380646,48.5));
#77492=CARTESIAN_POINT('Ctrl Pts',(189.151364190504,1.36248314380646,48.35));
#77493=CARTESIAN_POINT('Ctrl Pts',(188.825716299936,1.36248314380646,48.35));
#77494=CARTESIAN_POINT('Ctrl Pts',(188.626125527546,1.55532056093216,48.35));
#77495=CARTESIAN_POINT('Ctrl Pts',(189.676603002474,1.55457043647766,48.5));
#77496=CARTESIAN_POINT('Ctrl Pts',(189.676603002474,1.55457043647766,48.35));
#77497=CARTESIAN_POINT('Ctrl Pts',(189.477012379095,1.36248314380646,48.5));
#77498=CARTESIAN_POINT('Ctrl Pts',(189.477012379095,1.36248314380646,48.35));
#77499=CARTESIAN_POINT('Ctrl Pts',(189.151364190504,1.36248314380646,48.5));
#77500=CARTESIAN_POINT('Ctrl Pts',(189.151364190504,1.36248314380646,48.35));
#77501=CARTESIAN_POINT('',(189.676603002474,1.55457043647766,48.5));
#77502=CARTESIAN_POINT('Ctrl Pts',(189.676603002474,1.55457043647766,48.5));
#77503=CARTESIAN_POINT('Ctrl Pts',(189.477012379095,1.36248314380646,48.5));
#77504=CARTESIAN_POINT('Ctrl Pts',(189.151364190504,1.36248314380646,48.5));
#77505=CARTESIAN_POINT('',(189.676603002474,1.55457043647766,48.35));
#77506=CARTESIAN_POINT('',(189.676603002474,1.55457043647766,48.5));
#77507=CARTESIAN_POINT('Ctrl Pts',(189.676603002474,1.55457043647766,48.35));
#77508=CARTESIAN_POINT('Ctrl Pts',(189.477012379095,1.36248314380646,48.35));
#77509=CARTESIAN_POINT('Ctrl Pts',(189.151364190504,1.36248314380646,48.35));
#77510=CARTESIAN_POINT('Ctrl Pts',(189.876193625852,2.02878588438034,48.5));
#77511=CARTESIAN_POINT('Ctrl Pts',(189.876193625852,2.02878588438034,48.35));
#77512=CARTESIAN_POINT('Ctrl Pts',(189.876193625852,1.74665772914886,48.5));
#77513=CARTESIAN_POINT('Ctrl Pts',(189.876193625852,1.74665772914886,48.35));
#77514=CARTESIAN_POINT('Ctrl Pts',(189.676603002474,1.55457043647766,48.5));
#77515=CARTESIAN_POINT('Ctrl Pts',(189.676603002474,1.55457043647766,48.35));
#77516=CARTESIAN_POINT('',(189.876193625852,2.02878588438034,48.5));
#77517=CARTESIAN_POINT('Ctrl Pts',(189.876193625852,2.02878588438034,48.5));
#77518=CARTESIAN_POINT('Ctrl Pts',(189.876193625852,1.74665772914886,48.5));
#77519=CARTESIAN_POINT('Ctrl Pts',(189.676603002474,1.55457043647766,48.5));
#77520=CARTESIAN_POINT('',(189.876193625852,2.02878588438034,48.35));
#77521=CARTESIAN_POINT('',(189.876193625852,2.02878588438034,48.5));
#77522=CARTESIAN_POINT('Ctrl Pts',(189.876193625852,2.02878588438034,48.35));
#77523=CARTESIAN_POINT('Ctrl Pts',(189.876193625852,1.74665772914886,48.35));
#77524=CARTESIAN_POINT('Ctrl Pts',(189.676603002474,1.55457043647766,48.35));
#77525=CARTESIAN_POINT('Ctrl Pts',(189.770395679399,2.37994545698166,48.5));
#77526=CARTESIAN_POINT('Ctrl Pts',(189.770395679399,2.37994545698166,48.35));
#77527=CARTESIAN_POINT('Ctrl Pts',(189.876193625852,2.2328787446022,48.5));
#77528=CARTESIAN_POINT('Ctrl Pts',(189.876193625852,2.2328787446022,48.35));
#77529=CARTESIAN_POINT('Ctrl Pts',(189.876193625852,2.02878588438034,48.5));
#77530=CARTESIAN_POINT('Ctrl Pts',(189.876193625852,2.02878588438034,48.35));
#77531=CARTESIAN_POINT('',(189.770395679399,2.37994545698166,48.5));
#77532=CARTESIAN_POINT('Ctrl Pts',(189.770395679399,2.37994545698166,48.5));
#77533=CARTESIAN_POINT('Ctrl Pts',(189.876193625852,2.2328787446022,48.5));
#77534=CARTESIAN_POINT('Ctrl Pts',(189.876193625852,2.02878588438034,48.5));
#77535=CARTESIAN_POINT('',(189.770395679399,2.37994545698166,48.35));
#77536=CARTESIAN_POINT('',(189.770395679399,2.37994545698166,48.5));
#77537=CARTESIAN_POINT('Ctrl Pts',(189.770395679399,2.37994545698166,48.35));
#77538=CARTESIAN_POINT('Ctrl Pts',(189.876193625852,2.2328787446022,48.35));
#77539=CARTESIAN_POINT('Ctrl Pts',(189.876193625852,2.02878588438034,48.35));
#77540=CARTESIAN_POINT('Ctrl Pts',(189.462005419657,2.59304249286652,48.5));
#77541=CARTESIAN_POINT('Ctrl Pts',(189.462005419657,2.59304249286652,48.35));
#77542=CARTESIAN_POINT('Ctrl Pts',(189.664597434923,2.52701246738434,48.5));
#77543=CARTESIAN_POINT('Ctrl Pts',(189.664597434923,2.52701246738434,48.35));
#77544=CARTESIAN_POINT('Ctrl Pts',(189.770395679399,2.37994545698166,48.5));
#77545=CARTESIAN_POINT('Ctrl Pts',(189.770395679399,2.37994545698166,48.35));
#77546=CARTESIAN_POINT('',(189.462005419657,2.59304249286652,48.5));
#77547=CARTESIAN_POINT('Ctrl Pts',(189.462005419657,2.59304249286652,48.5));
#77548=CARTESIAN_POINT('Ctrl Pts',(189.664597434923,2.52701246738434,48.5));
#77549=CARTESIAN_POINT('Ctrl Pts',(189.770395679399,2.37994545698166,48.5));
#77550=CARTESIAN_POINT('',(189.462005419657,2.59304249286652,48.35));
#77551=CARTESIAN_POINT('',(189.462005419657,2.59304249286652,48.5));
#77552=CARTESIAN_POINT('Ctrl Pts',(189.462005419657,2.59304249286652,48.35));
#77553=CARTESIAN_POINT('Ctrl Pts',(189.664597434923,2.52701246738434,48.35));
#77554=CARTESIAN_POINT('Ctrl Pts',(189.770395679399,2.37994545698166,48.35));
#77555=CARTESIAN_POINT('Ctrl Pts',(189.705866200849,2.76787185668945,48.5));
#77556=CARTESIAN_POINT('Ctrl Pts',(189.705866200849,2.76787185668945,48.35));
#77557=CARTESIAN_POINT('Ctrl Pts',(189.625579638407,2.65457028150558,48.5));
#77558=CARTESIAN_POINT('Ctrl Pts',(189.625579638407,2.65457028150558,48.35));
#77559=CARTESIAN_POINT('Ctrl Pts',(189.462005419657,2.59304249286652,48.5));
#77560=CARTESIAN_POINT('Ctrl Pts',(189.462005419657,2.59304249286652,48.35));
#77561=CARTESIAN_POINT('',(189.705866200849,2.76787185668945,48.5));
#77562=CARTESIAN_POINT('Ctrl Pts',(189.705866200849,2.76787185668945,48.5));
#77563=CARTESIAN_POINT('Ctrl Pts',(189.625579638407,2.65457028150558,48.5));
#77564=CARTESIAN_POINT('Ctrl Pts',(189.462005419657,2.59304249286652,48.5));
#77565=CARTESIAN_POINT('',(189.705866200849,2.76787185668945,48.35));
#77566=CARTESIAN_POINT('',(189.705866200849,2.76787185668945,48.5));
#77567=CARTESIAN_POINT('Ctrl Pts',(189.705866200849,2.76787185668945,48.35));
#77568=CARTESIAN_POINT('Ctrl Pts',(189.625579638407,2.65457028150558,48.35));
#77569=CARTESIAN_POINT('Ctrl Pts',(189.462005419657,2.59304249286652,48.35));
#77570=CARTESIAN_POINT('Ctrl Pts',(189.786152763292,3.03424292802811,48.5));
#77571=CARTESIAN_POINT('Ctrl Pts',(189.786152763292,3.03424292802811,48.35));
#77572=CARTESIAN_POINT('Ctrl Pts',(189.786152763292,2.88117328286171,48.5));
#77573=CARTESIAN_POINT('Ctrl Pts',(189.786152763292,2.88117328286171,48.35));
#77574=CARTESIAN_POINT('Ctrl Pts',(189.705866200849,2.76787185668945,48.5));
#77575=CARTESIAN_POINT('Ctrl Pts',(189.705866200849,2.76787185668945,48.35));
#77576=CARTESIAN_POINT('',(189.786152763292,3.03424292802811,48.5));
#77577=CARTESIAN_POINT('Ctrl Pts',(189.786152763292,3.03424292802811,48.5));
#77578=CARTESIAN_POINT('Ctrl Pts',(189.786152763292,2.88117328286171,48.5));
#77579=CARTESIAN_POINT('Ctrl Pts',(189.705866200849,2.76787185668945,48.5));
#77580=CARTESIAN_POINT('',(189.786152763292,3.03424292802811,48.35));
#77581=CARTESIAN_POINT('',(189.786152763292,3.03424292802811,48.5));
#77582=CARTESIAN_POINT('Ctrl Pts',(189.786152763292,3.03424292802811,48.35));
#77583=CARTESIAN_POINT('Ctrl Pts',(189.786152763292,2.88117328286171,48.35));
#77584=CARTESIAN_POINT('Ctrl Pts',(189.705866200849,2.76787185668945,48.35));
#77585=CARTESIAN_POINT('Ctrl Pts',(189.610572976992,3.4416780769825,48.5));
#77586=CARTESIAN_POINT('Ctrl Pts',(189.610572976992,3.4416780769825,48.35));
#77587=CARTESIAN_POINT('Ctrl Pts',(189.786152763292,3.27435204386711,48.5));
#77588=CARTESIAN_POINT('Ctrl Pts',(189.786152763292,3.27435204386711,48.35));
#77589=CARTESIAN_POINT('Ctrl Pts',(189.786152763292,3.03424292802811,48.5));
#77590=CARTESIAN_POINT('Ctrl Pts',(189.786152763292,3.03424292802811,48.35));
#77591=CARTESIAN_POINT('',(189.610572976992,3.4416780769825,48.5));
#77592=CARTESIAN_POINT('Ctrl Pts',(189.610572976992,3.4416780769825,48.5));
#77593=CARTESIAN_POINT('Ctrl Pts',(189.786152763292,3.27435204386711,48.5));
#77594=CARTESIAN_POINT('Ctrl Pts',(189.786152763292,3.03424292802811,48.5));
#77595=CARTESIAN_POINT('',(189.610572976992,3.4416780769825,48.35));
#77596=CARTESIAN_POINT('',(189.610572976992,3.4416780769825,48.5));
#77597=CARTESIAN_POINT('Ctrl Pts',(189.610572976992,3.4416780769825,48.35));
#77598=CARTESIAN_POINT('Ctrl Pts',(189.786152763292,3.27435204386711,48.35));
#77599=CARTESIAN_POINT('Ctrl Pts',(189.786152763292,3.03424292802811,48.35));
#77600=CARTESIAN_POINT('Ctrl Pts',(189.146862251684,3.60900411009789,48.5));
#77601=CARTESIAN_POINT('Ctrl Pts',(189.146862251684,3.60900411009789,48.35));
#77602=CARTESIAN_POINT('Ctrl Pts',(189.434993190691,3.60900411009789,48.5));
#77603=CARTESIAN_POINT('Ctrl Pts',(189.434993190691,3.60900411009789,48.35));
#77604=CARTESIAN_POINT('Ctrl Pts',(189.610572976992,3.4416780769825,48.5));
#77605=CARTESIAN_POINT('Ctrl Pts',(189.610572976992,3.4416780769825,48.35));
#77606=CARTESIAN_POINT('',(189.146862251684,3.60900411009789,48.5));
#77607=CARTESIAN_POINT('Ctrl Pts',(189.146862251684,3.60900411009789,48.5));
#77608=CARTESIAN_POINT('Ctrl Pts',(189.434993190691,3.60900411009789,48.5));
#77609=CARTESIAN_POINT('Ctrl Pts',(189.610572976992,3.4416780769825,48.5));
#77610=CARTESIAN_POINT('',(189.146862251684,3.60900411009789,48.35));
#77611=CARTESIAN_POINT('',(189.146862251684,3.60900411009789,48.5));
#77612=CARTESIAN_POINT('Ctrl Pts',(189.146862251684,3.60900411009789,48.35));
#77613=CARTESIAN_POINT('Ctrl Pts',(189.434993190691,3.60900411009789,48.35));
#77614=CARTESIAN_POINT('Ctrl Pts',(189.610572976992,3.4416780769825,48.35));
#77615=CARTESIAN_POINT('Ctrl Pts',(188.687653465196,3.44542974233627,48.5));
#77616=CARTESIAN_POINT('Ctrl Pts',(188.687653465196,3.44542974233627,48.35));
#77617=CARTESIAN_POINT('Ctrl Pts',(188.860231859609,3.60900411009789,48.5));
#77618=CARTESIAN_POINT('Ctrl Pts',(188.860231859609,3.60900411009789,48.35));
#77619=CARTESIAN_POINT('Ctrl Pts',(189.146862251684,3.60900411009789,48.5));
#77620=CARTESIAN_POINT('Ctrl Pts',(189.146862251684,3.60900411009789,48.35));
#77621=CARTESIAN_POINT('',(188.687653465196,3.44542974233627,48.5));
#77622=CARTESIAN_POINT('Ctrl Pts',(188.687653465196,3.44542974233627,48.5));
#77623=CARTESIAN_POINT('Ctrl Pts',(188.860231859609,3.60900411009789,48.5));
#77624=CARTESIAN_POINT('Ctrl Pts',(189.146862251684,3.60900411009789,48.5));
#77625=CARTESIAN_POINT('',(188.687653465196,3.44542974233627,48.35));
#77626=CARTESIAN_POINT('',(188.687653465196,3.44542974233627,48.5));
#77627=CARTESIAN_POINT('Ctrl Pts',(188.687653465196,3.44542974233627,48.35));
#77628=CARTESIAN_POINT('Ctrl Pts',(188.860231859609,3.60900411009789,48.35));
#77629=CARTESIAN_POINT('Ctrl Pts',(189.146862251684,3.60900411009789,48.35));
#77630=CARTESIAN_POINT('Ctrl Pts',(188.515075070783,3.04174625873566,48.5));
#77631=CARTESIAN_POINT('Ctrl Pts',(188.515075070783,3.04174625873566,48.35));
#77632=CARTESIAN_POINT('Ctrl Pts',(188.515075070783,3.28185537457466,48.5));
#77633=CARTESIAN_POINT('Ctrl Pts',(188.515075070783,3.28185537457466,48.35));
#77634=CARTESIAN_POINT('Ctrl Pts',(188.687653465196,3.44542974233627,48.5));
#77635=CARTESIAN_POINT('Ctrl Pts',(188.687653465196,3.44542974233627,48.35));
#77636=CARTESIAN_POINT('',(188.515075070783,3.04174625873566,48.5));
#77637=CARTESIAN_POINT('Ctrl Pts',(188.515075070783,3.04174625873566,48.5));
#77638=CARTESIAN_POINT('Ctrl Pts',(188.515075070783,3.28185537457466,48.5));
#77639=CARTESIAN_POINT('Ctrl Pts',(188.687653465196,3.44542974233627,48.5));
#77640=CARTESIAN_POINT('',(188.515075070783,3.04174625873566,48.35));
#77641=CARTESIAN_POINT('',(188.515075070783,3.04174625873566,48.5));
#77642=CARTESIAN_POINT('Ctrl Pts',(188.515075070783,3.04174625873566,48.35));
#77643=CARTESIAN_POINT('Ctrl Pts',(188.515075070783,3.28185537457466,48.35));
#77644=CARTESIAN_POINT('Ctrl Pts',(188.687653465196,3.44542974233627,48.35));
#77645=CARTESIAN_POINT('Ctrl Pts',(188.596111906692,2.76862213015556,48.5));
#77646=CARTESIAN_POINT('Ctrl Pts',(188.596111906692,2.76862213015556,48.35));
#77647=CARTESIAN_POINT('Ctrl Pts',(188.515075070783,2.88267397880554,48.5));
#77648=CARTESIAN_POINT('Ctrl Pts',(188.515075070783,2.88267397880554,48.35));
#77649=CARTESIAN_POINT('Ctrl Pts',(188.515075070783,3.04174625873566,48.5));
#77650=CARTESIAN_POINT('Ctrl Pts',(188.515075070783,3.04174625873566,48.35));
#77651=CARTESIAN_POINT('',(188.596111906692,2.76862213015556,48.5));
#77652=CARTESIAN_POINT('Ctrl Pts',(188.596111906692,2.76862213015556,48.5));
#77653=CARTESIAN_POINT('Ctrl Pts',(188.515075070783,2.88267397880554,48.5));
#77654=CARTESIAN_POINT('Ctrl Pts',(188.515075070783,3.04174625873566,48.5));
#77655=CARTESIAN_POINT('',(188.596111906692,2.76862213015556,48.35));
#77656=CARTESIAN_POINT('',(188.596111906692,2.76862213015556,48.5));
#77657=CARTESIAN_POINT('Ctrl Pts',(188.596111906692,2.76862213015556,48.35));
#77658=CARTESIAN_POINT('Ctrl Pts',(188.515075070783,2.88267397880554,48.35));
#77659=CARTESIAN_POINT('Ctrl Pts',(188.515075070783,3.04174625873566,48.35));
#77660=CARTESIAN_POINT('Ctrl Pts',(188.845225049183,2.59304249286652,48.5));
#77661=CARTESIAN_POINT('Ctrl Pts',(188.845225049183,2.59304249286652,48.35));
#77662=CARTESIAN_POINT('Ctrl Pts',(188.677148742601,2.65457028150558,48.5));
#77663=CARTESIAN_POINT('Ctrl Pts',(188.677148742601,2.65457028150558,48.35));
#77664=CARTESIAN_POINT('Ctrl Pts',(188.596111906692,2.76862213015556,48.5));
#77665=CARTESIAN_POINT('Ctrl Pts',(188.596111906692,2.76862213015556,48.35));
#77666=CARTESIAN_POINT('',(188.845225049183,2.59304249286652,48.5));
#77667=CARTESIAN_POINT('Ctrl Pts',(188.845225049183,2.59304249286652,48.5));
#77668=CARTESIAN_POINT('Ctrl Pts',(188.677148742601,2.65457028150558,48.5));
#77669=CARTESIAN_POINT('Ctrl Pts',(188.596111906692,2.76862213015556,48.5));
#77670=CARTESIAN_POINT('',(188.845225049183,2.59304249286652,48.35));
#77671=CARTESIAN_POINT('',(188.845225049183,2.59304249286652,48.5));
#77672=CARTESIAN_POINT('Ctrl Pts',(188.845225049183,2.59304249286652,48.35));
#77673=CARTESIAN_POINT('Ctrl Pts',(188.677148742601,2.65457028150558,48.35));
#77674=CARTESIAN_POINT('Ctrl Pts',(188.596111906692,2.76862213015556,48.35));
#77675=CARTESIAN_POINT('Ctrl Pts',(188.535334242508,2.39570268988609,48.5));
#77676=CARTESIAN_POINT('Ctrl Pts',(188.535334242508,2.39570268988609,48.35));
#77677=CARTESIAN_POINT('Ctrl Pts',(188.64413372986,2.54051858186722,48.5));
#77678=CARTESIAN_POINT('Ctrl Pts',(188.64413372986,2.54051858186722,48.35));
#77679=CARTESIAN_POINT('Ctrl Pts',(188.845225049183,2.59304249286652,48.5));
#77680=CARTESIAN_POINT('Ctrl Pts',(188.845225049183,2.59304249286652,48.35));
#77681=CARTESIAN_POINT('Ctrl Pts',(188.535334242508,2.39570268988609,48.5));
#77682=CARTESIAN_POINT('Ctrl Pts',(188.64413372986,2.54051858186722,48.5));
#77683=CARTESIAN_POINT('Ctrl Pts',(188.845225049183,2.59304249286652,48.5));
#77684=CARTESIAN_POINT('Ctrl Pts',(188.535334242508,2.39570268988609,48.35));
#77685=CARTESIAN_POINT('Ctrl Pts',(188.64413372986,2.54051858186722,48.35));
#77686=CARTESIAN_POINT('Ctrl Pts',(188.845225049183,2.59304249286652,48.35));
#77687=CARTESIAN_POINT('Origin',(189.99999977462,2.48574362695217,48.35));
#77688=CARTESIAN_POINT('Origin',(0.,8.,48.5));
#77689=CARTESIAN_POINT('Origin',(0.,8.,48.5));
#77690=CARTESIAN_POINT('Origin',(0.,8.,48.5));
#77691=CARTESIAN_POINT('Ctrl Pts',(180.842633068562,3.38540250062943,48.5));
#77692=CARTESIAN_POINT('Ctrl Pts',(180.842633068562,3.38540250062943,48.35));
#77693=CARTESIAN_POINT('Ctrl Pts',(180.656548261642,3.38540250062943,48.5));
#77694=CARTESIAN_POINT('Ctrl Pts',(180.656548261642,3.38540250062943,48.35));
#77695=CARTESIAN_POINT('Ctrl Pts',(180.545497953892,3.22783091664314,48.5));
#77696=CARTESIAN_POINT('Ctrl Pts',(180.545497953892,3.22783091664314,48.35));
#77697=CARTESIAN_POINT('',(180.842633068562,3.38540250062943,48.5));
#77698=CARTESIAN_POINT('',(180.545497953892,3.22783091664314,48.5));
#77699=CARTESIAN_POINT('Ctrl Pts',(180.842633068562,3.38540250062943,48.5));
#77700=CARTESIAN_POINT('Ctrl Pts',(180.656548261642,3.38540250062943,48.5));
#77701=CARTESIAN_POINT('Ctrl Pts',(180.545497953892,3.22783091664314,48.5));
#77702=CARTESIAN_POINT('',(180.842633068562,3.38540250062943,48.35));
#77703=CARTESIAN_POINT('',(180.842633068562,3.38540250062943,48.5));
#77704=CARTESIAN_POINT('',(180.545497953892,3.22783091664314,48.35));
#77705=CARTESIAN_POINT('Ctrl Pts',(180.842633068562,3.38540250062943,48.35));
#77706=CARTESIAN_POINT('Ctrl Pts',(180.656548261642,3.38540250062943,48.35));
#77707=CARTESIAN_POINT('Ctrl Pts',(180.545497953892,3.22783091664314,48.35));
#77708=CARTESIAN_POINT('',(180.545497953892,3.22783091664314,48.5));
#77709=CARTESIAN_POINT('Ctrl Pts',(181.158526360989,3.2068213224411,48.5));
#77710=CARTESIAN_POINT('Ctrl Pts',(181.158526360989,3.2068213224411,48.35));
#77711=CARTESIAN_POINT('Ctrl Pts',(181.031718671322,3.38540250062943,48.5));
#77712=CARTESIAN_POINT('Ctrl Pts',(181.031718671322,3.38540250062943,48.35));
#77713=CARTESIAN_POINT('Ctrl Pts',(180.842633068562,3.38540250062943,48.5));
#77714=CARTESIAN_POINT('Ctrl Pts',(180.842633068562,3.38540250062943,48.35));
#77715=CARTESIAN_POINT('',(181.158526360989,3.2068213224411,48.5));
#77716=CARTESIAN_POINT('Ctrl Pts',(181.158526360989,3.2068213224411,48.5));
#77717=CARTESIAN_POINT('Ctrl Pts',(181.031718671322,3.38540250062943,48.5));
#77718=CARTESIAN_POINT('Ctrl Pts',(180.842633068562,3.38540250062943,48.5));
#77719=CARTESIAN_POINT('',(181.158526360989,3.2068213224411,48.35));
#77720=CARTESIAN_POINT('',(181.158526360989,3.2068213224411,48.5));
#77721=CARTESIAN_POINT('Ctrl Pts',(181.158526360989,3.2068213224411,48.35));
#77722=CARTESIAN_POINT('Ctrl Pts',(181.031718671322,3.38540250062943,48.35));
#77723=CARTESIAN_POINT('Ctrl Pts',(180.842633068562,3.38540250062943,48.35));
#77724=CARTESIAN_POINT('Ctrl Pts',(181.285334050655,2.48499327898026,48.5));
#77725=CARTESIAN_POINT('Ctrl Pts',(181.285334050655,2.48499327898026,48.35));
#77726=CARTESIAN_POINT('Ctrl Pts',(181.285334050655,3.02824014425278,48.5));
#77727=CARTESIAN_POINT('Ctrl Pts',(181.285334050655,3.02824014425278,48.35));
#77728=CARTESIAN_POINT('Ctrl Pts',(181.158526360989,3.2068213224411,48.5));
#77729=CARTESIAN_POINT('Ctrl Pts',(181.158526360989,3.2068213224411,48.35));
#77730=CARTESIAN_POINT('',(181.285334050655,2.48499327898026,48.5));
#77731=CARTESIAN_POINT('Ctrl Pts',(181.285334050655,2.48499327898026,48.5));
#77732=CARTESIAN_POINT('Ctrl Pts',(181.285334050655,3.02824014425278,48.5));
#77733=CARTESIAN_POINT('Ctrl Pts',(181.158526360989,3.2068213224411,48.5));
#77734=CARTESIAN_POINT('',(181.285334050655,2.48499327898026,48.35));
#77735=CARTESIAN_POINT('',(181.285334050655,2.48499327898026,48.5));
#77736=CARTESIAN_POINT('Ctrl Pts',(181.285334050655,2.48499327898026,48.35));
#77737=CARTESIAN_POINT('Ctrl Pts',(181.285334050655,3.02824014425278,48.35));
#77738=CARTESIAN_POINT('Ctrl Pts',(181.158526360989,3.2068213224411,48.35));
#77739=CARTESIAN_POINT('Ctrl Pts',(181.158526360989,1.76466578245163,48.5));
#77740=CARTESIAN_POINT('Ctrl Pts',(181.158526360989,1.76466578245163,48.35));
#77741=CARTESIAN_POINT('Ctrl Pts',(181.285334050655,1.9447478055954,48.5));
#77742=CARTESIAN_POINT('Ctrl Pts',(181.285334050655,1.9447478055954,48.35));
#77743=CARTESIAN_POINT('Ctrl Pts',(181.285334050655,2.48499327898026,48.5));
#77744=CARTESIAN_POINT('Ctrl Pts',(181.285334050655,2.48499327898026,48.35));
#77745=CARTESIAN_POINT('',(181.158526360989,1.76466578245163,48.5));
#77746=CARTESIAN_POINT('Ctrl Pts',(181.158526360989,1.76466578245163,48.5));
#77747=CARTESIAN_POINT('Ctrl Pts',(181.285334050655,1.9447478055954,48.5));
#77748=CARTESIAN_POINT('Ctrl Pts',(181.285334050655,2.48499327898026,48.5));
#77749=CARTESIAN_POINT('',(181.158526360989,1.76466578245163,48.35));
#77750=CARTESIAN_POINT('',(181.158526360989,1.76466578245163,48.5));
#77751=CARTESIAN_POINT('Ctrl Pts',(181.158526360989,1.76466578245163,48.35));
#77752=CARTESIAN_POINT('Ctrl Pts',(181.285334050655,1.9447478055954,48.35));
#77753=CARTESIAN_POINT('Ctrl Pts',(181.285334050655,2.48499327898026,48.35));
#77754=CARTESIAN_POINT('Ctrl Pts',(180.845634162426,1.58458405733109,48.5));
#77755=CARTESIAN_POINT('Ctrl Pts',(180.845634162426,1.58458405733109,48.35));
#77756=CARTESIAN_POINT('Ctrl Pts',(181.031718671322,1.58458405733109,48.5));
#77757=CARTESIAN_POINT('Ctrl Pts',(181.031718671322,1.58458405733109,48.35));
#77758=CARTESIAN_POINT('Ctrl Pts',(181.158526360989,1.76466578245163,48.5));
#77759=CARTESIAN_POINT('Ctrl Pts',(181.158526360989,1.76466578245163,48.35));
#77760=CARTESIAN_POINT('',(180.845634162426,1.58458405733109,48.5));
#77761=CARTESIAN_POINT('Ctrl Pts',(180.845634162426,1.58458405733109,48.5));
#77762=CARTESIAN_POINT('Ctrl Pts',(181.031718671322,1.58458405733109,48.5));
#77763=CARTESIAN_POINT('Ctrl Pts',(181.158526360989,1.76466578245163,48.5));
#77764=CARTESIAN_POINT('',(180.845634162426,1.58458405733109,48.35));
#77765=CARTESIAN_POINT('',(180.845634162426,1.58458405733109,48.5));
#77766=CARTESIAN_POINT('Ctrl Pts',(180.845634162426,1.58458405733109,48.35));
#77767=CARTESIAN_POINT('Ctrl Pts',(181.031718671322,1.58458405733109,48.35));
#77768=CARTESIAN_POINT('Ctrl Pts',(181.158526360989,1.76466578245163,48.35));
#77769=CARTESIAN_POINT('Ctrl Pts',(180.532741963863,1.76391565799713,48.5));
#77770=CARTESIAN_POINT('Ctrl Pts',(180.532741963863,1.76391565799713,48.35));
#77771=CARTESIAN_POINT('Ctrl Pts',(180.65954965353,1.58458405733109,48.5));
#77772=CARTESIAN_POINT('Ctrl Pts',(180.65954965353,1.58458405733109,48.35));
#77773=CARTESIAN_POINT('Ctrl Pts',(180.845634162426,1.58458405733109,48.5));
#77774=CARTESIAN_POINT('Ctrl Pts',(180.845634162426,1.58458405733109,48.35));
#77775=CARTESIAN_POINT('',(180.532741963863,1.76391565799713,48.5));
#77776=CARTESIAN_POINT('Ctrl Pts',(180.532741963863,1.76391565799713,48.5));
#77777=CARTESIAN_POINT('Ctrl Pts',(180.65954965353,1.58458405733109,48.5));
#77778=CARTESIAN_POINT('Ctrl Pts',(180.845634162426,1.58458405733109,48.5));
#77779=CARTESIAN_POINT('',(180.532741963863,1.76391565799713,48.35));
#77780=CARTESIAN_POINT('',(180.532741963863,1.76391565799713,48.5));
#77781=CARTESIAN_POINT('Ctrl Pts',(180.532741963863,1.76391565799713,48.35));
#77782=CARTESIAN_POINT('Ctrl Pts',(180.65954965353,1.58458405733109,48.35));
#77783=CARTESIAN_POINT('Ctrl Pts',(180.845634162426,1.58458405733109,48.35));
#77784=CARTESIAN_POINT('Ctrl Pts',(180.405934274197,2.48499327898026,48.5));
#77785=CARTESIAN_POINT('Ctrl Pts',(180.405934274197,2.48499327898026,48.35));
#77786=CARTESIAN_POINT('Ctrl Pts',(180.405934274197,1.94324696063995,48.5));
#77787=CARTESIAN_POINT('Ctrl Pts',(180.405934274197,1.94324696063995,48.35));
#77788=CARTESIAN_POINT('Ctrl Pts',(180.532741963863,1.76391565799713,48.5));
#77789=CARTESIAN_POINT('Ctrl Pts',(180.532741963863,1.76391565799713,48.35));
#77790=CARTESIAN_POINT('',(180.405934274197,2.48499327898026,48.5));
#77791=CARTESIAN_POINT('Ctrl Pts',(180.405934274197,2.48499327898026,48.5));
#77792=CARTESIAN_POINT('Ctrl Pts',(180.405934274197,1.94324696063995,48.5));
#77793=CARTESIAN_POINT('Ctrl Pts',(180.532741963863,1.76391565799713,48.5));
#77794=CARTESIAN_POINT('',(180.405934274197,2.48499327898026,48.35));
#77795=CARTESIAN_POINT('',(180.405934274197,2.48499327898026,48.5));
#77796=CARTESIAN_POINT('Ctrl Pts',(180.405934274197,2.48499327898026,48.35));
#77797=CARTESIAN_POINT('Ctrl Pts',(180.405934274197,1.94324696063995,48.35));
#77798=CARTESIAN_POINT('Ctrl Pts',(180.532741963863,1.76391565799713,48.35));
#77799=CARTESIAN_POINT('Ctrl Pts',(180.545497953892,3.22783091664314,48.5));
#77800=CARTESIAN_POINT('Ctrl Pts',(180.545497953892,3.22783091664314,48.35));
#77801=CARTESIAN_POINT('Ctrl Pts',(180.405934274197,3.02673944830894,48.5));
#77802=CARTESIAN_POINT('Ctrl Pts',(180.405934274197,3.02673944830894,48.35));
#77803=CARTESIAN_POINT('Ctrl Pts',(180.405934274197,2.48499327898026,48.5));
#77804=CARTESIAN_POINT('Ctrl Pts',(180.405934274197,2.48499327898026,48.35));
#77805=CARTESIAN_POINT('Ctrl Pts',(180.545497953892,3.22783091664314,48.5));
#77806=CARTESIAN_POINT('Ctrl Pts',(180.405934274197,3.02673944830894,48.5));
#77807=CARTESIAN_POINT('Ctrl Pts',(180.405934274197,2.48499327898026,48.5));
#77808=CARTESIAN_POINT('Ctrl Pts',(180.545497953892,3.22783091664314,48.35));
#77809=CARTESIAN_POINT('Ctrl Pts',(180.405934274197,3.02673944830894,48.35));
#77810=CARTESIAN_POINT('Ctrl Pts',(180.405934274197,2.48499327898026,48.35));
#77811=CARTESIAN_POINT('Ctrl Pts',(180.845634162426,1.36248314380646,48.5));
#77812=CARTESIAN_POINT('Ctrl Pts',(180.845634162426,1.36248314380646,48.35));
#77813=CARTESIAN_POINT('Ctrl Pts',(180.527489602566,1.36248314380646,48.5));
#77814=CARTESIAN_POINT('Ctrl Pts',(180.527489602566,1.36248314380646,48.35));
#77815=CARTESIAN_POINT('Ctrl Pts',(180.34590703249,1.59058684110642,48.5));
#77816=CARTESIAN_POINT('Ctrl Pts',(180.34590703249,1.59058684110642,48.35));
#77817=CARTESIAN_POINT('',(180.845634162426,1.36248314380646,48.5));
#77818=CARTESIAN_POINT('',(180.34590703249,1.59058684110642,48.5));
#77819=CARTESIAN_POINT('Ctrl Pts',(180.845634162426,1.36248314380646,48.5));
#77820=CARTESIAN_POINT('Ctrl Pts',(180.527489602566,1.36248314380646,48.5));
#77821=CARTESIAN_POINT('Ctrl Pts',(180.34590703249,1.59058684110642,48.5));
#77822=CARTESIAN_POINT('',(180.845634162426,1.36248314380646,48.35));
#77823=CARTESIAN_POINT('',(180.845634162426,1.36248314380646,48.5));
#77824=CARTESIAN_POINT('',(180.34590703249,1.59058684110642,48.35));
#77825=CARTESIAN_POINT('Ctrl Pts',(180.845634162426,1.36248314380646,48.35));
#77826=CARTESIAN_POINT('Ctrl Pts',(180.527489602566,1.36248314380646,48.35));
#77827=CARTESIAN_POINT('Ctrl Pts',(180.34590703249,1.59058684110642,48.35));
#77828=CARTESIAN_POINT('',(180.34590703249,1.59058684110642,48.5));
#77829=CARTESIAN_POINT('Ctrl Pts',(181.245565831661,1.49229192733765,48.5));
#77830=CARTESIAN_POINT('Ctrl Pts',(181.245565831661,1.49229192733765,48.35));
#77831=CARTESIAN_POINT('Ctrl Pts',(181.087243974209,1.36248314380646,48.5));
#77832=CARTESIAN_POINT('Ctrl Pts',(181.087243974209,1.36248314380646,48.35));
#77833=CARTESIAN_POINT('Ctrl Pts',(180.845634162426,1.36248314380646,48.5));
#77834=CARTESIAN_POINT('Ctrl Pts',(180.845634162426,1.36248314380646,48.35));
#77835=CARTESIAN_POINT('',(181.245565831661,1.49229192733765,48.5));
#77836=CARTESIAN_POINT('Ctrl Pts',(181.245565831661,1.49229192733765,48.5));
#77837=CARTESIAN_POINT('Ctrl Pts',(181.087243974209,1.36248314380646,48.5));
#77838=CARTESIAN_POINT('Ctrl Pts',(180.845634162426,1.36248314380646,48.5));
#77839=CARTESIAN_POINT('',(181.245565831661,1.49229192733765,48.35));
#77840=CARTESIAN_POINT('',(181.245565831661,1.49229192733765,48.5));
#77841=CARTESIAN_POINT('Ctrl Pts',(181.245565831661,1.49229192733765,48.35));
#77842=CARTESIAN_POINT('Ctrl Pts',(181.087243974209,1.36248314380646,48.35));
#77843=CARTESIAN_POINT('Ctrl Pts',(180.845634162426,1.36248314380646,48.35));
#77844=CARTESIAN_POINT('Ctrl Pts',(181.483424127102,1.85995900630951,48.5));
#77845=CARTESIAN_POINT('Ctrl Pts',(181.483424127102,1.85995900630951,48.35));
#77846=CARTESIAN_POINT('Ctrl Pts',(181.403887689114,1.62210100889206,48.5));
#77847=CARTESIAN_POINT('Ctrl Pts',(181.403887689114,1.62210100889206,48.35));
#77848=CARTESIAN_POINT('Ctrl Pts',(181.245565831661,1.49229192733765,48.5));
#77849=CARTESIAN_POINT('Ctrl Pts',(181.245565831661,1.49229192733765,48.35));
#77850=CARTESIAN_POINT('',(181.483424127102,1.85995900630951,48.5));
#77851=CARTESIAN_POINT('Ctrl Pts',(181.483424127102,1.85995900630951,48.5));
#77852=CARTESIAN_POINT('Ctrl Pts',(181.403887689114,1.62210100889206,48.5));
#77853=CARTESIAN_POINT('Ctrl Pts',(181.245565831661,1.49229192733765,48.5));
#77854=CARTESIAN_POINT('',(181.483424127102,1.85995900630951,48.35));
#77855=CARTESIAN_POINT('',(181.483424127102,1.85995900630951,48.5));
#77856=CARTESIAN_POINT('Ctrl Pts',(181.483424127102,1.85995900630951,48.35));
#77857=CARTESIAN_POINT('Ctrl Pts',(181.403887689114,1.62210100889206,48.35));
#77858=CARTESIAN_POINT('Ctrl Pts',(181.245565831661,1.49229192733765,48.35));
#77859=CARTESIAN_POINT('Ctrl Pts',(181.562959969044,2.48499327898026,48.5));
#77860=CARTESIAN_POINT('Ctrl Pts',(181.562959969044,2.48499327898026,48.35));
#77861=CARTESIAN_POINT('Ctrl Pts',(181.562959969044,2.09781730175018,48.5));
#77862=CARTESIAN_POINT('Ctrl Pts',(181.562959969044,2.09781730175018,48.35));
#77863=CARTESIAN_POINT('Ctrl Pts',(181.483424127102,1.85995900630951,48.5));
#77864=CARTESIAN_POINT('Ctrl Pts',(181.483424127102,1.85995900630951,48.35));
#77865=CARTESIAN_POINT('',(181.562959969044,2.48499327898026,48.5));
#77866=CARTESIAN_POINT('Ctrl Pts',(181.562959969044,2.48499327898026,48.5));
#77867=CARTESIAN_POINT('Ctrl Pts',(181.562959969044,2.09781730175018,48.5));
#77868=CARTESIAN_POINT('Ctrl Pts',(181.483424127102,1.85995900630951,48.5));
#77869=CARTESIAN_POINT('',(181.562959969044,2.48499327898026,48.35));
#77870=CARTESIAN_POINT('',(181.562959969044,2.48499327898026,48.5));
#77871=CARTESIAN_POINT('Ctrl Pts',(181.562959969044,2.48499327898026,48.35));
#77872=CARTESIAN_POINT('Ctrl Pts',(181.562959969044,2.09781730175018,48.35));
#77873=CARTESIAN_POINT('Ctrl Pts',(181.483424127102,1.85995900630951,48.35));
#77874=CARTESIAN_POINT('Ctrl Pts',(181.513437449932,3.00497958064079,48.5));
#77875=CARTESIAN_POINT('Ctrl Pts',(181.513437449932,3.00497958064079,48.35));
#77876=CARTESIAN_POINT('Ctrl Pts',(181.562959969044,2.81214186549187,48.5));
#77877=CARTESIAN_POINT('Ctrl Pts',(181.562959969044,2.81214186549187,48.35));
#77878=CARTESIAN_POINT('Ctrl Pts',(181.562959969044,2.48499327898026,48.5));
#77879=CARTESIAN_POINT('Ctrl Pts',(181.562959969044,2.48499327898026,48.35));
#77880=CARTESIAN_POINT('',(181.513437449932,3.00497958064079,48.5));
#77881=CARTESIAN_POINT('Ctrl Pts',(181.513437449932,3.00497958064079,48.5));
#77882=CARTESIAN_POINT('Ctrl Pts',(181.562959969044,2.81214186549187,48.5));
#77883=CARTESIAN_POINT('Ctrl Pts',(181.562959969044,2.48499327898026,48.5));
#77884=CARTESIAN_POINT('',(181.513437449932,3.00497958064079,48.35));
#77885=CARTESIAN_POINT('',(181.513437449932,3.00497958064079,48.5));
#77886=CARTESIAN_POINT('Ctrl Pts',(181.513437449932,3.00497958064079,48.35));
#77887=CARTESIAN_POINT('Ctrl Pts',(181.562959969044,2.81214186549187,48.35));
#77888=CARTESIAN_POINT('Ctrl Pts',(181.562959969044,2.48499327898026,48.35));
#77889=CARTESIAN_POINT('Ctrl Pts',(181.376875460148,3.33212831616402,48.5));
#77890=CARTESIAN_POINT('Ctrl Pts',(181.376875460148,3.33212831616402,48.35));
#77891=CARTESIAN_POINT('Ctrl Pts',(181.46391493082,3.19781729578972,48.5));
#77892=CARTESIAN_POINT('Ctrl Pts',(181.46391493082,3.19781729578972,48.35));
#77893=CARTESIAN_POINT('Ctrl Pts',(181.513437449932,3.00497958064079,48.5));
#77894=CARTESIAN_POINT('Ctrl Pts',(181.513437449932,3.00497958064079,48.35));
#77895=CARTESIAN_POINT('',(181.376875460148,3.33212831616402,48.5));
#77896=CARTESIAN_POINT('Ctrl Pts',(181.376875460148,3.33212831616402,48.5));
#77897=CARTESIAN_POINT('Ctrl Pts',(181.46391493082,3.19781729578972,48.5));
#77898=CARTESIAN_POINT('Ctrl Pts',(181.513437449932,3.00497958064079,48.5));
#77899=CARTESIAN_POINT('',(181.376875460148,3.33212831616402,48.35));
#77900=CARTESIAN_POINT('',(181.376875460148,3.33212831616402,48.5));
#77901=CARTESIAN_POINT('Ctrl Pts',(181.376875460148,3.33212831616402,48.35));
#77902=CARTESIAN_POINT('Ctrl Pts',(181.46391493082,3.19781729578972,48.35));
#77903=CARTESIAN_POINT('Ctrl Pts',(181.513437449932,3.00497958064079,48.35));
#77904=CARTESIAN_POINT('Ctrl Pts',(181.156275689602,3.5377217233181,48.5));
#77905=CARTESIAN_POINT('Ctrl Pts',(181.156275689602,3.5377217233181,48.35));
#77906=CARTESIAN_POINT('Ctrl Pts',(181.289835989475,3.46643933653831,48.5));
#77907=CARTESIAN_POINT('Ctrl Pts',(181.289835989475,3.46643933653831,48.35));
#77908=CARTESIAN_POINT('Ctrl Pts',(181.376875460148,3.33212831616402,48.5));
#77909=CARTESIAN_POINT('Ctrl Pts',(181.376875460148,3.33212831616402,48.35));
#77910=CARTESIAN_POINT('',(181.156275689602,3.5377217233181,48.5));
#77911=CARTESIAN_POINT('Ctrl Pts',(181.156275689602,3.5377217233181,48.5));
#77912=CARTESIAN_POINT('Ctrl Pts',(181.289835989475,3.46643933653831,48.5));
#77913=CARTESIAN_POINT('Ctrl Pts',(181.376875460148,3.33212831616402,48.5));
#77914=CARTESIAN_POINT('',(181.156275689602,3.5377217233181,48.35));
#77915=CARTESIAN_POINT('',(181.156275689602,3.5377217233181,48.5));
#77916=CARTESIAN_POINT('Ctrl Pts',(181.156275689602,3.5377217233181,48.35));
#77917=CARTESIAN_POINT('Ctrl Pts',(181.289835989475,3.46643933653831,48.35));
#77918=CARTESIAN_POINT('Ctrl Pts',(181.376875460148,3.33212831616402,48.35));
#77919=CARTESIAN_POINT('Ctrl Pts',(180.845634162426,3.60900411009789,48.5));
#77920=CARTESIAN_POINT('Ctrl Pts',(180.845634162426,3.60900411009789,48.35));
#77921=CARTESIAN_POINT('Ctrl Pts',(181.022714793682,3.60900411009789,48.5));
#77922=CARTESIAN_POINT('Ctrl Pts',(181.022714793682,3.60900411009789,48.35));
#77923=CARTESIAN_POINT('Ctrl Pts',(181.156275689602,3.5377217233181,48.5));
#77924=CARTESIAN_POINT('Ctrl Pts',(181.156275689602,3.5377217233181,48.35));
#77925=CARTESIAN_POINT('',(180.845634162426,3.60900411009789,48.5));
#77926=CARTESIAN_POINT('Ctrl Pts',(180.845634162426,3.60900411009789,48.5));
#77927=CARTESIAN_POINT('Ctrl Pts',(181.022714793682,3.60900411009789,48.5));
#77928=CARTESIAN_POINT('Ctrl Pts',(181.156275689602,3.5377217233181,48.5));
#77929=CARTESIAN_POINT('',(180.845634162426,3.60900411009789,48.35));
#77930=CARTESIAN_POINT('',(180.845634162426,3.60900411009789,48.5));
#77931=CARTESIAN_POINT('Ctrl Pts',(180.845634162426,3.60900411009789,48.35));
#77932=CARTESIAN_POINT('Ctrl Pts',(181.022714793682,3.60900411009789,48.35));
#77933=CARTESIAN_POINT('Ctrl Pts',(181.156275689602,3.5377217233181,48.35));
#77934=CARTESIAN_POINT('Ctrl Pts',(180.447203338146,3.47994545102119,48.5));
#77935=CARTESIAN_POINT('Ctrl Pts',(180.447203338146,3.47994545102119,48.35));
#77936=CARTESIAN_POINT('Ctrl Pts',(180.605525195599,3.60900411009789,48.5));
#77937=CARTESIAN_POINT('Ctrl Pts',(180.605525195599,3.60900411009789,48.35));
#77938=CARTESIAN_POINT('Ctrl Pts',(180.845634162426,3.60900411009789,48.5));
#77939=CARTESIAN_POINT('Ctrl Pts',(180.845634162426,3.60900411009789,48.35));
#77940=CARTESIAN_POINT('',(180.447203338146,3.47994545102119,48.5));
#77941=CARTESIAN_POINT('Ctrl Pts',(180.447203338146,3.47994545102119,48.5));
#77942=CARTESIAN_POINT('Ctrl Pts',(180.605525195599,3.60900411009789,48.5));
#77943=CARTESIAN_POINT('Ctrl Pts',(180.845634162426,3.60900411009789,48.5));
#77944=CARTESIAN_POINT('',(180.447203338146,3.47994545102119,48.35));
#77945=CARTESIAN_POINT('',(180.447203338146,3.47994545102119,48.5));
#77946=CARTESIAN_POINT('Ctrl Pts',(180.447203338146,3.47994545102119,48.35));
#77947=CARTESIAN_POINT('Ctrl Pts',(180.605525195599,3.60900411009789,48.35));
#77948=CARTESIAN_POINT('Ctrl Pts',(180.845634162426,3.60900411009789,48.35));
#77949=CARTESIAN_POINT('Ctrl Pts',(180.208594620228,3.11302864551544,48.5));
#77950=CARTESIAN_POINT('Ctrl Pts',(180.208594620228,3.11302864551544,48.35));
#77951=CARTESIAN_POINT('Ctrl Pts',(180.288881182671,3.3508867919445,48.5));
#77952=CARTESIAN_POINT('Ctrl Pts',(180.288881182671,3.3508867919445,48.35));
#77953=CARTESIAN_POINT('Ctrl Pts',(180.447203338146,3.47994545102119,48.5));
#77954=CARTESIAN_POINT('Ctrl Pts',(180.447203338146,3.47994545102119,48.35));
#77955=CARTESIAN_POINT('',(180.208594620228,3.11302864551544,48.5));
#77956=CARTESIAN_POINT('Ctrl Pts',(180.208594620228,3.11302864551544,48.5));
#77957=CARTESIAN_POINT('Ctrl Pts',(180.288881182671,3.3508867919445,48.5));
#77958=CARTESIAN_POINT('Ctrl Pts',(180.447203338146,3.47994545102119,48.5));
#77959=CARTESIAN_POINT('',(180.208594620228,3.11302864551544,48.35));
#77960=CARTESIAN_POINT('',(180.208594620228,3.11302864551544,48.5));
#77961=CARTESIAN_POINT('Ctrl Pts',(180.208594620228,3.11302864551544,48.35));
#77962=CARTESIAN_POINT('Ctrl Pts',(180.288881182671,3.3508867919445,48.35));
#77963=CARTESIAN_POINT('Ctrl Pts',(180.447203338146,3.47994545102119,48.35));
#77964=CARTESIAN_POINT('Ctrl Pts',(180.128308355808,2.48499327898026,48.5));
#77965=CARTESIAN_POINT('Ctrl Pts',(180.128308355808,2.48499327898026,48.35));
#77966=CARTESIAN_POINT('Ctrl Pts',(180.128308355808,2.87517049908638,48.5));
#77967=CARTESIAN_POINT('Ctrl Pts',(180.128308355808,2.87517049908638,48.35));
#77968=CARTESIAN_POINT('Ctrl Pts',(180.208594620228,3.11302864551544,48.5));
#77969=CARTESIAN_POINT('Ctrl Pts',(180.208594620228,3.11302864551544,48.35));
#77970=CARTESIAN_POINT('',(180.128308355808,2.48499327898026,48.5));
#77971=CARTESIAN_POINT('Ctrl Pts',(180.128308355808,2.48499327898026,48.5));
#77972=CARTESIAN_POINT('Ctrl Pts',(180.128308355808,2.87517049908638,48.5));
#77973=CARTESIAN_POINT('Ctrl Pts',(180.208594620228,3.11302864551544,48.5));
#77974=CARTESIAN_POINT('',(180.128308355808,2.48499327898026,48.35));
#77975=CARTESIAN_POINT('',(180.128308355808,2.48499327898026,48.5));
#77976=CARTESIAN_POINT('Ctrl Pts',(180.128308355808,2.48499327898026,48.35));
#77977=CARTESIAN_POINT('Ctrl Pts',(180.128308355808,2.87517049908638,48.35));
#77978=CARTESIAN_POINT('Ctrl Pts',(180.208594620228,3.11302864551544,48.35));
#77979=CARTESIAN_POINT('Ctrl Pts',(180.34590703249,1.59058684110642,48.5));
#77980=CARTESIAN_POINT('Ctrl Pts',(180.34590703249,1.59058684110642,48.35));
#77981=CARTESIAN_POINT('Ctrl Pts',(180.128308355808,1.86521166563034,48.5));
#77982=CARTESIAN_POINT('Ctrl Pts',(180.128308355808,1.86521166563034,48.35));
#77983=CARTESIAN_POINT('Ctrl Pts',(180.128308355808,2.48499327898026,48.5));
#77984=CARTESIAN_POINT('Ctrl Pts',(180.128308355808,2.48499327898026,48.35));
#77985=CARTESIAN_POINT('Ctrl Pts',(180.34590703249,1.59058684110642,48.5));
#77986=CARTESIAN_POINT('Ctrl Pts',(180.128308355808,1.86521166563034,48.5));
#77987=CARTESIAN_POINT('Ctrl Pts',(180.128308355808,2.48499327898026,48.5));
#77988=CARTESIAN_POINT('Ctrl Pts',(180.34590703249,1.59058684110642,48.35));
#77989=CARTESIAN_POINT('Ctrl Pts',(180.128308355808,1.86521166563034,48.35));
#77990=CARTESIAN_POINT('Ctrl Pts',(180.128308355808,2.48499327898026,48.35));
#77991=CARTESIAN_POINT('Origin',(179.99999974668,2.48574362695217,48.35));
#77992=CARTESIAN_POINT('Ctrl Pts',(179.126602977514,2.7363575398922,48.5));
#77993=CARTESIAN_POINT('Ctrl Pts',(179.126602977514,2.7363575398922,48.35));
#77994=CARTESIAN_POINT('Ctrl Pts',(179.308935821056,3.07776266336441,48.5));
#77995=CARTESIAN_POINT('Ctrl Pts',(179.308935821056,3.07776266336441,48.35));
#77996=CARTESIAN_POINT('Ctrl Pts',(179.51452922821,3.3118691444397,48.5));
#77997=CARTESIAN_POINT('Ctrl Pts',(179.51452922821,3.3118691444397,48.35));
#77998=CARTESIAN_POINT('',(179.126602977514,2.7363575398922,48.5));
#77999=CARTESIAN_POINT('',(179.51452922821,3.3118691444397,48.5));
#78000=CARTESIAN_POINT('Ctrl Pts',(179.126602977514,2.7363575398922,48.5));
#78001=CARTESIAN_POINT('Ctrl Pts',(179.308935821056,3.07776266336441,48.5));
#78002=CARTESIAN_POINT('Ctrl Pts',(179.51452922821,3.3118691444397,48.5));
#78003=CARTESIAN_POINT('',(179.126602977514,2.7363575398922,48.35));
#78004=CARTESIAN_POINT('',(179.126602977514,2.7363575398922,48.5));
#78005=CARTESIAN_POINT('',(179.51452922821,3.3118691444397,48.35));
#78006=CARTESIAN_POINT('Ctrl Pts',(179.126602977514,2.7363575398922,48.35));
#78007=CARTESIAN_POINT('Ctrl Pts',(179.308935821056,3.07776266336441,48.35));
#78008=CARTESIAN_POINT('Ctrl Pts',(179.51452922821,3.3118691444397,48.35));
#78009=CARTESIAN_POINT('',(179.51452922821,3.3118691444397,48.5));
#78010=CARTESIAN_POINT('Ctrl Pts',(178.846725791693,2.02728533744812,48.5));
#78011=CARTESIAN_POINT('Ctrl Pts',(178.846725791693,2.02728533744812,48.35));
#78012=CARTESIAN_POINT('Ctrl Pts',(178.944270133972,2.39495241641998,48.5));
#78013=CARTESIAN_POINT('Ctrl Pts',(178.944270133972,2.39495241641998,48.35));
#78014=CARTESIAN_POINT('Ctrl Pts',(179.126602977514,2.7363575398922,48.5));
#78015=CARTESIAN_POINT('Ctrl Pts',(179.126602977514,2.7363575398922,48.35));
#78016=CARTESIAN_POINT('',(178.846725791693,2.02728533744812,48.5));
#78017=CARTESIAN_POINT('Ctrl Pts',(178.846725791693,2.02728533744812,48.5));
#78018=CARTESIAN_POINT('Ctrl Pts',(178.944270133972,2.39495241641998,48.5));
#78019=CARTESIAN_POINT('Ctrl Pts',(179.126602977514,2.7363575398922,48.5));
#78020=CARTESIAN_POINT('',(178.846725791693,2.02728533744812,48.35));
#78021=CARTESIAN_POINT('',(178.846725791693,2.02728533744812,48.5));
#78022=CARTESIAN_POINT('Ctrl Pts',(178.846725791693,2.02728533744812,48.35));
#78023=CARTESIAN_POINT('Ctrl Pts',(178.944270133972,2.39495241641998,48.35));
#78024=CARTESIAN_POINT('Ctrl Pts',(179.126602977514,2.7363575398922,48.35));
#78025=CARTESIAN_POINT('Ctrl Pts',(178.744679361582,1.40000009536743,48.5));
#78026=CARTESIAN_POINT('Ctrl Pts',(178.744679361582,1.40000009536743,48.35));
#78027=CARTESIAN_POINT('Ctrl Pts',(178.749181449413,1.65961825847626,48.5));
#78028=CARTESIAN_POINT('Ctrl Pts',(178.749181449413,1.65961825847626,48.35));
#78029=CARTESIAN_POINT('Ctrl Pts',(178.846725791693,2.02728533744812,48.5));
#78030=CARTESIAN_POINT('Ctrl Pts',(178.846725791693,2.02728533744812,48.35));
#78031=CARTESIAN_POINT('',(178.744679361582,1.40000009536743,48.5));
#78032=CARTESIAN_POINT('Ctrl Pts',(178.744679361582,1.40000009536743,48.5));
#78033=CARTESIAN_POINT('Ctrl Pts',(178.749181449413,1.65961825847626,48.5));
#78034=CARTESIAN_POINT('Ctrl Pts',(178.846725791693,2.02728533744812,48.5));
#78035=CARTESIAN_POINT('',(178.744679361582,1.40000009536743,48.35));
#78036=CARTESIAN_POINT('',(178.744679361582,1.40000009536743,48.5));
#78037=CARTESIAN_POINT('Ctrl Pts',(178.744679361582,1.40000009536743,48.35));
#78038=CARTESIAN_POINT('Ctrl Pts',(178.749181449413,1.65961825847626,48.35));
#78039=CARTESIAN_POINT('Ctrl Pts',(178.846725791693,2.02728533744812,48.35));
#78040=CARTESIAN_POINT('Origin',(179.022305577993,1.40000009536743,48.5));
#78041=CARTESIAN_POINT('',(179.022305577993,1.40000009536743,48.5));
#78042=CARTESIAN_POINT('',(89.5111527889967,1.40000009536743,48.5));
#78043=CARTESIAN_POINT('',(179.022305577993,1.40000009536743,48.35));
#78044=CARTESIAN_POINT('',(179.022305577993,1.40000009536743,48.5));
#78045=CARTESIAN_POINT('',(179.022305577993,1.40000009536743,48.35));
#78046=CARTESIAN_POINT('Ctrl Pts',(179.125852704048,2.00477504730225,48.5));
#78047=CARTESIAN_POINT('Ctrl Pts',(179.125852704048,2.00477504730225,48.35));
#78048=CARTESIAN_POINT('Ctrl Pts',(179.044815719128,1.72864937782288,48.5));
#78049=CARTESIAN_POINT('Ctrl Pts',(179.044815719128,1.72864937782288,48.35));
#78050=CARTESIAN_POINT('Ctrl Pts',(179.022305577993,1.40000009536743,48.5));
#78051=CARTESIAN_POINT('Ctrl Pts',(179.022305577993,1.40000009536743,48.35));
#78052=CARTESIAN_POINT('',(179.125852704048,2.00477504730225,48.5));
#78053=CARTESIAN_POINT('Ctrl Pts',(179.125852704048,2.00477504730225,48.5));
#78054=CARTESIAN_POINT('Ctrl Pts',(179.044815719128,1.72864937782288,48.5));
#78055=CARTESIAN_POINT('Ctrl Pts',(179.022305577993,1.40000009536743,48.5));
#78056=CARTESIAN_POINT('',(179.125852704048,2.00477504730225,48.35));
#78057=CARTESIAN_POINT('',(179.125852704048,2.00477504730225,48.5));
#78058=CARTESIAN_POINT('Ctrl Pts',(179.125852704048,2.00477504730225,48.35));
#78059=CARTESIAN_POINT('Ctrl Pts',(179.044815719128,1.72864937782288,48.35));
#78060=CARTESIAN_POINT('Ctrl Pts',(179.022305577993,1.40000009536743,48.35));
#78061=CARTESIAN_POINT('Ctrl Pts',(179.444747388363,2.76712143421173,48.5));
#78062=CARTESIAN_POINT('Ctrl Pts',(179.444747388363,2.76712143421173,48.35));
#78063=CARTESIAN_POINT('Ctrl Pts',(179.238403856754,2.3964529633522,48.5));
#78064=CARTESIAN_POINT('Ctrl Pts',(179.238403856754,2.3964529633522,48.35));
#78065=CARTESIAN_POINT('Ctrl Pts',(179.125852704048,2.00477504730225,48.5));
#78066=CARTESIAN_POINT('Ctrl Pts',(179.125852704048,2.00477504730225,48.35));
#78067=CARTESIAN_POINT('',(179.444747388363,2.76712143421173,48.5));
#78068=CARTESIAN_POINT('Ctrl Pts',(179.444747388363,2.76712143421173,48.5));
#78069=CARTESIAN_POINT('Ctrl Pts',(179.238403856754,2.3964529633522,48.5));
#78070=CARTESIAN_POINT('Ctrl Pts',(179.125852704048,2.00477504730225,48.5));
#78071=CARTESIAN_POINT('',(179.444747388363,2.76712143421173,48.35));
#78072=CARTESIAN_POINT('',(179.444747388363,2.76712143421173,48.5));
#78073=CARTESIAN_POINT('Ctrl Pts',(179.444747388363,2.76712143421173,48.35));
#78074=CARTESIAN_POINT('Ctrl Pts',(179.238403856754,2.3964529633522,48.35));
#78075=CARTESIAN_POINT('Ctrl Pts',(179.125852704048,2.00477504730225,48.35));
#78076=CARTESIAN_POINT('Ctrl Pts',(179.861186861992,3.36139166355133,48.5));
#78077=CARTESIAN_POINT('Ctrl Pts',(179.861186861992,3.36139166355133,48.35));
#78078=CARTESIAN_POINT('Ctrl Pts',(179.651091516018,3.13779005408287,48.5));
#78079=CARTESIAN_POINT('Ctrl Pts',(179.651091516018,3.13779005408287,48.35));
#78080=CARTESIAN_POINT('Ctrl Pts',(179.444747388363,2.76712143421173,48.5));
#78081=CARTESIAN_POINT('Ctrl Pts',(179.444747388363,2.76712143421173,48.35));
#78082=CARTESIAN_POINT('',(179.861186861992,3.36139166355133,48.5));
#78083=CARTESIAN_POINT('Ctrl Pts',(179.861186861992,3.36139166355133,48.5));
#78084=CARTESIAN_POINT('Ctrl Pts',(179.651091516018,3.13779005408287,48.5));
#78085=CARTESIAN_POINT('Ctrl Pts',(179.444747388363,2.76712143421173,48.5));
#78086=CARTESIAN_POINT('',(179.861186861992,3.36139166355133,48.35));
#78087=CARTESIAN_POINT('',(179.861186861992,3.36139166355133,48.5));
#78088=CARTESIAN_POINT('Ctrl Pts',(179.861186861992,3.36139166355133,48.35));
#78089=CARTESIAN_POINT('Ctrl Pts',(179.651091516018,3.13779005408287,48.35));
#78090=CARTESIAN_POINT('Ctrl Pts',(179.444747388363,2.76712143421173,48.35));
#78091=CARTESIAN_POINT('Origin',(179.861186861992,3.57148715853691,48.5));
#78092=CARTESIAN_POINT('',(179.861186861992,3.57148715853691,48.5));
#78093=CARTESIAN_POINT('',(179.861186861992,5.78574357926846,48.5));
#78094=CARTESIAN_POINT('',(179.861186861992,3.57148715853691,48.35));
#78095=CARTESIAN_POINT('',(179.861186861992,3.57148715853691,48.5));
#78096=CARTESIAN_POINT('',(179.861186861992,3.57148715853691,48.35));
#78097=CARTESIAN_POINT('Origin',(178.437039524317,3.57148715853691,48.5));
#78098=CARTESIAN_POINT('',(178.437039524317,3.57148715853691,48.5));
#78099=CARTESIAN_POINT('',(89.2185197621584,3.57148715853691,48.5));
#78100=CARTESIAN_POINT('',(178.437039524317,3.57148715853691,48.35));
#78101=CARTESIAN_POINT('',(178.437039524317,3.57148715853691,48.5));
#78102=CARTESIAN_POINT('',(178.437039524317,3.57148715853691,48.35));
#78103=CARTESIAN_POINT('Origin',(178.437039524317,3.3118691444397,48.5));
#78104=CARTESIAN_POINT('',(178.437039524317,3.3118691444397,48.5));
#78105=CARTESIAN_POINT('',(178.437039524317,5.65593457221985,48.5));
#78106=CARTESIAN_POINT('',(178.437039524317,3.3118691444397,48.35));
#78107=CARTESIAN_POINT('',(178.437039524317,3.3118691444397,48.5));
#78108=CARTESIAN_POINT('',(178.437039524317,3.3118691444397,48.35));
#78109=CARTESIAN_POINT('Origin',(179.51452922821,3.3118691444397,48.5));
#78110=CARTESIAN_POINT('',(89.7572646141052,3.3118691444397,48.5));
#78111=CARTESIAN_POINT('',(179.51452922821,3.3118691444397,48.35));
#78112=CARTESIAN_POINT('Origin',(179.99999974668,2.48574362695217,48.35));
#78113=CARTESIAN_POINT('Origin',(0.,8.,48.5));
#78114=CARTESIAN_POINT('Ctrl Pts',(170.857640046626,3.38540250062943,48.5));
#78115=CARTESIAN_POINT('Ctrl Pts',(170.857640046626,3.38540250062943,48.35));
#78116=CARTESIAN_POINT('Ctrl Pts',(170.671555239707,3.38540250062943,48.5));
#78117=CARTESIAN_POINT('Ctrl Pts',(170.671555239707,3.38540250062943,48.35));
#78118=CARTESIAN_POINT('Ctrl Pts',(170.560504931957,3.22783091664314,48.5));
#78119=CARTESIAN_POINT('Ctrl Pts',(170.560504931957,3.22783091664314,48.35));
#78120=CARTESIAN_POINT('',(170.857640046626,3.38540250062943,48.5));
#78121=CARTESIAN_POINT('',(170.560504931957,3.22783091664314,48.5));
#78122=CARTESIAN_POINT('Ctrl Pts',(170.857640046626,3.38540250062943,48.5));
#78123=CARTESIAN_POINT('Ctrl Pts',(170.671555239707,3.38540250062943,48.5));
#78124=CARTESIAN_POINT('Ctrl Pts',(170.560504931957,3.22783091664314,48.5));
#78125=CARTESIAN_POINT('',(170.857640046626,3.38540250062943,48.35));
#78126=CARTESIAN_POINT('',(170.857640046626,3.38540250062943,48.5));
#78127=CARTESIAN_POINT('',(170.560504931957,3.22783091664314,48.35));
#78128=CARTESIAN_POINT('Ctrl Pts',(170.857640046626,3.38540250062943,48.35));
#78129=CARTESIAN_POINT('Ctrl Pts',(170.671555239707,3.38540250062943,48.35));
#78130=CARTESIAN_POINT('Ctrl Pts',(170.560504931957,3.22783091664314,48.35));
#78131=CARTESIAN_POINT('',(170.560504931957,3.22783091664314,48.5));
#78132=CARTESIAN_POINT('Ctrl Pts',(171.173533339053,3.2068213224411,48.5));
#78133=CARTESIAN_POINT('Ctrl Pts',(171.173533339053,3.2068213224411,48.35));
#78134=CARTESIAN_POINT('Ctrl Pts',(171.046725649387,3.38540250062943,48.5));
#78135=CARTESIAN_POINT('Ctrl Pts',(171.046725649387,3.38540250062943,48.35));
#78136=CARTESIAN_POINT('Ctrl Pts',(170.857640046626,3.38540250062943,48.5));
#78137=CARTESIAN_POINT('Ctrl Pts',(170.857640046626,3.38540250062943,48.35));
#78138=CARTESIAN_POINT('',(171.173533339053,3.2068213224411,48.5));
#78139=CARTESIAN_POINT('Ctrl Pts',(171.173533339053,3.2068213224411,48.5));
#78140=CARTESIAN_POINT('Ctrl Pts',(171.046725649387,3.38540250062943,48.5));
#78141=CARTESIAN_POINT('Ctrl Pts',(170.857640046626,3.38540250062943,48.5));
#78142=CARTESIAN_POINT('',(171.173533339053,3.2068213224411,48.35));
#78143=CARTESIAN_POINT('',(171.173533339053,3.2068213224411,48.5));
#78144=CARTESIAN_POINT('Ctrl Pts',(171.173533339053,3.2068213224411,48.35));
#78145=CARTESIAN_POINT('Ctrl Pts',(171.046725649387,3.38540250062943,48.35));
#78146=CARTESIAN_POINT('Ctrl Pts',(170.857640046626,3.38540250062943,48.35));
#78147=CARTESIAN_POINT('Ctrl Pts',(171.30034102872,2.48499327898026,48.5));
#78148=CARTESIAN_POINT('Ctrl Pts',(171.30034102872,2.48499327898026,48.35));
#78149=CARTESIAN_POINT('Ctrl Pts',(171.30034102872,3.02824014425278,48.5));
#78150=CARTESIAN_POINT('Ctrl Pts',(171.30034102872,3.02824014425278,48.35));
#78151=CARTESIAN_POINT('Ctrl Pts',(171.173533339053,3.2068213224411,48.5));
#78152=CARTESIAN_POINT('Ctrl Pts',(171.173533339053,3.2068213224411,48.35));
#78153=CARTESIAN_POINT('',(171.30034102872,2.48499327898026,48.5));
#78154=CARTESIAN_POINT('Ctrl Pts',(171.30034102872,2.48499327898026,48.5));
#78155=CARTESIAN_POINT('Ctrl Pts',(171.30034102872,3.02824014425278,48.5));
#78156=CARTESIAN_POINT('Ctrl Pts',(171.173533339053,3.2068213224411,48.5));
#78157=CARTESIAN_POINT('',(171.30034102872,2.48499327898026,48.35));
#78158=CARTESIAN_POINT('',(171.30034102872,2.48499327898026,48.5));
#78159=CARTESIAN_POINT('Ctrl Pts',(171.30034102872,2.48499327898026,48.35));
#78160=CARTESIAN_POINT('Ctrl Pts',(171.30034102872,3.02824014425278,48.35));
#78161=CARTESIAN_POINT('Ctrl Pts',(171.173533339053,3.2068213224411,48.35));
#78162=CARTESIAN_POINT('Ctrl Pts',(171.173533339053,1.76466578245163,48.5));
#78163=CARTESIAN_POINT('Ctrl Pts',(171.173533339053,1.76466578245163,48.35));
#78164=CARTESIAN_POINT('Ctrl Pts',(171.30034102872,1.9447478055954,48.5));
#78165=CARTESIAN_POINT('Ctrl Pts',(171.30034102872,1.9447478055954,48.35));
#78166=CARTESIAN_POINT('Ctrl Pts',(171.30034102872,2.48499327898026,48.5));
#78167=CARTESIAN_POINT('Ctrl Pts',(171.30034102872,2.48499327898026,48.35));
#78168=CARTESIAN_POINT('',(171.173533339053,1.76466578245163,48.5));
#78169=CARTESIAN_POINT('Ctrl Pts',(171.173533339053,1.76466578245163,48.5));
#78170=CARTESIAN_POINT('Ctrl Pts',(171.30034102872,1.9447478055954,48.5));
#78171=CARTESIAN_POINT('Ctrl Pts',(171.30034102872,2.48499327898026,48.5));
#78172=CARTESIAN_POINT('',(171.173533339053,1.76466578245163,48.35));
#78173=CARTESIAN_POINT('',(171.173533339053,1.76466578245163,48.5));
#78174=CARTESIAN_POINT('Ctrl Pts',(171.173533339053,1.76466578245163,48.35));
#78175=CARTESIAN_POINT('Ctrl Pts',(171.30034102872,1.9447478055954,48.35));
#78176=CARTESIAN_POINT('Ctrl Pts',(171.30034102872,2.48499327898026,48.35));
#78177=CARTESIAN_POINT('Ctrl Pts',(170.860641140491,1.58458405733109,48.5));
#78178=CARTESIAN_POINT('Ctrl Pts',(170.860641140491,1.58458405733109,48.35));
#78179=CARTESIAN_POINT('Ctrl Pts',(171.046725649387,1.58458405733109,48.5));
#78180=CARTESIAN_POINT('Ctrl Pts',(171.046725649387,1.58458405733109,48.35));
#78181=CARTESIAN_POINT('Ctrl Pts',(171.173533339053,1.76466578245163,48.5));
#78182=CARTESIAN_POINT('Ctrl Pts',(171.173533339053,1.76466578245163,48.35));
#78183=CARTESIAN_POINT('',(170.860641140491,1.58458405733109,48.5));
#78184=CARTESIAN_POINT('Ctrl Pts',(170.860641140491,1.58458405733109,48.5));
#78185=CARTESIAN_POINT('Ctrl Pts',(171.046725649387,1.58458405733109,48.5));
#78186=CARTESIAN_POINT('Ctrl Pts',(171.173533339053,1.76466578245163,48.5));
#78187=CARTESIAN_POINT('',(170.860641140491,1.58458405733109,48.35));
#78188=CARTESIAN_POINT('',(170.860641140491,1.58458405733109,48.5));
#78189=CARTESIAN_POINT('Ctrl Pts',(170.860641140491,1.58458405733109,48.35));
#78190=CARTESIAN_POINT('Ctrl Pts',(171.046725649387,1.58458405733109,48.35));
#78191=CARTESIAN_POINT('Ctrl Pts',(171.173533339053,1.76466578245163,48.35));
#78192=CARTESIAN_POINT('Ctrl Pts',(170.547748941928,1.76391565799713,48.5));
#78193=CARTESIAN_POINT('Ctrl Pts',(170.547748941928,1.76391565799713,48.35));
#78194=CARTESIAN_POINT('Ctrl Pts',(170.674556631595,1.58458405733109,48.5));
#78195=CARTESIAN_POINT('Ctrl Pts',(170.674556631595,1.58458405733109,48.35));
#78196=CARTESIAN_POINT('Ctrl Pts',(170.860641140491,1.58458405733109,48.5));
#78197=CARTESIAN_POINT('Ctrl Pts',(170.860641140491,1.58458405733109,48.35));
#78198=CARTESIAN_POINT('',(170.547748941928,1.76391565799713,48.5));
#78199=CARTESIAN_POINT('Ctrl Pts',(170.547748941928,1.76391565799713,48.5));
#78200=CARTESIAN_POINT('Ctrl Pts',(170.674556631595,1.58458405733109,48.5));
#78201=CARTESIAN_POINT('Ctrl Pts',(170.860641140491,1.58458405733109,48.5));
#78202=CARTESIAN_POINT('',(170.547748941928,1.76391565799713,48.35));
#78203=CARTESIAN_POINT('',(170.547748941928,1.76391565799713,48.5));
#78204=CARTESIAN_POINT('Ctrl Pts',(170.547748941928,1.76391565799713,48.35));
#78205=CARTESIAN_POINT('Ctrl Pts',(170.674556631595,1.58458405733109,48.35));
#78206=CARTESIAN_POINT('Ctrl Pts',(170.860641140491,1.58458405733109,48.35));
#78207=CARTESIAN_POINT('Ctrl Pts',(170.420941252261,2.48499327898026,48.5));
#78208=CARTESIAN_POINT('Ctrl Pts',(170.420941252261,2.48499327898026,48.35));
#78209=CARTESIAN_POINT('Ctrl Pts',(170.420941252261,1.94324696063995,48.5));
#78210=CARTESIAN_POINT('Ctrl Pts',(170.420941252261,1.94324696063995,48.35));
#78211=CARTESIAN_POINT('Ctrl Pts',(170.547748941928,1.76391565799713,48.5));
#78212=CARTESIAN_POINT('Ctrl Pts',(170.547748941928,1.76391565799713,48.35));
#78213=CARTESIAN_POINT('',(170.420941252261,2.48499327898026,48.5));
#78214=CARTESIAN_POINT('Ctrl Pts',(170.420941252261,2.48499327898026,48.5));
#78215=CARTESIAN_POINT('Ctrl Pts',(170.420941252261,1.94324696063995,48.5));
#78216=CARTESIAN_POINT('Ctrl Pts',(170.547748941928,1.76391565799713,48.5));
#78217=CARTESIAN_POINT('',(170.420941252261,2.48499327898026,48.35));
#78218=CARTESIAN_POINT('',(170.420941252261,2.48499327898026,48.5));
#78219=CARTESIAN_POINT('Ctrl Pts',(170.420941252261,2.48499327898026,48.35));
#78220=CARTESIAN_POINT('Ctrl Pts',(170.420941252261,1.94324696063995,48.35));
#78221=CARTESIAN_POINT('Ctrl Pts',(170.547748941928,1.76391565799713,48.35));
#78222=CARTESIAN_POINT('Ctrl Pts',(170.560504931957,3.22783091664314,48.5));
#78223=CARTESIAN_POINT('Ctrl Pts',(170.560504931957,3.22783091664314,48.35));
#78224=CARTESIAN_POINT('Ctrl Pts',(170.420941252261,3.02673944830894,48.5));
#78225=CARTESIAN_POINT('Ctrl Pts',(170.420941252261,3.02673944830894,48.35));
#78226=CARTESIAN_POINT('Ctrl Pts',(170.420941252261,2.48499327898026,48.5));
#78227=CARTESIAN_POINT('Ctrl Pts',(170.420941252261,2.48499327898026,48.35));
#78228=CARTESIAN_POINT('Ctrl Pts',(170.560504931957,3.22783091664314,48.5));
#78229=CARTESIAN_POINT('Ctrl Pts',(170.420941252261,3.02673944830894,48.5));
#78230=CARTESIAN_POINT('Ctrl Pts',(170.420941252261,2.48499327898026,48.5));
#78231=CARTESIAN_POINT('Ctrl Pts',(170.560504931957,3.22783091664314,48.35));
#78232=CARTESIAN_POINT('Ctrl Pts',(170.420941252261,3.02673944830894,48.35));
#78233=CARTESIAN_POINT('Ctrl Pts',(170.420941252261,2.48499327898026,48.35));
#78234=CARTESIAN_POINT('Ctrl Pts',(170.860641140491,1.36248314380646,48.5));
#78235=CARTESIAN_POINT('Ctrl Pts',(170.860641140491,1.36248314380646,48.35));
#78236=CARTESIAN_POINT('Ctrl Pts',(170.542496580631,1.36248314380646,48.5));
#78237=CARTESIAN_POINT('Ctrl Pts',(170.542496580631,1.36248314380646,48.35));
#78238=CARTESIAN_POINT('Ctrl Pts',(170.360914010555,1.59058684110642,48.5));
#78239=CARTESIAN_POINT('Ctrl Pts',(170.360914010555,1.59058684110642,48.35));
#78240=CARTESIAN_POINT('',(170.860641140491,1.36248314380646,48.5));
#78241=CARTESIAN_POINT('',(170.360914010555,1.59058684110642,48.5));
#78242=CARTESIAN_POINT('Ctrl Pts',(170.860641140491,1.36248314380646,48.5));
#78243=CARTESIAN_POINT('Ctrl Pts',(170.542496580631,1.36248314380646,48.5));
#78244=CARTESIAN_POINT('Ctrl Pts',(170.360914010555,1.59058684110642,48.5));
#78245=CARTESIAN_POINT('',(170.860641140491,1.36248314380646,48.35));
#78246=CARTESIAN_POINT('',(170.860641140491,1.36248314380646,48.5));
#78247=CARTESIAN_POINT('',(170.360914010555,1.59058684110642,48.35));
#78248=CARTESIAN_POINT('Ctrl Pts',(170.860641140491,1.36248314380646,48.35));
#78249=CARTESIAN_POINT('Ctrl Pts',(170.542496580631,1.36248314380646,48.35));
#78250=CARTESIAN_POINT('Ctrl Pts',(170.360914010555,1.59058684110642,48.35));
#78251=CARTESIAN_POINT('',(170.360914010555,1.59058684110642,48.5));
#78252=CARTESIAN_POINT('Ctrl Pts',(171.260572809726,1.49229192733765,48.5));
#78253=CARTESIAN_POINT('Ctrl Pts',(171.260572809726,1.49229192733765,48.35));
#78254=CARTESIAN_POINT('Ctrl Pts',(171.102250952274,1.36248314380646,48.5));
#78255=CARTESIAN_POINT('Ctrl Pts',(171.102250952274,1.36248314380646,48.35));
#78256=CARTESIAN_POINT('Ctrl Pts',(170.860641140491,1.36248314380646,48.5));
#78257=CARTESIAN_POINT('Ctrl Pts',(170.860641140491,1.36248314380646,48.35));
#78258=CARTESIAN_POINT('',(171.260572809726,1.49229192733765,48.5));
#78259=CARTESIAN_POINT('Ctrl Pts',(171.260572809726,1.49229192733765,48.5));
#78260=CARTESIAN_POINT('Ctrl Pts',(171.102250952274,1.36248314380646,48.5));
#78261=CARTESIAN_POINT('Ctrl Pts',(170.860641140491,1.36248314380646,48.5));
#78262=CARTESIAN_POINT('',(171.260572809726,1.49229192733765,48.35));
#78263=CARTESIAN_POINT('',(171.260572809726,1.49229192733765,48.5));
#78264=CARTESIAN_POINT('Ctrl Pts',(171.260572809726,1.49229192733765,48.35));
#78265=CARTESIAN_POINT('Ctrl Pts',(171.102250952274,1.36248314380646,48.35));
#78266=CARTESIAN_POINT('Ctrl Pts',(170.860641140491,1.36248314380646,48.35));
#78267=CARTESIAN_POINT('Ctrl Pts',(171.498431105167,1.85995900630951,48.5));
#78268=CARTESIAN_POINT('Ctrl Pts',(171.498431105167,1.85995900630951,48.35));
#78269=CARTESIAN_POINT('Ctrl Pts',(171.418894667178,1.62210100889206,48.5));
#78270=CARTESIAN_POINT('Ctrl Pts',(171.418894667178,1.62210100889206,48.35));
#78271=CARTESIAN_POINT('Ctrl Pts',(171.260572809726,1.49229192733765,48.5));
#78272=CARTESIAN_POINT('Ctrl Pts',(171.260572809726,1.49229192733765,48.35));
#78273=CARTESIAN_POINT('',(171.498431105167,1.85995900630951,48.5));
#78274=CARTESIAN_POINT('Ctrl Pts',(171.498431105167,1.85995900630951,48.5));
#78275=CARTESIAN_POINT('Ctrl Pts',(171.418894667178,1.62210100889206,48.5));
#78276=CARTESIAN_POINT('Ctrl Pts',(171.260572809726,1.49229192733765,48.5));
#78277=CARTESIAN_POINT('',(171.498431105167,1.85995900630951,48.35));
#78278=CARTESIAN_POINT('',(171.498431105167,1.85995900630951,48.5));
#78279=CARTESIAN_POINT('Ctrl Pts',(171.498431105167,1.85995900630951,48.35));
#78280=CARTESIAN_POINT('Ctrl Pts',(171.418894667178,1.62210100889206,48.35));
#78281=CARTESIAN_POINT('Ctrl Pts',(171.260572809726,1.49229192733765,48.35));
#78282=CARTESIAN_POINT('Ctrl Pts',(171.577966947109,2.48499327898026,48.5));
#78283=CARTESIAN_POINT('Ctrl Pts',(171.577966947109,2.48499327898026,48.35));
#78284=CARTESIAN_POINT('Ctrl Pts',(171.577966947109,2.09781730175018,48.5));
#78285=CARTESIAN_POINT('Ctrl Pts',(171.577966947109,2.09781730175018,48.35));
#78286=CARTESIAN_POINT('Ctrl Pts',(171.498431105167,1.85995900630951,48.5));
#78287=CARTESIAN_POINT('Ctrl Pts',(171.498431105167,1.85995900630951,48.35));
#78288=CARTESIAN_POINT('',(171.577966947109,2.48499327898026,48.5));
#78289=CARTESIAN_POINT('Ctrl Pts',(171.577966947109,2.48499327898026,48.5));
#78290=CARTESIAN_POINT('Ctrl Pts',(171.577966947109,2.09781730175018,48.5));
#78291=CARTESIAN_POINT('Ctrl Pts',(171.498431105167,1.85995900630951,48.5));
#78292=CARTESIAN_POINT('',(171.577966947109,2.48499327898026,48.35));
#78293=CARTESIAN_POINT('',(171.577966947109,2.48499327898026,48.5));
#78294=CARTESIAN_POINT('Ctrl Pts',(171.577966947109,2.48499327898026,48.35));
#78295=CARTESIAN_POINT('Ctrl Pts',(171.577966947109,2.09781730175018,48.35));
#78296=CARTESIAN_POINT('Ctrl Pts',(171.498431105167,1.85995900630951,48.35));
#78297=CARTESIAN_POINT('Ctrl Pts',(171.528444427997,3.00497958064079,48.5));
#78298=CARTESIAN_POINT('Ctrl Pts',(171.528444427997,3.00497958064079,48.35));
#78299=CARTESIAN_POINT('Ctrl Pts',(171.577966947109,2.81214186549187,48.5));
#78300=CARTESIAN_POINT('Ctrl Pts',(171.577966947109,2.81214186549187,48.35));
#78301=CARTESIAN_POINT('Ctrl Pts',(171.577966947109,2.48499327898026,48.5));
#78302=CARTESIAN_POINT('Ctrl Pts',(171.577966947109,2.48499327898026,48.35));
#78303=CARTESIAN_POINT('',(171.528444427997,3.00497958064079,48.5));
#78304=CARTESIAN_POINT('Ctrl Pts',(171.528444427997,3.00497958064079,48.5));
#78305=CARTESIAN_POINT('Ctrl Pts',(171.577966947109,2.81214186549187,48.5));
#78306=CARTESIAN_POINT('Ctrl Pts',(171.577966947109,2.48499327898026,48.5));
#78307=CARTESIAN_POINT('',(171.528444427997,3.00497958064079,48.35));
#78308=CARTESIAN_POINT('',(171.528444427997,3.00497958064079,48.5));
#78309=CARTESIAN_POINT('Ctrl Pts',(171.528444427997,3.00497958064079,48.35));
#78310=CARTESIAN_POINT('Ctrl Pts',(171.577966947109,2.81214186549187,48.35));
#78311=CARTESIAN_POINT('Ctrl Pts',(171.577966947109,2.48499327898026,48.35));
#78312=CARTESIAN_POINT('Ctrl Pts',(171.391882438213,3.33212831616402,48.5));
#78313=CARTESIAN_POINT('Ctrl Pts',(171.391882438213,3.33212831616402,48.35));
#78314=CARTESIAN_POINT('Ctrl Pts',(171.478921908885,3.19781729578972,48.5));
#78315=CARTESIAN_POINT('Ctrl Pts',(171.478921908885,3.19781729578972,48.35));
#78316=CARTESIAN_POINT('Ctrl Pts',(171.528444427997,3.00497958064079,48.5));
#78317=CARTESIAN_POINT('Ctrl Pts',(171.528444427997,3.00497958064079,48.35));
#78318=CARTESIAN_POINT('',(171.391882438213,3.33212831616402,48.5));
#78319=CARTESIAN_POINT('Ctrl Pts',(171.391882438213,3.33212831616402,48.5));
#78320=CARTESIAN_POINT('Ctrl Pts',(171.478921908885,3.19781729578972,48.5));
#78321=CARTESIAN_POINT('Ctrl Pts',(171.528444427997,3.00497958064079,48.5));
#78322=CARTESIAN_POINT('',(171.391882438213,3.33212831616402,48.35));
#78323=CARTESIAN_POINT('',(171.391882438213,3.33212831616402,48.5));
#78324=CARTESIAN_POINT('Ctrl Pts',(171.391882438213,3.33212831616402,48.35));
#78325=CARTESIAN_POINT('Ctrl Pts',(171.478921908885,3.19781729578972,48.35));
#78326=CARTESIAN_POINT('Ctrl Pts',(171.528444427997,3.00497958064079,48.35));
#78327=CARTESIAN_POINT('Ctrl Pts',(171.171282667667,3.5377217233181,48.5));
#78328=CARTESIAN_POINT('Ctrl Pts',(171.171282667667,3.5377217233181,48.35));
#78329=CARTESIAN_POINT('Ctrl Pts',(171.30484296754,3.46643933653831,48.5));
#78330=CARTESIAN_POINT('Ctrl Pts',(171.30484296754,3.46643933653831,48.35));
#78331=CARTESIAN_POINT('Ctrl Pts',(171.391882438213,3.33212831616402,48.5));
#78332=CARTESIAN_POINT('Ctrl Pts',(171.391882438213,3.33212831616402,48.35));
#78333=CARTESIAN_POINT('',(171.171282667667,3.5377217233181,48.5));
#78334=CARTESIAN_POINT('Ctrl Pts',(171.171282667667,3.5377217233181,48.5));
#78335=CARTESIAN_POINT('Ctrl Pts',(171.30484296754,3.46643933653831,48.5));
#78336=CARTESIAN_POINT('Ctrl Pts',(171.391882438213,3.33212831616402,48.5));
#78337=CARTESIAN_POINT('',(171.171282667667,3.5377217233181,48.35));
#78338=CARTESIAN_POINT('',(171.171282667667,3.5377217233181,48.5));
#78339=CARTESIAN_POINT('Ctrl Pts',(171.171282667667,3.5377217233181,48.35));
#78340=CARTESIAN_POINT('Ctrl Pts',(171.30484296754,3.46643933653831,48.35));
#78341=CARTESIAN_POINT('Ctrl Pts',(171.391882438213,3.33212831616402,48.35));
#78342=CARTESIAN_POINT('Ctrl Pts',(170.860641140491,3.60900411009789,48.5));
#78343=CARTESIAN_POINT('Ctrl Pts',(170.860641140491,3.60900411009789,48.35));
#78344=CARTESIAN_POINT('Ctrl Pts',(171.037721771747,3.60900411009789,48.5));
#78345=CARTESIAN_POINT('Ctrl Pts',(171.037721771747,3.60900411009789,48.35));
#78346=CARTESIAN_POINT('Ctrl Pts',(171.171282667667,3.5377217233181,48.5));
#78347=CARTESIAN_POINT('Ctrl Pts',(171.171282667667,3.5377217233181,48.35));
#78348=CARTESIAN_POINT('',(170.860641140491,3.60900411009789,48.5));
#78349=CARTESIAN_POINT('Ctrl Pts',(170.860641140491,3.60900411009789,48.5));
#78350=CARTESIAN_POINT('Ctrl Pts',(171.037721771747,3.60900411009789,48.5));
#78351=CARTESIAN_POINT('Ctrl Pts',(171.171282667667,3.5377217233181,48.5));
#78352=CARTESIAN_POINT('',(170.860641140491,3.60900411009789,48.35));
#78353=CARTESIAN_POINT('',(170.860641140491,3.60900411009789,48.5));
#78354=CARTESIAN_POINT('Ctrl Pts',(170.860641140491,3.60900411009789,48.35));
#78355=CARTESIAN_POINT('Ctrl Pts',(171.037721771747,3.60900411009789,48.35));
#78356=CARTESIAN_POINT('Ctrl Pts',(171.171282667667,3.5377217233181,48.35));
#78357=CARTESIAN_POINT('Ctrl Pts',(170.462210316211,3.47994545102119,48.5));
#78358=CARTESIAN_POINT('Ctrl Pts',(170.462210316211,3.47994545102119,48.35));
#78359=CARTESIAN_POINT('Ctrl Pts',(170.620532173663,3.60900411009789,48.5));
#78360=CARTESIAN_POINT('Ctrl Pts',(170.620532173663,3.60900411009789,48.35));
#78361=CARTESIAN_POINT('Ctrl Pts',(170.860641140491,3.60900411009789,48.5));
#78362=CARTESIAN_POINT('Ctrl Pts',(170.860641140491,3.60900411009789,48.35));
#78363=CARTESIAN_POINT('',(170.462210316211,3.47994545102119,48.5));
#78364=CARTESIAN_POINT('Ctrl Pts',(170.462210316211,3.47994545102119,48.5));
#78365=CARTESIAN_POINT('Ctrl Pts',(170.620532173663,3.60900411009789,48.5));
#78366=CARTESIAN_POINT('Ctrl Pts',(170.860641140491,3.60900411009789,48.5));
#78367=CARTESIAN_POINT('',(170.462210316211,3.47994545102119,48.35));
#78368=CARTESIAN_POINT('',(170.462210316211,3.47994545102119,48.5));
#78369=CARTESIAN_POINT('Ctrl Pts',(170.462210316211,3.47994545102119,48.35));
#78370=CARTESIAN_POINT('Ctrl Pts',(170.620532173663,3.60900411009789,48.35));
#78371=CARTESIAN_POINT('Ctrl Pts',(170.860641140491,3.60900411009789,48.35));
#78372=CARTESIAN_POINT('Ctrl Pts',(170.223601598293,3.11302864551544,48.5));
#78373=CARTESIAN_POINT('Ctrl Pts',(170.223601598293,3.11302864551544,48.35));
#78374=CARTESIAN_POINT('Ctrl Pts',(170.303888160735,3.3508867919445,48.5));
#78375=CARTESIAN_POINT('Ctrl Pts',(170.303888160735,3.3508867919445,48.35));
#78376=CARTESIAN_POINT('Ctrl Pts',(170.462210316211,3.47994545102119,48.5));
#78377=CARTESIAN_POINT('Ctrl Pts',(170.462210316211,3.47994545102119,48.35));
#78378=CARTESIAN_POINT('',(170.223601598293,3.11302864551544,48.5));
#78379=CARTESIAN_POINT('Ctrl Pts',(170.223601598293,3.11302864551544,48.5));
#78380=CARTESIAN_POINT('Ctrl Pts',(170.303888160735,3.3508867919445,48.5));
#78381=CARTESIAN_POINT('Ctrl Pts',(170.462210316211,3.47994545102119,48.5));
#78382=CARTESIAN_POINT('',(170.223601598293,3.11302864551544,48.35));
#78383=CARTESIAN_POINT('',(170.223601598293,3.11302864551544,48.5));
#78384=CARTESIAN_POINT('Ctrl Pts',(170.223601598293,3.11302864551544,48.35));
#78385=CARTESIAN_POINT('Ctrl Pts',(170.303888160735,3.3508867919445,48.35));
#78386=CARTESIAN_POINT('Ctrl Pts',(170.462210316211,3.47994545102119,48.35));
#78387=CARTESIAN_POINT('Ctrl Pts',(170.143315333873,2.48499327898026,48.5));
#78388=CARTESIAN_POINT('Ctrl Pts',(170.143315333873,2.48499327898026,48.35));
#78389=CARTESIAN_POINT('Ctrl Pts',(170.143315333873,2.87517049908638,48.5));
#78390=CARTESIAN_POINT('Ctrl Pts',(170.143315333873,2.87517049908638,48.35));
#78391=CARTESIAN_POINT('Ctrl Pts',(170.223601598293,3.11302864551544,48.5));
#78392=CARTESIAN_POINT('Ctrl Pts',(170.223601598293,3.11302864551544,48.35));
#78393=CARTESIAN_POINT('',(170.143315333873,2.48499327898026,48.5));
#78394=CARTESIAN_POINT('Ctrl Pts',(170.143315333873,2.48499327898026,48.5));
#78395=CARTESIAN_POINT('Ctrl Pts',(170.143315333873,2.87517049908638,48.5));
#78396=CARTESIAN_POINT('Ctrl Pts',(170.223601598293,3.11302864551544,48.5));
#78397=CARTESIAN_POINT('',(170.143315333873,2.48499327898026,48.35));
#78398=CARTESIAN_POINT('',(170.143315333873,2.48499327898026,48.5));
#78399=CARTESIAN_POINT('Ctrl Pts',(170.143315333873,2.48499327898026,48.35));
#78400=CARTESIAN_POINT('Ctrl Pts',(170.143315333873,2.87517049908638,48.35));
#78401=CARTESIAN_POINT('Ctrl Pts',(170.223601598293,3.11302864551544,48.35));
#78402=CARTESIAN_POINT('Ctrl Pts',(170.360914010555,1.59058684110642,48.5));
#78403=CARTESIAN_POINT('Ctrl Pts',(170.360914010555,1.59058684110642,48.35));
#78404=CARTESIAN_POINT('Ctrl Pts',(170.143315333873,1.86521166563034,48.5));
#78405=CARTESIAN_POINT('Ctrl Pts',(170.143315333873,1.86521166563034,48.35));
#78406=CARTESIAN_POINT('Ctrl Pts',(170.143315333873,2.48499327898026,48.5));
#78407=CARTESIAN_POINT('Ctrl Pts',(170.143315333873,2.48499327898026,48.35));
#78408=CARTESIAN_POINT('Ctrl Pts',(170.360914010555,1.59058684110642,48.5));
#78409=CARTESIAN_POINT('Ctrl Pts',(170.143315333873,1.86521166563034,48.5));
#78410=CARTESIAN_POINT('Ctrl Pts',(170.143315333873,2.48499327898026,48.5));
#78411=CARTESIAN_POINT('Ctrl Pts',(170.360914010555,1.59058684110642,48.35));
#78412=CARTESIAN_POINT('Ctrl Pts',(170.143315333873,1.86521166563034,48.35));
#78413=CARTESIAN_POINT('Ctrl Pts',(170.143315333873,2.48499327898026,48.35));
#78414=CARTESIAN_POINT('Origin',(169.999999914318,2.48574362695217,48.35));
#78415=CARTESIAN_POINT('Ctrl Pts',(169.170873302966,2.58854025602341,48.5));
#78416=CARTESIAN_POINT('Ctrl Pts',(169.170873302966,2.58854025602341,48.35));
#78417=CARTESIAN_POINT('Ctrl Pts',(168.987790036947,2.58854025602341,48.5));
#78418=CARTESIAN_POINT('Ctrl Pts',(168.987790036947,2.58854025602341,48.35));
#78419=CARTESIAN_POINT('Ctrl Pts',(168.860232073814,2.45723062753677,48.5));
#78420=CARTESIAN_POINT('Ctrl Pts',(168.860232073814,2.45723062753677,48.35));
#78421=CARTESIAN_POINT('',(169.170873302966,2.58854025602341,48.5));
#78422=CARTESIAN_POINT('',(168.860232073814,2.45723062753677,48.5));
#78423=CARTESIAN_POINT('Ctrl Pts',(169.170873302966,2.58854025602341,48.5));
#78424=CARTESIAN_POINT('Ctrl Pts',(168.987790036947,2.58854025602341,48.5));
#78425=CARTESIAN_POINT('Ctrl Pts',(168.860232073814,2.45723062753677,48.5));
#78426=CARTESIAN_POINT('',(169.170873302966,2.58854025602341,48.35));
#78427=CARTESIAN_POINT('',(169.170873302966,2.58854025602341,48.5));
#78428=CARTESIAN_POINT('',(168.860232073814,2.45723062753677,48.35));
#78429=CARTESIAN_POINT('Ctrl Pts',(169.170873302966,2.58854025602341,48.35));
#78430=CARTESIAN_POINT('Ctrl Pts',(168.987790036947,2.58854025602341,48.35));
#78431=CARTESIAN_POINT('Ctrl Pts',(168.860232073814,2.45723062753677,48.35));
#78432=CARTESIAN_POINT('',(168.860232073814,2.45723062753677,48.5));
#78433=CARTESIAN_POINT('Ctrl Pts',(169.477012295276,2.45723062753677,48.5));
#78434=CARTESIAN_POINT('Ctrl Pts',(169.477012295276,2.45723062753677,48.35));
#78435=CARTESIAN_POINT('Ctrl Pts',(169.35545726493,2.58854025602341,48.5));
#78436=CARTESIAN_POINT('Ctrl Pts',(169.35545726493,2.58854025602341,48.35));
#78437=CARTESIAN_POINT('Ctrl Pts',(169.170873302966,2.58854025602341,48.5));
#78438=CARTESIAN_POINT('Ctrl Pts',(169.170873302966,2.58854025602341,48.35));
#78439=CARTESIAN_POINT('',(169.477012295276,2.45723062753677,48.5));
#78440=CARTESIAN_POINT('Ctrl Pts',(169.477012295276,2.45723062753677,48.5));
#78441=CARTESIAN_POINT('Ctrl Pts',(169.35545726493,2.58854025602341,48.5));
#78442=CARTESIAN_POINT('Ctrl Pts',(169.170873302966,2.58854025602341,48.5));
#78443=CARTESIAN_POINT('',(169.477012295276,2.45723062753677,48.35));
#78444=CARTESIAN_POINT('',(169.477012295276,2.45723062753677,48.5));
#78445=CARTESIAN_POINT('Ctrl Pts',(169.477012295276,2.45723062753677,48.35));
#78446=CARTESIAN_POINT('Ctrl Pts',(169.35545726493,2.58854025602341,48.35));
#78447=CARTESIAN_POINT('Ctrl Pts',(169.170873302966,2.58854025602341,48.35));
#78448=CARTESIAN_POINT('Ctrl Pts',(169.598567623645,2.09781730175018,48.5));
#78449=CARTESIAN_POINT('Ctrl Pts',(169.598567623645,2.09781730175018,48.35));
#78450=CARTESIAN_POINT('Ctrl Pts',(169.598567623645,2.32592099905014,48.5));
#78451=CARTESIAN_POINT('Ctrl Pts',(169.598567623645,2.32592099905014,48.35));
#78452=CARTESIAN_POINT('Ctrl Pts',(169.477012295276,2.45723062753677,48.5));
#78453=CARTESIAN_POINT('Ctrl Pts',(169.477012295276,2.45723062753677,48.35));
#78454=CARTESIAN_POINT('',(169.598567623645,2.09781730175018,48.5));
#78455=CARTESIAN_POINT('Ctrl Pts',(169.598567623645,2.09781730175018,48.5));
#78456=CARTESIAN_POINT('Ctrl Pts',(169.598567623645,2.32592099905014,48.5));
#78457=CARTESIAN_POINT('Ctrl Pts',(169.477012295276,2.45723062753677,48.5));
#78458=CARTESIAN_POINT('',(169.598567623645,2.09781730175018,48.35));
#78459=CARTESIAN_POINT('',(169.598567623645,2.09781730175018,48.5));
#78460=CARTESIAN_POINT('Ctrl Pts',(169.598567623645,2.09781730175018,48.35));
#78461=CARTESIAN_POINT('Ctrl Pts',(169.598567623645,2.32592099905014,48.35));
#78462=CARTESIAN_POINT('Ctrl Pts',(169.477012295276,2.45723062753677,48.35));
#78463=CARTESIAN_POINT('Ctrl Pts',(169.475511748344,1.72264659404755,48.5));
#78464=CARTESIAN_POINT('Ctrl Pts',(169.475511748344,1.72264659404755,48.35));
#78465=CARTESIAN_POINT('Ctrl Pts',(169.598567623645,1.86070942878723,48.5));
#78466=CARTESIAN_POINT('Ctrl Pts',(169.598567623645,1.86070942878723,48.35));
#78467=CARTESIAN_POINT('Ctrl Pts',(169.598567623645,2.09781730175018,48.5));
#78468=CARTESIAN_POINT('Ctrl Pts',(169.598567623645,2.09781730175018,48.35));
#78469=CARTESIAN_POINT('',(169.475511748344,1.72264659404755,48.5));
#78470=CARTESIAN_POINT('Ctrl Pts',(169.475511748344,1.72264659404755,48.5));
#78471=CARTESIAN_POINT('Ctrl Pts',(169.598567623645,1.86070942878723,48.5));
#78472=CARTESIAN_POINT('Ctrl Pts',(169.598567623645,2.09781730175018,48.5));
#78473=CARTESIAN_POINT('',(169.475511748344,1.72264659404755,48.35));
#78474=CARTESIAN_POINT('',(169.475511748344,1.72264659404755,48.5));
#78475=CARTESIAN_POINT('Ctrl Pts',(169.475511748344,1.72264659404755,48.35));
#78476=CARTESIAN_POINT('Ctrl Pts',(169.598567623645,1.86070942878723,48.35));
#78477=CARTESIAN_POINT('Ctrl Pts',(169.598567623645,2.09781730175018,48.35));
#78478=CARTESIAN_POINT('Ctrl Pts',(169.181378025562,1.58458405733109,48.5));
#78479=CARTESIAN_POINT('Ctrl Pts',(169.181378025562,1.58458405733109,48.35));
#78480=CARTESIAN_POINT('Ctrl Pts',(169.352455873042,1.58458405733109,48.5));
#78481=CARTESIAN_POINT('Ctrl Pts',(169.352455873042,1.58458405733109,48.35));
#78482=CARTESIAN_POINT('Ctrl Pts',(169.475511748344,1.72264659404755,48.5));
#78483=CARTESIAN_POINT('Ctrl Pts',(169.475511748344,1.72264659404755,48.35));
#78484=CARTESIAN_POINT('',(169.181378025562,1.58458405733109,48.5));
#78485=CARTESIAN_POINT('Ctrl Pts',(169.181378025562,1.58458405733109,48.5));
#78486=CARTESIAN_POINT('Ctrl Pts',(169.352455873042,1.58458405733109,48.5));
#78487=CARTESIAN_POINT('Ctrl Pts',(169.475511748344,1.72264659404755,48.5));
#78488=CARTESIAN_POINT('',(169.181378025562,1.58458405733109,48.35));
#78489=CARTESIAN_POINT('',(169.181378025562,1.58458405733109,48.5));
#78490=CARTESIAN_POINT('Ctrl Pts',(169.181378025562,1.58458405733109,48.35));
#78491=CARTESIAN_POINT('Ctrl Pts',(169.352455873042,1.58458405733109,48.35));
#78492=CARTESIAN_POINT('Ctrl Pts',(169.475511748344,1.72264659404755,48.35));
#78493=CARTESIAN_POINT('Ctrl Pts',(168.957776416093,1.65136420726776,48.5));
#78494=CARTESIAN_POINT('Ctrl Pts',(168.957776416093,1.65136420726776,48.35));
#78495=CARTESIAN_POINT('Ctrl Pts',(169.064324934036,1.58458405733109,48.5));
#78496=CARTESIAN_POINT('Ctrl Pts',(169.064324934036,1.58458405733109,48.35));
#78497=CARTESIAN_POINT('Ctrl Pts',(169.181378025562,1.58458405733109,48.5));
#78498=CARTESIAN_POINT('Ctrl Pts',(169.181378025562,1.58458405733109,48.35));
#78499=CARTESIAN_POINT('',(168.957776416093,1.65136420726776,48.5));
#78500=CARTESIAN_POINT('Ctrl Pts',(168.957776416093,1.65136420726776,48.5));
#78501=CARTESIAN_POINT('Ctrl Pts',(169.064324934036,1.58458405733109,48.5));
#78502=CARTESIAN_POINT('Ctrl Pts',(169.181378025562,1.58458405733109,48.5));
#78503=CARTESIAN_POINT('',(168.957776416093,1.65136420726776,48.35));
#78504=CARTESIAN_POINT('',(168.957776416093,1.65136420726776,48.5));
#78505=CARTESIAN_POINT('Ctrl Pts',(168.957776416093,1.65136420726776,48.35));
#78506=CARTESIAN_POINT('Ctrl Pts',(169.064324934036,1.58458405733109,48.35));
#78507=CARTESIAN_POINT('Ctrl Pts',(169.181378025562,1.58458405733109,48.35));
#78508=CARTESIAN_POINT('Ctrl Pts',(168.791951078922,1.84570276737213,48.5));
#78509=CARTESIAN_POINT('Ctrl Pts',(168.791951078922,1.84570276737213,48.35));
#78510=CARTESIAN_POINT('Ctrl Pts',(168.851227898151,1.71814465522766,48.5));
#78511=CARTESIAN_POINT('Ctrl Pts',(168.851227898151,1.71814465522766,48.35));
#78512=CARTESIAN_POINT('Ctrl Pts',(168.957776416093,1.65136420726776,48.5));
#78513=CARTESIAN_POINT('Ctrl Pts',(168.957776416093,1.65136420726776,48.35));
#78514=CARTESIAN_POINT('',(168.791951078922,1.84570276737213,48.5));
#78515=CARTESIAN_POINT('Ctrl Pts',(168.791951078922,1.84570276737213,48.5));
#78516=CARTESIAN_POINT('Ctrl Pts',(168.851227898151,1.71814465522766,48.5));
#78517=CARTESIAN_POINT('Ctrl Pts',(168.957776416093,1.65136420726776,48.5));
#78518=CARTESIAN_POINT('',(168.791951078922,1.84570276737213,48.35));
#78519=CARTESIAN_POINT('',(168.791951078922,1.84570276737213,48.5));
#78520=CARTESIAN_POINT('Ctrl Pts',(168.791951078922,1.84570276737213,48.35));
#78521=CARTESIAN_POINT('Ctrl Pts',(168.851227898151,1.71814465522766,48.35));
#78522=CARTESIAN_POINT('Ctrl Pts',(168.957776416093,1.65136420726776,48.35));
#78523=CARTESIAN_POINT('Ctrl Pts',(168.732673961669,2.1128241121769,48.5));
#78524=CARTESIAN_POINT('Ctrl Pts',(168.732673961669,2.1128241121769,48.35));
#78525=CARTESIAN_POINT('Ctrl Pts',(168.732673961669,1.97326058149338,48.5));
#78526=CARTESIAN_POINT('Ctrl Pts',(168.732673961669,1.97326058149338,48.35));
#78527=CARTESIAN_POINT('Ctrl Pts',(168.791951078922,1.84570276737213,48.5));
#78528=CARTESIAN_POINT('Ctrl Pts',(168.791951078922,1.84570276737213,48.35));
#78529=CARTESIAN_POINT('',(168.732673961669,2.1128241121769,48.5));
#78530=CARTESIAN_POINT('Ctrl Pts',(168.732673961669,2.1128241121769,48.5));
#78531=CARTESIAN_POINT('Ctrl Pts',(168.732673961669,1.97326058149338,48.5));
#78532=CARTESIAN_POINT('Ctrl Pts',(168.791951078922,1.84570276737213,48.5));
#78533=CARTESIAN_POINT('',(168.732673961669,2.1128241121769,48.35));
#78534=CARTESIAN_POINT('',(168.732673961669,2.1128241121769,48.5));
#78535=CARTESIAN_POINT('Ctrl Pts',(168.732673961669,2.1128241121769,48.35));
#78536=CARTESIAN_POINT('Ctrl Pts',(168.732673961669,1.97326058149338,48.35));
#78537=CARTESIAN_POINT('Ctrl Pts',(168.791951078922,1.84570276737213,48.35));
#78538=CARTESIAN_POINT('Ctrl Pts',(168.860232073814,2.45723062753677,48.5));
#78539=CARTESIAN_POINT('Ctrl Pts',(168.860232073814,2.45723062753677,48.35));
#78540=CARTESIAN_POINT('Ctrl Pts',(168.732673961669,2.32592099905014,48.5));
#78541=CARTESIAN_POINT('Ctrl Pts',(168.732673961669,2.32592099905014,48.35));
#78542=CARTESIAN_POINT('Ctrl Pts',(168.732673961669,2.1128241121769,48.5));
#78543=CARTESIAN_POINT('Ctrl Pts',(168.732673961669,2.1128241121769,48.35));
#78544=CARTESIAN_POINT('Ctrl Pts',(168.860232073814,2.45723062753677,48.5));
#78545=CARTESIAN_POINT('Ctrl Pts',(168.732673961669,2.32592099905014,48.5));
#78546=CARTESIAN_POINT('Ctrl Pts',(168.732673961669,2.1128241121769,48.5));
#78547=CARTESIAN_POINT('Ctrl Pts',(168.860232073814,2.45723062753677,48.35));
#78548=CARTESIAN_POINT('Ctrl Pts',(168.732673961669,2.32592099905014,48.35));
#78549=CARTESIAN_POINT('Ctrl Pts',(168.732673961669,2.1128241121769,48.35));
#78550=CARTESIAN_POINT('Ctrl Pts',(169.211391646415,3.60900411009789,48.5));
#78551=CARTESIAN_POINT('Ctrl Pts',(169.211391646415,3.60900411009789,48.35));
#78552=CARTESIAN_POINT('Ctrl Pts',(169.471009511501,3.60900411009789,48.5));
#78553=CARTESIAN_POINT('Ctrl Pts',(169.471009511501,3.60900411009789,48.35));
#78554=CARTESIAN_POINT('Ctrl Pts',(169.636834997684,3.46343794465065,48.5));
#78555=CARTESIAN_POINT('Ctrl Pts',(169.636834997684,3.46343794465065,48.35));
#78556=CARTESIAN_POINT('',(169.211391646415,3.60900411009789,48.5));
#78557=CARTESIAN_POINT('',(169.636834997684,3.46343794465065,48.5));
#78558=CARTESIAN_POINT('Ctrl Pts',(169.211391646415,3.60900411009789,48.5));
#78559=CARTESIAN_POINT('Ctrl Pts',(169.471009511501,3.60900411009789,48.5));
#78560=CARTESIAN_POINT('Ctrl Pts',(169.636834997684,3.46343794465065,48.5));
#78561=CARTESIAN_POINT('',(169.211391646415,3.60900411009789,48.35));
#78562=CARTESIAN_POINT('',(169.211391646415,3.60900411009789,48.5));
#78563=CARTESIAN_POINT('',(169.636834997684,3.46343794465065,48.35));
#78564=CARTESIAN_POINT('Ctrl Pts',(169.211391646415,3.60900411009789,48.35));
#78565=CARTESIAN_POINT('Ctrl Pts',(169.471009511501,3.60900411009789,48.35));
#78566=CARTESIAN_POINT('Ctrl Pts',(169.636834997684,3.46343794465065,48.35));
#78567=CARTESIAN_POINT('',(169.636834997684,3.46343794465065,48.5));
#78568=CARTESIAN_POINT('Ctrl Pts',(168.657639909536,3.35688957571983,48.5));
#78569=CARTESIAN_POINT('Ctrl Pts',(168.657639909536,3.35688957571983,48.35));
#78570=CARTESIAN_POINT('Ctrl Pts',(168.863233465701,3.60900411009789,48.5));
#78571=CARTESIAN_POINT('Ctrl Pts',(168.863233465701,3.60900411009789,48.35));
#78572=CARTESIAN_POINT('Ctrl Pts',(169.211391646415,3.60900411009789,48.5));
#78573=CARTESIAN_POINT('Ctrl Pts',(169.211391646415,3.60900411009789,48.35));
#78574=CARTESIAN_POINT('',(168.657639909536,3.35688957571983,48.5));
#78575=CARTESIAN_POINT('Ctrl Pts',(168.657639909536,3.35688957571983,48.5));
#78576=CARTESIAN_POINT('Ctrl Pts',(168.863233465701,3.60900411009789,48.5));
#78577=CARTESIAN_POINT('Ctrl Pts',(169.211391646415,3.60900411009789,48.5));
#78578=CARTESIAN_POINT('',(168.657639909536,3.35688957571983,48.35));
#78579=CARTESIAN_POINT('',(168.657639909536,3.35688957571983,48.5));
#78580=CARTESIAN_POINT('Ctrl Pts',(168.657639909536,3.35688957571983,48.35));
#78581=CARTESIAN_POINT('Ctrl Pts',(168.863233465701,3.60900411009789,48.35));
#78582=CARTESIAN_POINT('Ctrl Pts',(169.211391646415,3.60900411009789,48.35));
#78583=CARTESIAN_POINT('Ctrl Pts',(168.422032881528,2.42946797609329,48.5));
#78584=CARTESIAN_POINT('Ctrl Pts',(168.422032881528,2.42946797609329,48.35));
#78585=CARTESIAN_POINT('Ctrl Pts',(168.422032881528,3.0672579407692,48.5));
#78586=CARTESIAN_POINT('Ctrl Pts',(168.422032881528,3.0672579407692,48.35));
#78587=CARTESIAN_POINT('Ctrl Pts',(168.657639909536,3.35688957571983,48.5));
#78588=CARTESIAN_POINT('Ctrl Pts',(168.657639909536,3.35688957571983,48.35));
#78589=CARTESIAN_POINT('',(168.422032881528,2.42946797609329,48.5));
#78590=CARTESIAN_POINT('Ctrl Pts',(168.422032881528,2.42946797609329,48.5));
#78591=CARTESIAN_POINT('Ctrl Pts',(168.422032881528,3.0672579407692,48.5));
#78592=CARTESIAN_POINT('Ctrl Pts',(168.657639909536,3.35688957571983,48.5));
#78593=CARTESIAN_POINT('',(168.422032881528,2.42946797609329,48.35));
#78594=CARTESIAN_POINT('',(168.422032881528,2.42946797609329,48.5));
#78595=CARTESIAN_POINT('Ctrl Pts',(168.422032881528,2.42946797609329,48.35));
#78596=CARTESIAN_POINT('Ctrl Pts',(168.422032881528,3.0672579407692,48.35));
#78597=CARTESIAN_POINT('Ctrl Pts',(168.657639909536,3.35688957571983,48.35));
#78598=CARTESIAN_POINT('Ctrl Pts',(168.635129768401,1.61084586381912,48.5));
#78599=CARTESIAN_POINT('Ctrl Pts',(168.635129768401,1.61084586381912,48.35));
#78600=CARTESIAN_POINT('Ctrl Pts',(168.422032881528,1.85920888185501,48.5));
#78601=CARTESIAN_POINT('Ctrl Pts',(168.422032881528,1.85920888185501,48.35));
#78602=CARTESIAN_POINT('Ctrl Pts',(168.422032881528,2.42946797609329,48.5));
#78603=CARTESIAN_POINT('Ctrl Pts',(168.422032881528,2.42946797609329,48.35));
#78604=CARTESIAN_POINT('',(168.635129768401,1.61084586381912,48.5));
#78605=CARTESIAN_POINT('Ctrl Pts',(168.635129768401,1.61084586381912,48.5));
#78606=CARTESIAN_POINT('Ctrl Pts',(168.422032881528,1.85920888185501,48.5));
#78607=CARTESIAN_POINT('Ctrl Pts',(168.422032881528,2.42946797609329,48.5));
#78608=CARTESIAN_POINT('',(168.635129768401,1.61084586381912,48.35));
#78609=CARTESIAN_POINT('',(168.635129768401,1.61084586381912,48.5));
#78610=CARTESIAN_POINT('Ctrl Pts',(168.635129768401,1.61084586381912,48.35));
#78611=CARTESIAN_POINT('Ctrl Pts',(168.422032881528,1.85920888185501,48.35));
#78612=CARTESIAN_POINT('Ctrl Pts',(168.422032881528,2.42946797609329,48.35));
#78613=CARTESIAN_POINT('Ctrl Pts',(169.185880113393,1.36248314380646,48.5));
#78614=CARTESIAN_POINT('Ctrl Pts',(169.185880113393,1.36248314380646,48.35));
#78615=CARTESIAN_POINT('Ctrl Pts',(168.848226506263,1.36248314380646,48.5));
#78616=CARTESIAN_POINT('Ctrl Pts',(168.848226506263,1.36248314380646,48.35));
#78617=CARTESIAN_POINT('Ctrl Pts',(168.635129768401,1.61084586381912,48.5));
#78618=CARTESIAN_POINT('Ctrl Pts',(168.635129768401,1.61084586381912,48.35));
#78619=CARTESIAN_POINT('',(169.185880113393,1.36248314380646,48.5));
#78620=CARTESIAN_POINT('Ctrl Pts',(169.185880113393,1.36248314380646,48.5));
#78621=CARTESIAN_POINT('Ctrl Pts',(168.848226506263,1.36248314380646,48.5));
#78622=CARTESIAN_POINT('Ctrl Pts',(168.635129768401,1.61084586381912,48.5));
#78623=CARTESIAN_POINT('',(169.185880113393,1.36248314380646,48.35));
#78624=CARTESIAN_POINT('',(169.185880113393,1.36248314380646,48.5));
#78625=CARTESIAN_POINT('Ctrl Pts',(169.185880113393,1.36248314380646,48.35));
#78626=CARTESIAN_POINT('Ctrl Pts',(168.848226506263,1.36248314380646,48.35));
#78627=CARTESIAN_POINT('Ctrl Pts',(168.635129768401,1.61084586381912,48.35));
#78628=CARTESIAN_POINT('Ctrl Pts',(169.540041226894,1.45702594518662,48.5));
#78629=CARTESIAN_POINT('Ctrl Pts',(169.540041226894,1.45702594518662,48.35));
#78630=CARTESIAN_POINT('Ctrl Pts',(169.383970040828,1.36248314380646,48.5));
#78631=CARTESIAN_POINT('Ctrl Pts',(169.383970040828,1.36248314380646,48.35));
#78632=CARTESIAN_POINT('Ctrl Pts',(169.185880113393,1.36248314380646,48.5));
#78633=CARTESIAN_POINT('Ctrl Pts',(169.185880113393,1.36248314380646,48.35));
#78634=CARTESIAN_POINT('',(169.540041226894,1.45702594518662,48.5));
#78635=CARTESIAN_POINT('Ctrl Pts',(169.540041226894,1.45702594518662,48.5));
#78636=CARTESIAN_POINT('Ctrl Pts',(169.383970040828,1.36248314380646,48.5));
#78637=CARTESIAN_POINT('Ctrl Pts',(169.185880113393,1.36248314380646,48.5));
#78638=CARTESIAN_POINT('',(169.540041226894,1.45702594518662,48.35));
#78639=CARTESIAN_POINT('',(169.540041226894,1.45702594518662,48.5));
#78640=CARTESIAN_POINT('Ctrl Pts',(169.540041226894,1.45702594518662,48.35));
#78641=CARTESIAN_POINT('Ctrl Pts',(169.383970040828,1.36248314380646,48.35));
#78642=CARTESIAN_POINT('Ctrl Pts',(169.185880113393,1.36248314380646,48.35));
#78643=CARTESIAN_POINT('Ctrl Pts',(169.785402555019,1.7293998003006,48.5));
#78644=CARTESIAN_POINT('Ctrl Pts',(169.785402555019,1.7293998003006,48.35));
#78645=CARTESIAN_POINT('Ctrl Pts',(169.696111816913,1.55156904459,48.5));
#78646=CARTESIAN_POINT('Ctrl Pts',(169.696111816913,1.55156904459,48.35));
#78647=CARTESIAN_POINT('Ctrl Pts',(169.540041226894,1.45702594518662,48.5));
#78648=CARTESIAN_POINT('Ctrl Pts',(169.540041226894,1.45702594518662,48.35));
#78649=CARTESIAN_POINT('',(169.785402555019,1.7293998003006,48.5));
#78650=CARTESIAN_POINT('Ctrl Pts',(169.785402555019,1.7293998003006,48.5));
#78651=CARTESIAN_POINT('Ctrl Pts',(169.696111816913,1.55156904459,48.5));
#78652=CARTESIAN_POINT('Ctrl Pts',(169.540041226894,1.45702594518662,48.5));
#78653=CARTESIAN_POINT('',(169.785402555019,1.7293998003006,48.35));
#78654=CARTESIAN_POINT('',(169.785402555019,1.7293998003006,48.5));
#78655=CARTESIAN_POINT('Ctrl Pts',(169.785402555019,1.7293998003006,48.35));
#78656=CARTESIAN_POINT('Ctrl Pts',(169.696111816913,1.55156904459,48.35));
#78657=CARTESIAN_POINT('Ctrl Pts',(169.540041226894,1.45702594518662,48.35));
#78658=CARTESIAN_POINT('Ctrl Pts',(169.874693293124,2.11432480812073,48.5));
#78659=CARTESIAN_POINT('Ctrl Pts',(169.874693293124,2.11432480812073,48.35));
#78660=CARTESIAN_POINT('Ctrl Pts',(169.874693293124,1.9072305560112,48.5));
#78661=CARTESIAN_POINT('Ctrl Pts',(169.874693293124,1.9072305560112,48.35));
#78662=CARTESIAN_POINT('Ctrl Pts',(169.785402555019,1.7293998003006,48.5));
#78663=CARTESIAN_POINT('Ctrl Pts',(169.785402555019,1.7293998003006,48.35));
#78664=CARTESIAN_POINT('',(169.874693293124,2.11432480812073,48.5));
#78665=CARTESIAN_POINT('Ctrl Pts',(169.874693293124,2.11432480812073,48.5));
#78666=CARTESIAN_POINT('Ctrl Pts',(169.874693293124,1.9072305560112,48.5));
#78667=CARTESIAN_POINT('Ctrl Pts',(169.785402555019,1.7293998003006,48.5));
#78668=CARTESIAN_POINT('',(169.874693293124,2.11432480812073,48.35));
#78669=CARTESIAN_POINT('',(169.874693293124,2.11432480812073,48.5));
#78670=CARTESIAN_POINT('Ctrl Pts',(169.874693293124,2.11432480812073,48.35));
#78671=CARTESIAN_POINT('Ctrl Pts',(169.874693293124,1.9072305560112,48.35));
#78672=CARTESIAN_POINT('Ctrl Pts',(169.785402555019,1.7293998003006,48.35));
#78673=CARTESIAN_POINT('Ctrl Pts',(169.68485667184,2.62830847501755,48.5));
#78674=CARTESIAN_POINT('Ctrl Pts',(169.68485667184,2.62830847501755,48.35));
#78675=CARTESIAN_POINT('Ctrl Pts',(169.874693293124,2.42946797609329,48.5));
#78676=CARTESIAN_POINT('Ctrl Pts',(169.874693293124,2.42946797609329,48.35));
#78677=CARTESIAN_POINT('Ctrl Pts',(169.874693293124,2.11432480812073,48.5));
#78678=CARTESIAN_POINT('Ctrl Pts',(169.874693293124,2.11432480812073,48.35));
#78679=CARTESIAN_POINT('',(169.68485667184,2.62830847501755,48.5));
#78680=CARTESIAN_POINT('Ctrl Pts',(169.68485667184,2.62830847501755,48.5));
#78681=CARTESIAN_POINT('Ctrl Pts',(169.874693293124,2.42946797609329,48.5));
#78682=CARTESIAN_POINT('Ctrl Pts',(169.874693293124,2.11432480812073,48.5));
#78683=CARTESIAN_POINT('',(169.68485667184,2.62830847501755,48.35));
#78684=CARTESIAN_POINT('',(169.68485667184,2.62830847501755,48.5));
#78685=CARTESIAN_POINT('Ctrl Pts',(169.68485667184,2.62830847501755,48.35));
#78686=CARTESIAN_POINT('Ctrl Pts',(169.874693293124,2.42946797609329,48.35));
#78687=CARTESIAN_POINT('Ctrl Pts',(169.874693293124,2.11432480812073,48.35));
#78688=CARTESIAN_POINT('Ctrl Pts',(169.224897760898,2.82714867591858,48.5));
#78689=CARTESIAN_POINT('Ctrl Pts',(169.224897760898,2.82714867591858,48.35));
#78690=CARTESIAN_POINT('Ctrl Pts',(169.495020646602,2.82714867591858,48.5));
#78691=CARTESIAN_POINT('Ctrl Pts',(169.495020646602,2.82714867591858,48.35));
#78692=CARTESIAN_POINT('Ctrl Pts',(169.68485667184,2.62830847501755,48.5));
#78693=CARTESIAN_POINT('Ctrl Pts',(169.68485667184,2.62830847501755,48.35));
#78694=CARTESIAN_POINT('',(169.224897760898,2.82714867591858,48.5));
#78695=CARTESIAN_POINT('Ctrl Pts',(169.224897760898,2.82714867591858,48.5));
#78696=CARTESIAN_POINT('Ctrl Pts',(169.495020646602,2.82714867591858,48.5));
#78697=CARTESIAN_POINT('Ctrl Pts',(169.68485667184,2.62830847501755,48.5));
#78698=CARTESIAN_POINT('',(169.224897760898,2.82714867591858,48.35));
#78699=CARTESIAN_POINT('',(169.224897760898,2.82714867591858,48.5));
#78700=CARTESIAN_POINT('Ctrl Pts',(169.224897760898,2.82714867591858,48.35));
#78701=CARTESIAN_POINT('Ctrl Pts',(169.495020646602,2.82714867591858,48.35));
#78702=CARTESIAN_POINT('Ctrl Pts',(169.68485667184,2.62830847501755,48.35));
#78703=CARTESIAN_POINT('Ctrl Pts',(168.929263491184,2.75511601567268,48.5));
#78704=CARTESIAN_POINT('Ctrl Pts',(168.929263491184,2.75511601567268,48.35));
#78705=CARTESIAN_POINT('Ctrl Pts',(169.070327568799,2.82714867591858,48.5));
#78706=CARTESIAN_POINT('Ctrl Pts',(169.070327568799,2.82714867591858,48.35));
#78707=CARTESIAN_POINT('Ctrl Pts',(169.224897760898,2.82714867591858,48.5));
#78708=CARTESIAN_POINT('Ctrl Pts',(169.224897760898,2.82714867591858,48.35));
#78709=CARTESIAN_POINT('',(168.929263491184,2.75511601567268,48.5));
#78710=CARTESIAN_POINT('Ctrl Pts',(168.929263491184,2.75511601567268,48.5));
#78711=CARTESIAN_POINT('Ctrl Pts',(169.070327568799,2.82714867591858,48.5));
#78712=CARTESIAN_POINT('Ctrl Pts',(169.224897760898,2.82714867591858,48.5));
#78713=CARTESIAN_POINT('',(168.929263491184,2.75511601567268,48.35));
#78714=CARTESIAN_POINT('',(168.929263491184,2.75511601567268,48.5));
#78715=CARTESIAN_POINT('Ctrl Pts',(168.929263491184,2.75511601567268,48.35));
#78716=CARTESIAN_POINT('Ctrl Pts',(169.070327568799,2.82714867591858,48.35));
#78717=CARTESIAN_POINT('Ctrl Pts',(169.224897760898,2.82714867591858,48.35));
#78718=CARTESIAN_POINT('Ctrl Pts',(168.690654922277,2.53451579809189,48.5));
#78719=CARTESIAN_POINT('Ctrl Pts',(168.690654922277,2.53451579809189,48.35));
#78720=CARTESIAN_POINT('Ctrl Pts',(168.788199264556,2.68308320641518,48.5));
#78721=CARTESIAN_POINT('Ctrl Pts',(168.788199264556,2.68308320641518,48.35));
#78722=CARTESIAN_POINT('Ctrl Pts',(168.929263491184,2.75511601567268,48.5));
#78723=CARTESIAN_POINT('Ctrl Pts',(168.929263491184,2.75511601567268,48.35));
#78724=CARTESIAN_POINT('',(168.690654922277,2.53451579809189,48.5));
#78725=CARTESIAN_POINT('Ctrl Pts',(168.690654922277,2.53451579809189,48.5));
#78726=CARTESIAN_POINT('Ctrl Pts',(168.788199264556,2.68308320641518,48.5));
#78727=CARTESIAN_POINT('Ctrl Pts',(168.929263491184,2.75511601567268,48.5));
#78728=CARTESIAN_POINT('',(168.690654922277,2.53451579809189,48.35));
#78729=CARTESIAN_POINT('',(168.690654922277,2.53451579809189,48.5));
#78730=CARTESIAN_POINT('Ctrl Pts',(168.690654922277,2.53451579809189,48.35));
#78731=CARTESIAN_POINT('Ctrl Pts',(168.788199264556,2.68308320641518,48.35));
#78732=CARTESIAN_POINT('Ctrl Pts',(168.929263491184,2.75511601567268,48.35));
#78733=CARTESIAN_POINT('Ctrl Pts',(168.767189819366,3.04324695467949,48.5));
#78734=CARTESIAN_POINT('Ctrl Pts',(168.767189819366,3.04324695467949,48.35));
#78735=CARTESIAN_POINT('Ctrl Pts',(168.693656314164,2.86466577649117,48.5));
#78736=CARTESIAN_POINT('Ctrl Pts',(168.693656314164,2.86466577649117,48.35));
#78737=CARTESIAN_POINT('Ctrl Pts',(168.690654922277,2.53451579809189,48.5));
#78738=CARTESIAN_POINT('Ctrl Pts',(168.690654922277,2.53451579809189,48.35));
#78739=CARTESIAN_POINT('',(168.767189819366,3.04324695467949,48.5));
#78740=CARTESIAN_POINT('Ctrl Pts',(168.767189819366,3.04324695467949,48.5));
#78741=CARTESIAN_POINT('Ctrl Pts',(168.693656314164,2.86466577649117,48.5));
#78742=CARTESIAN_POINT('Ctrl Pts',(168.690654922277,2.53451579809189,48.5));
#78743=CARTESIAN_POINT('',(168.767189819366,3.04324695467949,48.35));
#78744=CARTESIAN_POINT('',(168.767189819366,3.04324695467949,48.5));
#78745=CARTESIAN_POINT('Ctrl Pts',(168.767189819366,3.04324695467949,48.35));
#78746=CARTESIAN_POINT('Ctrl Pts',(168.693656314164,2.86466577649117,48.35));
#78747=CARTESIAN_POINT('Ctrl Pts',(168.690654922277,2.53451579809189,48.35));
#78748=CARTESIAN_POINT('Ctrl Pts',(168.968281138688,3.31487038731575,48.5));
#78749=CARTESIAN_POINT('Ctrl Pts',(168.968281138688,3.31487038731575,48.35));
#78750=CARTESIAN_POINT('Ctrl Pts',(168.840723175555,3.22182813286781,48.5));
#78751=CARTESIAN_POINT('Ctrl Pts',(168.840723175555,3.22182813286781,48.35));
#78752=CARTESIAN_POINT('Ctrl Pts',(168.767189819366,3.04324695467949,48.5));
#78753=CARTESIAN_POINT('Ctrl Pts',(168.767189819366,3.04324695467949,48.35));
#78754=CARTESIAN_POINT('',(168.968281138688,3.31487038731575,48.5));
#78755=CARTESIAN_POINT('Ctrl Pts',(168.968281138688,3.31487038731575,48.5));
#78756=CARTESIAN_POINT('Ctrl Pts',(168.840723175555,3.22182813286781,48.5));
#78757=CARTESIAN_POINT('Ctrl Pts',(168.767189819366,3.04324695467949,48.5));
#78758=CARTESIAN_POINT('',(168.968281138688,3.31487038731575,48.35));
#78759=CARTESIAN_POINT('',(168.968281138688,3.31487038731575,48.5));
#78760=CARTESIAN_POINT('Ctrl Pts',(168.968281138688,3.31487038731575,48.35));
#78761=CARTESIAN_POINT('Ctrl Pts',(168.840723175555,3.22182813286781,48.35));
#78762=CARTESIAN_POINT('Ctrl Pts',(168.767189819366,3.04324695467949,48.35));
#78763=CARTESIAN_POINT('Ctrl Pts',(169.194884140044,3.38690319657326,48.5));
#78764=CARTESIAN_POINT('Ctrl Pts',(169.194884140044,3.38690319657326,48.35));
#78765=CARTESIAN_POINT('Ctrl Pts',(169.065825480968,3.38690319657326,48.5));
#78766=CARTESIAN_POINT('Ctrl Pts',(169.065825480968,3.38690319657326,48.35));
#78767=CARTESIAN_POINT('Ctrl Pts',(168.968281138688,3.31487038731575,48.5));
#78768=CARTESIAN_POINT('Ctrl Pts',(168.968281138688,3.31487038731575,48.35));
#78769=CARTESIAN_POINT('',(169.194884140044,3.38690319657326,48.5));
#78770=CARTESIAN_POINT('Ctrl Pts',(169.194884140044,3.38690319657326,48.5));
#78771=CARTESIAN_POINT('Ctrl Pts',(169.065825480968,3.38690319657326,48.5));
#78772=CARTESIAN_POINT('Ctrl Pts',(168.968281138688,3.31487038731575,48.5));
#78773=CARTESIAN_POINT('',(169.194884140044,3.38690319657326,48.35));
#78774=CARTESIAN_POINT('',(169.194884140044,3.38690319657326,48.5));
#78775=CARTESIAN_POINT('Ctrl Pts',(169.194884140044,3.38690319657326,48.35));
#78776=CARTESIAN_POINT('Ctrl Pts',(169.065825480968,3.38690319657326,48.35));
#78777=CARTESIAN_POINT('Ctrl Pts',(168.968281138688,3.31487038731575,48.35));
#78778=CARTESIAN_POINT('Ctrl Pts',(169.465007025748,3.27135065197945,48.5));
#78779=CARTESIAN_POINT('Ctrl Pts',(169.465007025748,3.27135065197945,48.35));
#78780=CARTESIAN_POINT('Ctrl Pts',(169.35545726493,3.38690319657326,48.5));
#78781=CARTESIAN_POINT('Ctrl Pts',(169.35545726493,3.38690319657326,48.35));
#78782=CARTESIAN_POINT('Ctrl Pts',(169.194884140044,3.38690319657326,48.5));
#78783=CARTESIAN_POINT('Ctrl Pts',(169.194884140044,3.38690319657326,48.35));
#78784=CARTESIAN_POINT('',(169.465007025748,3.27135065197945,48.5));
#78785=CARTESIAN_POINT('Ctrl Pts',(169.465007025748,3.27135065197945,48.5));
#78786=CARTESIAN_POINT('Ctrl Pts',(169.35545726493,3.38690319657326,48.5));
#78787=CARTESIAN_POINT('Ctrl Pts',(169.194884140044,3.38690319657326,48.5));
#78788=CARTESIAN_POINT('',(169.465007025748,3.27135065197945,48.35));
#78789=CARTESIAN_POINT('',(169.465007025748,3.27135065197945,48.5));
#78790=CARTESIAN_POINT('Ctrl Pts',(169.465007025748,3.27135065197945,48.35));
#78791=CARTESIAN_POINT('Ctrl Pts',(169.35545726493,3.38690319657326,48.35));
#78792=CARTESIAN_POINT('Ctrl Pts',(169.194884140044,3.38690319657326,48.35));
#78793=CARTESIAN_POINT('Ctrl Pts',(169.567053455859,3.04024556279182,48.5));
#78794=CARTESIAN_POINT('Ctrl Pts',(169.567053455859,3.04024556279182,48.35));
#78795=CARTESIAN_POINT('Ctrl Pts',(169.531037051231,3.19931784272194,48.5));
#78796=CARTESIAN_POINT('Ctrl Pts',(169.531037051231,3.19931784272194,48.35));
#78797=CARTESIAN_POINT('Ctrl Pts',(169.465007025748,3.27135065197945,48.5));
#78798=CARTESIAN_POINT('Ctrl Pts',(169.465007025748,3.27135065197945,48.35));
#78799=CARTESIAN_POINT('',(169.567053455859,3.04024556279182,48.5));
#78800=CARTESIAN_POINT('Ctrl Pts',(169.567053455859,3.04024556279182,48.5));
#78801=CARTESIAN_POINT('Ctrl Pts',(169.531037051231,3.19931784272194,48.5));
#78802=CARTESIAN_POINT('Ctrl Pts',(169.465007025748,3.27135065197945,48.5));
#78803=CARTESIAN_POINT('',(169.567053455859,3.04024556279182,48.35));
#78804=CARTESIAN_POINT('',(169.567053455859,3.04024556279182,48.5));
#78805=CARTESIAN_POINT('Ctrl Pts',(169.567053455859,3.04024556279182,48.35));
#78806=CARTESIAN_POINT('Ctrl Pts',(169.531037051231,3.19931784272194,48.35));
#78807=CARTESIAN_POINT('Ctrl Pts',(169.465007025748,3.27135065197945,48.35));
#78808=CARTESIAN_POINT('Origin',(169.835675496608,3.06125515699387,48.5));
#78809=CARTESIAN_POINT('',(169.835675496608,3.06125515699387,48.5));
#78810=CARTESIAN_POINT('',(85.6260995320938,-3.52498405855974,48.5));
#78811=CARTESIAN_POINT('',(169.835675496608,3.06125515699387,48.35));
#78812=CARTESIAN_POINT('',(169.835675496608,3.06125515699387,48.5));
#78813=CARTESIAN_POINT('',(169.835675496608,3.06125515699387,48.35));
#78814=CARTESIAN_POINT('Ctrl Pts',(169.636834997684,3.46343794465065,48.5));
#78815=CARTESIAN_POINT('Ctrl Pts',(169.636834997684,3.46343794465065,48.35));
#78816=CARTESIAN_POINT('Ctrl Pts',(169.802660483867,3.31787177920341,48.5));
#78817=CARTESIAN_POINT('Ctrl Pts',(169.802660483867,3.31787177920341,48.35));
#78818=CARTESIAN_POINT('Ctrl Pts',(169.835675496608,3.06125515699387,48.5));
#78819=CARTESIAN_POINT('Ctrl Pts',(169.835675496608,3.06125515699387,48.35));
#78820=CARTESIAN_POINT('Ctrl Pts',(169.636834997684,3.46343794465065,48.5));
#78821=CARTESIAN_POINT('Ctrl Pts',(169.802660483867,3.31787177920341,48.5));
#78822=CARTESIAN_POINT('Ctrl Pts',(169.835675496608,3.06125515699387,48.5));
#78823=CARTESIAN_POINT('Ctrl Pts',(169.636834997684,3.46343794465065,48.35));
#78824=CARTESIAN_POINT('Ctrl Pts',(169.802660483867,3.31787177920341,48.35));
#78825=CARTESIAN_POINT('Ctrl Pts',(169.835675496608,3.06125515699387,48.35));
#78826=CARTESIAN_POINT('Origin',(169.999999914318,2.48574362695217,48.35));
#78827=CARTESIAN_POINT('Origin',(0.,8.,48.5));
#78828=CARTESIAN_POINT('Origin',(0.,8.,48.5));
#78829=CARTESIAN_POINT('Ctrl Pts',(160.85163737461,3.38540250062943,48.5));
#78830=CARTESIAN_POINT('Ctrl Pts',(160.85163737461,3.38540250062943,48.35));
#78831=CARTESIAN_POINT('Ctrl Pts',(160.665552567691,3.38540250062943,48.5));
#78832=CARTESIAN_POINT('Ctrl Pts',(160.665552567691,3.38540250062943,48.35));
#78833=CARTESIAN_POINT('Ctrl Pts',(160.55450225994,3.22783091664314,48.5));
#78834=CARTESIAN_POINT('Ctrl Pts',(160.55450225994,3.22783091664314,48.35));
#78835=CARTESIAN_POINT('',(160.85163737461,3.38540250062943,48.5));
#78836=CARTESIAN_POINT('',(160.55450225994,3.22783091664314,48.5));
#78837=CARTESIAN_POINT('Ctrl Pts',(160.85163737461,3.38540250062943,48.5));
#78838=CARTESIAN_POINT('Ctrl Pts',(160.665552567691,3.38540250062943,48.5));
#78839=CARTESIAN_POINT('Ctrl Pts',(160.55450225994,3.22783091664314,48.5));
#78840=CARTESIAN_POINT('',(160.85163737461,3.38540250062943,48.35));
#78841=CARTESIAN_POINT('',(160.85163737461,3.38540250062943,48.5));
#78842=CARTESIAN_POINT('',(160.55450225994,3.22783091664314,48.35));
#78843=CARTESIAN_POINT('Ctrl Pts',(160.85163737461,3.38540250062943,48.35));
#78844=CARTESIAN_POINT('Ctrl Pts',(160.665552567691,3.38540250062943,48.35));
#78845=CARTESIAN_POINT('Ctrl Pts',(160.55450225994,3.22783091664314,48.35));
#78846=CARTESIAN_POINT('',(160.55450225994,3.22783091664314,48.5));
#78847=CARTESIAN_POINT('Ctrl Pts',(161.167530667037,3.2068213224411,48.5));
#78848=CARTESIAN_POINT('Ctrl Pts',(161.167530667037,3.2068213224411,48.35));
#78849=CARTESIAN_POINT('Ctrl Pts',(161.04072297737,3.38540250062943,48.5));
#78850=CARTESIAN_POINT('Ctrl Pts',(161.04072297737,3.38540250062943,48.35));
#78851=CARTESIAN_POINT('Ctrl Pts',(160.85163737461,3.38540250062943,48.5));
#78852=CARTESIAN_POINT('Ctrl Pts',(160.85163737461,3.38540250062943,48.35));
#78853=CARTESIAN_POINT('',(161.167530667037,3.2068213224411,48.5));
#78854=CARTESIAN_POINT('Ctrl Pts',(161.167530667037,3.2068213224411,48.5));
#78855=CARTESIAN_POINT('Ctrl Pts',(161.04072297737,3.38540250062943,48.5));
#78856=CARTESIAN_POINT('Ctrl Pts',(160.85163737461,3.38540250062943,48.5));
#78857=CARTESIAN_POINT('',(161.167530667037,3.2068213224411,48.35));
#78858=CARTESIAN_POINT('',(161.167530667037,3.2068213224411,48.5));
#78859=CARTESIAN_POINT('Ctrl Pts',(161.167530667037,3.2068213224411,48.35));
#78860=CARTESIAN_POINT('Ctrl Pts',(161.04072297737,3.38540250062943,48.35));
#78861=CARTESIAN_POINT('Ctrl Pts',(160.85163737461,3.38540250062943,48.35));
#78862=CARTESIAN_POINT('Ctrl Pts',(161.294338356704,2.48499327898026,48.5));
#78863=CARTESIAN_POINT('Ctrl Pts',(161.294338356704,2.48499327898026,48.35));
#78864=CARTESIAN_POINT('Ctrl Pts',(161.294338356704,3.02824014425278,48.5));
#78865=CARTESIAN_POINT('Ctrl Pts',(161.294338356704,3.02824014425278,48.35));
#78866=CARTESIAN_POINT('Ctrl Pts',(161.167530667037,3.2068213224411,48.5));
#78867=CARTESIAN_POINT('Ctrl Pts',(161.167530667037,3.2068213224411,48.35));
#78868=CARTESIAN_POINT('',(161.294338356704,2.48499327898026,48.5));
#78869=CARTESIAN_POINT('Ctrl Pts',(161.294338356704,2.48499327898026,48.5));
#78870=CARTESIAN_POINT('Ctrl Pts',(161.294338356704,3.02824014425278,48.5));
#78871=CARTESIAN_POINT('Ctrl Pts',(161.167530667037,3.2068213224411,48.5));
#78872=CARTESIAN_POINT('',(161.294338356704,2.48499327898026,48.35));
#78873=CARTESIAN_POINT('',(161.294338356704,2.48499327898026,48.5));
#78874=CARTESIAN_POINT('Ctrl Pts',(161.294338356704,2.48499327898026,48.35));
#78875=CARTESIAN_POINT('Ctrl Pts',(161.294338356704,3.02824014425278,48.35));
#78876=CARTESIAN_POINT('Ctrl Pts',(161.167530667037,3.2068213224411,48.35));
#78877=CARTESIAN_POINT('Ctrl Pts',(161.167530667037,1.76466578245163,48.5));
#78878=CARTESIAN_POINT('Ctrl Pts',(161.167530667037,1.76466578245163,48.35));
#78879=CARTESIAN_POINT('Ctrl Pts',(161.294338356704,1.9447478055954,48.5));
#78880=CARTESIAN_POINT('Ctrl Pts',(161.294338356704,1.9447478055954,48.35));
#78881=CARTESIAN_POINT('Ctrl Pts',(161.294338356704,2.48499327898026,48.5));
#78882=CARTESIAN_POINT('Ctrl Pts',(161.294338356704,2.48499327898026,48.35));
#78883=CARTESIAN_POINT('',(161.167530667037,1.76466578245163,48.5));
#78884=CARTESIAN_POINT('Ctrl Pts',(161.167530667037,1.76466578245163,48.5));
#78885=CARTESIAN_POINT('Ctrl Pts',(161.294338356704,1.9447478055954,48.5));
#78886=CARTESIAN_POINT('Ctrl Pts',(161.294338356704,2.48499327898026,48.5));
#78887=CARTESIAN_POINT('',(161.167530667037,1.76466578245163,48.35));
#78888=CARTESIAN_POINT('',(161.167530667037,1.76466578245163,48.5));
#78889=CARTESIAN_POINT('Ctrl Pts',(161.167530667037,1.76466578245163,48.35));
#78890=CARTESIAN_POINT('Ctrl Pts',(161.294338356704,1.9447478055954,48.35));
#78891=CARTESIAN_POINT('Ctrl Pts',(161.294338356704,2.48499327898026,48.35));
#78892=CARTESIAN_POINT('Ctrl Pts',(160.854638468474,1.58458405733109,48.5));
#78893=CARTESIAN_POINT('Ctrl Pts',(160.854638468474,1.58458405733109,48.35));
#78894=CARTESIAN_POINT('Ctrl Pts',(161.04072297737,1.58458405733109,48.5));
#78895=CARTESIAN_POINT('Ctrl Pts',(161.04072297737,1.58458405733109,48.35));
#78896=CARTESIAN_POINT('Ctrl Pts',(161.167530667037,1.76466578245163,48.5));
#78897=CARTESIAN_POINT('Ctrl Pts',(161.167530667037,1.76466578245163,48.35));
#78898=CARTESIAN_POINT('',(160.854638468474,1.58458405733109,48.5));
#78899=CARTESIAN_POINT('Ctrl Pts',(160.854638468474,1.58458405733109,48.5));
#78900=CARTESIAN_POINT('Ctrl Pts',(161.04072297737,1.58458405733109,48.5));
#78901=CARTESIAN_POINT('Ctrl Pts',(161.167530667037,1.76466578245163,48.5));
#78902=CARTESIAN_POINT('',(160.854638468474,1.58458405733109,48.35));
#78903=CARTESIAN_POINT('',(160.854638468474,1.58458405733109,48.5));
#78904=CARTESIAN_POINT('Ctrl Pts',(160.854638468474,1.58458405733109,48.35));
#78905=CARTESIAN_POINT('Ctrl Pts',(161.04072297737,1.58458405733109,48.35));
#78906=CARTESIAN_POINT('Ctrl Pts',(161.167530667037,1.76466578245163,48.35));
#78907=CARTESIAN_POINT('Ctrl Pts',(160.541746269912,1.76391565799713,48.5));
#78908=CARTESIAN_POINT('Ctrl Pts',(160.541746269912,1.76391565799713,48.35));
#78909=CARTESIAN_POINT('Ctrl Pts',(160.668553959578,1.58458405733109,48.5));
#78910=CARTESIAN_POINT('Ctrl Pts',(160.668553959578,1.58458405733109,48.35));
#78911=CARTESIAN_POINT('Ctrl Pts',(160.854638468474,1.58458405733109,48.5));
#78912=CARTESIAN_POINT('Ctrl Pts',(160.854638468474,1.58458405733109,48.35));
#78913=CARTESIAN_POINT('',(160.541746269912,1.76391565799713,48.5));
#78914=CARTESIAN_POINT('Ctrl Pts',(160.541746269912,1.76391565799713,48.5));
#78915=CARTESIAN_POINT('Ctrl Pts',(160.668553959578,1.58458405733109,48.5));
#78916=CARTESIAN_POINT('Ctrl Pts',(160.854638468474,1.58458405733109,48.5));
#78917=CARTESIAN_POINT('',(160.541746269912,1.76391565799713,48.35));
#78918=CARTESIAN_POINT('',(160.541746269912,1.76391565799713,48.5));
#78919=CARTESIAN_POINT('Ctrl Pts',(160.541746269912,1.76391565799713,48.35));
#78920=CARTESIAN_POINT('Ctrl Pts',(160.668553959578,1.58458405733109,48.35));
#78921=CARTESIAN_POINT('Ctrl Pts',(160.854638468474,1.58458405733109,48.35));
#78922=CARTESIAN_POINT('Ctrl Pts',(160.414938580245,2.48499327898026,48.5));
#78923=CARTESIAN_POINT('Ctrl Pts',(160.414938580245,2.48499327898026,48.35));
#78924=CARTESIAN_POINT('Ctrl Pts',(160.414938580245,1.94324696063995,48.5));
#78925=CARTESIAN_POINT('Ctrl Pts',(160.414938580245,1.94324696063995,48.35));
#78926=CARTESIAN_POINT('Ctrl Pts',(160.541746269912,1.76391565799713,48.5));
#78927=CARTESIAN_POINT('Ctrl Pts',(160.541746269912,1.76391565799713,48.35));
#78928=CARTESIAN_POINT('',(160.414938580245,2.48499327898026,48.5));
#78929=CARTESIAN_POINT('Ctrl Pts',(160.414938580245,2.48499327898026,48.5));
#78930=CARTESIAN_POINT('Ctrl Pts',(160.414938580245,1.94324696063995,48.5));
#78931=CARTESIAN_POINT('Ctrl Pts',(160.541746269912,1.76391565799713,48.5));
#78932=CARTESIAN_POINT('',(160.414938580245,2.48499327898026,48.35));
#78933=CARTESIAN_POINT('',(160.414938580245,2.48499327898026,48.5));
#78934=CARTESIAN_POINT('Ctrl Pts',(160.414938580245,2.48499327898026,48.35));
#78935=CARTESIAN_POINT('Ctrl Pts',(160.414938580245,1.94324696063995,48.35));
#78936=CARTESIAN_POINT('Ctrl Pts',(160.541746269912,1.76391565799713,48.35));
#78937=CARTESIAN_POINT('Ctrl Pts',(160.55450225994,3.22783091664314,48.5));
#78938=CARTESIAN_POINT('Ctrl Pts',(160.55450225994,3.22783091664314,48.35));
#78939=CARTESIAN_POINT('Ctrl Pts',(160.414938580245,3.02673944830894,48.5));
#78940=CARTESIAN_POINT('Ctrl Pts',(160.414938580245,3.02673944830894,48.35));
#78941=CARTESIAN_POINT('Ctrl Pts',(160.414938580245,2.48499327898026,48.5));
#78942=CARTESIAN_POINT('Ctrl Pts',(160.414938580245,2.48499327898026,48.35));
#78943=CARTESIAN_POINT('Ctrl Pts',(160.55450225994,3.22783091664314,48.5));
#78944=CARTESIAN_POINT('Ctrl Pts',(160.414938580245,3.02673944830894,48.5));
#78945=CARTESIAN_POINT('Ctrl Pts',(160.414938580245,2.48499327898026,48.5));
#78946=CARTESIAN_POINT('Ctrl Pts',(160.55450225994,3.22783091664314,48.35));
#78947=CARTESIAN_POINT('Ctrl Pts',(160.414938580245,3.02673944830894,48.35));
#78948=CARTESIAN_POINT('Ctrl Pts',(160.414938580245,2.48499327898026,48.35));
#78949=CARTESIAN_POINT('Ctrl Pts',(160.854638468474,1.36248314380646,48.5));
#78950=CARTESIAN_POINT('Ctrl Pts',(160.854638468474,1.36248314380646,48.35));
#78951=CARTESIAN_POINT('Ctrl Pts',(160.536493908614,1.36248314380646,48.5));
#78952=CARTESIAN_POINT('Ctrl Pts',(160.536493908614,1.36248314380646,48.35));
#78953=CARTESIAN_POINT('Ctrl Pts',(160.354911338538,1.59058684110642,48.5));
#78954=CARTESIAN_POINT('Ctrl Pts',(160.354911338538,1.59058684110642,48.35));
#78955=CARTESIAN_POINT('',(160.854638468474,1.36248314380646,48.5));
#78956=CARTESIAN_POINT('',(160.354911338538,1.59058684110642,48.5));
#78957=CARTESIAN_POINT('Ctrl Pts',(160.854638468474,1.36248314380646,48.5));
#78958=CARTESIAN_POINT('Ctrl Pts',(160.536493908614,1.36248314380646,48.5));
#78959=CARTESIAN_POINT('Ctrl Pts',(160.354911338538,1.59058684110642,48.5));
#78960=CARTESIAN_POINT('',(160.854638468474,1.36248314380646,48.35));
#78961=CARTESIAN_POINT('',(160.854638468474,1.36248314380646,48.5));
#78962=CARTESIAN_POINT('',(160.354911338538,1.59058684110642,48.35));
#78963=CARTESIAN_POINT('Ctrl Pts',(160.854638468474,1.36248314380646,48.35));
#78964=CARTESIAN_POINT('Ctrl Pts',(160.536493908614,1.36248314380646,48.35));
#78965=CARTESIAN_POINT('Ctrl Pts',(160.354911338538,1.59058684110642,48.35));
#78966=CARTESIAN_POINT('',(160.354911338538,1.59058684110642,48.5));
#78967=CARTESIAN_POINT('Ctrl Pts',(161.254570137709,1.49229192733765,48.5));
#78968=CARTESIAN_POINT('Ctrl Pts',(161.254570137709,1.49229192733765,48.35));
#78969=CARTESIAN_POINT('Ctrl Pts',(161.096248280257,1.36248314380646,48.5));
#78970=CARTESIAN_POINT('Ctrl Pts',(161.096248280257,1.36248314380646,48.35));
#78971=CARTESIAN_POINT('Ctrl Pts',(160.854638468474,1.36248314380646,48.5));
#78972=CARTESIAN_POINT('Ctrl Pts',(160.854638468474,1.36248314380646,48.35));
#78973=CARTESIAN_POINT('',(161.254570137709,1.49229192733765,48.5));
#78974=CARTESIAN_POINT('Ctrl Pts',(161.254570137709,1.49229192733765,48.5));
#78975=CARTESIAN_POINT('Ctrl Pts',(161.096248280257,1.36248314380646,48.5));
#78976=CARTESIAN_POINT('Ctrl Pts',(160.854638468474,1.36248314380646,48.5));
#78977=CARTESIAN_POINT('',(161.254570137709,1.49229192733765,48.35));
#78978=CARTESIAN_POINT('',(161.254570137709,1.49229192733765,48.5));
#78979=CARTESIAN_POINT('Ctrl Pts',(161.254570137709,1.49229192733765,48.35));
#78980=CARTESIAN_POINT('Ctrl Pts',(161.096248280257,1.36248314380646,48.35));
#78981=CARTESIAN_POINT('Ctrl Pts',(160.854638468474,1.36248314380646,48.35));
#78982=CARTESIAN_POINT('Ctrl Pts',(161.49242843315,1.85995900630951,48.5));
#78983=CARTESIAN_POINT('Ctrl Pts',(161.49242843315,1.85995900630951,48.35));
#78984=CARTESIAN_POINT('Ctrl Pts',(161.412891995162,1.62210100889206,48.5));
#78985=CARTESIAN_POINT('Ctrl Pts',(161.412891995162,1.62210100889206,48.35));
#78986=CARTESIAN_POINT('Ctrl Pts',(161.254570137709,1.49229192733765,48.5));
#78987=CARTESIAN_POINT('Ctrl Pts',(161.254570137709,1.49229192733765,48.35));
#78988=CARTESIAN_POINT('',(161.49242843315,1.85995900630951,48.5));
#78989=CARTESIAN_POINT('Ctrl Pts',(161.49242843315,1.85995900630951,48.5));
#78990=CARTESIAN_POINT('Ctrl Pts',(161.412891995162,1.62210100889206,48.5));
#78991=CARTESIAN_POINT('Ctrl Pts',(161.254570137709,1.49229192733765,48.5));
#78992=CARTESIAN_POINT('',(161.49242843315,1.85995900630951,48.35));
#78993=CARTESIAN_POINT('',(161.49242843315,1.85995900630951,48.5));
#78994=CARTESIAN_POINT('Ctrl Pts',(161.49242843315,1.85995900630951,48.35));
#78995=CARTESIAN_POINT('Ctrl Pts',(161.412891995162,1.62210100889206,48.35));
#78996=CARTESIAN_POINT('Ctrl Pts',(161.254570137709,1.49229192733765,48.35));
#78997=CARTESIAN_POINT('Ctrl Pts',(161.571964275092,2.48499327898026,48.5));
#78998=CARTESIAN_POINT('Ctrl Pts',(161.571964275092,2.48499327898026,48.35));
#78999=CARTESIAN_POINT('Ctrl Pts',(161.571964275092,2.09781730175018,48.5));
#79000=CARTESIAN_POINT('Ctrl Pts',(161.571964275092,2.09781730175018,48.35));
#79001=CARTESIAN_POINT('Ctrl Pts',(161.49242843315,1.85995900630951,48.5));
#79002=CARTESIAN_POINT('Ctrl Pts',(161.49242843315,1.85995900630951,48.35));
#79003=CARTESIAN_POINT('',(161.571964275092,2.48499327898026,48.5));
#79004=CARTESIAN_POINT('Ctrl Pts',(161.571964275092,2.48499327898026,48.5));
#79005=CARTESIAN_POINT('Ctrl Pts',(161.571964275092,2.09781730175018,48.5));
#79006=CARTESIAN_POINT('Ctrl Pts',(161.49242843315,1.85995900630951,48.5));
#79007=CARTESIAN_POINT('',(161.571964275092,2.48499327898026,48.35));
#79008=CARTESIAN_POINT('',(161.571964275092,2.48499327898026,48.5));
#79009=CARTESIAN_POINT('Ctrl Pts',(161.571964275092,2.48499327898026,48.35));
#79010=CARTESIAN_POINT('Ctrl Pts',(161.571964275092,2.09781730175018,48.35));
#79011=CARTESIAN_POINT('Ctrl Pts',(161.49242843315,1.85995900630951,48.35));
#79012=CARTESIAN_POINT('Ctrl Pts',(161.52244175598,3.00497958064079,48.5));
#79013=CARTESIAN_POINT('Ctrl Pts',(161.52244175598,3.00497958064079,48.35));
#79014=CARTESIAN_POINT('Ctrl Pts',(161.571964275092,2.81214186549187,48.5));
#79015=CARTESIAN_POINT('Ctrl Pts',(161.571964275092,2.81214186549187,48.35));
#79016=CARTESIAN_POINT('Ctrl Pts',(161.571964275092,2.48499327898026,48.5));
#79017=CARTESIAN_POINT('Ctrl Pts',(161.571964275092,2.48499327898026,48.35));
#79018=CARTESIAN_POINT('',(161.52244175598,3.00497958064079,48.5));
#79019=CARTESIAN_POINT('Ctrl Pts',(161.52244175598,3.00497958064079,48.5));
#79020=CARTESIAN_POINT('Ctrl Pts',(161.571964275092,2.81214186549187,48.5));
#79021=CARTESIAN_POINT('Ctrl Pts',(161.571964275092,2.48499327898026,48.5));
#79022=CARTESIAN_POINT('',(161.52244175598,3.00497958064079,48.35));
#79023=CARTESIAN_POINT('',(161.52244175598,3.00497958064079,48.5));
#79024=CARTESIAN_POINT('Ctrl Pts',(161.52244175598,3.00497958064079,48.35));
#79025=CARTESIAN_POINT('Ctrl Pts',(161.571964275092,2.81214186549187,48.35));
#79026=CARTESIAN_POINT('Ctrl Pts',(161.571964275092,2.48499327898026,48.35));
#79027=CARTESIAN_POINT('Ctrl Pts',(161.385879766196,3.33212831616402,48.5));
#79028=CARTESIAN_POINT('Ctrl Pts',(161.385879766196,3.33212831616402,48.35));
#79029=CARTESIAN_POINT('Ctrl Pts',(161.472919236869,3.19781729578972,48.5));
#79030=CARTESIAN_POINT('Ctrl Pts',(161.472919236869,3.19781729578972,48.35));
#79031=CARTESIAN_POINT('Ctrl Pts',(161.52244175598,3.00497958064079,48.5));
#79032=CARTESIAN_POINT('Ctrl Pts',(161.52244175598,3.00497958064079,48.35));
#79033=CARTESIAN_POINT('',(161.385879766196,3.33212831616402,48.5));
#79034=CARTESIAN_POINT('Ctrl Pts',(161.385879766196,3.33212831616402,48.5));
#79035=CARTESIAN_POINT('Ctrl Pts',(161.472919236869,3.19781729578972,48.5));
#79036=CARTESIAN_POINT('Ctrl Pts',(161.52244175598,3.00497958064079,48.5));
#79037=CARTESIAN_POINT('',(161.385879766196,3.33212831616402,48.35));
#79038=CARTESIAN_POINT('',(161.385879766196,3.33212831616402,48.5));
#79039=CARTESIAN_POINT('Ctrl Pts',(161.385879766196,3.33212831616402,48.35));
#79040=CARTESIAN_POINT('Ctrl Pts',(161.472919236869,3.19781729578972,48.35));
#79041=CARTESIAN_POINT('Ctrl Pts',(161.52244175598,3.00497958064079,48.35));
#79042=CARTESIAN_POINT('Ctrl Pts',(161.16527999565,3.5377217233181,48.5));
#79043=CARTESIAN_POINT('Ctrl Pts',(161.16527999565,3.5377217233181,48.35));
#79044=CARTESIAN_POINT('Ctrl Pts',(161.298840295523,3.46643933653831,48.5));
#79045=CARTESIAN_POINT('Ctrl Pts',(161.298840295523,3.46643933653831,48.35));
#79046=CARTESIAN_POINT('Ctrl Pts',(161.385879766196,3.33212831616402,48.5));
#79047=CARTESIAN_POINT('Ctrl Pts',(161.385879766196,3.33212831616402,48.35));
#79048=CARTESIAN_POINT('',(161.16527999565,3.5377217233181,48.5));
#79049=CARTESIAN_POINT('Ctrl Pts',(161.16527999565,3.5377217233181,48.5));
#79050=CARTESIAN_POINT('Ctrl Pts',(161.298840295523,3.46643933653831,48.5));
#79051=CARTESIAN_POINT('Ctrl Pts',(161.385879766196,3.33212831616402,48.5));
#79052=CARTESIAN_POINT('',(161.16527999565,3.5377217233181,48.35));
#79053=CARTESIAN_POINT('',(161.16527999565,3.5377217233181,48.5));
#79054=CARTESIAN_POINT('Ctrl Pts',(161.16527999565,3.5377217233181,48.35));
#79055=CARTESIAN_POINT('Ctrl Pts',(161.298840295523,3.46643933653831,48.35));
#79056=CARTESIAN_POINT('Ctrl Pts',(161.385879766196,3.33212831616402,48.35));
#79057=CARTESIAN_POINT('Ctrl Pts',(160.854638468474,3.60900411009789,48.5));
#79058=CARTESIAN_POINT('Ctrl Pts',(160.854638468474,3.60900411009789,48.35));
#79059=CARTESIAN_POINT('Ctrl Pts',(161.03171909973,3.60900411009789,48.5));
#79060=CARTESIAN_POINT('Ctrl Pts',(161.03171909973,3.60900411009789,48.35));
#79061=CARTESIAN_POINT('Ctrl Pts',(161.16527999565,3.5377217233181,48.5));
#79062=CARTESIAN_POINT('Ctrl Pts',(161.16527999565,3.5377217233181,48.35));
#79063=CARTESIAN_POINT('',(160.854638468474,3.60900411009789,48.5));
#79064=CARTESIAN_POINT('Ctrl Pts',(160.854638468474,3.60900411009789,48.5));
#79065=CARTESIAN_POINT('Ctrl Pts',(161.03171909973,3.60900411009789,48.5));
#79066=CARTESIAN_POINT('Ctrl Pts',(161.16527999565,3.5377217233181,48.5));
#79067=CARTESIAN_POINT('',(160.854638468474,3.60900411009789,48.35));
#79068=CARTESIAN_POINT('',(160.854638468474,3.60900411009789,48.5));
#79069=CARTESIAN_POINT('Ctrl Pts',(160.854638468474,3.60900411009789,48.35));
#79070=CARTESIAN_POINT('Ctrl Pts',(161.03171909973,3.60900411009789,48.35));
#79071=CARTESIAN_POINT('Ctrl Pts',(161.16527999565,3.5377217233181,48.35));
#79072=CARTESIAN_POINT('Ctrl Pts',(160.456207644194,3.47994545102119,48.5));
#79073=CARTESIAN_POINT('Ctrl Pts',(160.456207644194,3.47994545102119,48.35));
#79074=CARTESIAN_POINT('Ctrl Pts',(160.614529501647,3.60900411009789,48.5));
#79075=CARTESIAN_POINT('Ctrl Pts',(160.614529501647,3.60900411009789,48.35));
#79076=CARTESIAN_POINT('Ctrl Pts',(160.854638468474,3.60900411009789,48.5));
#79077=CARTESIAN_POINT('Ctrl Pts',(160.854638468474,3.60900411009789,48.35));
#79078=CARTESIAN_POINT('',(160.456207644194,3.47994545102119,48.5));
#79079=CARTESIAN_POINT('Ctrl Pts',(160.456207644194,3.47994545102119,48.5));
#79080=CARTESIAN_POINT('Ctrl Pts',(160.614529501647,3.60900411009789,48.5));
#79081=CARTESIAN_POINT('Ctrl Pts',(160.854638468474,3.60900411009789,48.5));
#79082=CARTESIAN_POINT('',(160.456207644194,3.47994545102119,48.35));
#79083=CARTESIAN_POINT('',(160.456207644194,3.47994545102119,48.5));
#79084=CARTESIAN_POINT('Ctrl Pts',(160.456207644194,3.47994545102119,48.35));
#79085=CARTESIAN_POINT('Ctrl Pts',(160.614529501647,3.60900411009789,48.35));
#79086=CARTESIAN_POINT('Ctrl Pts',(160.854638468474,3.60900411009789,48.35));
#79087=CARTESIAN_POINT('Ctrl Pts',(160.217598926276,3.11302864551544,48.5));
#79088=CARTESIAN_POINT('Ctrl Pts',(160.217598926276,3.11302864551544,48.35));
#79089=CARTESIAN_POINT('Ctrl Pts',(160.297885488719,3.3508867919445,48.5));
#79090=CARTESIAN_POINT('Ctrl Pts',(160.297885488719,3.3508867919445,48.35));
#79091=CARTESIAN_POINT('Ctrl Pts',(160.456207644194,3.47994545102119,48.5));
#79092=CARTESIAN_POINT('Ctrl Pts',(160.456207644194,3.47994545102119,48.35));
#79093=CARTESIAN_POINT('',(160.217598926276,3.11302864551544,48.5));
#79094=CARTESIAN_POINT('Ctrl Pts',(160.217598926276,3.11302864551544,48.5));
#79095=CARTESIAN_POINT('Ctrl Pts',(160.297885488719,3.3508867919445,48.5));
#79096=CARTESIAN_POINT('Ctrl Pts',(160.456207644194,3.47994545102119,48.5));
#79097=CARTESIAN_POINT('',(160.217598926276,3.11302864551544,48.35));
#79098=CARTESIAN_POINT('',(160.217598926276,3.11302864551544,48.5));
#79099=CARTESIAN_POINT('Ctrl Pts',(160.217598926276,3.11302864551544,48.35));
#79100=CARTESIAN_POINT('Ctrl Pts',(160.297885488719,3.3508867919445,48.35));
#79101=CARTESIAN_POINT('Ctrl Pts',(160.456207644194,3.47994545102119,48.35));
#79102=CARTESIAN_POINT('Ctrl Pts',(160.137312661856,2.48499327898026,48.5));
#79103=CARTESIAN_POINT('Ctrl Pts',(160.137312661856,2.48499327898026,48.35));
#79104=CARTESIAN_POINT('Ctrl Pts',(160.137312661856,2.87517049908638,48.5));
#79105=CARTESIAN_POINT('Ctrl Pts',(160.137312661856,2.87517049908638,48.35));
#79106=CARTESIAN_POINT('Ctrl Pts',(160.217598926276,3.11302864551544,48.5));
#79107=CARTESIAN_POINT('Ctrl Pts',(160.217598926276,3.11302864551544,48.35));
#79108=CARTESIAN_POINT('',(160.137312661856,2.48499327898026,48.5));
#79109=CARTESIAN_POINT('Ctrl Pts',(160.137312661856,2.48499327898026,48.5));
#79110=CARTESIAN_POINT('Ctrl Pts',(160.137312661856,2.87517049908638,48.5));
#79111=CARTESIAN_POINT('Ctrl Pts',(160.217598926276,3.11302864551544,48.5));
#79112=CARTESIAN_POINT('',(160.137312661856,2.48499327898026,48.35));
#79113=CARTESIAN_POINT('',(160.137312661856,2.48499327898026,48.5));
#79114=CARTESIAN_POINT('Ctrl Pts',(160.137312661856,2.48499327898026,48.35));
#79115=CARTESIAN_POINT('Ctrl Pts',(160.137312661856,2.87517049908638,48.35));
#79116=CARTESIAN_POINT('Ctrl Pts',(160.217598926276,3.11302864551544,48.35));
#79117=CARTESIAN_POINT('Ctrl Pts',(160.354911338538,1.59058684110642,48.5));
#79118=CARTESIAN_POINT('Ctrl Pts',(160.354911338538,1.59058684110642,48.35));
#79119=CARTESIAN_POINT('Ctrl Pts',(160.137312661856,1.86521166563034,48.5));
#79120=CARTESIAN_POINT('Ctrl Pts',(160.137312661856,1.86521166563034,48.35));
#79121=CARTESIAN_POINT('Ctrl Pts',(160.137312661856,2.48499327898026,48.5));
#79122=CARTESIAN_POINT('Ctrl Pts',(160.137312661856,2.48499327898026,48.35));
#79123=CARTESIAN_POINT('Ctrl Pts',(160.354911338538,1.59058684110642,48.5));
#79124=CARTESIAN_POINT('Ctrl Pts',(160.137312661856,1.86521166563034,48.5));
#79125=CARTESIAN_POINT('Ctrl Pts',(160.137312661856,2.48499327898026,48.5));
#79126=CARTESIAN_POINT('Ctrl Pts',(160.354911338538,1.59058684110642,48.35));
#79127=CARTESIAN_POINT('Ctrl Pts',(160.137312661856,1.86521166563034,48.35));
#79128=CARTESIAN_POINT('Ctrl Pts',(160.137312661856,2.48499327898026,48.35));
#79129=CARTESIAN_POINT('Origin',(159.999999951571,2.48574362695217,48.35));
#79130=CARTESIAN_POINT('Ctrl Pts',(159.134857010096,1.36248314380646,48.5));
#79131=CARTESIAN_POINT('Ctrl Pts',(159.134857010096,1.36248314380646,48.35));
#79132=CARTESIAN_POINT('Ctrl Pts',(158.834720503539,1.36248314380646,48.5));
#79133=CARTESIAN_POINT('Ctrl Pts',(158.834720503539,1.36248314380646,48.35));
#79134=CARTESIAN_POINT('Ctrl Pts',(158.644884180278,1.53055930137634,48.5));
#79135=CARTESIAN_POINT('Ctrl Pts',(158.644884180278,1.53055930137634,48.35));
#79136=CARTESIAN_POINT('',(159.134857010096,1.36248314380646,48.5));
#79137=CARTESIAN_POINT('',(158.644884180278,1.53055930137634,48.5));
#79138=CARTESIAN_POINT('Ctrl Pts',(159.134857010096,1.36248314380646,48.5));
#79139=CARTESIAN_POINT('Ctrl Pts',(158.834720503539,1.36248314380646,48.5));
#79140=CARTESIAN_POINT('Ctrl Pts',(158.644884180278,1.53055930137634,48.5));
#79141=CARTESIAN_POINT('',(159.134857010096,1.36248314380646,48.35));
#79142=CARTESIAN_POINT('',(159.134857010096,1.36248314380646,48.5));
#79143=CARTESIAN_POINT('',(158.644884180278,1.53055930137634,48.35));
#79144=CARTESIAN_POINT('Ctrl Pts',(159.134857010096,1.36248314380646,48.35));
#79145=CARTESIAN_POINT('Ctrl Pts',(158.834720503539,1.36248314380646,48.35));
#79146=CARTESIAN_POINT('Ctrl Pts',(158.644884180278,1.53055930137634,48.35));
#79147=CARTESIAN_POINT('',(158.644884180278,1.53055930137634,48.5));
#79148=CARTESIAN_POINT('Ctrl Pts',(159.712619435042,1.62960433959961,48.5));
#79149=CARTESIAN_POINT('Ctrl Pts',(159.712619435042,1.62960433959961,48.35));
#79150=CARTESIAN_POINT('Ctrl Pts',(159.501023244113,1.36248314380646,48.5));
#79151=CARTESIAN_POINT('Ctrl Pts',(159.501023244113,1.36248314380646,48.35));
#79152=CARTESIAN_POINT('Ctrl Pts',(159.134857010096,1.36248314380646,48.5));
#79153=CARTESIAN_POINT('Ctrl Pts',(159.134857010096,1.36248314380646,48.35));
#79154=CARTESIAN_POINT('',(159.712619435042,1.62960433959961,48.5));
#79155=CARTESIAN_POINT('Ctrl Pts',(159.712619435042,1.62960433959961,48.5));
#79156=CARTESIAN_POINT('Ctrl Pts',(159.501023244113,1.36248314380646,48.5));
#79157=CARTESIAN_POINT('Ctrl Pts',(159.134857010096,1.36248314380646,48.5));
#79158=CARTESIAN_POINT('',(159.712619435042,1.62960433959961,48.35));
#79159=CARTESIAN_POINT('',(159.712619435042,1.62960433959961,48.5));
#79160=CARTESIAN_POINT('Ctrl Pts',(159.712619435042,1.62960433959961,48.35));
#79161=CARTESIAN_POINT('Ctrl Pts',(159.501023244113,1.36248314380646,48.35));
#79162=CARTESIAN_POINT('Ctrl Pts',(159.134857010096,1.36248314380646,48.35));
#79163=CARTESIAN_POINT('Ctrl Pts',(159.886698674411,2.14583912491798,48.5));
#79164=CARTESIAN_POINT('Ctrl Pts',(159.886698674411,2.14583912491798,48.35));
#79165=CARTESIAN_POINT('Ctrl Pts',(159.886698674411,1.84720331430435,48.5));
#79166=CARTESIAN_POINT('Ctrl Pts',(159.886698674411,1.84720331430435,48.35));
#79167=CARTESIAN_POINT('Ctrl Pts',(159.712619435042,1.62960433959961,48.5));
#79168=CARTESIAN_POINT('Ctrl Pts',(159.712619435042,1.62960433959961,48.35));
#79169=CARTESIAN_POINT('',(159.886698674411,2.14583912491798,48.5));
#79170=CARTESIAN_POINT('Ctrl Pts',(159.886698674411,2.14583912491798,48.5));
#79171=CARTESIAN_POINT('Ctrl Pts',(159.886698674411,1.84720331430435,48.5));
#79172=CARTESIAN_POINT('Ctrl Pts',(159.712619435042,1.62960433959961,48.5));
#79173=CARTESIAN_POINT('',(159.886698674411,2.14583912491798,48.35));
#79174=CARTESIAN_POINT('',(159.886698674411,2.14583912491798,48.5));
#79175=CARTESIAN_POINT('Ctrl Pts',(159.886698674411,2.14583912491798,48.35));
#79176=CARTESIAN_POINT('Ctrl Pts',(159.886698674411,1.84720331430435,48.35));
#79177=CARTESIAN_POINT('Ctrl Pts',(159.712619435042,1.62960433959961,48.35));
#79178=CARTESIAN_POINT('Ctrl Pts',(159.688608597964,2.65907236933708,48.5));
#79179=CARTESIAN_POINT('Ctrl Pts',(159.688608597964,2.65907236933708,48.35));
#79180=CARTESIAN_POINT('Ctrl Pts',(159.886698674411,2.45948159694672,48.5));
#79181=CARTESIAN_POINT('Ctrl Pts',(159.886698674411,2.45948159694672,48.35));
#79182=CARTESIAN_POINT('Ctrl Pts',(159.886698674411,2.14583912491798,48.5));
#79183=CARTESIAN_POINT('Ctrl Pts',(159.886698674411,2.14583912491798,48.35));
#79184=CARTESIAN_POINT('',(159.688608597964,2.65907236933708,48.5));
#79185=CARTESIAN_POINT('Ctrl Pts',(159.688608597964,2.65907236933708,48.5));
#79186=CARTESIAN_POINT('Ctrl Pts',(159.886698674411,2.45948159694672,48.5));
#79187=CARTESIAN_POINT('Ctrl Pts',(159.886698674411,2.14583912491798,48.5));
#79188=CARTESIAN_POINT('',(159.688608597964,2.65907236933708,48.35));
#79189=CARTESIAN_POINT('',(159.688608597964,2.65907236933708,48.5));
#79190=CARTESIAN_POINT('Ctrl Pts',(159.688608597964,2.65907236933708,48.35));
#79191=CARTESIAN_POINT('Ctrl Pts',(159.886698674411,2.45948159694672,48.35));
#79192=CARTESIAN_POINT('Ctrl Pts',(159.886698674411,2.14583912491798,48.35));
#79193=CARTESIAN_POINT('Ctrl Pts',(159.202387582511,2.85866314172745,48.5));
#79194=CARTESIAN_POINT('Ctrl Pts',(159.202387582511,2.85866314172745,48.35));
#79195=CARTESIAN_POINT('Ctrl Pts',(159.490518521518,2.85866314172745,48.5));
#79196=CARTESIAN_POINT('Ctrl Pts',(159.490518521518,2.85866314172745,48.35));
#79197=CARTESIAN_POINT('Ctrl Pts',(159.688608597964,2.65907236933708,48.5));
#79198=CARTESIAN_POINT('Ctrl Pts',(159.688608597964,2.65907236933708,48.35));
#79199=CARTESIAN_POINT('',(159.202387582511,2.85866314172745,48.5));
#79200=CARTESIAN_POINT('Ctrl Pts',(159.202387582511,2.85866314172745,48.5));
#79201=CARTESIAN_POINT('Ctrl Pts',(159.490518521518,2.85866314172745,48.5));
#79202=CARTESIAN_POINT('Ctrl Pts',(159.688608597964,2.65907236933708,48.5));
#79203=CARTESIAN_POINT('',(159.202387582511,2.85866314172745,48.35));
#79204=CARTESIAN_POINT('',(159.202387582511,2.85866314172745,48.5));
#79205=CARTESIAN_POINT('Ctrl Pts',(159.202387582511,2.85866314172745,48.35));
#79206=CARTESIAN_POINT('Ctrl Pts',(159.490518521518,2.85866314172745,48.35));
#79207=CARTESIAN_POINT('Ctrl Pts',(159.688608597964,2.65907236933708,48.35));
#79208=CARTESIAN_POINT('Ctrl Pts',(158.786698680371,2.72060030698776,48.5));
#79209=CARTESIAN_POINT('Ctrl Pts',(158.786698680371,2.72060030698776,48.35));
#79210=CARTESIAN_POINT('Ctrl Pts',(158.984788607806,2.85866314172745,48.5));
#79211=CARTESIAN_POINT('Ctrl Pts',(158.984788607806,2.85866314172745,48.35));
#79212=CARTESIAN_POINT('Ctrl Pts',(159.202387582511,2.85866314172745,48.5));
#79213=CARTESIAN_POINT('Ctrl Pts',(159.202387582511,2.85866314172745,48.35));
#79214=CARTESIAN_POINT('',(158.786698680371,2.72060030698776,48.5));
#79215=CARTESIAN_POINT('Ctrl Pts',(158.786698680371,2.72060030698776,48.5));
#79216=CARTESIAN_POINT('Ctrl Pts',(158.984788607806,2.85866314172745,48.5));
#79217=CARTESIAN_POINT('Ctrl Pts',(159.202387582511,2.85866314172745,48.5));
#79218=CARTESIAN_POINT('',(158.786698680371,2.72060030698776,48.35));
#79219=CARTESIAN_POINT('',(158.786698680371,2.72060030698776,48.5));
#79220=CARTESIAN_POINT('Ctrl Pts',(158.786698680371,2.72060030698776,48.35));
#79221=CARTESIAN_POINT('Ctrl Pts',(158.984788607806,2.85866314172745,48.35));
#79222=CARTESIAN_POINT('Ctrl Pts',(159.202387582511,2.85866314172745,48.35));
#79223=CARTESIAN_POINT('Origin',(158.905252467841,3.31186899542809,48.5));
#79224=CARTESIAN_POINT('',(158.905252467841,3.31186899542809,48.5));
#79225=CARTESIAN_POINT('',(156.286292429022,-9.74978934782317,48.5));
#79226=CARTESIAN_POINT('',(158.905252467841,3.31186899542809,48.35));
#79227=CARTESIAN_POINT('',(158.905252467841,3.31186899542809,48.5));
#79228=CARTESIAN_POINT('',(158.905252467841,3.31186899542809,48.35));
#79229=CARTESIAN_POINT('Origin',(159.783151399344,3.31186899542809,48.5));
#79230=CARTESIAN_POINT('',(159.783151399344,3.31186899542809,48.5));
#79231=CARTESIAN_POINT('',(79.8915756996721,3.31186899542809,48.5));
#79232=CARTESIAN_POINT('',(159.783151399344,3.31186899542809,48.35));
#79233=CARTESIAN_POINT('',(159.783151399344,3.31186899542809,48.5));
#79234=CARTESIAN_POINT('',(159.783151399344,3.31186899542809,48.35));
#79235=CARTESIAN_POINT('Origin',(159.783151399344,3.56998646259308,48.5));
#79236=CARTESIAN_POINT('',(159.783151399344,3.56998646259308,48.5));
#79237=CARTESIAN_POINT('',(159.783151399344,5.78499323129654,48.5));
#79238=CARTESIAN_POINT('',(159.783151399344,3.56998646259308,48.35));
#79239=CARTESIAN_POINT('',(159.783151399344,3.56998646259308,48.5));
#79240=CARTESIAN_POINT('',(159.783151399344,3.56998646259308,48.35));
#79241=CARTESIAN_POINT('Origin',(158.689154338092,3.56998646259308,48.5));
#79242=CARTESIAN_POINT('',(158.689154338092,3.56998646259308,48.5));
#79243=CARTESIAN_POINT('',(79.3445771690458,3.56998646259308,48.5));
#79244=CARTESIAN_POINT('',(158.689154338092,3.56998646259308,48.35));
#79245=CARTESIAN_POINT('',(158.689154338092,3.56998646259308,48.5));
#79246=CARTESIAN_POINT('',(158.689154338092,3.56998646259308,48.35));
#79247=CARTESIAN_POINT('Origin',(158.476057451218,2.43997284770012,48.5));
#79248=CARTESIAN_POINT('',(158.476057451218,2.43997284770012,48.5));
#79249=CARTESIAN_POINT('',(156.261207188242,-9.30497091396423,48.5));
#79250=CARTESIAN_POINT('',(158.476057451218,2.43997284770012,48.35));
#79251=CARTESIAN_POINT('',(158.476057451218,2.43997284770012,48.5));
#79252=CARTESIAN_POINT('',(158.476057451218,2.43997284770012,48.35));
#79253=CARTESIAN_POINT('Origin',(158.72967268154,2.40695783495903,48.5));
#79254=CARTESIAN_POINT('',(158.72967268154,2.40695783495903,48.5));
#79255=CARTESIAN_POINT('',(80.3293789433537,12.6129170487894,48.5));
#79256=CARTESIAN_POINT('',(158.72967268154,2.40695783495903,48.35));
#79257=CARTESIAN_POINT('',(158.72967268154,2.40695783495903,48.5));
#79258=CARTESIAN_POINT('',(158.72967268154,2.40695783495903,48.35));
#79259=CARTESIAN_POINT('Ctrl Pts',(158.894747745246,2.56077775359154,48.5));
#79260=CARTESIAN_POINT('Ctrl Pts',(158.894747745246,2.56077775359154,48.35));
#79261=CARTESIAN_POINT('Ctrl Pts',(158.789700072259,2.5015007853508,48.5));
#79262=CARTESIAN_POINT('Ctrl Pts',(158.789700072259,2.5015007853508,48.35));
#79263=CARTESIAN_POINT('Ctrl Pts',(158.72967268154,2.40695783495903,48.5));
#79264=CARTESIAN_POINT('Ctrl Pts',(158.72967268154,2.40695783495903,48.35));
#79265=CARTESIAN_POINT('',(158.894747745246,2.56077775359154,48.5));
#79266=CARTESIAN_POINT('Ctrl Pts',(158.894747745246,2.56077775359154,48.5));
#79267=CARTESIAN_POINT('Ctrl Pts',(158.789700072259,2.5015007853508,48.5));
#79268=CARTESIAN_POINT('Ctrl Pts',(158.72967268154,2.40695783495903,48.5));
#79269=CARTESIAN_POINT('',(158.894747745246,2.56077775359154,48.35));
#79270=CARTESIAN_POINT('',(158.894747745246,2.56077775359154,48.5));
#79271=CARTESIAN_POINT('Ctrl Pts',(158.894747745246,2.56077775359154,48.35));
#79272=CARTESIAN_POINT('Ctrl Pts',(158.789700072259,2.5015007853508,48.35));
#79273=CARTESIAN_POINT('Ctrl Pts',(158.72967268154,2.40695783495903,48.35));
#79274=CARTESIAN_POINT('Ctrl Pts',(159.130354773253,2.62005472183228,48.5));
#79275=CARTESIAN_POINT('Ctrl Pts',(159.130354773253,2.62005472183228,48.35));
#79276=CARTESIAN_POINT('Ctrl Pts',(158.999795567244,2.62005472183228,48.5));
#79277=CARTESIAN_POINT('Ctrl Pts',(158.999795567244,2.62005472183228,48.35));
#79278=CARTESIAN_POINT('Ctrl Pts',(158.894747745246,2.56077775359154,48.5));
#79279=CARTESIAN_POINT('Ctrl Pts',(158.894747745246,2.56077775359154,48.35));
#79280=CARTESIAN_POINT('',(159.130354773253,2.62005472183228,48.5));
#79281=CARTESIAN_POINT('Ctrl Pts',(159.130354773253,2.62005472183228,48.5));
#79282=CARTESIAN_POINT('Ctrl Pts',(158.999795567244,2.62005472183228,48.5));
#79283=CARTESIAN_POINT('Ctrl Pts',(158.894747745246,2.56077775359154,48.5));
#79284=CARTESIAN_POINT('',(159.130354773253,2.62005472183228,48.35));
#79285=CARTESIAN_POINT('',(159.130354773253,2.62005472183228,48.5));
#79286=CARTESIAN_POINT('Ctrl Pts',(159.130354773253,2.62005472183228,48.35));
#79287=CARTESIAN_POINT('Ctrl Pts',(158.999795567244,2.62005472183228,48.35));
#79288=CARTESIAN_POINT('Ctrl Pts',(158.894747745246,2.56077775359154,48.35));
#79289=CARTESIAN_POINT('Ctrl Pts',(159.470259200782,2.48649397492409,48.5));
#79290=CARTESIAN_POINT('Ctrl Pts',(159.470259200782,2.48649397492409,48.35));
#79291=CARTESIAN_POINT('Ctrl Pts',(159.34045041725,2.62005472183228,48.5));
#79292=CARTESIAN_POINT('Ctrl Pts',(159.34045041725,2.62005472183228,48.35));
#79293=CARTESIAN_POINT('Ctrl Pts',(159.130354773253,2.62005472183228,48.5));
#79294=CARTESIAN_POINT('Ctrl Pts',(159.130354773253,2.62005472183228,48.35));
#79295=CARTESIAN_POINT('',(159.470259200782,2.48649397492409,48.5));
#79296=CARTESIAN_POINT('Ctrl Pts',(159.470259200782,2.48649397492409,48.5));
#79297=CARTESIAN_POINT('Ctrl Pts',(159.34045041725,2.62005472183228,48.5));
#79298=CARTESIAN_POINT('Ctrl Pts',(159.130354773253,2.62005472183228,48.5));
#79299=CARTESIAN_POINT('',(159.470259200782,2.48649397492409,48.35));
#79300=CARTESIAN_POINT('',(159.470259200782,2.48649397492409,48.5));
#79301=CARTESIAN_POINT('Ctrl Pts',(159.470259200782,2.48649397492409,48.35));
#79302=CARTESIAN_POINT('Ctrl Pts',(159.34045041725,2.62005472183228,48.35));
#79303=CARTESIAN_POINT('Ctrl Pts',(159.130354773253,2.62005472183228,48.35));
#79304=CARTESIAN_POINT('Ctrl Pts',(159.600068580359,2.12182813882828,48.5));
#79305=CARTESIAN_POINT('Ctrl Pts',(159.600068580359,2.12182813882828,48.35));
#79306=CARTESIAN_POINT('Ctrl Pts',(159.600068580359,2.3529332280159,48.5));
#79307=CARTESIAN_POINT('Ctrl Pts',(159.600068580359,2.3529332280159,48.35));
#79308=CARTESIAN_POINT('Ctrl Pts',(159.470259200782,2.48649397492409,48.5));
#79309=CARTESIAN_POINT('Ctrl Pts',(159.470259200782,2.48649397492409,48.35));
#79310=CARTESIAN_POINT('',(159.600068580359,2.12182813882828,48.5));
#79311=CARTESIAN_POINT('Ctrl Pts',(159.600068580359,2.12182813882828,48.5));
#79312=CARTESIAN_POINT('Ctrl Pts',(159.600068580359,2.3529332280159,48.5));
#79313=CARTESIAN_POINT('Ctrl Pts',(159.470259200782,2.48649397492409,48.5));
#79314=CARTESIAN_POINT('',(159.600068580359,2.12182813882828,48.35));
#79315=CARTESIAN_POINT('',(159.600068580359,2.12182813882828,48.5));
#79316=CARTESIAN_POINT('Ctrl Pts',(159.600068580359,2.12182813882828,48.35));
#79317=CARTESIAN_POINT('Ctrl Pts',(159.600068580359,2.3529332280159,48.35));
#79318=CARTESIAN_POINT('Ctrl Pts',(159.470259200782,2.48649397492409,48.35));
#79319=CARTESIAN_POINT('Ctrl Pts',(159.465006839484,1.73165076971054,48.5));
#79320=CARTESIAN_POINT('Ctrl Pts',(159.465006839484,1.73165076971054,48.35));
#79321=CARTESIAN_POINT('Ctrl Pts',(159.600068580359,1.87871778011322,48.5));
#79322=CARTESIAN_POINT('Ctrl Pts',(159.600068580359,1.87871778011322,48.35));
#79323=CARTESIAN_POINT('Ctrl Pts',(159.600068580359,2.12182813882828,48.5));
#79324=CARTESIAN_POINT('Ctrl Pts',(159.600068580359,2.12182813882828,48.35));
#79325=CARTESIAN_POINT('',(159.465006839484,1.73165076971054,48.5));
#79326=CARTESIAN_POINT('Ctrl Pts',(159.465006839484,1.73165076971054,48.5));
#79327=CARTESIAN_POINT('Ctrl Pts',(159.600068580359,1.87871778011322,48.5));
#79328=CARTESIAN_POINT('Ctrl Pts',(159.600068580359,2.12182813882828,48.5));
#79329=CARTESIAN_POINT('',(159.465006839484,1.73165076971054,48.35));
#79330=CARTESIAN_POINT('',(159.465006839484,1.73165076971054,48.5));
#79331=CARTESIAN_POINT('Ctrl Pts',(159.465006839484,1.73165076971054,48.35));
#79332=CARTESIAN_POINT('Ctrl Pts',(159.600068580359,1.87871778011322,48.35));
#79333=CARTESIAN_POINT('Ctrl Pts',(159.600068580359,2.12182813882828,48.35));
#79334=CARTESIAN_POINT('Ctrl Pts',(159.134857010096,1.58458405733109,48.5));
#79335=CARTESIAN_POINT('Ctrl Pts',(159.134857010096,1.58458405733109,48.35));
#79336=CARTESIAN_POINT('Ctrl Pts',(159.329945545644,1.58458405733109,48.5));
#79337=CARTESIAN_POINT('Ctrl Pts',(159.329945545644,1.58458405733109,48.35));
#79338=CARTESIAN_POINT('Ctrl Pts',(159.465006839484,1.73165076971054,48.5));
#79339=CARTESIAN_POINT('Ctrl Pts',(159.465006839484,1.73165076971054,48.35));
#79340=CARTESIAN_POINT('',(159.134857010096,1.58458405733109,48.5));
#79341=CARTESIAN_POINT('Ctrl Pts',(159.134857010096,1.58458405733109,48.5));
#79342=CARTESIAN_POINT('Ctrl Pts',(159.329945545644,1.58458405733109,48.5));
#79343=CARTESIAN_POINT('Ctrl Pts',(159.465006839484,1.73165076971054,48.5));
#79344=CARTESIAN_POINT('',(159.134857010096,1.58458405733109,48.35));
#79345=CARTESIAN_POINT('',(159.134857010096,1.58458405733109,48.5));
#79346=CARTESIAN_POINT('Ctrl Pts',(159.134857010096,1.58458405733109,48.35));
#79347=CARTESIAN_POINT('Ctrl Pts',(159.329945545644,1.58458405733109,48.35));
#79348=CARTESIAN_POINT('Ctrl Pts',(159.465006839484,1.73165076971054,48.35));
#79349=CARTESIAN_POINT('Ctrl Pts',(158.857981067151,1.68888145685196,48.5));
#79350=CARTESIAN_POINT('Ctrl Pts',(158.857981067151,1.68888145685196,48.35));
#79351=CARTESIAN_POINT('Ctrl Pts',(158.972783338279,1.58458405733109,48.5));
#79352=CARTESIAN_POINT('Ctrl Pts',(158.972783338279,1.58458405733109,48.35));
#79353=CARTESIAN_POINT('Ctrl Pts',(159.134857010096,1.58458405733109,48.5));
#79354=CARTESIAN_POINT('Ctrl Pts',(159.134857010096,1.58458405733109,48.35));
#79355=CARTESIAN_POINT('',(158.857981067151,1.68888145685196,48.5));
#79356=CARTESIAN_POINT('Ctrl Pts',(158.857981067151,1.68888145685196,48.5));
#79357=CARTESIAN_POINT('Ctrl Pts',(158.972783338279,1.58458405733109,48.5));
#79358=CARTESIAN_POINT('Ctrl Pts',(159.134857010096,1.58458405733109,48.5));
#79359=CARTESIAN_POINT('',(158.857981067151,1.68888145685196,48.35));
#79360=CARTESIAN_POINT('',(158.857981067151,1.68888145685196,48.5));
#79361=CARTESIAN_POINT('Ctrl Pts',(158.857981067151,1.68888145685196,48.35));
#79362=CARTESIAN_POINT('Ctrl Pts',(158.972783338279,1.58458405733109,48.35));
#79363=CARTESIAN_POINT('Ctrl Pts',(159.134857010096,1.58458405733109,48.35));
#79364=CARTESIAN_POINT('Ctrl Pts',(158.711664628237,2.00027281045914,48.5));
#79365=CARTESIAN_POINT('Ctrl Pts',(158.711664628237,2.00027281045914,48.35));
#79366=CARTESIAN_POINT('Ctrl Pts',(158.743178796023,1.79317885637283,48.5));
#79367=CARTESIAN_POINT('Ctrl Pts',(158.743178796023,1.79317885637283,48.35));
#79368=CARTESIAN_POINT('Ctrl Pts',(158.857981067151,1.68888145685196,48.5));
#79369=CARTESIAN_POINT('Ctrl Pts',(158.857981067151,1.68888145685196,48.35));
#79370=CARTESIAN_POINT('',(158.711664628237,2.00027281045914,48.5));
#79371=CARTESIAN_POINT('Ctrl Pts',(158.711664628237,2.00027281045914,48.5));
#79372=CARTESIAN_POINT('Ctrl Pts',(158.743178796023,1.79317885637283,48.5));
#79373=CARTESIAN_POINT('Ctrl Pts',(158.857981067151,1.68888145685196,48.5));
#79374=CARTESIAN_POINT('',(158.711664628237,2.00027281045914,48.35));
#79375=CARTESIAN_POINT('',(158.711664628237,2.00027281045914,48.5));
#79376=CARTESIAN_POINT('Ctrl Pts',(158.711664628237,2.00027281045914,48.35));
#79377=CARTESIAN_POINT('Ctrl Pts',(158.743178796023,1.79317885637283,48.35));
#79378=CARTESIAN_POINT('Ctrl Pts',(158.857981067151,1.68888145685196,48.35));
#79379=CARTESIAN_POINT('Origin',(158.428035628051,1.97626197338104,48.5));
#79380=CARTESIAN_POINT('',(158.428035628051,1.97626197338104,48.5));
#79381=CARTESIAN_POINT('',(80.0308315852229,-4.6605152687554,48.5));
#79382=CARTESIAN_POINT('',(158.428035628051,1.97626197338104,48.35));
#79383=CARTESIAN_POINT('',(158.428035628051,1.97626197338104,48.5));
#79384=CARTESIAN_POINT('',(158.428035628051,1.97626197338104,48.35));
#79385=CARTESIAN_POINT('Ctrl Pts',(158.644884180278,1.53055930137634,48.5));
#79386=CARTESIAN_POINT('Ctrl Pts',(158.644884180278,1.53055930137634,48.35));
#79387=CARTESIAN_POINT('Ctrl Pts',(158.455047857016,1.69863575696945,48.5));
#79388=CARTESIAN_POINT('Ctrl Pts',(158.455047857016,1.69863575696945,48.35));
#79389=CARTESIAN_POINT('Ctrl Pts',(158.428035628051,1.97626197338104,48.5));
#79390=CARTESIAN_POINT('Ctrl Pts',(158.428035628051,1.97626197338104,48.35));
#79391=CARTESIAN_POINT('Ctrl Pts',(158.644884180278,1.53055930137634,48.5));
#79392=CARTESIAN_POINT('Ctrl Pts',(158.455047857016,1.69863575696945,48.5));
#79393=CARTESIAN_POINT('Ctrl Pts',(158.428035628051,1.97626197338104,48.5));
#79394=CARTESIAN_POINT('Ctrl Pts',(158.644884180278,1.53055930137634,48.35));
#79395=CARTESIAN_POINT('Ctrl Pts',(158.455047857016,1.69863575696945,48.35));
#79396=CARTESIAN_POINT('Ctrl Pts',(158.428035628051,1.97626197338104,48.35));
#79397=CARTESIAN_POINT('Origin',(159.999999951571,2.48574362695217,48.35));
#79398=CARTESIAN_POINT('Origin',(0.,8.,48.5));
#79399=CARTESIAN_POINT('Ctrl Pts',(150.895907462575,3.38540250062943,48.5));
#79400=CARTESIAN_POINT('Ctrl Pts',(150.895907462575,3.38540250062943,48.35));
#79401=CARTESIAN_POINT('Ctrl Pts',(150.709822655655,3.38540250062943,48.5));
#79402=CARTESIAN_POINT('Ctrl Pts',(150.709822655655,3.38540250062943,48.35));
#79403=CARTESIAN_POINT('Ctrl Pts',(150.598772347905,3.22783091664314,48.5));
#79404=CARTESIAN_POINT('Ctrl Pts',(150.598772347905,3.22783091664314,48.35));
#79405=CARTESIAN_POINT('',(150.895907462575,3.38540250062943,48.5));
#79406=CARTESIAN_POINT('',(150.598772347905,3.22783091664314,48.5));
#79407=CARTESIAN_POINT('Ctrl Pts',(150.895907462575,3.38540250062943,48.5));
#79408=CARTESIAN_POINT('Ctrl Pts',(150.709822655655,3.38540250062943,48.5));
#79409=CARTESIAN_POINT('Ctrl Pts',(150.598772347905,3.22783091664314,48.5));
#79410=CARTESIAN_POINT('',(150.895907462575,3.38540250062943,48.35));
#79411=CARTESIAN_POINT('',(150.895907462575,3.38540250062943,48.5));
#79412=CARTESIAN_POINT('',(150.598772347905,3.22783091664314,48.35));
#79413=CARTESIAN_POINT('Ctrl Pts',(150.895907462575,3.38540250062943,48.35));
#79414=CARTESIAN_POINT('Ctrl Pts',(150.709822655655,3.38540250062943,48.35));
#79415=CARTESIAN_POINT('Ctrl Pts',(150.598772347905,3.22783091664314,48.35));
#79416=CARTESIAN_POINT('',(150.598772347905,3.22783091664314,48.5));
#79417=CARTESIAN_POINT('Ctrl Pts',(151.211800755002,3.2068213224411,48.5));
#79418=CARTESIAN_POINT('Ctrl Pts',(151.211800755002,3.2068213224411,48.35));
#79419=CARTESIAN_POINT('Ctrl Pts',(151.084993065335,3.38540250062943,48.5));
#79420=CARTESIAN_POINT('Ctrl Pts',(151.084993065335,3.38540250062943,48.35));
#79421=CARTESIAN_POINT('Ctrl Pts',(150.895907462575,3.38540250062943,48.5));
#79422=CARTESIAN_POINT('Ctrl Pts',(150.895907462575,3.38540250062943,48.35));
#79423=CARTESIAN_POINT('',(151.211800755002,3.2068213224411,48.5));
#79424=CARTESIAN_POINT('Ctrl Pts',(151.211800755002,3.2068213224411,48.5));
#79425=CARTESIAN_POINT('Ctrl Pts',(151.084993065335,3.38540250062943,48.5));
#79426=CARTESIAN_POINT('Ctrl Pts',(150.895907462575,3.38540250062943,48.5));
#79427=CARTESIAN_POINT('',(151.211800755002,3.2068213224411,48.35));
#79428=CARTESIAN_POINT('',(151.211800755002,3.2068213224411,48.5));
#79429=CARTESIAN_POINT('Ctrl Pts',(151.211800755002,3.2068213224411,48.35));
#79430=CARTESIAN_POINT('Ctrl Pts',(151.084993065335,3.38540250062943,48.35));
#79431=CARTESIAN_POINT('Ctrl Pts',(150.895907462575,3.38540250062943,48.35));
#79432=CARTESIAN_POINT('Ctrl Pts',(151.338608444668,2.48499327898026,48.5));
#79433=CARTESIAN_POINT('Ctrl Pts',(151.338608444668,2.48499327898026,48.35));
#79434=CARTESIAN_POINT('Ctrl Pts',(151.338608444668,3.02824014425278,48.5));
#79435=CARTESIAN_POINT('Ctrl Pts',(151.338608444668,3.02824014425278,48.35));
#79436=CARTESIAN_POINT('Ctrl Pts',(151.211800755002,3.2068213224411,48.5));
#79437=CARTESIAN_POINT('Ctrl Pts',(151.211800755002,3.2068213224411,48.35));
#79438=CARTESIAN_POINT('',(151.338608444668,2.48499327898026,48.5));
#79439=CARTESIAN_POINT('Ctrl Pts',(151.338608444668,2.48499327898026,48.5));
#79440=CARTESIAN_POINT('Ctrl Pts',(151.338608444668,3.02824014425278,48.5));
#79441=CARTESIAN_POINT('Ctrl Pts',(151.211800755002,3.2068213224411,48.5));
#79442=CARTESIAN_POINT('',(151.338608444668,2.48499327898026,48.35));
#79443=CARTESIAN_POINT('',(151.338608444668,2.48499327898026,48.5));
#79444=CARTESIAN_POINT('Ctrl Pts',(151.338608444668,2.48499327898026,48.35));
#79445=CARTESIAN_POINT('Ctrl Pts',(151.338608444668,3.02824014425278,48.35));
#79446=CARTESIAN_POINT('Ctrl Pts',(151.211800755002,3.2068213224411,48.35));
#79447=CARTESIAN_POINT('Ctrl Pts',(151.211800755002,1.76466578245163,48.5));
#79448=CARTESIAN_POINT('Ctrl Pts',(151.211800755002,1.76466578245163,48.35));
#79449=CARTESIAN_POINT('Ctrl Pts',(151.338608444668,1.9447478055954,48.5));
#79450=CARTESIAN_POINT('Ctrl Pts',(151.338608444668,1.9447478055954,48.35));
#79451=CARTESIAN_POINT('Ctrl Pts',(151.338608444668,2.48499327898026,48.5));
#79452=CARTESIAN_POINT('Ctrl Pts',(151.338608444668,2.48499327898026,48.35));
#79453=CARTESIAN_POINT('',(151.211800755002,1.76466578245163,48.5));
#79454=CARTESIAN_POINT('Ctrl Pts',(151.211800755002,1.76466578245163,48.5));
#79455=CARTESIAN_POINT('Ctrl Pts',(151.338608444668,1.9447478055954,48.5));
#79456=CARTESIAN_POINT('Ctrl Pts',(151.338608444668,2.48499327898026,48.5));
#79457=CARTESIAN_POINT('',(151.211800755002,1.76466578245163,48.35));
#79458=CARTESIAN_POINT('',(151.211800755002,1.76466578245163,48.5));
#79459=CARTESIAN_POINT('Ctrl Pts',(151.211800755002,1.76466578245163,48.35));
#79460=CARTESIAN_POINT('Ctrl Pts',(151.338608444668,1.9447478055954,48.35));
#79461=CARTESIAN_POINT('Ctrl Pts',(151.338608444668,2.48499327898026,48.35));
#79462=CARTESIAN_POINT('Ctrl Pts',(150.898908556439,1.58458405733109,48.5));
#79463=CARTESIAN_POINT('Ctrl Pts',(150.898908556439,1.58458405733109,48.35));
#79464=CARTESIAN_POINT('Ctrl Pts',(151.084993065335,1.58458405733109,48.5));
#79465=CARTESIAN_POINT('Ctrl Pts',(151.084993065335,1.58458405733109,48.35));
#79466=CARTESIAN_POINT('Ctrl Pts',(151.211800755002,1.76466578245163,48.5));
#79467=CARTESIAN_POINT('Ctrl Pts',(151.211800755002,1.76466578245163,48.35));
#79468=CARTESIAN_POINT('',(150.898908556439,1.58458405733109,48.5));
#79469=CARTESIAN_POINT('Ctrl Pts',(150.898908556439,1.58458405733109,48.5));
#79470=CARTESIAN_POINT('Ctrl Pts',(151.084993065335,1.58458405733109,48.5));
#79471=CARTESIAN_POINT('Ctrl Pts',(151.211800755002,1.76466578245163,48.5));
#79472=CARTESIAN_POINT('',(150.898908556439,1.58458405733109,48.35));
#79473=CARTESIAN_POINT('',(150.898908556439,1.58458405733109,48.5));
#79474=CARTESIAN_POINT('Ctrl Pts',(150.898908556439,1.58458405733109,48.35));
#79475=CARTESIAN_POINT('Ctrl Pts',(151.084993065335,1.58458405733109,48.35));
#79476=CARTESIAN_POINT('Ctrl Pts',(151.211800755002,1.76466578245163,48.35));
#79477=CARTESIAN_POINT('Ctrl Pts',(150.586016357876,1.76391565799713,48.5));
#79478=CARTESIAN_POINT('Ctrl Pts',(150.586016357876,1.76391565799713,48.35));
#79479=CARTESIAN_POINT('Ctrl Pts',(150.712824047543,1.58458405733109,48.5));
#79480=CARTESIAN_POINT('Ctrl Pts',(150.712824047543,1.58458405733109,48.35));
#79481=CARTESIAN_POINT('Ctrl Pts',(150.898908556439,1.58458405733109,48.5));
#79482=CARTESIAN_POINT('Ctrl Pts',(150.898908556439,1.58458405733109,48.35));
#79483=CARTESIAN_POINT('',(150.586016357876,1.76391565799713,48.5));
#79484=CARTESIAN_POINT('Ctrl Pts',(150.586016357876,1.76391565799713,48.5));
#79485=CARTESIAN_POINT('Ctrl Pts',(150.712824047543,1.58458405733109,48.5));
#79486=CARTESIAN_POINT('Ctrl Pts',(150.898908556439,1.58458405733109,48.5));
#79487=CARTESIAN_POINT('',(150.586016357876,1.76391565799713,48.35));
#79488=CARTESIAN_POINT('',(150.586016357876,1.76391565799713,48.5));
#79489=CARTESIAN_POINT('Ctrl Pts',(150.586016357876,1.76391565799713,48.35));
#79490=CARTESIAN_POINT('Ctrl Pts',(150.712824047543,1.58458405733109,48.35));
#79491=CARTESIAN_POINT('Ctrl Pts',(150.898908556439,1.58458405733109,48.35));
#79492=CARTESIAN_POINT('Ctrl Pts',(150.45920866821,2.48499327898026,48.5));
#79493=CARTESIAN_POINT('Ctrl Pts',(150.45920866821,2.48499327898026,48.35));
#79494=CARTESIAN_POINT('Ctrl Pts',(150.45920866821,1.94324696063995,48.5));
#79495=CARTESIAN_POINT('Ctrl Pts',(150.45920866821,1.94324696063995,48.35));
#79496=CARTESIAN_POINT('Ctrl Pts',(150.586016357876,1.76391565799713,48.5));
#79497=CARTESIAN_POINT('Ctrl Pts',(150.586016357876,1.76391565799713,48.35));
#79498=CARTESIAN_POINT('',(150.45920866821,2.48499327898026,48.5));
#79499=CARTESIAN_POINT('Ctrl Pts',(150.45920866821,2.48499327898026,48.5));
#79500=CARTESIAN_POINT('Ctrl Pts',(150.45920866821,1.94324696063995,48.5));
#79501=CARTESIAN_POINT('Ctrl Pts',(150.586016357876,1.76391565799713,48.5));
#79502=CARTESIAN_POINT('',(150.45920866821,2.48499327898026,48.35));
#79503=CARTESIAN_POINT('',(150.45920866821,2.48499327898026,48.5));
#79504=CARTESIAN_POINT('Ctrl Pts',(150.45920866821,2.48499327898026,48.35));
#79505=CARTESIAN_POINT('Ctrl Pts',(150.45920866821,1.94324696063995,48.35));
#79506=CARTESIAN_POINT('Ctrl Pts',(150.586016357876,1.76391565799713,48.35));
#79507=CARTESIAN_POINT('Ctrl Pts',(150.598772347905,3.22783091664314,48.5));
#79508=CARTESIAN_POINT('Ctrl Pts',(150.598772347905,3.22783091664314,48.35));
#79509=CARTESIAN_POINT('Ctrl Pts',(150.45920866821,3.02673944830894,48.5));
#79510=CARTESIAN_POINT('Ctrl Pts',(150.45920866821,3.02673944830894,48.35));
#79511=CARTESIAN_POINT('Ctrl Pts',(150.45920866821,2.48499327898026,48.5));
#79512=CARTESIAN_POINT('Ctrl Pts',(150.45920866821,2.48499327898026,48.35));
#79513=CARTESIAN_POINT('Ctrl Pts',(150.598772347905,3.22783091664314,48.5));
#79514=CARTESIAN_POINT('Ctrl Pts',(150.45920866821,3.02673944830894,48.5));
#79515=CARTESIAN_POINT('Ctrl Pts',(150.45920866821,2.48499327898026,48.5));
#79516=CARTESIAN_POINT('Ctrl Pts',(150.598772347905,3.22783091664314,48.35));
#79517=CARTESIAN_POINT('Ctrl Pts',(150.45920866821,3.02673944830894,48.35));
#79518=CARTESIAN_POINT('Ctrl Pts',(150.45920866821,2.48499327898026,48.35));
#79519=CARTESIAN_POINT('Ctrl Pts',(150.898908556439,1.36248314380646,48.5));
#79520=CARTESIAN_POINT('Ctrl Pts',(150.898908556439,1.36248314380646,48.35));
#79521=CARTESIAN_POINT('Ctrl Pts',(150.580763996579,1.36248314380646,48.5));
#79522=CARTESIAN_POINT('Ctrl Pts',(150.580763996579,1.36248314380646,48.35));
#79523=CARTESIAN_POINT('Ctrl Pts',(150.399181426503,1.59058684110642,48.5));
#79524=CARTESIAN_POINT('Ctrl Pts',(150.399181426503,1.59058684110642,48.35));
#79525=CARTESIAN_POINT('',(150.898908556439,1.36248314380646,48.5));
#79526=CARTESIAN_POINT('',(150.399181426503,1.59058684110642,48.5));
#79527=CARTESIAN_POINT('Ctrl Pts',(150.898908556439,1.36248314380646,48.5));
#79528=CARTESIAN_POINT('Ctrl Pts',(150.580763996579,1.36248314380646,48.5));
#79529=CARTESIAN_POINT('Ctrl Pts',(150.399181426503,1.59058684110642,48.5));
#79530=CARTESIAN_POINT('',(150.898908556439,1.36248314380646,48.35));
#79531=CARTESIAN_POINT('',(150.898908556439,1.36248314380646,48.5));
#79532=CARTESIAN_POINT('',(150.399181426503,1.59058684110642,48.35));
#79533=CARTESIAN_POINT('Ctrl Pts',(150.898908556439,1.36248314380646,48.35));
#79534=CARTESIAN_POINT('Ctrl Pts',(150.580763996579,1.36248314380646,48.35));
#79535=CARTESIAN_POINT('Ctrl Pts',(150.399181426503,1.59058684110642,48.35));
#79536=CARTESIAN_POINT('',(150.399181426503,1.59058684110642,48.5));
#79537=CARTESIAN_POINT('Ctrl Pts',(151.298840225674,1.49229192733765,48.5));
#79538=CARTESIAN_POINT('Ctrl Pts',(151.298840225674,1.49229192733765,48.35));
#79539=CARTESIAN_POINT('Ctrl Pts',(151.140518368222,1.36248314380646,48.5));
#79540=CARTESIAN_POINT('Ctrl Pts',(151.140518368222,1.36248314380646,48.35));
#79541=CARTESIAN_POINT('Ctrl Pts',(150.898908556439,1.36248314380646,48.5));
#79542=CARTESIAN_POINT('Ctrl Pts',(150.898908556439,1.36248314380646,48.35));
#79543=CARTESIAN_POINT('',(151.298840225674,1.49229192733765,48.5));
#79544=CARTESIAN_POINT('Ctrl Pts',(151.298840225674,1.49229192733765,48.5));
#79545=CARTESIAN_POINT('Ctrl Pts',(151.140518368222,1.36248314380646,48.5));
#79546=CARTESIAN_POINT('Ctrl Pts',(150.898908556439,1.36248314380646,48.5));
#79547=CARTESIAN_POINT('',(151.298840225674,1.49229192733765,48.35));
#79548=CARTESIAN_POINT('',(151.298840225674,1.49229192733765,48.5));
#79549=CARTESIAN_POINT('Ctrl Pts',(151.298840225674,1.49229192733765,48.35));
#79550=CARTESIAN_POINT('Ctrl Pts',(151.140518368222,1.36248314380646,48.35));
#79551=CARTESIAN_POINT('Ctrl Pts',(150.898908556439,1.36248314380646,48.35));
#79552=CARTESIAN_POINT('Ctrl Pts',(151.536698521115,1.85995900630951,48.5));
#79553=CARTESIAN_POINT('Ctrl Pts',(151.536698521115,1.85995900630951,48.35));
#79554=CARTESIAN_POINT('Ctrl Pts',(151.457162083127,1.62210100889206,48.5));
#79555=CARTESIAN_POINT('Ctrl Pts',(151.457162083127,1.62210100889206,48.35));
#79556=CARTESIAN_POINT('Ctrl Pts',(151.298840225674,1.49229192733765,48.5));
#79557=CARTESIAN_POINT('Ctrl Pts',(151.298840225674,1.49229192733765,48.35));
#79558=CARTESIAN_POINT('',(151.536698521115,1.85995900630951,48.5));
#79559=CARTESIAN_POINT('Ctrl Pts',(151.536698521115,1.85995900630951,48.5));
#79560=CARTESIAN_POINT('Ctrl Pts',(151.457162083127,1.62210100889206,48.5));
#79561=CARTESIAN_POINT('Ctrl Pts',(151.298840225674,1.49229192733765,48.5));
#79562=CARTESIAN_POINT('',(151.536698521115,1.85995900630951,48.35));
#79563=CARTESIAN_POINT('',(151.536698521115,1.85995900630951,48.5));
#79564=CARTESIAN_POINT('Ctrl Pts',(151.536698521115,1.85995900630951,48.35));
#79565=CARTESIAN_POINT('Ctrl Pts',(151.457162083127,1.62210100889206,48.35));
#79566=CARTESIAN_POINT('Ctrl Pts',(151.298840225674,1.49229192733765,48.35));
#79567=CARTESIAN_POINT('Ctrl Pts',(151.616234363057,2.48499327898026,48.5));
#79568=CARTESIAN_POINT('Ctrl Pts',(151.616234363057,2.48499327898026,48.35));
#79569=CARTESIAN_POINT('Ctrl Pts',(151.616234363057,2.09781730175018,48.5));
#79570=CARTESIAN_POINT('Ctrl Pts',(151.616234363057,2.09781730175018,48.35));
#79571=CARTESIAN_POINT('Ctrl Pts',(151.536698521115,1.85995900630951,48.5));
#79572=CARTESIAN_POINT('Ctrl Pts',(151.536698521115,1.85995900630951,48.35));
#79573=CARTESIAN_POINT('',(151.616234363057,2.48499327898026,48.5));
#79574=CARTESIAN_POINT('Ctrl Pts',(151.616234363057,2.48499327898026,48.5));
#79575=CARTESIAN_POINT('Ctrl Pts',(151.616234363057,2.09781730175018,48.5));
#79576=CARTESIAN_POINT('Ctrl Pts',(151.536698521115,1.85995900630951,48.5));
#79577=CARTESIAN_POINT('',(151.616234363057,2.48499327898026,48.35));
#79578=CARTESIAN_POINT('',(151.616234363057,2.48499327898026,48.5));
#79579=CARTESIAN_POINT('Ctrl Pts',(151.616234363057,2.48499327898026,48.35));
#79580=CARTESIAN_POINT('Ctrl Pts',(151.616234363057,2.09781730175018,48.35));
#79581=CARTESIAN_POINT('Ctrl Pts',(151.536698521115,1.85995900630951,48.35));
#79582=CARTESIAN_POINT('Ctrl Pts',(151.566711843945,3.00497958064079,48.5));
#79583=CARTESIAN_POINT('Ctrl Pts',(151.566711843945,3.00497958064079,48.35));
#79584=CARTESIAN_POINT('Ctrl Pts',(151.616234363057,2.81214186549187,48.5));
#79585=CARTESIAN_POINT('Ctrl Pts',(151.616234363057,2.81214186549187,48.35));
#79586=CARTESIAN_POINT('Ctrl Pts',(151.616234363057,2.48499327898026,48.5));
#79587=CARTESIAN_POINT('Ctrl Pts',(151.616234363057,2.48499327898026,48.35));
#79588=CARTESIAN_POINT('',(151.566711843945,3.00497958064079,48.5));
#79589=CARTESIAN_POINT('Ctrl Pts',(151.566711843945,3.00497958064079,48.5));
#79590=CARTESIAN_POINT('Ctrl Pts',(151.616234363057,2.81214186549187,48.5));
#79591=CARTESIAN_POINT('Ctrl Pts',(151.616234363057,2.48499327898026,48.5));
#79592=CARTESIAN_POINT('',(151.566711843945,3.00497958064079,48.35));
#79593=CARTESIAN_POINT('',(151.566711843945,3.00497958064079,48.5));
#79594=CARTESIAN_POINT('Ctrl Pts',(151.566711843945,3.00497958064079,48.35));
#79595=CARTESIAN_POINT('Ctrl Pts',(151.616234363057,2.81214186549187,48.35));
#79596=CARTESIAN_POINT('Ctrl Pts',(151.616234363057,2.48499327898026,48.35));
#79597=CARTESIAN_POINT('Ctrl Pts',(151.430149854161,3.33212831616402,48.5));
#79598=CARTESIAN_POINT('Ctrl Pts',(151.430149854161,3.33212831616402,48.35));
#79599=CARTESIAN_POINT('Ctrl Pts',(151.517189324833,3.19781729578972,48.5));
#79600=CARTESIAN_POINT('Ctrl Pts',(151.517189324833,3.19781729578972,48.35));
#79601=CARTESIAN_POINT('Ctrl Pts',(151.566711843945,3.00497958064079,48.5));
#79602=CARTESIAN_POINT('Ctrl Pts',(151.566711843945,3.00497958064079,48.35));
#79603=CARTESIAN_POINT('',(151.430149854161,3.33212831616402,48.5));
#79604=CARTESIAN_POINT('Ctrl Pts',(151.430149854161,3.33212831616402,48.5));
#79605=CARTESIAN_POINT('Ctrl Pts',(151.517189324833,3.19781729578972,48.5));
#79606=CARTESIAN_POINT('Ctrl Pts',(151.566711843945,3.00497958064079,48.5));
#79607=CARTESIAN_POINT('',(151.430149854161,3.33212831616402,48.35));
#79608=CARTESIAN_POINT('',(151.430149854161,3.33212831616402,48.5));
#79609=CARTESIAN_POINT('Ctrl Pts',(151.430149854161,3.33212831616402,48.35));
#79610=CARTESIAN_POINT('Ctrl Pts',(151.517189324833,3.19781729578972,48.35));
#79611=CARTESIAN_POINT('Ctrl Pts',(151.566711843945,3.00497958064079,48.35));
#79612=CARTESIAN_POINT('Ctrl Pts',(151.209550083615,3.5377217233181,48.5));
#79613=CARTESIAN_POINT('Ctrl Pts',(151.209550083615,3.5377217233181,48.35));
#79614=CARTESIAN_POINT('Ctrl Pts',(151.343110383488,3.46643933653831,48.5));
#79615=CARTESIAN_POINT('Ctrl Pts',(151.343110383488,3.46643933653831,48.35));
#79616=CARTESIAN_POINT('Ctrl Pts',(151.430149854161,3.33212831616402,48.5));
#79617=CARTESIAN_POINT('Ctrl Pts',(151.430149854161,3.33212831616402,48.35));
#79618=CARTESIAN_POINT('',(151.209550083615,3.5377217233181,48.5));
#79619=CARTESIAN_POINT('Ctrl Pts',(151.209550083615,3.5377217233181,48.5));
#79620=CARTESIAN_POINT('Ctrl Pts',(151.343110383488,3.46643933653831,48.5));
#79621=CARTESIAN_POINT('Ctrl Pts',(151.430149854161,3.33212831616402,48.5));
#79622=CARTESIAN_POINT('',(151.209550083615,3.5377217233181,48.35));
#79623=CARTESIAN_POINT('',(151.209550083615,3.5377217233181,48.5));
#79624=CARTESIAN_POINT('Ctrl Pts',(151.209550083615,3.5377217233181,48.35));
#79625=CARTESIAN_POINT('Ctrl Pts',(151.343110383488,3.46643933653831,48.35));
#79626=CARTESIAN_POINT('Ctrl Pts',(151.430149854161,3.33212831616402,48.35));
#79627=CARTESIAN_POINT('Ctrl Pts',(150.898908556439,3.60900411009789,48.5));
#79628=CARTESIAN_POINT('Ctrl Pts',(150.898908556439,3.60900411009789,48.35));
#79629=CARTESIAN_POINT('Ctrl Pts',(151.075989187695,3.60900411009789,48.5));
#79630=CARTESIAN_POINT('Ctrl Pts',(151.075989187695,3.60900411009789,48.35));
#79631=CARTESIAN_POINT('Ctrl Pts',(151.209550083615,3.5377217233181,48.5));
#79632=CARTESIAN_POINT('Ctrl Pts',(151.209550083615,3.5377217233181,48.35));
#79633=CARTESIAN_POINT('',(150.898908556439,3.60900411009789,48.5));
#79634=CARTESIAN_POINT('Ctrl Pts',(150.898908556439,3.60900411009789,48.5));
#79635=CARTESIAN_POINT('Ctrl Pts',(151.075989187695,3.60900411009789,48.5));
#79636=CARTESIAN_POINT('Ctrl Pts',(151.209550083615,3.5377217233181,48.5));
#79637=CARTESIAN_POINT('',(150.898908556439,3.60900411009789,48.35));
#79638=CARTESIAN_POINT('',(150.898908556439,3.60900411009789,48.5));
#79639=CARTESIAN_POINT('Ctrl Pts',(150.898908556439,3.60900411009789,48.35));
#79640=CARTESIAN_POINT('Ctrl Pts',(151.075989187695,3.60900411009789,48.35));
#79641=CARTESIAN_POINT('Ctrl Pts',(151.209550083615,3.5377217233181,48.35));
#79642=CARTESIAN_POINT('Ctrl Pts',(150.500477732159,3.47994545102119,48.5));
#79643=CARTESIAN_POINT('Ctrl Pts',(150.500477732159,3.47994545102119,48.35));
#79644=CARTESIAN_POINT('Ctrl Pts',(150.658799589612,3.60900411009789,48.5));
#79645=CARTESIAN_POINT('Ctrl Pts',(150.658799589612,3.60900411009789,48.35));
#79646=CARTESIAN_POINT('Ctrl Pts',(150.898908556439,3.60900411009789,48.5));
#79647=CARTESIAN_POINT('Ctrl Pts',(150.898908556439,3.60900411009789,48.35));
#79648=CARTESIAN_POINT('',(150.500477732159,3.47994545102119,48.5));
#79649=CARTESIAN_POINT('Ctrl Pts',(150.500477732159,3.47994545102119,48.5));
#79650=CARTESIAN_POINT('Ctrl Pts',(150.658799589612,3.60900411009789,48.5));
#79651=CARTESIAN_POINT('Ctrl Pts',(150.898908556439,3.60900411009789,48.5));
#79652=CARTESIAN_POINT('',(150.500477732159,3.47994545102119,48.35));
#79653=CARTESIAN_POINT('',(150.500477732159,3.47994545102119,48.5));
#79654=CARTESIAN_POINT('Ctrl Pts',(150.500477732159,3.47994545102119,48.35));
#79655=CARTESIAN_POINT('Ctrl Pts',(150.658799589612,3.60900411009789,48.35));
#79656=CARTESIAN_POINT('Ctrl Pts',(150.898908556439,3.60900411009789,48.35));
#79657=CARTESIAN_POINT('Ctrl Pts',(150.261869014241,3.11302864551544,48.5));
#79658=CARTESIAN_POINT('Ctrl Pts',(150.261869014241,3.11302864551544,48.35));
#79659=CARTESIAN_POINT('Ctrl Pts',(150.342155576684,3.3508867919445,48.5));
#79660=CARTESIAN_POINT('Ctrl Pts',(150.342155576684,3.3508867919445,48.35));
#79661=CARTESIAN_POINT('Ctrl Pts',(150.500477732159,3.47994545102119,48.5));
#79662=CARTESIAN_POINT('Ctrl Pts',(150.500477732159,3.47994545102119,48.35));
#79663=CARTESIAN_POINT('',(150.261869014241,3.11302864551544,48.5));
#79664=CARTESIAN_POINT('Ctrl Pts',(150.261869014241,3.11302864551544,48.5));
#79665=CARTESIAN_POINT('Ctrl Pts',(150.342155576684,3.3508867919445,48.5));
#79666=CARTESIAN_POINT('Ctrl Pts',(150.500477732159,3.47994545102119,48.5));
#79667=CARTESIAN_POINT('',(150.261869014241,3.11302864551544,48.35));
#79668=CARTESIAN_POINT('',(150.261869014241,3.11302864551544,48.5));
#79669=CARTESIAN_POINT('Ctrl Pts',(150.261869014241,3.11302864551544,48.35));
#79670=CARTESIAN_POINT('Ctrl Pts',(150.342155576684,3.3508867919445,48.35));
#79671=CARTESIAN_POINT('Ctrl Pts',(150.500477732159,3.47994545102119,48.35));
#79672=CARTESIAN_POINT('Ctrl Pts',(150.181582749821,2.48499327898026,48.5));
#79673=CARTESIAN_POINT('Ctrl Pts',(150.181582749821,2.48499327898026,48.35));
#79674=CARTESIAN_POINT('Ctrl Pts',(150.181582749821,2.87517049908638,48.5));
#79675=CARTESIAN_POINT('Ctrl Pts',(150.181582749821,2.87517049908638,48.35));
#79676=CARTESIAN_POINT('Ctrl Pts',(150.261869014241,3.11302864551544,48.5));
#79677=CARTESIAN_POINT('Ctrl Pts',(150.261869014241,3.11302864551544,48.35));
#79678=CARTESIAN_POINT('',(150.181582749821,2.48499327898026,48.5));
#79679=CARTESIAN_POINT('Ctrl Pts',(150.181582749821,2.48499327898026,48.5));
#79680=CARTESIAN_POINT('Ctrl Pts',(150.181582749821,2.87517049908638,48.5));
#79681=CARTESIAN_POINT('Ctrl Pts',(150.261869014241,3.11302864551544,48.5));
#79682=CARTESIAN_POINT('',(150.181582749821,2.48499327898026,48.35));
#79683=CARTESIAN_POINT('',(150.181582749821,2.48499327898026,48.5));
#79684=CARTESIAN_POINT('Ctrl Pts',(150.181582749821,2.48499327898026,48.35));
#79685=CARTESIAN_POINT('Ctrl Pts',(150.181582749821,2.87517049908638,48.35));
#79686=CARTESIAN_POINT('Ctrl Pts',(150.261869014241,3.11302864551544,48.35));
#79687=CARTESIAN_POINT('Ctrl Pts',(150.399181426503,1.59058684110642,48.5));
#79688=CARTESIAN_POINT('Ctrl Pts',(150.399181426503,1.59058684110642,48.35));
#79689=CARTESIAN_POINT('Ctrl Pts',(150.181582749821,1.86521166563034,48.5));
#79690=CARTESIAN_POINT('Ctrl Pts',(150.181582749821,1.86521166563034,48.35));
#79691=CARTESIAN_POINT('Ctrl Pts',(150.181582749821,2.48499327898026,48.5));
#79692=CARTESIAN_POINT('Ctrl Pts',(150.181582749821,2.48499327898026,48.35));
#79693=CARTESIAN_POINT('Ctrl Pts',(150.399181426503,1.59058684110642,48.5));
#79694=CARTESIAN_POINT('Ctrl Pts',(150.181582749821,1.86521166563034,48.5));
#79695=CARTESIAN_POINT('Ctrl Pts',(150.181582749821,2.48499327898026,48.5));
#79696=CARTESIAN_POINT('Ctrl Pts',(150.399181426503,1.59058684110642,48.35));
#79697=CARTESIAN_POINT('Ctrl Pts',(150.181582749821,1.86521166563034,48.35));
#79698=CARTESIAN_POINT('Ctrl Pts',(150.181582749821,2.48499327898026,48.35));
#79699=CARTESIAN_POINT('Origin',(149.999999956228,2.48574362695217,48.35));
#79700=CARTESIAN_POINT('Origin',(149.338199377991,3.16630297899246,48.5));
#79701=CARTESIAN_POINT('',(149.338199377991,3.16630297899246,48.5));
#79702=CARTESIAN_POINT('',(148.64938619826,2.17435204982758,48.5));
#79703=CARTESIAN_POINT('',(126.178769980074,-30.1852910180208,48.5));
#79704=CARTESIAN_POINT('',(149.338199377991,3.16630297899246,48.35));
#79705=CARTESIAN_POINT('',(149.338199377991,3.16630297899246,48.5));
#79706=CARTESIAN_POINT('',(148.64938619826,2.17435204982758,48.35));
#79707=CARTESIAN_POINT('',(149.338199377991,3.16630297899246,48.35));
#79708=CARTESIAN_POINT('',(148.64938619826,2.17435204982758,48.5));
#79709=CARTESIAN_POINT('Origin',(149.338199377991,2.17435204982758,48.5));
#79710=CARTESIAN_POINT('',(149.338199377991,2.17435204982758,48.5));
#79711=CARTESIAN_POINT('',(149.338199377991,5.08717602491379,48.5));
#79712=CARTESIAN_POINT('',(149.338199377991,2.17435204982758,48.35));
#79713=CARTESIAN_POINT('',(149.338199377991,2.17435204982758,48.5));
#79714=CARTESIAN_POINT('',(149.338199377991,2.17435204982758,48.35));
#79715=CARTESIAN_POINT('Origin',(148.64938619826,2.17435204982758,48.5));
#79716=CARTESIAN_POINT('',(74.3246930991299,2.17435204982758,48.5));
#79717=CARTESIAN_POINT('',(148.64938619826,2.17435204982758,48.35));
#79718=CARTESIAN_POINT('Origin',(149.608321965672,1.92673945426941,48.5));
#79719=CARTESIAN_POINT('',(149.608321965672,1.92673945426941,48.5));
#79720=CARTESIAN_POINT('',(149.608321965672,1.40000009536743,48.5));
#79721=CARTESIAN_POINT('',(149.608321965672,4.9633697271347,48.5));
#79722=CARTESIAN_POINT('',(149.608321965672,1.92673945426941,48.35));
#79723=CARTESIAN_POINT('',(149.608321965672,1.92673945426941,48.5));
#79724=CARTESIAN_POINT('',(149.608321965672,1.40000009536743,48.35));
#79725=CARTESIAN_POINT('',(149.608321965672,1.92673945426941,48.35));
#79726=CARTESIAN_POINT('',(149.608321965672,1.40000009536743,48.5));
#79727=CARTESIAN_POINT('Origin',(149.905457080342,1.92673945426941,48.5));
#79728=CARTESIAN_POINT('',(149.905457080342,1.92673945426941,48.5));
#79729=CARTESIAN_POINT('',(74.9527285401709,1.92673945426941,48.5));
#79730=CARTESIAN_POINT('',(149.905457080342,1.92673945426941,48.35));
#79731=CARTESIAN_POINT('',(149.905457080342,1.92673945426941,48.5));
#79732=CARTESIAN_POINT('',(149.905457080342,1.92673945426941,48.35));
#79733=CARTESIAN_POINT('Origin',(149.905457080342,2.17435204982758,48.5));
#79734=CARTESIAN_POINT('',(149.905457080342,2.17435204982758,48.5));
#79735=CARTESIAN_POINT('',(149.905457080342,5.08717602491379,48.5));
#79736=CARTESIAN_POINT('',(149.905457080342,2.17435204982758,48.35));
#79737=CARTESIAN_POINT('',(149.905457080342,2.17435204982758,48.5));
#79738=CARTESIAN_POINT('',(149.905457080342,2.17435204982758,48.35));
#79739=CARTESIAN_POINT('Origin',(149.608321965672,2.17435204982758,48.5));
#79740=CARTESIAN_POINT('',(149.608321965672,2.17435204982758,48.5));
#79741=CARTESIAN_POINT('',(74.804160982836,2.17435204982758,48.5));
#79742=CARTESIAN_POINT('',(149.608321965672,2.17435204982758,48.35));
#79743=CARTESIAN_POINT('',(149.608321965672,2.17435204982758,48.5));
#79744=CARTESIAN_POINT('',(149.608321965672,2.17435204982758,48.35));
#79745=CARTESIAN_POINT('Origin',(149.608321965672,3.6000000834465,48.5));
#79746=CARTESIAN_POINT('',(149.608321965672,3.6000000834465,48.5));
#79747=CARTESIAN_POINT('',(149.608321965672,5.80000004172325,48.5));
#79748=CARTESIAN_POINT('',(149.608321965672,3.6000000834465,48.35));
#79749=CARTESIAN_POINT('',(149.608321965672,3.6000000834465,48.5));
#79750=CARTESIAN_POINT('',(149.608321965672,3.6000000834465,48.35));
#79751=CARTESIAN_POINT('Origin',(149.387721897103,3.6000000834465,48.5));
#79752=CARTESIAN_POINT('',(149.387721897103,3.6000000834465,48.5));
#79753=CARTESIAN_POINT('',(74.6938609485514,3.6000000834465,48.5));
#79754=CARTESIAN_POINT('',(149.387721897103,3.6000000834465,48.35));
#79755=CARTESIAN_POINT('',(149.387721897103,3.6000000834465,48.5));
#79756=CARTESIAN_POINT('',(149.387721897103,3.6000000834465,48.35));
#79757=CARTESIAN_POINT('Origin',(148.383765549399,2.17435204982758,48.5));
#79758=CARTESIAN_POINT('',(148.383765549399,2.17435204982758,48.5));
#79759=CARTESIAN_POINT('',(125.159520291088,-30.8047706585614,48.5));
#79760=CARTESIAN_POINT('',(148.383765549399,2.17435204982758,48.35));
#79761=CARTESIAN_POINT('',(148.383765549399,2.17435204982758,48.5));
#79762=CARTESIAN_POINT('',(148.383765549399,2.17435204982758,48.35));
#79763=CARTESIAN_POINT('Origin',(148.383765549399,1.92673945426941,48.5));
#79764=CARTESIAN_POINT('',(148.383765549399,1.92673945426941,48.5));
#79765=CARTESIAN_POINT('',(148.383765549399,4.9633697271347,48.5));
#79766=CARTESIAN_POINT('',(148.383765549399,1.92673945426941,48.35));
#79767=CARTESIAN_POINT('',(148.383765549399,1.92673945426941,48.5));
#79768=CARTESIAN_POINT('',(148.383765549399,1.92673945426941,48.35));
#79769=CARTESIAN_POINT('Origin',(149.338199377991,1.92673945426941,48.5));
#79770=CARTESIAN_POINT('',(149.338199377991,1.92673945426941,48.5));
#79771=CARTESIAN_POINT('',(74.6690996889956,1.92673945426941,48.5));
#79772=CARTESIAN_POINT('',(149.338199377991,1.92673945426941,48.35));
#79773=CARTESIAN_POINT('',(149.338199377991,1.92673945426941,48.5));
#79774=CARTESIAN_POINT('',(149.338199377991,1.92673945426941,48.35));
#79775=CARTESIAN_POINT('Origin',(149.338199377991,1.40000009536743,48.5));
#79776=CARTESIAN_POINT('',(149.338199377991,1.40000009536743,48.5));
#79777=CARTESIAN_POINT('',(149.338199377991,4.70000004768372,48.5));
#79778=CARTESIAN_POINT('',(149.338199377991,1.40000009536743,48.35));
#79779=CARTESIAN_POINT('',(149.338199377991,1.40000009536743,48.5));
#79780=CARTESIAN_POINT('',(149.338199377991,1.40000009536743,48.35));
#79781=CARTESIAN_POINT('Origin',(149.608321965672,1.40000009536743,48.5));
#79782=CARTESIAN_POINT('',(74.804160982836,1.40000009536743,48.5));
#79783=CARTESIAN_POINT('',(149.608321965672,1.40000009536743,48.35));
#79784=CARTESIAN_POINT('Origin',(149.999999956228,2.48574362695217,48.35));
#79785=CARTESIAN_POINT('Origin',(0.,8.,48.5));
#79786=CARTESIAN_POINT('Origin',(0.,8.,48.5));
#79787=CARTESIAN_POINT('Ctrl Pts',(140.850886523724,3.38540250062943,48.5));
#79788=CARTESIAN_POINT('Ctrl Pts',(140.850886523724,3.38540250062943,48.35));
#79789=CARTESIAN_POINT('Ctrl Pts',(140.664802014828,3.38540250062943,48.5));
#79790=CARTESIAN_POINT('Ctrl Pts',(140.664802014828,3.38540250062943,48.35));
#79791=CARTESIAN_POINT('Ctrl Pts',(140.553751409054,3.22783091664314,48.5));
#79792=CARTESIAN_POINT('Ctrl Pts',(140.553751409054,3.22783091664314,48.35));
#79793=CARTESIAN_POINT('',(140.850886523724,3.38540250062943,48.5));
#79794=CARTESIAN_POINT('',(140.553751409054,3.22783091664314,48.5));
#79795=CARTESIAN_POINT('Ctrl Pts',(140.850886523724,3.38540250062943,48.5));
#79796=CARTESIAN_POINT('Ctrl Pts',(140.664802014828,3.38540250062943,48.5));
#79797=CARTESIAN_POINT('Ctrl Pts',(140.553751409054,3.22783091664314,48.5));
#79798=CARTESIAN_POINT('',(140.850886523724,3.38540250062943,48.35));
#79799=CARTESIAN_POINT('',(140.850886523724,3.38540250062943,48.5));
#79800=CARTESIAN_POINT('',(140.553751409054,3.22783091664314,48.35));
#79801=CARTESIAN_POINT('Ctrl Pts',(140.850886523724,3.38540250062943,48.35));
#79802=CARTESIAN_POINT('Ctrl Pts',(140.664802014828,3.38540250062943,48.35));
#79803=CARTESIAN_POINT('Ctrl Pts',(140.553751409054,3.22783091664314,48.35));
#79804=CARTESIAN_POINT('',(140.553751409054,3.22783091664314,48.5));
#79805=CARTESIAN_POINT('Ctrl Pts',(141.166780412197,3.2068213224411,48.5));
#79806=CARTESIAN_POINT('Ctrl Pts',(141.166780412197,3.2068213224411,48.35));
#79807=CARTESIAN_POINT('Ctrl Pts',(141.03997272253,3.38540250062943,48.5));
#79808=CARTESIAN_POINT('Ctrl Pts',(141.03997272253,3.38540250062943,48.35));
#79809=CARTESIAN_POINT('Ctrl Pts',(140.850886523724,3.38540250062943,48.5));
#79810=CARTESIAN_POINT('Ctrl Pts',(140.850886523724,3.38540250062943,48.35));
#79811=CARTESIAN_POINT('',(141.166780412197,3.2068213224411,48.5));
#79812=CARTESIAN_POINT('Ctrl Pts',(141.166780412197,3.2068213224411,48.5));
#79813=CARTESIAN_POINT('Ctrl Pts',(141.03997272253,3.38540250062943,48.5));
#79814=CARTESIAN_POINT('Ctrl Pts',(140.850886523724,3.38540250062943,48.5));
#79815=CARTESIAN_POINT('',(141.166780412197,3.2068213224411,48.35));
#79816=CARTESIAN_POINT('',(141.166780412197,3.2068213224411,48.5));
#79817=CARTESIAN_POINT('Ctrl Pts',(141.166780412197,3.2068213224411,48.35));
#79818=CARTESIAN_POINT('Ctrl Pts',(141.03997272253,3.38540250062943,48.35));
#79819=CARTESIAN_POINT('Ctrl Pts',(140.850886523724,3.38540250062943,48.35));
#79820=CARTESIAN_POINT('Ctrl Pts',(141.293588101864,2.48499327898026,48.5));
#79821=CARTESIAN_POINT('Ctrl Pts',(141.293588101864,2.48499327898026,48.35));
#79822=CARTESIAN_POINT('Ctrl Pts',(141.293588101864,3.02824014425278,48.5));
#79823=CARTESIAN_POINT('Ctrl Pts',(141.293588101864,3.02824014425278,48.35));
#79824=CARTESIAN_POINT('Ctrl Pts',(141.166780412197,3.2068213224411,48.5));
#79825=CARTESIAN_POINT('Ctrl Pts',(141.166780412197,3.2068213224411,48.35));
#79826=CARTESIAN_POINT('',(141.293588101864,2.48499327898026,48.5));
#79827=CARTESIAN_POINT('Ctrl Pts',(141.293588101864,2.48499327898026,48.5));
#79828=CARTESIAN_POINT('Ctrl Pts',(141.293588101864,3.02824014425278,48.5));
#79829=CARTESIAN_POINT('Ctrl Pts',(141.166780412197,3.2068213224411,48.5));
#79830=CARTESIAN_POINT('',(141.293588101864,2.48499327898026,48.35));
#79831=CARTESIAN_POINT('',(141.293588101864,2.48499327898026,48.5));
#79832=CARTESIAN_POINT('Ctrl Pts',(141.293588101864,2.48499327898026,48.35));
#79833=CARTESIAN_POINT('Ctrl Pts',(141.293588101864,3.02824014425278,48.35));
#79834=CARTESIAN_POINT('Ctrl Pts',(141.166780412197,3.2068213224411,48.35));
#79835=CARTESIAN_POINT('Ctrl Pts',(141.166780412197,1.76466578245163,48.5));
#79836=CARTESIAN_POINT('Ctrl Pts',(141.166780412197,1.76466578245163,48.35));
#79837=CARTESIAN_POINT('Ctrl Pts',(141.293588101864,1.9447478055954,48.5));
#79838=CARTESIAN_POINT('Ctrl Pts',(141.293588101864,1.9447478055954,48.35));
#79839=CARTESIAN_POINT('Ctrl Pts',(141.293588101864,2.48499327898026,48.5));
#79840=CARTESIAN_POINT('Ctrl Pts',(141.293588101864,2.48499327898026,48.35));
#79841=CARTESIAN_POINT('',(141.166780412197,1.76466578245163,48.5));
#79842=CARTESIAN_POINT('Ctrl Pts',(141.166780412197,1.76466578245163,48.5));
#79843=CARTESIAN_POINT('Ctrl Pts',(141.293588101864,1.9447478055954,48.5));
#79844=CARTESIAN_POINT('Ctrl Pts',(141.293588101864,2.48499327898026,48.5));
#79845=CARTESIAN_POINT('',(141.166780412197,1.76466578245163,48.35));
#79846=CARTESIAN_POINT('',(141.166780412197,1.76466578245163,48.5));
#79847=CARTESIAN_POINT('Ctrl Pts',(141.166780412197,1.76466578245163,48.35));
#79848=CARTESIAN_POINT('Ctrl Pts',(141.293588101864,1.9447478055954,48.35));
#79849=CARTESIAN_POINT('Ctrl Pts',(141.293588101864,2.48499327898026,48.35));
#79850=CARTESIAN_POINT('Ctrl Pts',(140.853888213634,1.58458405733109,48.5));
#79851=CARTESIAN_POINT('Ctrl Pts',(140.853888213634,1.58458405733109,48.35));
#79852=CARTESIAN_POINT('Ctrl Pts',(141.03997272253,1.58458405733109,48.5));
#79853=CARTESIAN_POINT('Ctrl Pts',(141.03997272253,1.58458405733109,48.35));
#79854=CARTESIAN_POINT('Ctrl Pts',(141.166780412197,1.76466578245163,48.5));
#79855=CARTESIAN_POINT('Ctrl Pts',(141.166780412197,1.76466578245163,48.35));
#79856=CARTESIAN_POINT('',(140.853888213634,1.58458405733109,48.5));
#79857=CARTESIAN_POINT('Ctrl Pts',(140.853888213634,1.58458405733109,48.5));
#79858=CARTESIAN_POINT('Ctrl Pts',(141.03997272253,1.58458405733109,48.5));
#79859=CARTESIAN_POINT('Ctrl Pts',(141.166780412197,1.76466578245163,48.5));
#79860=CARTESIAN_POINT('',(140.853888213634,1.58458405733109,48.35));
#79861=CARTESIAN_POINT('',(140.853888213634,1.58458405733109,48.5));
#79862=CARTESIAN_POINT('Ctrl Pts',(140.853888213634,1.58458405733109,48.35));
#79863=CARTESIAN_POINT('Ctrl Pts',(141.03997272253,1.58458405733109,48.35));
#79864=CARTESIAN_POINT('Ctrl Pts',(141.166780412197,1.76466578245163,48.35));
#79865=CARTESIAN_POINT('Ctrl Pts',(140.540996015072,1.76391565799713,48.5));
#79866=CARTESIAN_POINT('Ctrl Pts',(140.540996015072,1.76391565799713,48.35));
#79867=CARTESIAN_POINT('Ctrl Pts',(140.667803406715,1.58458405733109,48.5));
#79868=CARTESIAN_POINT('Ctrl Pts',(140.667803406715,1.58458405733109,48.35));
#79869=CARTESIAN_POINT('Ctrl Pts',(140.853888213634,1.58458405733109,48.5));
#79870=CARTESIAN_POINT('Ctrl Pts',(140.853888213634,1.58458405733109,48.35));
#79871=CARTESIAN_POINT('',(140.540996015072,1.76391565799713,48.5));
#79872=CARTESIAN_POINT('Ctrl Pts',(140.540996015072,1.76391565799713,48.5));
#79873=CARTESIAN_POINT('Ctrl Pts',(140.667803406715,1.58458405733109,48.5));
#79874=CARTESIAN_POINT('Ctrl Pts',(140.853888213634,1.58458405733109,48.5));
#79875=CARTESIAN_POINT('',(140.540996015072,1.76391565799713,48.35));
#79876=CARTESIAN_POINT('',(140.540996015072,1.76391565799713,48.5));
#79877=CARTESIAN_POINT('Ctrl Pts',(140.540996015072,1.76391565799713,48.35));
#79878=CARTESIAN_POINT('Ctrl Pts',(140.667803406715,1.58458405733109,48.35));
#79879=CARTESIAN_POINT('Ctrl Pts',(140.853888213634,1.58458405733109,48.35));
#79880=CARTESIAN_POINT('Ctrl Pts',(140.414188325405,2.48499327898026,48.5));
#79881=CARTESIAN_POINT('Ctrl Pts',(140.414188325405,2.48499327898026,48.35));
#79882=CARTESIAN_POINT('Ctrl Pts',(140.414188325405,1.94324696063995,48.5));
#79883=CARTESIAN_POINT('Ctrl Pts',(140.414188325405,1.94324696063995,48.35));
#79884=CARTESIAN_POINT('Ctrl Pts',(140.540996015072,1.76391565799713,48.5));
#79885=CARTESIAN_POINT('Ctrl Pts',(140.540996015072,1.76391565799713,48.35));
#79886=CARTESIAN_POINT('',(140.414188325405,2.48499327898026,48.5));
#79887=CARTESIAN_POINT('Ctrl Pts',(140.414188325405,2.48499327898026,48.5));
#79888=CARTESIAN_POINT('Ctrl Pts',(140.414188325405,1.94324696063995,48.5));
#79889=CARTESIAN_POINT('Ctrl Pts',(140.540996015072,1.76391565799713,48.5));
#79890=CARTESIAN_POINT('',(140.414188325405,2.48499327898026,48.35));
#79891=CARTESIAN_POINT('',(140.414188325405,2.48499327898026,48.5));
#79892=CARTESIAN_POINT('Ctrl Pts',(140.414188325405,2.48499327898026,48.35));
#79893=CARTESIAN_POINT('Ctrl Pts',(140.414188325405,1.94324696063995,48.35));
#79894=CARTESIAN_POINT('Ctrl Pts',(140.540996015072,1.76391565799713,48.35));
#79895=CARTESIAN_POINT('Ctrl Pts',(140.553751409054,3.22783091664314,48.5));
#79896=CARTESIAN_POINT('Ctrl Pts',(140.553751409054,3.22783091664314,48.35));
#79897=CARTESIAN_POINT('Ctrl Pts',(140.414188325405,3.02673944830894,48.5));
#79898=CARTESIAN_POINT('Ctrl Pts',(140.414188325405,3.02673944830894,48.35));
#79899=CARTESIAN_POINT('Ctrl Pts',(140.414188325405,2.48499327898026,48.5));
#79900=CARTESIAN_POINT('Ctrl Pts',(140.414188325405,2.48499327898026,48.35));
#79901=CARTESIAN_POINT('Ctrl Pts',(140.553751409054,3.22783091664314,48.5));
#79902=CARTESIAN_POINT('Ctrl Pts',(140.414188325405,3.02673944830894,48.5));
#79903=CARTESIAN_POINT('Ctrl Pts',(140.414188325405,2.48499327898026,48.5));
#79904=CARTESIAN_POINT('Ctrl Pts',(140.553751409054,3.22783091664314,48.35));
#79905=CARTESIAN_POINT('Ctrl Pts',(140.414188325405,3.02673944830894,48.35));
#79906=CARTESIAN_POINT('Ctrl Pts',(140.414188325405,2.48499327898026,48.35));
#79907=CARTESIAN_POINT('Ctrl Pts',(140.853888213634,1.36248314380646,48.5));
#79908=CARTESIAN_POINT('Ctrl Pts',(140.853888213634,1.36248314380646,48.35));
#79909=CARTESIAN_POINT('Ctrl Pts',(140.535743355751,1.36248314380646,48.5));
#79910=CARTESIAN_POINT('Ctrl Pts',(140.535743355751,1.36248314380646,48.35));
#79911=CARTESIAN_POINT('Ctrl Pts',(140.354161083698,1.59058684110642,48.5));
#79912=CARTESIAN_POINT('Ctrl Pts',(140.354161083698,1.59058684110642,48.35));
#79913=CARTESIAN_POINT('',(140.853888213634,1.36248314380646,48.5));
#79914=CARTESIAN_POINT('',(140.354161083698,1.59058684110642,48.5));
#79915=CARTESIAN_POINT('Ctrl Pts',(140.853888213634,1.36248314380646,48.5));
#79916=CARTESIAN_POINT('Ctrl Pts',(140.535743355751,1.36248314380646,48.5));
#79917=CARTESIAN_POINT('Ctrl Pts',(140.354161083698,1.59058684110642,48.5));
#79918=CARTESIAN_POINT('',(140.853888213634,1.36248314380646,48.35));
#79919=CARTESIAN_POINT('',(140.853888213634,1.36248314380646,48.5));
#79920=CARTESIAN_POINT('',(140.354161083698,1.59058684110642,48.35));
#79921=CARTESIAN_POINT('Ctrl Pts',(140.853888213634,1.36248314380646,48.35));
#79922=CARTESIAN_POINT('Ctrl Pts',(140.535743355751,1.36248314380646,48.35));
#79923=CARTESIAN_POINT('Ctrl Pts',(140.354161083698,1.59058684110642,48.35));
#79924=CARTESIAN_POINT('',(140.354161083698,1.59058684110642,48.5));
#79925=CARTESIAN_POINT('Ctrl Pts',(141.25381988287,1.49229192733765,48.5));
#79926=CARTESIAN_POINT('Ctrl Pts',(141.25381988287,1.49229192733765,48.35));
#79927=CARTESIAN_POINT('Ctrl Pts',(141.095498025417,1.36248314380646,48.5));
#79928=CARTESIAN_POINT('Ctrl Pts',(141.095498025417,1.36248314380646,48.35));
#79929=CARTESIAN_POINT('Ctrl Pts',(140.853888213634,1.36248314380646,48.5));
#79930=CARTESIAN_POINT('Ctrl Pts',(140.853888213634,1.36248314380646,48.35));
#79931=CARTESIAN_POINT('',(141.25381988287,1.49229192733765,48.5));
#79932=CARTESIAN_POINT('Ctrl Pts',(141.25381988287,1.49229192733765,48.5));
#79933=CARTESIAN_POINT('Ctrl Pts',(141.095498025417,1.36248314380646,48.5));
#79934=CARTESIAN_POINT('Ctrl Pts',(140.853888213634,1.36248314380646,48.5));
#79935=CARTESIAN_POINT('',(141.25381988287,1.49229192733765,48.35));
#79936=CARTESIAN_POINT('',(141.25381988287,1.49229192733765,48.5));
#79937=CARTESIAN_POINT('Ctrl Pts',(141.25381988287,1.49229192733765,48.35));
#79938=CARTESIAN_POINT('Ctrl Pts',(141.095498025417,1.36248314380646,48.35));
#79939=CARTESIAN_POINT('Ctrl Pts',(140.853888213634,1.36248314380646,48.35));
#79940=CARTESIAN_POINT('Ctrl Pts',(141.49167817831,1.85995900630951,48.5));
#79941=CARTESIAN_POINT('Ctrl Pts',(141.49167817831,1.85995900630951,48.35));
#79942=CARTESIAN_POINT('Ctrl Pts',(141.412141740322,1.62210100889206,48.5));
#79943=CARTESIAN_POINT('Ctrl Pts',(141.412141740322,1.62210100889206,48.35));
#79944=CARTESIAN_POINT('Ctrl Pts',(141.25381988287,1.49229192733765,48.5));
#79945=CARTESIAN_POINT('Ctrl Pts',(141.25381988287,1.49229192733765,48.35));
#79946=CARTESIAN_POINT('',(141.49167817831,1.85995900630951,48.5));
#79947=CARTESIAN_POINT('Ctrl Pts',(141.49167817831,1.85995900630951,48.5));
#79948=CARTESIAN_POINT('Ctrl Pts',(141.412141740322,1.62210100889206,48.5));
#79949=CARTESIAN_POINT('Ctrl Pts',(141.25381988287,1.49229192733765,48.5));
#79950=CARTESIAN_POINT('',(141.49167817831,1.85995900630951,48.35));
#79951=CARTESIAN_POINT('',(141.49167817831,1.85995900630951,48.5));
#79952=CARTESIAN_POINT('Ctrl Pts',(141.49167817831,1.85995900630951,48.35));
#79953=CARTESIAN_POINT('Ctrl Pts',(141.412141740322,1.62210100889206,48.35));
#79954=CARTESIAN_POINT('Ctrl Pts',(141.25381988287,1.49229192733765,48.35));
#79955=CARTESIAN_POINT('Ctrl Pts',(141.571214020252,2.48499327898026,48.5));
#79956=CARTESIAN_POINT('Ctrl Pts',(141.571214020252,2.48499327898026,48.35));
#79957=CARTESIAN_POINT('Ctrl Pts',(141.571214020252,2.09781730175018,48.5));
#79958=CARTESIAN_POINT('Ctrl Pts',(141.571214020252,2.09781730175018,48.35));
#79959=CARTESIAN_POINT('Ctrl Pts',(141.49167817831,1.85995900630951,48.5));
#79960=CARTESIAN_POINT('Ctrl Pts',(141.49167817831,1.85995900630951,48.35));
#79961=CARTESIAN_POINT('',(141.571214020252,2.48499327898026,48.5));
#79962=CARTESIAN_POINT('Ctrl Pts',(141.571214020252,2.48499327898026,48.5));
#79963=CARTESIAN_POINT('Ctrl Pts',(141.571214020252,2.09781730175018,48.5));
#79964=CARTESIAN_POINT('Ctrl Pts',(141.49167817831,1.85995900630951,48.5));
#79965=CARTESIAN_POINT('',(141.571214020252,2.48499327898026,48.35));
#79966=CARTESIAN_POINT('',(141.571214020252,2.48499327898026,48.5));
#79967=CARTESIAN_POINT('Ctrl Pts',(141.571214020252,2.48499327898026,48.35));
#79968=CARTESIAN_POINT('Ctrl Pts',(141.571214020252,2.09781730175018,48.35));
#79969=CARTESIAN_POINT('Ctrl Pts',(141.49167817831,1.85995900630951,48.35));
#79970=CARTESIAN_POINT('Ctrl Pts',(141.521691501141,3.00497958064079,48.5));
#79971=CARTESIAN_POINT('Ctrl Pts',(141.521691501141,3.00497958064079,48.35));
#79972=CARTESIAN_POINT('Ctrl Pts',(141.571214020252,2.81214186549187,48.5));
#79973=CARTESIAN_POINT('Ctrl Pts',(141.571214020252,2.81214186549187,48.35));
#79974=CARTESIAN_POINT('Ctrl Pts',(141.571214020252,2.48499327898026,48.5));
#79975=CARTESIAN_POINT('Ctrl Pts',(141.571214020252,2.48499327898026,48.35));
#79976=CARTESIAN_POINT('',(141.521691501141,3.00497958064079,48.5));
#79977=CARTESIAN_POINT('Ctrl Pts',(141.521691501141,3.00497958064079,48.5));
#79978=CARTESIAN_POINT('Ctrl Pts',(141.571214020252,2.81214186549187,48.5));
#79979=CARTESIAN_POINT('Ctrl Pts',(141.571214020252,2.48499327898026,48.5));
#79980=CARTESIAN_POINT('',(141.521691501141,3.00497958064079,48.35));
#79981=CARTESIAN_POINT('',(141.521691501141,3.00497958064079,48.5));
#79982=CARTESIAN_POINT('Ctrl Pts',(141.521691501141,3.00497958064079,48.35));
#79983=CARTESIAN_POINT('Ctrl Pts',(141.571214020252,2.81214186549187,48.35));
#79984=CARTESIAN_POINT('Ctrl Pts',(141.571214020252,2.48499327898026,48.35));
#79985=CARTESIAN_POINT('Ctrl Pts',(141.385129511356,3.33212831616402,48.5));
#79986=CARTESIAN_POINT('Ctrl Pts',(141.385129511356,3.33212831616402,48.35));
#79987=CARTESIAN_POINT('Ctrl Pts',(141.472168982029,3.19781729578972,48.5));
#79988=CARTESIAN_POINT('Ctrl Pts',(141.472168982029,3.19781729578972,48.35));
#79989=CARTESIAN_POINT('Ctrl Pts',(141.521691501141,3.00497958064079,48.5));
#79990=CARTESIAN_POINT('Ctrl Pts',(141.521691501141,3.00497958064079,48.35));
#79991=CARTESIAN_POINT('',(141.385129511356,3.33212831616402,48.5));
#79992=CARTESIAN_POINT('Ctrl Pts',(141.385129511356,3.33212831616402,48.5));
#79993=CARTESIAN_POINT('Ctrl Pts',(141.472168982029,3.19781729578972,48.5));
#79994=CARTESIAN_POINT('Ctrl Pts',(141.521691501141,3.00497958064079,48.5));
#79995=CARTESIAN_POINT('',(141.385129511356,3.33212831616402,48.35));
#79996=CARTESIAN_POINT('',(141.385129511356,3.33212831616402,48.5));
#79997=CARTESIAN_POINT('Ctrl Pts',(141.385129511356,3.33212831616402,48.35));
#79998=CARTESIAN_POINT('Ctrl Pts',(141.472168982029,3.19781729578972,48.35));
#79999=CARTESIAN_POINT('Ctrl Pts',(141.521691501141,3.00497958064079,48.35));
#80000=CARTESIAN_POINT('Ctrl Pts',(141.164529144764,3.5377217233181,48.5));
#80001=CARTESIAN_POINT('Ctrl Pts',(141.164529144764,3.5377217233181,48.35));
#80002=CARTESIAN_POINT('Ctrl Pts',(141.298090040684,3.46643933653831,48.5));
#80003=CARTESIAN_POINT('Ctrl Pts',(141.298090040684,3.46643933653831,48.35));
#80004=CARTESIAN_POINT('Ctrl Pts',(141.385129511356,3.33212831616402,48.5));
#80005=CARTESIAN_POINT('Ctrl Pts',(141.385129511356,3.33212831616402,48.35));
#80006=CARTESIAN_POINT('',(141.164529144764,3.5377217233181,48.5));
#80007=CARTESIAN_POINT('Ctrl Pts',(141.164529144764,3.5377217233181,48.5));
#80008=CARTESIAN_POINT('Ctrl Pts',(141.298090040684,3.46643933653831,48.5));
#80009=CARTESIAN_POINT('Ctrl Pts',(141.385129511356,3.33212831616402,48.5));
#80010=CARTESIAN_POINT('',(141.164529144764,3.5377217233181,48.35));
#80011=CARTESIAN_POINT('',(141.164529144764,3.5377217233181,48.5));
#80012=CARTESIAN_POINT('Ctrl Pts',(141.164529144764,3.5377217233181,48.35));
#80013=CARTESIAN_POINT('Ctrl Pts',(141.298090040684,3.46643933653831,48.35));
#80014=CARTESIAN_POINT('Ctrl Pts',(141.385129511356,3.33212831616402,48.35));
#80015=CARTESIAN_POINT('Ctrl Pts',(140.853888213634,3.60900411009789,48.5));
#80016=CARTESIAN_POINT('Ctrl Pts',(140.853888213634,3.60900411009789,48.35));
#80017=CARTESIAN_POINT('Ctrl Pts',(141.030968248844,3.60900411009789,48.5));
#80018=CARTESIAN_POINT('Ctrl Pts',(141.030968248844,3.60900411009789,48.35));
#80019=CARTESIAN_POINT('Ctrl Pts',(141.164529144764,3.5377217233181,48.5));
#80020=CARTESIAN_POINT('Ctrl Pts',(141.164529144764,3.5377217233181,48.35));
#80021=CARTESIAN_POINT('',(140.853888213634,3.60900411009789,48.5));
#80022=CARTESIAN_POINT('Ctrl Pts',(140.853888213634,3.60900411009789,48.5));
#80023=CARTESIAN_POINT('Ctrl Pts',(141.030968248844,3.60900411009789,48.5));
#80024=CARTESIAN_POINT('Ctrl Pts',(141.164529144764,3.5377217233181,48.5));
#80025=CARTESIAN_POINT('',(140.853888213634,3.60900411009789,48.35));
#80026=CARTESIAN_POINT('',(140.853888213634,3.60900411009789,48.5));
#80027=CARTESIAN_POINT('Ctrl Pts',(140.853888213634,3.60900411009789,48.35));
#80028=CARTESIAN_POINT('Ctrl Pts',(141.030968248844,3.60900411009789,48.35));
#80029=CARTESIAN_POINT('Ctrl Pts',(141.164529144764,3.5377217233181,48.35));
#80030=CARTESIAN_POINT('Ctrl Pts',(140.455456793308,3.47994545102119,48.5));
#80031=CARTESIAN_POINT('Ctrl Pts',(140.455456793308,3.47994545102119,48.35));
#80032=CARTESIAN_POINT('Ctrl Pts',(140.613778650761,3.60900411009789,48.5));
#80033=CARTESIAN_POINT('Ctrl Pts',(140.613778650761,3.60900411009789,48.35));
#80034=CARTESIAN_POINT('Ctrl Pts',(140.853888213634,3.60900411009789,48.5));
#80035=CARTESIAN_POINT('Ctrl Pts',(140.853888213634,3.60900411009789,48.35));
#80036=CARTESIAN_POINT('',(140.455456793308,3.47994545102119,48.5));
#80037=CARTESIAN_POINT('Ctrl Pts',(140.455456793308,3.47994545102119,48.5));
#80038=CARTESIAN_POINT('Ctrl Pts',(140.613778650761,3.60900411009789,48.5));
#80039=CARTESIAN_POINT('Ctrl Pts',(140.853888213634,3.60900411009789,48.5));
#80040=CARTESIAN_POINT('',(140.455456793308,3.47994545102119,48.35));
#80041=CARTESIAN_POINT('',(140.455456793308,3.47994545102119,48.5));
#80042=CARTESIAN_POINT('Ctrl Pts',(140.455456793308,3.47994545102119,48.35));
#80043=CARTESIAN_POINT('Ctrl Pts',(140.613778650761,3.60900411009789,48.35));
#80044=CARTESIAN_POINT('Ctrl Pts',(140.853888213634,3.60900411009789,48.35));
#80045=CARTESIAN_POINT('Ctrl Pts',(140.216848671436,3.11302864551544,48.5));
#80046=CARTESIAN_POINT('Ctrl Pts',(140.216848671436,3.11302864551544,48.35));
#80047=CARTESIAN_POINT('Ctrl Pts',(140.297134935856,3.3508867919445,48.5));
#80048=CARTESIAN_POINT('Ctrl Pts',(140.297134935856,3.3508867919445,48.35));
#80049=CARTESIAN_POINT('Ctrl Pts',(140.455456793308,3.47994545102119,48.5));
#80050=CARTESIAN_POINT('Ctrl Pts',(140.455456793308,3.47994545102119,48.35));
#80051=CARTESIAN_POINT('',(140.216848671436,3.11302864551544,48.5));
#80052=CARTESIAN_POINT('Ctrl Pts',(140.216848671436,3.11302864551544,48.5));
#80053=CARTESIAN_POINT('Ctrl Pts',(140.297134935856,3.3508867919445,48.5));
#80054=CARTESIAN_POINT('Ctrl Pts',(140.455456793308,3.47994545102119,48.5));
#80055=CARTESIAN_POINT('',(140.216848671436,3.11302864551544,48.35));
#80056=CARTESIAN_POINT('',(140.216848671436,3.11302864551544,48.5));
#80057=CARTESIAN_POINT('Ctrl Pts',(140.216848671436,3.11302864551544,48.35));
#80058=CARTESIAN_POINT('Ctrl Pts',(140.297134935856,3.3508867919445,48.35));
#80059=CARTESIAN_POINT('Ctrl Pts',(140.455456793308,3.47994545102119,48.35));
#80060=CARTESIAN_POINT('Ctrl Pts',(140.13656181097,2.48499327898026,48.5));
#80061=CARTESIAN_POINT('Ctrl Pts',(140.13656181097,2.48499327898026,48.35));
#80062=CARTESIAN_POINT('Ctrl Pts',(140.13656181097,2.87517049908638,48.5));
#80063=CARTESIAN_POINT('Ctrl Pts',(140.13656181097,2.87517049908638,48.35));
#80064=CARTESIAN_POINT('Ctrl Pts',(140.216848671436,3.11302864551544,48.5));
#80065=CARTESIAN_POINT('Ctrl Pts',(140.216848671436,3.11302864551544,48.35));
#80066=CARTESIAN_POINT('',(140.13656181097,2.48499327898026,48.5));
#80067=CARTESIAN_POINT('Ctrl Pts',(140.13656181097,2.48499327898026,48.5));
#80068=CARTESIAN_POINT('Ctrl Pts',(140.13656181097,2.87517049908638,48.5));
#80069=CARTESIAN_POINT('Ctrl Pts',(140.216848671436,3.11302864551544,48.5));
#80070=CARTESIAN_POINT('',(140.13656181097,2.48499327898026,48.35));
#80071=CARTESIAN_POINT('',(140.13656181097,2.48499327898026,48.5));
#80072=CARTESIAN_POINT('Ctrl Pts',(140.13656181097,2.48499327898026,48.35));
#80073=CARTESIAN_POINT('Ctrl Pts',(140.13656181097,2.87517049908638,48.35));
#80074=CARTESIAN_POINT('Ctrl Pts',(140.216848671436,3.11302864551544,48.35));
#80075=CARTESIAN_POINT('Ctrl Pts',(140.354161083698,1.59058684110642,48.5));
#80076=CARTESIAN_POINT('Ctrl Pts',(140.354161083698,1.59058684110642,48.35));
#80077=CARTESIAN_POINT('Ctrl Pts',(140.13656181097,1.86521166563034,48.5));
#80078=CARTESIAN_POINT('Ctrl Pts',(140.13656181097,1.86521166563034,48.35));
#80079=CARTESIAN_POINT('Ctrl Pts',(140.13656181097,2.48499327898026,48.5));
#80080=CARTESIAN_POINT('Ctrl Pts',(140.13656181097,2.48499327898026,48.35));
#80081=CARTESIAN_POINT('Ctrl Pts',(140.354161083698,1.59058684110642,48.5));
#80082=CARTESIAN_POINT('Ctrl Pts',(140.13656181097,1.86521166563034,48.5));
#80083=CARTESIAN_POINT('Ctrl Pts',(140.13656181097,2.48499327898026,48.5));
#80084=CARTESIAN_POINT('Ctrl Pts',(140.354161083698,1.59058684110642,48.35));
#80085=CARTESIAN_POINT('Ctrl Pts',(140.13656181097,1.86521166563034,48.35));
#80086=CARTESIAN_POINT('Ctrl Pts',(140.13656181097,2.48499327898026,48.35));
#80087=CARTESIAN_POINT('Origin',(139.999999895692,2.48499320447445,48.35));
#80088=CARTESIAN_POINT('Ctrl Pts',(139.128103673458,1.36098229885101,48.5));
#80089=CARTESIAN_POINT('Ctrl Pts',(139.128103673458,1.36098229885101,48.35));
#80090=CARTESIAN_POINT('Ctrl Pts',(138.838472038507,1.36098229885101,48.5));
#80091=CARTESIAN_POINT('Ctrl Pts',(138.838472038507,1.36098229885101,48.35));
#80092=CARTESIAN_POINT('Ctrl Pts',(138.647135019302,1.53356069326401,48.5));
#80093=CARTESIAN_POINT('Ctrl Pts',(138.647135019302,1.53356069326401,48.35));
#80094=CARTESIAN_POINT('',(139.128103673458,1.36098229885101,48.5));
#80095=CARTESIAN_POINT('',(138.647135019302,1.53356069326401,48.5));
#80096=CARTESIAN_POINT('Ctrl Pts',(139.128103673458,1.36098229885101,48.5));
#80097=CARTESIAN_POINT('Ctrl Pts',(138.838472038507,1.36098229885101,48.5));
#80098=CARTESIAN_POINT('Ctrl Pts',(138.647135019302,1.53356069326401,48.5));
#80099=CARTESIAN_POINT('',(139.128103673458,1.36098229885101,48.35));
#80100=CARTESIAN_POINT('',(139.128103673458,1.36098229885101,48.5));
#80101=CARTESIAN_POINT('',(138.647135019302,1.53356069326401,48.35));
#80102=CARTESIAN_POINT('Ctrl Pts',(139.128103673458,1.36098229885101,48.35));
#80103=CARTESIAN_POINT('Ctrl Pts',(138.838472038507,1.36098229885101,48.35));
#80104=CARTESIAN_POINT('Ctrl Pts',(138.647135019302,1.53356069326401,48.35));
#80105=CARTESIAN_POINT('',(138.647135019302,1.53356069326401,48.5));
#80106=CARTESIAN_POINT('Ctrl Pts',(139.65934497118,1.56132334470749,48.5));
#80107=CARTESIAN_POINT('Ctrl Pts',(139.65934497118,1.56132334470749,48.35));
#80108=CARTESIAN_POINT('Ctrl Pts',(139.449249625206,1.36098229885101,48.5));
#80109=CARTESIAN_POINT('Ctrl Pts',(139.449249625206,1.36098229885101,48.35));
#80110=CARTESIAN_POINT('Ctrl Pts',(139.128103673458,1.36098229885101,48.5));
#80111=CARTESIAN_POINT('Ctrl Pts',(139.128103673458,1.36098229885101,48.35));
#80112=CARTESIAN_POINT('',(139.65934497118,1.56132334470749,48.5));
#80113=CARTESIAN_POINT('Ctrl Pts',(139.65934497118,1.56132334470749,48.5));
#80114=CARTESIAN_POINT('Ctrl Pts',(139.449249625206,1.36098229885101,48.5));
#80115=CARTESIAN_POINT('Ctrl Pts',(139.128103673458,1.36098229885101,48.5));
#80116=CARTESIAN_POINT('',(139.65934497118,1.56132334470749,48.35));
#80117=CARTESIAN_POINT('',(139.65934497118,1.56132334470749,48.5));
#80118=CARTESIAN_POINT('Ctrl Pts',(139.65934497118,1.56132334470749,48.35));
#80119=CARTESIAN_POINT('Ctrl Pts',(139.449249625206,1.36098229885101,48.35));
#80120=CARTESIAN_POINT('Ctrl Pts',(139.128103673458,1.36098229885101,48.35));
#80121=CARTESIAN_POINT('Ctrl Pts',(139.869440615177,2.04979562759399,48.5));
#80122=CARTESIAN_POINT('Ctrl Pts',(139.869440615177,2.04979562759399,48.35));
#80123=CARTESIAN_POINT('Ctrl Pts',(139.869440615177,1.76166439056397,48.5));
#80124=CARTESIAN_POINT('Ctrl Pts',(139.869440615177,1.76166439056397,48.35));
#80125=CARTESIAN_POINT('Ctrl Pts',(139.65934497118,1.56132334470749,48.5));
#80126=CARTESIAN_POINT('Ctrl Pts',(139.65934497118,1.56132334470749,48.35));
#80127=CARTESIAN_POINT('',(139.869440615177,2.04979562759399,48.5));
#80128=CARTESIAN_POINT('Ctrl Pts',(139.869440615177,2.04979562759399,48.5));
#80129=CARTESIAN_POINT('Ctrl Pts',(139.869440615177,1.76166439056397,48.5));
#80130=CARTESIAN_POINT('Ctrl Pts',(139.65934497118,1.56132334470749,48.5));
#80131=CARTESIAN_POINT('',(139.869440615177,2.04979562759399,48.35));
#80132=CARTESIAN_POINT('',(139.869440615177,2.04979562759399,48.5));
#80133=CARTESIAN_POINT('Ctrl Pts',(139.869440615177,2.04979562759399,48.35));
#80134=CARTESIAN_POINT('Ctrl Pts',(139.869440615177,1.76166439056397,48.35));
#80135=CARTESIAN_POINT('Ctrl Pts',(139.65934497118,1.56132334470749,48.35));
#80136=CARTESIAN_POINT('Ctrl Pts',(139.761391699314,2.40470671653748,48.5));
#80137=CARTESIAN_POINT('Ctrl Pts',(139.761391699314,2.40470671653748,48.35));
#80138=CARTESIAN_POINT('Ctrl Pts',(139.869440615177,2.26289236545563,48.5));
#80139=CARTESIAN_POINT('Ctrl Pts',(139.869440615177,2.26289236545563,48.35));
#80140=CARTESIAN_POINT('Ctrl Pts',(139.869440615177,2.04979562759399,48.5));
#80141=CARTESIAN_POINT('Ctrl Pts',(139.869440615177,2.04979562759399,48.35));
#80142=CARTESIAN_POINT('',(139.761391699314,2.40470671653748,48.5));
#80143=CARTESIAN_POINT('Ctrl Pts',(139.761391699314,2.40470671653748,48.5));
#80144=CARTESIAN_POINT('Ctrl Pts',(139.869440615177,2.26289236545563,48.5));
#80145=CARTESIAN_POINT('Ctrl Pts',(139.869440615177,2.04979562759399,48.5));
#80146=CARTESIAN_POINT('',(139.761391699314,2.40470671653748,48.35));
#80147=CARTESIAN_POINT('',(139.761391699314,2.40470671653748,48.5));
#80148=CARTESIAN_POINT('Ctrl Pts',(139.761391699314,2.40470671653748,48.35));
#80149=CARTESIAN_POINT('Ctrl Pts',(139.869440615177,2.26289236545563,48.35));
#80150=CARTESIAN_POINT('Ctrl Pts',(139.869440615177,2.04979562759399,48.35));
#80151=CARTESIAN_POINT('Ctrl Pts',(139.458253800869,2.59154164791107,48.5));
#80152=CARTESIAN_POINT('Ctrl Pts',(139.458253800869,2.59154164791107,48.35));
#80153=CARTESIAN_POINT('Ctrl Pts',(139.653342187405,2.54652121663094,48.5));
#80154=CARTESIAN_POINT('Ctrl Pts',(139.653342187405,2.54652121663094,48.35));
#80155=CARTESIAN_POINT('Ctrl Pts',(139.761391699314,2.40470671653748,48.5));
#80156=CARTESIAN_POINT('Ctrl Pts',(139.761391699314,2.40470671653748,48.35));
#80157=CARTESIAN_POINT('',(139.458253800869,2.59154164791107,48.5));
#80158=CARTESIAN_POINT('Ctrl Pts',(139.458253800869,2.59154164791107,48.5));
#80159=CARTESIAN_POINT('Ctrl Pts',(139.653342187405,2.54652121663094,48.5));
#80160=CARTESIAN_POINT('Ctrl Pts',(139.761391699314,2.40470671653748,48.5));
#80161=CARTESIAN_POINT('',(139.458253800869,2.59154164791107,48.35));
#80162=CARTESIAN_POINT('',(139.458253800869,2.59154164791107,48.5));
#80163=CARTESIAN_POINT('Ctrl Pts',(139.458253800869,2.59154164791107,48.35));
#80164=CARTESIAN_POINT('Ctrl Pts',(139.653342187405,2.54652121663094,48.35));
#80165=CARTESIAN_POINT('Ctrl Pts',(139.761391699314,2.40470671653748,48.35));
#80166=CARTESIAN_POINT('Ctrl Pts',(139.684856653214,2.77762615680695,48.5));
#80167=CARTESIAN_POINT('Ctrl Pts',(139.684856653214,2.77762615680695,48.35));
#80168=CARTESIAN_POINT('Ctrl Pts',(139.608321905136,2.66057306528091,48.5));
#80169=CARTESIAN_POINT('Ctrl Pts',(139.608321905136,2.66057306528091,48.35));
#80170=CARTESIAN_POINT('Ctrl Pts',(139.458253800869,2.59154164791107,48.5));
#80171=CARTESIAN_POINT('Ctrl Pts',(139.458253800869,2.59154164791107,48.35));
#80172=CARTESIAN_POINT('',(139.684856653214,2.77762615680695,48.5));
#80173=CARTESIAN_POINT('Ctrl Pts',(139.684856653214,2.77762615680695,48.5));
#80174=CARTESIAN_POINT('Ctrl Pts',(139.608321905136,2.66057306528091,48.5));
#80175=CARTESIAN_POINT('Ctrl Pts',(139.458253800869,2.59154164791107,48.5));
#80176=CARTESIAN_POINT('',(139.684856653214,2.77762615680695,48.35));
#80177=CARTESIAN_POINT('',(139.684856653214,2.77762615680695,48.5));
#80178=CARTESIAN_POINT('Ctrl Pts',(139.684856653214,2.77762615680695,48.35));
#80179=CARTESIAN_POINT('Ctrl Pts',(139.608321905136,2.66057306528091,48.35));
#80180=CARTESIAN_POINT('Ctrl Pts',(139.458253800869,2.59154164791107,48.35));
#80181=CARTESIAN_POINT('Ctrl Pts',(139.761391699314,3.03724417090416,48.5));
#80182=CARTESIAN_POINT('Ctrl Pts',(139.761391699314,3.03724417090416,48.35));
#80183=CARTESIAN_POINT('Ctrl Pts',(139.761391699314,2.89467939734459,48.5));
#80184=CARTESIAN_POINT('Ctrl Pts',(139.761391699314,2.89467939734459,48.35));
#80185=CARTESIAN_POINT('Ctrl Pts',(139.684856653214,2.77762615680695,48.5));
#80186=CARTESIAN_POINT('Ctrl Pts',(139.684856653214,2.77762615680695,48.35));
#80187=CARTESIAN_POINT('',(139.761391699314,3.03724417090416,48.5));
#80188=CARTESIAN_POINT('Ctrl Pts',(139.761391699314,3.03724417090416,48.5));
#80189=CARTESIAN_POINT('Ctrl Pts',(139.761391699314,2.89467939734459,48.5));
#80190=CARTESIAN_POINT('Ctrl Pts',(139.684856653214,2.77762615680695,48.5));
#80191=CARTESIAN_POINT('',(139.761391699314,3.03724417090416,48.35));
#80192=CARTESIAN_POINT('',(139.761391699314,3.03724417090416,48.5));
#80193=CARTESIAN_POINT('Ctrl Pts',(139.761391699314,3.03724417090416,48.35));
#80194=CARTESIAN_POINT('Ctrl Pts',(139.761391699314,2.89467939734459,48.35));
#80195=CARTESIAN_POINT('Ctrl Pts',(139.684856653214,2.77762615680695,48.35));
#80196=CARTESIAN_POINT('Ctrl Pts',(139.681104838848,3.32087317109108,48.5));
#80197=CARTESIAN_POINT('Ctrl Pts',(139.681104838848,3.32087317109108,48.35));
#80198=CARTESIAN_POINT('Ctrl Pts',(139.761391699314,3.18731242418289,48.5));
#80199=CARTESIAN_POINT('Ctrl Pts',(139.761391699314,3.18731242418289,48.35));
#80200=CARTESIAN_POINT('Ctrl Pts',(139.761391699314,3.03724417090416,48.5));
#80201=CARTESIAN_POINT('Ctrl Pts',(139.761391699314,3.03724417090416,48.35));
#80202=CARTESIAN_POINT('',(139.681104838848,3.32087317109108,48.5));
#80203=CARTESIAN_POINT('Ctrl Pts',(139.681104838848,3.32087317109108,48.5));
#80204=CARTESIAN_POINT('Ctrl Pts',(139.761391699314,3.18731242418289,48.5));
#80205=CARTESIAN_POINT('Ctrl Pts',(139.761391699314,3.03724417090416,48.5));
#80206=CARTESIAN_POINT('',(139.681104838848,3.32087317109108,48.35));
#80207=CARTESIAN_POINT('',(139.681104838848,3.32087317109108,48.5));
#80208=CARTESIAN_POINT('Ctrl Pts',(139.681104838848,3.32087317109108,48.35));
#80209=CARTESIAN_POINT('Ctrl Pts',(139.761391699314,3.18731242418289,48.35));
#80210=CARTESIAN_POINT('Ctrl Pts',(139.761391699314,3.03724417090416,48.35));
#80211=CARTESIAN_POINT('Ctrl Pts',(139.449249625206,3.53171893954277,48.5));
#80212=CARTESIAN_POINT('Ctrl Pts',(139.449249625206,3.53171893954277,48.35));
#80213=CARTESIAN_POINT('Ctrl Pts',(139.600818574429,3.45443391799927,48.5));
#80214=CARTESIAN_POINT('Ctrl Pts',(139.600818574429,3.45443391799927,48.35));
#80215=CARTESIAN_POINT('Ctrl Pts',(139.681104838848,3.32087317109108,48.5));
#80216=CARTESIAN_POINT('Ctrl Pts',(139.681104838848,3.32087317109108,48.35));
#80217=CARTESIAN_POINT('',(139.449249625206,3.53171893954277,48.5));
#80218=CARTESIAN_POINT('Ctrl Pts',(139.449249625206,3.53171893954277,48.5));
#80219=CARTESIAN_POINT('Ctrl Pts',(139.600818574429,3.45443391799927,48.5));
#80220=CARTESIAN_POINT('Ctrl Pts',(139.681104838848,3.32087317109108,48.5));
#80221=CARTESIAN_POINT('',(139.449249625206,3.53171893954277,48.35));
#80222=CARTESIAN_POINT('',(139.449249625206,3.53171893954277,48.5));
#80223=CARTESIAN_POINT('Ctrl Pts',(139.449249625206,3.53171893954277,48.35));
#80224=CARTESIAN_POINT('Ctrl Pts',(139.600818574429,3.45443391799927,48.35));
#80225=CARTESIAN_POINT('Ctrl Pts',(139.681104838848,3.32087317109108,48.35));
#80226=CARTESIAN_POINT('Ctrl Pts',(139.117598950863,3.60900411009789,48.5));
#80227=CARTESIAN_POINT('Ctrl Pts',(139.117598950863,3.60900411009789,48.35));
#80228=CARTESIAN_POINT('Ctrl Pts',(139.297680675983,3.60900411009789,48.5));
#80229=CARTESIAN_POINT('Ctrl Pts',(139.297680675983,3.60900411009789,48.35));
#80230=CARTESIAN_POINT('Ctrl Pts',(139.449249625206,3.53171893954277,48.5));
#80231=CARTESIAN_POINT('Ctrl Pts',(139.449249625206,3.53171893954277,48.35));
#80232=CARTESIAN_POINT('',(139.117598950863,3.60900411009789,48.5));
#80233=CARTESIAN_POINT('Ctrl Pts',(139.117598950863,3.60900411009789,48.5));
#80234=CARTESIAN_POINT('Ctrl Pts',(139.297680675983,3.60900411009789,48.5));
#80235=CARTESIAN_POINT('Ctrl Pts',(139.449249625206,3.53171893954277,48.5));
#80236=CARTESIAN_POINT('',(139.117598950863,3.60900411009789,48.35));
#80237=CARTESIAN_POINT('',(139.117598950863,3.60900411009789,48.5));
#80238=CARTESIAN_POINT('Ctrl Pts',(139.117598950863,3.60900411009789,48.35));
#80239=CARTESIAN_POINT('Ctrl Pts',(139.297680675983,3.60900411009789,48.35));
#80240=CARTESIAN_POINT('Ctrl Pts',(139.449249625206,3.53171893954277,48.35));
#80241=CARTESIAN_POINT('Ctrl Pts',(138.680900454521,3.45968627929688,48.5));
#80242=CARTESIAN_POINT('Ctrl Pts',(138.680900454521,3.45968627929688,48.35));
#80243=CARTESIAN_POINT('Ctrl Pts',(138.856480240822,3.60900411009789,48.5));
#80244=CARTESIAN_POINT('Ctrl Pts',(138.856480240822,3.60900411009789,48.35));
#80245=CARTESIAN_POINT('Ctrl Pts',(139.117598950863,3.60900411009789,48.5));
#80246=CARTESIAN_POINT('Ctrl Pts',(139.117598950863,3.60900411009789,48.35));
#80247=CARTESIAN_POINT('',(138.680900454521,3.45968627929688,48.5));
#80248=CARTESIAN_POINT('Ctrl Pts',(138.680900454521,3.45968627929688,48.5));
#80249=CARTESIAN_POINT('Ctrl Pts',(138.856480240822,3.60900411009789,48.5));
#80250=CARTESIAN_POINT('Ctrl Pts',(139.117598950863,3.60900411009789,48.5));
#80251=CARTESIAN_POINT('',(138.680900454521,3.45968627929688,48.35));
#80252=CARTESIAN_POINT('',(138.680900454521,3.45968627929688,48.5));
#80253=CARTESIAN_POINT('Ctrl Pts',(138.680900454521,3.45968627929688,48.35));
#80254=CARTESIAN_POINT('Ctrl Pts',(138.856480240822,3.60900411009789,48.35));
#80255=CARTESIAN_POINT('Ctrl Pts',(139.117598950863,3.60900411009789,48.35));
#80256=CARTESIAN_POINT('Ctrl Pts',(138.455798000097,3.03874486684799,48.5));
#80257=CARTESIAN_POINT('Ctrl Pts',(138.455798000097,3.03874486684799,48.35));
#80258=CARTESIAN_POINT('Ctrl Pts',(138.505320519209,3.31036829948425,48.5));
#80259=CARTESIAN_POINT('Ctrl Pts',(138.505320519209,3.31036829948425,48.35));
#80260=CARTESIAN_POINT('Ctrl Pts',(138.680900454521,3.45968627929688,48.5));
#80261=CARTESIAN_POINT('Ctrl Pts',(138.680900454521,3.45968627929688,48.35));
#80262=CARTESIAN_POINT('',(138.455798000097,3.03874486684799,48.5));
#80263=CARTESIAN_POINT('Ctrl Pts',(138.455798000097,3.03874486684799,48.5));
#80264=CARTESIAN_POINT('Ctrl Pts',(138.505320519209,3.31036829948425,48.5));
#80265=CARTESIAN_POINT('Ctrl Pts',(138.680900454521,3.45968627929688,48.5));
#80266=CARTESIAN_POINT('',(138.455798000097,3.03874486684799,48.35));
#80267=CARTESIAN_POINT('',(138.455798000097,3.03874486684799,48.5));
#80268=CARTESIAN_POINT('Ctrl Pts',(138.455798000097,3.03874486684799,48.35));
#80269=CARTESIAN_POINT('Ctrl Pts',(138.505320519209,3.31036829948425,48.35));
#80270=CARTESIAN_POINT('Ctrl Pts',(138.680900454521,3.45968627929688,48.35));
#80271=CARTESIAN_POINT('Origin',(138.72592073679,2.99072304368019,48.5));
#80272=CARTESIAN_POINT('',(138.72592073679,2.99072304368019,48.5));
#80273=CARTESIAN_POINT('',(71.0563831288241,15.0208638924185,48.5));
#80274=CARTESIAN_POINT('',(138.72592073679,2.99072304368019,48.35));
#80275=CARTESIAN_POINT('',(138.72592073679,2.99072304368019,48.5));
#80276=CARTESIAN_POINT('',(138.72592073679,2.99072304368019,48.35));
#80277=CARTESIAN_POINT('Ctrl Pts',(138.860982179642,3.28785815834999,48.5));
#80278=CARTESIAN_POINT('Ctrl Pts',(138.860982179642,3.28785815834999,48.35));
#80279=CARTESIAN_POINT('Ctrl Pts',(138.755934506655,3.18881312012672,48.5));
#80280=CARTESIAN_POINT('Ctrl Pts',(138.755934506655,3.18881312012672,48.35));
#80281=CARTESIAN_POINT('Ctrl Pts',(138.72592073679,2.99072304368019,48.5));
#80282=CARTESIAN_POINT('Ctrl Pts',(138.72592073679,2.99072304368019,48.35));
#80283=CARTESIAN_POINT('',(138.860982179642,3.28785815834999,48.5));
#80284=CARTESIAN_POINT('Ctrl Pts',(138.860982179642,3.28785815834999,48.5));
#80285=CARTESIAN_POINT('Ctrl Pts',(138.755934506655,3.18881312012672,48.5));
#80286=CARTESIAN_POINT('Ctrl Pts',(138.72592073679,2.99072304368019,48.5));
#80287=CARTESIAN_POINT('',(138.860982179642,3.28785815834999,48.35));
#80288=CARTESIAN_POINT('',(138.860982179642,3.28785815834999,48.5));
#80289=CARTESIAN_POINT('Ctrl Pts',(138.860982179642,3.28785815834999,48.35));
#80290=CARTESIAN_POINT('Ctrl Pts',(138.755934506655,3.18881312012672,48.35));
#80291=CARTESIAN_POINT('Ctrl Pts',(138.72592073679,2.99072304368019,48.35));
#80292=CARTESIAN_POINT('Ctrl Pts',(139.123601585627,3.38690319657326,48.5));
#80293=CARTESIAN_POINT('Ctrl Pts',(139.123601585627,3.38690319657326,48.35));
#80294=CARTESIAN_POINT('Ctrl Pts',(138.96603000164,3.38690319657326,48.5));
#80295=CARTESIAN_POINT('Ctrl Pts',(138.96603000164,3.38690319657326,48.35));
#80296=CARTESIAN_POINT('Ctrl Pts',(138.860982179642,3.28785815834999,48.5));
#80297=CARTESIAN_POINT('Ctrl Pts',(138.860982179642,3.28785815834999,48.35));
#80298=CARTESIAN_POINT('',(139.123601585627,3.38690319657326,48.5));
#80299=CARTESIAN_POINT('Ctrl Pts',(139.123601585627,3.38690319657326,48.5));
#80300=CARTESIAN_POINT('Ctrl Pts',(138.96603000164,3.38690319657326,48.5));
#80301=CARTESIAN_POINT('Ctrl Pts',(138.860982179642,3.28785815834999,48.5));
#80302=CARTESIAN_POINT('',(139.123601585627,3.38690319657326,48.35));
#80303=CARTESIAN_POINT('',(139.123601585627,3.38690319657326,48.5));
#80304=CARTESIAN_POINT('Ctrl Pts',(139.123601585627,3.38690319657326,48.35));
#80305=CARTESIAN_POINT('Ctrl Pts',(138.96603000164,3.38690319657326,48.35));
#80306=CARTESIAN_POINT('Ctrl Pts',(138.860982179642,3.28785815834999,48.35));
#80307=CARTESIAN_POINT('Ctrl Pts',(139.383219599724,3.28935885429382,48.5));
#80308=CARTESIAN_POINT('Ctrl Pts',(139.383219599724,3.28935885429382,48.35));
#80309=CARTESIAN_POINT('Ctrl Pts',(139.282673865557,3.38690319657326,48.5));
#80310=CARTESIAN_POINT('Ctrl Pts',(139.282673865557,3.38690319657326,48.35));
#80311=CARTESIAN_POINT('Ctrl Pts',(139.123601585627,3.38690319657326,48.5));
#80312=CARTESIAN_POINT('Ctrl Pts',(139.123601585627,3.38690319657326,48.35));
#80313=CARTESIAN_POINT('',(139.383219599724,3.28935885429382,48.5));
#80314=CARTESIAN_POINT('Ctrl Pts',(139.383219599724,3.28935885429382,48.5));
#80315=CARTESIAN_POINT('Ctrl Pts',(139.282673865557,3.38690319657326,48.5));
#80316=CARTESIAN_POINT('Ctrl Pts',(139.123601585627,3.38690319657326,48.5));
#80317=CARTESIAN_POINT('',(139.383219599724,3.28935885429382,48.35));
#80318=CARTESIAN_POINT('',(139.383219599724,3.28935885429382,48.5));
#80319=CARTESIAN_POINT('Ctrl Pts',(139.383219599724,3.28935885429382,48.35));
#80320=CARTESIAN_POINT('Ctrl Pts',(139.282673865557,3.38690319657326,48.35));
#80321=CARTESIAN_POINT('Ctrl Pts',(139.123601585627,3.38690319657326,48.35));
#80322=CARTESIAN_POINT('Ctrl Pts',(139.483765184879,3.04324695467949,48.5));
#80323=CARTESIAN_POINT('Ctrl Pts',(139.483765184879,3.04324695467949,48.35));
#80324=CARTESIAN_POINT('Ctrl Pts',(139.483765184879,3.19181451201439,48.5));
#80325=CARTESIAN_POINT('Ctrl Pts',(139.483765184879,3.19181451201439,48.35));
#80326=CARTESIAN_POINT('Ctrl Pts',(139.383219599724,3.28935885429382,48.5));
#80327=CARTESIAN_POINT('Ctrl Pts',(139.383219599724,3.28935885429382,48.35));
#80328=CARTESIAN_POINT('',(139.483765184879,3.04324695467949,48.5));
#80329=CARTESIAN_POINT('Ctrl Pts',(139.483765184879,3.04324695467949,48.5));
#80330=CARTESIAN_POINT('Ctrl Pts',(139.483765184879,3.19181451201439,48.5));
#80331=CARTESIAN_POINT('Ctrl Pts',(139.383219599724,3.28935885429382,48.5));
#80332=CARTESIAN_POINT('',(139.483765184879,3.04324695467949,48.35));
#80333=CARTESIAN_POINT('',(139.483765184879,3.04324695467949,48.5));
#80334=CARTESIAN_POINT('Ctrl Pts',(139.483765184879,3.04324695467949,48.35));
#80335=CARTESIAN_POINT('Ctrl Pts',(139.483765184879,3.19181451201439,48.35));
#80336=CARTESIAN_POINT('Ctrl Pts',(139.383219599724,3.28935885429382,48.35));
#80337=CARTESIAN_POINT('Ctrl Pts',(139.345702648163,2.7656207382679,48.5));
#80338=CARTESIAN_POINT('Ctrl Pts',(139.345702648163,2.7656207382679,48.35));
#80339=CARTESIAN_POINT('Ctrl Pts',(139.483765184879,2.85566174983978,48.5));
#80340=CARTESIAN_POINT('Ctrl Pts',(139.483765184879,2.85566174983978,48.35));
#80341=CARTESIAN_POINT('Ctrl Pts',(139.483765184879,3.04324695467949,48.5));
#80342=CARTESIAN_POINT('Ctrl Pts',(139.483765184879,3.04324695467949,48.35));
#80343=CARTESIAN_POINT('',(139.345702648163,2.7656207382679,48.5));
#80344=CARTESIAN_POINT('Ctrl Pts',(139.345702648163,2.7656207382679,48.5));
#80345=CARTESIAN_POINT('Ctrl Pts',(139.483765184879,2.85566174983978,48.5));
#80346=CARTESIAN_POINT('Ctrl Pts',(139.483765184879,3.04324695467949,48.5));
#80347=CARTESIAN_POINT('',(139.345702648163,2.7656207382679,48.35));
#80348=CARTESIAN_POINT('',(139.345702648163,2.7656207382679,48.5));
#80349=CARTESIAN_POINT('Ctrl Pts',(139.345702648163,2.7656207382679,48.35));
#80350=CARTESIAN_POINT('Ctrl Pts',(139.483765184879,2.85566174983978,48.35));
#80351=CARTESIAN_POINT('Ctrl Pts',(139.483765184879,3.04324695467949,48.35));
#80352=CARTESIAN_POINT('Ctrl Pts',(139.03506141901,2.67557987570763,48.5));
#80353=CARTESIAN_POINT('Ctrl Pts',(139.03506141901,2.67557987570763,48.35));
#80354=CARTESIAN_POINT('Ctrl Pts',(139.207639813423,2.67557987570763,48.5));
#80355=CARTESIAN_POINT('Ctrl Pts',(139.207639813423,2.67557987570763,48.35));
#80356=CARTESIAN_POINT('Ctrl Pts',(139.345702648163,2.7656207382679,48.5));
#80357=CARTESIAN_POINT('Ctrl Pts',(139.345702648163,2.7656207382679,48.35));
#80358=CARTESIAN_POINT('',(139.03506141901,2.67557987570763,48.5));
#80359=CARTESIAN_POINT('Ctrl Pts',(139.03506141901,2.67557987570763,48.5));
#80360=CARTESIAN_POINT('Ctrl Pts',(139.207639813423,2.67557987570763,48.5));
#80361=CARTESIAN_POINT('Ctrl Pts',(139.345702648163,2.7656207382679,48.5));
#80362=CARTESIAN_POINT('',(139.03506141901,2.67557987570763,48.35));
#80363=CARTESIAN_POINT('',(139.03506141901,2.67557987570763,48.5));
#80364=CARTESIAN_POINT('Ctrl Pts',(139.03506141901,2.67557987570763,48.35));
#80365=CARTESIAN_POINT('Ctrl Pts',(139.207639813423,2.67557987570763,48.35));
#80366=CARTESIAN_POINT('Ctrl Pts',(139.345702648163,2.7656207382679,48.35));
#80367=CARTESIAN_POINT('Ctrl Pts',(138.991541534662,2.67858126759529,48.5));
#80368=CARTESIAN_POINT('Ctrl Pts',(138.991541534662,2.67858126759529,48.35));
#80369=CARTESIAN_POINT('Ctrl Pts',(139.01855391264,2.67557987570763,48.5));
#80370=CARTESIAN_POINT('Ctrl Pts',(139.01855391264,2.67557987570763,48.35));
#80371=CARTESIAN_POINT('Ctrl Pts',(139.03506141901,2.67557987570763,48.5));
#80372=CARTESIAN_POINT('Ctrl Pts',(139.03506141901,2.67557987570763,48.35));
#80373=CARTESIAN_POINT('',(138.991541534662,2.67858126759529,48.5));
#80374=CARTESIAN_POINT('Ctrl Pts',(138.991541534662,2.67858126759529,48.5));
#80375=CARTESIAN_POINT('Ctrl Pts',(139.01855391264,2.67557987570763,48.5));
#80376=CARTESIAN_POINT('Ctrl Pts',(139.03506141901,2.67557987570763,48.5));
#80377=CARTESIAN_POINT('',(138.991541534662,2.67858126759529,48.35));
#80378=CARTESIAN_POINT('',(138.991541534662,2.67858126759529,48.5));
#80379=CARTESIAN_POINT('Ctrl Pts',(138.991541534662,2.67858126759529,48.35));
#80380=CARTESIAN_POINT('Ctrl Pts',(139.01855391264,2.67557987570763,48.35));
#80381=CARTESIAN_POINT('Ctrl Pts',(139.03506141901,2.67557987570763,48.35));
#80382=CARTESIAN_POINT('Origin',(138.961527913809,2.44147354364395,48.5));
#80383=CARTESIAN_POINT('',(138.961527913809,2.44147354364395,48.5));
#80384=CARTESIAN_POINT('',(138.212047920404,-3.47942138107244,48.5));
#80385=CARTESIAN_POINT('',(138.961527913809,2.44147354364395,48.35));
#80386=CARTESIAN_POINT('',(138.961527913809,2.44147354364395,48.5));
#80387=CARTESIAN_POINT('',(138.961527913809,2.44147354364395,48.35));
#80388=CARTESIAN_POINT('Ctrl Pts',(139.152114510536,2.47148716449738,48.5));
#80389=CARTESIAN_POINT('Ctrl Pts',(139.152114510536,2.47148716449738,48.35));
#80390=CARTESIAN_POINT('Ctrl Pts',(139.075579762459,2.47148716449738,48.5));
#80391=CARTESIAN_POINT('Ctrl Pts',(139.075579762459,2.47148716449738,48.35));
#80392=CARTESIAN_POINT('Ctrl Pts',(138.961527913809,2.44147354364395,48.5));
#80393=CARTESIAN_POINT('Ctrl Pts',(138.961527913809,2.44147354364395,48.35));
#80394=CARTESIAN_POINT('',(139.152114510536,2.47148716449738,48.5));
#80395=CARTESIAN_POINT('Ctrl Pts',(139.152114510536,2.47148716449738,48.5));
#80396=CARTESIAN_POINT('Ctrl Pts',(139.075579762459,2.47148716449738,48.5));
#80397=CARTESIAN_POINT('Ctrl Pts',(138.961527913809,2.44147354364395,48.5));
#80398=CARTESIAN_POINT('',(139.152114510536,2.47148716449738,48.35));
#80399=CARTESIAN_POINT('',(139.152114510536,2.47148716449738,48.5));
#80400=CARTESIAN_POINT('Ctrl Pts',(139.152114510536,2.47148716449738,48.35));
#80401=CARTESIAN_POINT('Ctrl Pts',(139.075579762459,2.47148716449738,48.35));
#80402=CARTESIAN_POINT('Ctrl Pts',(138.961527913809,2.44147354364395,48.35));
#80403=CARTESIAN_POINT('Ctrl Pts',(139.461254894733,2.35068225860596,48.5));
#80404=CARTESIAN_POINT('Ctrl Pts',(139.461254894733,2.35068225860596,48.35));
#80405=CARTESIAN_POINT('Ctrl Pts',(139.339699864388,2.47148716449738,48.5));
#80406=CARTESIAN_POINT('Ctrl Pts',(139.339699864388,2.47148716449738,48.35));
#80407=CARTESIAN_POINT('Ctrl Pts',(139.152114510536,2.47148716449738,48.5));
#80408=CARTESIAN_POINT('Ctrl Pts',(139.152114510536,2.47148716449738,48.35));
#80409=CARTESIAN_POINT('',(139.461254894733,2.35068225860596,48.5));
#80410=CARTESIAN_POINT('Ctrl Pts',(139.461254894733,2.35068225860596,48.5));
#80411=CARTESIAN_POINT('Ctrl Pts',(139.339699864388,2.47148716449738,48.5));
#80412=CARTESIAN_POINT('Ctrl Pts',(139.152114510536,2.47148716449738,48.5));
#80413=CARTESIAN_POINT('',(139.461254894733,2.35068225860596,48.35));
#80414=CARTESIAN_POINT('',(139.461254894733,2.35068225860596,48.5));
#80415=CARTESIAN_POINT('Ctrl Pts',(139.461254894733,2.35068225860596,48.35));
#80416=CARTESIAN_POINT('Ctrl Pts',(139.339699864388,2.47148716449738,48.35));
#80417=CARTESIAN_POINT('Ctrl Pts',(139.152114510536,2.47148716449738,48.35));
#80418=CARTESIAN_POINT('Ctrl Pts',(139.582810223103,2.04379284381866,48.5));
#80419=CARTESIAN_POINT('Ctrl Pts',(139.582810223103,2.04379284381866,48.35));
#80420=CARTESIAN_POINT('Ctrl Pts',(139.582810223103,2.22987735271454,48.5));
#80421=CARTESIAN_POINT('Ctrl Pts',(139.582810223103,2.22987735271454,48.35));
#80422=CARTESIAN_POINT('Ctrl Pts',(139.461254894733,2.35068225860596,48.5));
#80423=CARTESIAN_POINT('Ctrl Pts',(139.461254894733,2.35068225860596,48.35));
#80424=CARTESIAN_POINT('',(139.582810223103,2.04379284381866,48.5));
#80425=CARTESIAN_POINT('Ctrl Pts',(139.582810223103,2.04379284381866,48.5));
#80426=CARTESIAN_POINT('Ctrl Pts',(139.582810223103,2.22987735271454,48.5));
#80427=CARTESIAN_POINT('Ctrl Pts',(139.461254894733,2.35068225860596,48.5));
#80428=CARTESIAN_POINT('',(139.582810223103,2.04379284381866,48.35));
#80429=CARTESIAN_POINT('',(139.582810223103,2.04379284381866,48.5));
#80430=CARTESIAN_POINT('Ctrl Pts',(139.582810223103,2.04379284381866,48.35));
#80431=CARTESIAN_POINT('Ctrl Pts',(139.582810223103,2.22987735271454,48.35));
#80432=CARTESIAN_POINT('Ctrl Pts',(139.461254894733,2.35068225860596,48.35));
#80433=CARTESIAN_POINT('Ctrl Pts',(139.451500594616,1.71664410829544,48.5));
#80434=CARTESIAN_POINT('Ctrl Pts',(139.451500594616,1.71664410829544,48.35));
#80435=CARTESIAN_POINT('Ctrl Pts',(139.582810223103,1.8487041592598,48.5));
#80436=CARTESIAN_POINT('Ctrl Pts',(139.582810223103,1.8487041592598,48.35));
#80437=CARTESIAN_POINT('Ctrl Pts',(139.582810223103,2.04379284381866,48.5));
#80438=CARTESIAN_POINT('Ctrl Pts',(139.582810223103,2.04379284381866,48.35));
#80439=CARTESIAN_POINT('',(139.451500594616,1.71664410829544,48.5));
#80440=CARTESIAN_POINT('Ctrl Pts',(139.451500594616,1.71664410829544,48.5));
#80441=CARTESIAN_POINT('Ctrl Pts',(139.582810223103,1.8487041592598,48.5));
#80442=CARTESIAN_POINT('Ctrl Pts',(139.582810223103,2.04379284381866,48.5));
#80443=CARTESIAN_POINT('',(139.451500594616,1.71664410829544,48.35));
#80444=CARTESIAN_POINT('',(139.451500594616,1.71664410829544,48.5));
#80445=CARTESIAN_POINT('Ctrl Pts',(139.451500594616,1.71664410829544,48.35));
#80446=CARTESIAN_POINT('Ctrl Pts',(139.582810223103,1.8487041592598,48.35));
#80447=CARTESIAN_POINT('Ctrl Pts',(139.582810223103,2.04379284381866,48.35));
#80448=CARTESIAN_POINT('Ctrl Pts',(139.12960422039,1.58458405733109,48.5));
#80449=CARTESIAN_POINT('Ctrl Pts',(139.12960422039,1.58458405733109,48.35));
#80450=CARTESIAN_POINT('Ctrl Pts',(139.320190966129,1.58458405733109,48.5));
#80451=CARTESIAN_POINT('Ctrl Pts',(139.320190966129,1.58458405733109,48.35));
#80452=CARTESIAN_POINT('Ctrl Pts',(139.451500594616,1.71664410829544,48.5));
#80453=CARTESIAN_POINT('Ctrl Pts',(139.451500594616,1.71664410829544,48.35));
#80454=CARTESIAN_POINT('',(139.12960422039,1.58458405733109,48.5));
#80455=CARTESIAN_POINT('Ctrl Pts',(139.12960422039,1.58458405733109,48.5));
#80456=CARTESIAN_POINT('Ctrl Pts',(139.320190966129,1.58458405733109,48.5));
#80457=CARTESIAN_POINT('Ctrl Pts',(139.451500594616,1.71664410829544,48.5));
#80458=CARTESIAN_POINT('',(139.12960422039,1.58458405733109,48.35));
#80459=CARTESIAN_POINT('',(139.12960422039,1.58458405733109,48.5));
#80460=CARTESIAN_POINT('Ctrl Pts',(139.12960422039,1.58458405733109,48.35));
#80461=CARTESIAN_POINT('Ctrl Pts',(139.320190966129,1.58458405733109,48.35));
#80462=CARTESIAN_POINT('Ctrl Pts',(139.451500594616,1.71664410829544,48.35));
#80463=CARTESIAN_POINT('Ctrl Pts',(138.857230514288,1.68588006496429,48.5));
#80464=CARTESIAN_POINT('Ctrl Pts',(138.857230514288,1.68588006496429,48.35));
#80465=CARTESIAN_POINT('Ctrl Pts',(138.969031393528,1.58458405733109,48.5));
#80466=CARTESIAN_POINT('Ctrl Pts',(138.969031393528,1.58458405733109,48.35));
#80467=CARTESIAN_POINT('Ctrl Pts',(139.12960422039,1.58458405733109,48.5));
#80468=CARTESIAN_POINT('Ctrl Pts',(139.12960422039,1.58458405733109,48.35));
#80469=CARTESIAN_POINT('',(138.857230514288,1.68588006496429,48.5));
#80470=CARTESIAN_POINT('Ctrl Pts',(138.857230514288,1.68588006496429,48.5));
#80471=CARTESIAN_POINT('Ctrl Pts',(138.969031393528,1.58458405733109,48.5));
#80472=CARTESIAN_POINT('Ctrl Pts',(139.12960422039,1.58458405733109,48.5));
#80473=CARTESIAN_POINT('',(138.857230514288,1.68588006496429,48.35));
#80474=CARTESIAN_POINT('',(138.857230514288,1.68588006496429,48.5));
#80475=CARTESIAN_POINT('Ctrl Pts',(138.857230514288,1.68588006496429,48.35));
#80476=CARTESIAN_POINT('Ctrl Pts',(138.969031393528,1.58458405733109,48.35));
#80477=CARTESIAN_POINT('Ctrl Pts',(139.12960422039,1.58458405733109,48.35));
#80478=CARTESIAN_POINT('Ctrl Pts',(138.698908507824,2.01678061485291,48.5));
#80479=CARTESIAN_POINT('Ctrl Pts',(138.698908507824,2.01678061485291,48.35));
#80480=CARTESIAN_POINT('Ctrl Pts',(138.745429635048,1.7871760725975,48.5));
#80481=CARTESIAN_POINT('Ctrl Pts',(138.745429635048,1.7871760725975,48.35));
#80482=CARTESIAN_POINT('Ctrl Pts',(138.857230514288,1.68588006496429,48.5));
#80483=CARTESIAN_POINT('Ctrl Pts',(138.857230514288,1.68588006496429,48.35));
#80484=CARTESIAN_POINT('',(138.698908507824,2.01678061485291,48.5));
#80485=CARTESIAN_POINT('Ctrl Pts',(138.698908507824,2.01678061485291,48.5));
#80486=CARTESIAN_POINT('Ctrl Pts',(138.745429635048,1.7871760725975,48.5));
#80487=CARTESIAN_POINT('Ctrl Pts',(138.857230514288,1.68588006496429,48.5));
#80488=CARTESIAN_POINT('',(138.698908507824,2.01678061485291,48.35));
#80489=CARTESIAN_POINT('',(138.698908507824,2.01678061485291,48.5));
#80490=CARTESIAN_POINT('Ctrl Pts',(138.698908507824,2.01678061485291,48.35));
#80491=CARTESIAN_POINT('Ctrl Pts',(138.745429635048,1.7871760725975,48.35));
#80492=CARTESIAN_POINT('Ctrl Pts',(138.857230514288,1.68588006496429,48.35));
#80493=CARTESIAN_POINT('Origin',(138.428785771132,1.98076421022415,48.5));
#80494=CARTESIAN_POINT('',(138.428785771132,1.98076421022415,48.5));
#80495=CARTESIAN_POINT('',(70.817654041723,-7.03406329963869,48.5));
#80496=CARTESIAN_POINT('',(138.428785771132,1.98076421022415,48.35));
#80497=CARTESIAN_POINT('',(138.428785771132,1.98076421022415,48.5));
#80498=CARTESIAN_POINT('',(138.428785771132,1.98076421022415,48.35));
#80499=CARTESIAN_POINT('Ctrl Pts',(138.647135019302,1.53356069326401,48.5));
#80500=CARTESIAN_POINT('Ctrl Pts',(138.647135019302,1.53356069326401,48.35));
#80501=CARTESIAN_POINT('Ctrl Pts',(138.455798000097,1.70613938570023,48.5));
#80502=CARTESIAN_POINT('Ctrl Pts',(138.455798000097,1.70613938570023,48.35));
#80503=CARTESIAN_POINT('Ctrl Pts',(138.428785771132,1.98076421022415,48.5));
#80504=CARTESIAN_POINT('Ctrl Pts',(138.428785771132,1.98076421022415,48.35));
#80505=CARTESIAN_POINT('Ctrl Pts',(138.647135019302,1.53356069326401,48.5));
#80506=CARTESIAN_POINT('Ctrl Pts',(138.455798000097,1.70613938570023,48.5));
#80507=CARTESIAN_POINT('Ctrl Pts',(138.428785771132,1.98076421022415,48.5));
#80508=CARTESIAN_POINT('Ctrl Pts',(138.647135019302,1.53356069326401,48.35));
#80509=CARTESIAN_POINT('Ctrl Pts',(138.455798000097,1.70613938570023,48.35));
#80510=CARTESIAN_POINT('Ctrl Pts',(138.428785771132,1.98076421022415,48.35));
#80511=CARTESIAN_POINT('Origin',(139.999999895692,2.48499320447445,48.35));
#80512=CARTESIAN_POINT('Origin',(0.,8.,48.5));
#80513=CARTESIAN_POINT('Ctrl Pts',(130.870395654812,3.38540250062943,48.5));
#80514=CARTESIAN_POINT('Ctrl Pts',(130.870395654812,3.38540250062943,48.35));
#80515=CARTESIAN_POINT('Ctrl Pts',(130.684310847893,3.38540250062943,48.5));
#80516=CARTESIAN_POINT('Ctrl Pts',(130.684310847893,3.38540250062943,48.35));
#80517=CARTESIAN_POINT('Ctrl Pts',(130.573260540143,3.22783091664314,48.5));
#80518=CARTESIAN_POINT('Ctrl Pts',(130.573260540143,3.22783091664314,48.35));
#80519=CARTESIAN_POINT('',(130.870395654812,3.38540250062943,48.5));
#80520=CARTESIAN_POINT('',(130.573260540143,3.22783091664314,48.5));
#80521=CARTESIAN_POINT('Ctrl Pts',(130.870395654812,3.38540250062943,48.5));
#80522=CARTESIAN_POINT('Ctrl Pts',(130.684310847893,3.38540250062943,48.5));
#80523=CARTESIAN_POINT('Ctrl Pts',(130.573260540143,3.22783091664314,48.5));
#80524=CARTESIAN_POINT('',(130.870395654812,3.38540250062943,48.35));
#80525=CARTESIAN_POINT('',(130.870395654812,3.38540250062943,48.5));
#80526=CARTESIAN_POINT('',(130.573260540143,3.22783091664314,48.35));
#80527=CARTESIAN_POINT('Ctrl Pts',(130.870395654812,3.38540250062943,48.35));
#80528=CARTESIAN_POINT('Ctrl Pts',(130.684310847893,3.38540250062943,48.35));
#80529=CARTESIAN_POINT('Ctrl Pts',(130.573260540143,3.22783091664314,48.35));
#80530=CARTESIAN_POINT('',(130.573260540143,3.22783091664314,48.5));
#80531=CARTESIAN_POINT('Ctrl Pts',(131.18628894724,3.2068213224411,48.5));
#80532=CARTESIAN_POINT('Ctrl Pts',(131.18628894724,3.2068213224411,48.35));
#80533=CARTESIAN_POINT('Ctrl Pts',(131.059481257573,3.38540250062943,48.5));
#80534=CARTESIAN_POINT('Ctrl Pts',(131.059481257573,3.38540250062943,48.35));
#80535=CARTESIAN_POINT('Ctrl Pts',(130.870395654812,3.38540250062943,48.5));
#80536=CARTESIAN_POINT('Ctrl Pts',(130.870395654812,3.38540250062943,48.35));
#80537=CARTESIAN_POINT('',(131.18628894724,3.2068213224411,48.5));
#80538=CARTESIAN_POINT('Ctrl Pts',(131.18628894724,3.2068213224411,48.5));
#80539=CARTESIAN_POINT('Ctrl Pts',(131.059481257573,3.38540250062943,48.5));
#80540=CARTESIAN_POINT('Ctrl Pts',(130.870395654812,3.38540250062943,48.5));
#80541=CARTESIAN_POINT('',(131.18628894724,3.2068213224411,48.35));
#80542=CARTESIAN_POINT('',(131.18628894724,3.2068213224411,48.5));
#80543=CARTESIAN_POINT('Ctrl Pts',(131.18628894724,3.2068213224411,48.35));
#80544=CARTESIAN_POINT('Ctrl Pts',(131.059481257573,3.38540250062943,48.35));
#80545=CARTESIAN_POINT('Ctrl Pts',(130.870395654812,3.38540250062943,48.35));
#80546=CARTESIAN_POINT('Ctrl Pts',(131.313096636906,2.48499327898026,48.5));
#80547=CARTESIAN_POINT('Ctrl Pts',(131.313096636906,2.48499327898026,48.35));
#80548=CARTESIAN_POINT('Ctrl Pts',(131.313096636906,3.02824014425278,48.5));
#80549=CARTESIAN_POINT('Ctrl Pts',(131.313096636906,3.02824014425278,48.35));
#80550=CARTESIAN_POINT('Ctrl Pts',(131.18628894724,3.2068213224411,48.5));
#80551=CARTESIAN_POINT('Ctrl Pts',(131.18628894724,3.2068213224411,48.35));
#80552=CARTESIAN_POINT('',(131.313096636906,2.48499327898026,48.5));
#80553=CARTESIAN_POINT('Ctrl Pts',(131.313096636906,2.48499327898026,48.5));
#80554=CARTESIAN_POINT('Ctrl Pts',(131.313096636906,3.02824014425278,48.5));
#80555=CARTESIAN_POINT('Ctrl Pts',(131.18628894724,3.2068213224411,48.5));
#80556=CARTESIAN_POINT('',(131.313096636906,2.48499327898026,48.35));
#80557=CARTESIAN_POINT('',(131.313096636906,2.48499327898026,48.5));
#80558=CARTESIAN_POINT('Ctrl Pts',(131.313096636906,2.48499327898026,48.35));
#80559=CARTESIAN_POINT('Ctrl Pts',(131.313096636906,3.02824014425278,48.35));
#80560=CARTESIAN_POINT('Ctrl Pts',(131.18628894724,3.2068213224411,48.35));
#80561=CARTESIAN_POINT('Ctrl Pts',(131.18628894724,1.76466578245163,48.5));
#80562=CARTESIAN_POINT('Ctrl Pts',(131.18628894724,1.76466578245163,48.35));
#80563=CARTESIAN_POINT('Ctrl Pts',(131.313096636906,1.9447478055954,48.5));
#80564=CARTESIAN_POINT('Ctrl Pts',(131.313096636906,1.9447478055954,48.35));
#80565=CARTESIAN_POINT('Ctrl Pts',(131.313096636906,2.48499327898026,48.5));
#80566=CARTESIAN_POINT('Ctrl Pts',(131.313096636906,2.48499327898026,48.35));
#80567=CARTESIAN_POINT('',(131.18628894724,1.76466578245163,48.5));
#80568=CARTESIAN_POINT('Ctrl Pts',(131.18628894724,1.76466578245163,48.5));
#80569=CARTESIAN_POINT('Ctrl Pts',(131.313096636906,1.9447478055954,48.5));
#80570=CARTESIAN_POINT('Ctrl Pts',(131.313096636906,2.48499327898026,48.5));
#80571=CARTESIAN_POINT('',(131.18628894724,1.76466578245163,48.35));
#80572=CARTESIAN_POINT('',(131.18628894724,1.76466578245163,48.5));
#80573=CARTESIAN_POINT('Ctrl Pts',(131.18628894724,1.76466578245163,48.35));
#80574=CARTESIAN_POINT('Ctrl Pts',(131.313096636906,1.9447478055954,48.35));
#80575=CARTESIAN_POINT('Ctrl Pts',(131.313096636906,2.48499327898026,48.35));
#80576=CARTESIAN_POINT('Ctrl Pts',(130.873396748677,1.58458405733109,48.5));
#80577=CARTESIAN_POINT('Ctrl Pts',(130.873396748677,1.58458405733109,48.35));
#80578=CARTESIAN_POINT('Ctrl Pts',(131.059481257573,1.58458405733109,48.5));
#80579=CARTESIAN_POINT('Ctrl Pts',(131.059481257573,1.58458405733109,48.35));
#80580=CARTESIAN_POINT('Ctrl Pts',(131.18628894724,1.76466578245163,48.5));
#80581=CARTESIAN_POINT('Ctrl Pts',(131.18628894724,1.76466578245163,48.35));
#80582=CARTESIAN_POINT('',(130.873396748677,1.58458405733109,48.5));
#80583=CARTESIAN_POINT('Ctrl Pts',(130.873396748677,1.58458405733109,48.5));
#80584=CARTESIAN_POINT('Ctrl Pts',(131.059481257573,1.58458405733109,48.5));
#80585=CARTESIAN_POINT('Ctrl Pts',(131.18628894724,1.76466578245163,48.5));
#80586=CARTESIAN_POINT('',(130.873396748677,1.58458405733109,48.35));
#80587=CARTESIAN_POINT('',(130.873396748677,1.58458405733109,48.5));
#80588=CARTESIAN_POINT('Ctrl Pts',(130.873396748677,1.58458405733109,48.35));
#80589=CARTESIAN_POINT('Ctrl Pts',(131.059481257573,1.58458405733109,48.35));
#80590=CARTESIAN_POINT('Ctrl Pts',(131.18628894724,1.76466578245163,48.35));
#80591=CARTESIAN_POINT('Ctrl Pts',(130.560504550114,1.76391565799713,48.5));
#80592=CARTESIAN_POINT('Ctrl Pts',(130.560504550114,1.76391565799713,48.35));
#80593=CARTESIAN_POINT('Ctrl Pts',(130.687312239781,1.58458405733109,48.5));
#80594=CARTESIAN_POINT('Ctrl Pts',(130.687312239781,1.58458405733109,48.35));
#80595=CARTESIAN_POINT('Ctrl Pts',(130.873396748677,1.58458405733109,48.5));
#80596=CARTESIAN_POINT('Ctrl Pts',(130.873396748677,1.58458405733109,48.35));
#80597=CARTESIAN_POINT('',(130.560504550114,1.76391565799713,48.5));
#80598=CARTESIAN_POINT('Ctrl Pts',(130.560504550114,1.76391565799713,48.5));
#80599=CARTESIAN_POINT('Ctrl Pts',(130.687312239781,1.58458405733109,48.5));
#80600=CARTESIAN_POINT('Ctrl Pts',(130.873396748677,1.58458405733109,48.5));
#80601=CARTESIAN_POINT('',(130.560504550114,1.76391565799713,48.35));
#80602=CARTESIAN_POINT('',(130.560504550114,1.76391565799713,48.5));
#80603=CARTESIAN_POINT('Ctrl Pts',(130.560504550114,1.76391565799713,48.35));
#80604=CARTESIAN_POINT('Ctrl Pts',(130.687312239781,1.58458405733109,48.35));
#80605=CARTESIAN_POINT('Ctrl Pts',(130.873396748677,1.58458405733109,48.35));
#80606=CARTESIAN_POINT('Ctrl Pts',(130.433696860448,2.48499327898026,48.5));
#80607=CARTESIAN_POINT('Ctrl Pts',(130.433696860448,2.48499327898026,48.35));
#80608=CARTESIAN_POINT('Ctrl Pts',(130.433696860448,1.94324696063995,48.5));
#80609=CARTESIAN_POINT('Ctrl Pts',(130.433696860448,1.94324696063995,48.35));
#80610=CARTESIAN_POINT('Ctrl Pts',(130.560504550114,1.76391565799713,48.5));
#80611=CARTESIAN_POINT('Ctrl Pts',(130.560504550114,1.76391565799713,48.35));
#80612=CARTESIAN_POINT('',(130.433696860448,2.48499327898026,48.5));
#80613=CARTESIAN_POINT('Ctrl Pts',(130.433696860448,2.48499327898026,48.5));
#80614=CARTESIAN_POINT('Ctrl Pts',(130.433696860448,1.94324696063995,48.5));
#80615=CARTESIAN_POINT('Ctrl Pts',(130.560504550114,1.76391565799713,48.5));
#80616=CARTESIAN_POINT('',(130.433696860448,2.48499327898026,48.35));
#80617=CARTESIAN_POINT('',(130.433696860448,2.48499327898026,48.5));
#80618=CARTESIAN_POINT('Ctrl Pts',(130.433696860448,2.48499327898026,48.35));
#80619=CARTESIAN_POINT('Ctrl Pts',(130.433696860448,1.94324696063995,48.35));
#80620=CARTESIAN_POINT('Ctrl Pts',(130.560504550114,1.76391565799713,48.35));
#80621=CARTESIAN_POINT('Ctrl Pts',(130.573260540143,3.22783091664314,48.5));
#80622=CARTESIAN_POINT('Ctrl Pts',(130.573260540143,3.22783091664314,48.35));
#80623=CARTESIAN_POINT('Ctrl Pts',(130.433696860448,3.02673944830894,48.5));
#80624=CARTESIAN_POINT('Ctrl Pts',(130.433696860448,3.02673944830894,48.35));
#80625=CARTESIAN_POINT('Ctrl Pts',(130.433696860448,2.48499327898026,48.5));
#80626=CARTESIAN_POINT('Ctrl Pts',(130.433696860448,2.48499327898026,48.35));
#80627=CARTESIAN_POINT('Ctrl Pts',(130.573260540143,3.22783091664314,48.5));
#80628=CARTESIAN_POINT('Ctrl Pts',(130.433696860448,3.02673944830894,48.5));
#80629=CARTESIAN_POINT('Ctrl Pts',(130.433696860448,2.48499327898026,48.5));
#80630=CARTESIAN_POINT('Ctrl Pts',(130.573260540143,3.22783091664314,48.35));
#80631=CARTESIAN_POINT('Ctrl Pts',(130.433696860448,3.02673944830894,48.35));
#80632=CARTESIAN_POINT('Ctrl Pts',(130.433696860448,2.48499327898026,48.35));
#80633=CARTESIAN_POINT('Ctrl Pts',(130.873396748677,1.36248314380646,48.5));
#80634=CARTESIAN_POINT('Ctrl Pts',(130.873396748677,1.36248314380646,48.35));
#80635=CARTESIAN_POINT('Ctrl Pts',(130.555252188817,1.36248314380646,48.5));
#80636=CARTESIAN_POINT('Ctrl Pts',(130.555252188817,1.36248314380646,48.35));
#80637=CARTESIAN_POINT('Ctrl Pts',(130.373669618741,1.59058684110642,48.5));
#80638=CARTESIAN_POINT('Ctrl Pts',(130.373669618741,1.59058684110642,48.35));
#80639=CARTESIAN_POINT('',(130.873396748677,1.36248314380646,48.5));
#80640=CARTESIAN_POINT('',(130.373669618741,1.59058684110642,48.5));
#80641=CARTESIAN_POINT('Ctrl Pts',(130.873396748677,1.36248314380646,48.5));
#80642=CARTESIAN_POINT('Ctrl Pts',(130.555252188817,1.36248314380646,48.5));
#80643=CARTESIAN_POINT('Ctrl Pts',(130.373669618741,1.59058684110642,48.5));
#80644=CARTESIAN_POINT('',(130.873396748677,1.36248314380646,48.35));
#80645=CARTESIAN_POINT('',(130.873396748677,1.36248314380646,48.5));
#80646=CARTESIAN_POINT('',(130.373669618741,1.59058684110642,48.35));
#80647=CARTESIAN_POINT('Ctrl Pts',(130.873396748677,1.36248314380646,48.35));
#80648=CARTESIAN_POINT('Ctrl Pts',(130.555252188817,1.36248314380646,48.35));
#80649=CARTESIAN_POINT('Ctrl Pts',(130.373669618741,1.59058684110642,48.35));
#80650=CARTESIAN_POINT('',(130.373669618741,1.59058684110642,48.5));
#80651=CARTESIAN_POINT('Ctrl Pts',(131.273328417912,1.49229192733765,48.5));
#80652=CARTESIAN_POINT('Ctrl Pts',(131.273328417912,1.49229192733765,48.35));
#80653=CARTESIAN_POINT('Ctrl Pts',(131.11500656046,1.36248314380646,48.5));
#80654=CARTESIAN_POINT('Ctrl Pts',(131.11500656046,1.36248314380646,48.35));
#80655=CARTESIAN_POINT('Ctrl Pts',(130.873396748677,1.36248314380646,48.5));
#80656=CARTESIAN_POINT('Ctrl Pts',(130.873396748677,1.36248314380646,48.35));
#80657=CARTESIAN_POINT('',(131.273328417912,1.49229192733765,48.5));
#80658=CARTESIAN_POINT('Ctrl Pts',(131.273328417912,1.49229192733765,48.5));
#80659=CARTESIAN_POINT('Ctrl Pts',(131.11500656046,1.36248314380646,48.5));
#80660=CARTESIAN_POINT('Ctrl Pts',(130.873396748677,1.36248314380646,48.5));
#80661=CARTESIAN_POINT('',(131.273328417912,1.49229192733765,48.35));
#80662=CARTESIAN_POINT('',(131.273328417912,1.49229192733765,48.5));
#80663=CARTESIAN_POINT('Ctrl Pts',(131.273328417912,1.49229192733765,48.35));
#80664=CARTESIAN_POINT('Ctrl Pts',(131.11500656046,1.36248314380646,48.35));
#80665=CARTESIAN_POINT('Ctrl Pts',(130.873396748677,1.36248314380646,48.35));
#80666=CARTESIAN_POINT('Ctrl Pts',(131.511186713353,1.85995900630951,48.5));
#80667=CARTESIAN_POINT('Ctrl Pts',(131.511186713353,1.85995900630951,48.35));
#80668=CARTESIAN_POINT('Ctrl Pts',(131.431650275365,1.62210100889206,48.5));
#80669=CARTESIAN_POINT('Ctrl Pts',(131.431650275365,1.62210100889206,48.35));
#80670=CARTESIAN_POINT('Ctrl Pts',(131.273328417912,1.49229192733765,48.5));
#80671=CARTESIAN_POINT('Ctrl Pts',(131.273328417912,1.49229192733765,48.35));
#80672=CARTESIAN_POINT('',(131.511186713353,1.85995900630951,48.5));
#80673=CARTESIAN_POINT('Ctrl Pts',(131.511186713353,1.85995900630951,48.5));
#80674=CARTESIAN_POINT('Ctrl Pts',(131.431650275365,1.62210100889206,48.5));
#80675=CARTESIAN_POINT('Ctrl Pts',(131.273328417912,1.49229192733765,48.5));
#80676=CARTESIAN_POINT('',(131.511186713353,1.85995900630951,48.35));
#80677=CARTESIAN_POINT('',(131.511186713353,1.85995900630951,48.5));
#80678=CARTESIAN_POINT('Ctrl Pts',(131.511186713353,1.85995900630951,48.35));
#80679=CARTESIAN_POINT('Ctrl Pts',(131.431650275365,1.62210100889206,48.35));
#80680=CARTESIAN_POINT('Ctrl Pts',(131.273328417912,1.49229192733765,48.35));
#80681=CARTESIAN_POINT('Ctrl Pts',(131.590722555295,2.48499327898026,48.5));
#80682=CARTESIAN_POINT('Ctrl Pts',(131.590722555295,2.48499327898026,48.35));
#80683=CARTESIAN_POINT('Ctrl Pts',(131.590722555295,2.09781730175018,48.5));
#80684=CARTESIAN_POINT('Ctrl Pts',(131.590722555295,2.09781730175018,48.35));
#80685=CARTESIAN_POINT('Ctrl Pts',(131.511186713353,1.85995900630951,48.5));
#80686=CARTESIAN_POINT('Ctrl Pts',(131.511186713353,1.85995900630951,48.35));
#80687=CARTESIAN_POINT('',(131.590722555295,2.48499327898026,48.5));
#80688=CARTESIAN_POINT('Ctrl Pts',(131.590722555295,2.48499327898026,48.5));
#80689=CARTESIAN_POINT('Ctrl Pts',(131.590722555295,2.09781730175018,48.5));
#80690=CARTESIAN_POINT('Ctrl Pts',(131.511186713353,1.85995900630951,48.5));
#80691=CARTESIAN_POINT('',(131.590722555295,2.48499327898026,48.35));
#80692=CARTESIAN_POINT('',(131.590722555295,2.48499327898026,48.5));
#80693=CARTESIAN_POINT('Ctrl Pts',(131.590722555295,2.48499327898026,48.35));
#80694=CARTESIAN_POINT('Ctrl Pts',(131.590722555295,2.09781730175018,48.35));
#80695=CARTESIAN_POINT('Ctrl Pts',(131.511186713353,1.85995900630951,48.35));
#80696=CARTESIAN_POINT('Ctrl Pts',(131.541200036183,3.00497958064079,48.5));
#80697=CARTESIAN_POINT('Ctrl Pts',(131.541200036183,3.00497958064079,48.35));
#80698=CARTESIAN_POINT('Ctrl Pts',(131.590722555295,2.81214186549187,48.5));
#80699=CARTESIAN_POINT('Ctrl Pts',(131.590722555295,2.81214186549187,48.35));
#80700=CARTESIAN_POINT('Ctrl Pts',(131.590722555295,2.48499327898026,48.5));
#80701=CARTESIAN_POINT('Ctrl Pts',(131.590722555295,2.48499327898026,48.35));
#80702=CARTESIAN_POINT('',(131.541200036183,3.00497958064079,48.5));
#80703=CARTESIAN_POINT('Ctrl Pts',(131.541200036183,3.00497958064079,48.5));
#80704=CARTESIAN_POINT('Ctrl Pts',(131.590722555295,2.81214186549187,48.5));
#80705=CARTESIAN_POINT('Ctrl Pts',(131.590722555295,2.48499327898026,48.5));
#80706=CARTESIAN_POINT('',(131.541200036183,3.00497958064079,48.35));
#80707=CARTESIAN_POINT('',(131.541200036183,3.00497958064079,48.5));
#80708=CARTESIAN_POINT('Ctrl Pts',(131.541200036183,3.00497958064079,48.35));
#80709=CARTESIAN_POINT('Ctrl Pts',(131.590722555295,2.81214186549187,48.35));
#80710=CARTESIAN_POINT('Ctrl Pts',(131.590722555295,2.48499327898026,48.35));
#80711=CARTESIAN_POINT('Ctrl Pts',(131.404638046399,3.33212831616402,48.5));
#80712=CARTESIAN_POINT('Ctrl Pts',(131.404638046399,3.33212831616402,48.35));
#80713=CARTESIAN_POINT('Ctrl Pts',(131.491677517071,3.19781729578972,48.5));
#80714=CARTESIAN_POINT('Ctrl Pts',(131.491677517071,3.19781729578972,48.35));
#80715=CARTESIAN_POINT('Ctrl Pts',(131.541200036183,3.00497958064079,48.5));
#80716=CARTESIAN_POINT('Ctrl Pts',(131.541200036183,3.00497958064079,48.35));
#80717=CARTESIAN_POINT('',(131.404638046399,3.33212831616402,48.5));
#80718=CARTESIAN_POINT('Ctrl Pts',(131.404638046399,3.33212831616402,48.5));
#80719=CARTESIAN_POINT('Ctrl Pts',(131.491677517071,3.19781729578972,48.5));
#80720=CARTESIAN_POINT('Ctrl Pts',(131.541200036183,3.00497958064079,48.5));
#80721=CARTESIAN_POINT('',(131.404638046399,3.33212831616402,48.35));
#80722=CARTESIAN_POINT('',(131.404638046399,3.33212831616402,48.5));
#80723=CARTESIAN_POINT('Ctrl Pts',(131.404638046399,3.33212831616402,48.35));
#80724=CARTESIAN_POINT('Ctrl Pts',(131.491677517071,3.19781729578972,48.35));
#80725=CARTESIAN_POINT('Ctrl Pts',(131.541200036183,3.00497958064079,48.35));
#80726=CARTESIAN_POINT('Ctrl Pts',(131.184038275853,3.5377217233181,48.5));
#80727=CARTESIAN_POINT('Ctrl Pts',(131.184038275853,3.5377217233181,48.35));
#80728=CARTESIAN_POINT('Ctrl Pts',(131.317598575726,3.46643933653831,48.5));
#80729=CARTESIAN_POINT('Ctrl Pts',(131.317598575726,3.46643933653831,48.35));
#80730=CARTESIAN_POINT('Ctrl Pts',(131.404638046399,3.33212831616402,48.5));
#80731=CARTESIAN_POINT('Ctrl Pts',(131.404638046399,3.33212831616402,48.35));
#80732=CARTESIAN_POINT('',(131.184038275853,3.5377217233181,48.5));
#80733=CARTESIAN_POINT('Ctrl Pts',(131.184038275853,3.5377217233181,48.5));
#80734=CARTESIAN_POINT('Ctrl Pts',(131.317598575726,3.46643933653831,48.5));
#80735=CARTESIAN_POINT('Ctrl Pts',(131.404638046399,3.33212831616402,48.5));
#80736=CARTESIAN_POINT('',(131.184038275853,3.5377217233181,48.35));
#80737=CARTESIAN_POINT('',(131.184038275853,3.5377217233181,48.5));
#80738=CARTESIAN_POINT('Ctrl Pts',(131.184038275853,3.5377217233181,48.35));
#80739=CARTESIAN_POINT('Ctrl Pts',(131.317598575726,3.46643933653831,48.35));
#80740=CARTESIAN_POINT('Ctrl Pts',(131.404638046399,3.33212831616402,48.35));
#80741=CARTESIAN_POINT('Ctrl Pts',(130.873396748677,3.60900411009789,48.5));
#80742=CARTESIAN_POINT('Ctrl Pts',(130.873396748677,3.60900411009789,48.35));
#80743=CARTESIAN_POINT('Ctrl Pts',(131.050477379933,3.60900411009789,48.5));
#80744=CARTESIAN_POINT('Ctrl Pts',(131.050477379933,3.60900411009789,48.35));
#80745=CARTESIAN_POINT('Ctrl Pts',(131.184038275853,3.5377217233181,48.5));
#80746=CARTESIAN_POINT('Ctrl Pts',(131.184038275853,3.5377217233181,48.35));
#80747=CARTESIAN_POINT('',(130.873396748677,3.60900411009789,48.5));
#80748=CARTESIAN_POINT('Ctrl Pts',(130.873396748677,3.60900411009789,48.5));
#80749=CARTESIAN_POINT('Ctrl Pts',(131.050477379933,3.60900411009789,48.5));
#80750=CARTESIAN_POINT('Ctrl Pts',(131.184038275853,3.5377217233181,48.5));
#80751=CARTESIAN_POINT('',(130.873396748677,3.60900411009789,48.35));
#80752=CARTESIAN_POINT('',(130.873396748677,3.60900411009789,48.5));
#80753=CARTESIAN_POINT('Ctrl Pts',(130.873396748677,3.60900411009789,48.35));
#80754=CARTESIAN_POINT('Ctrl Pts',(131.050477379933,3.60900411009789,48.35));
#80755=CARTESIAN_POINT('Ctrl Pts',(131.184038275853,3.5377217233181,48.35));
#80756=CARTESIAN_POINT('Ctrl Pts',(130.474965924397,3.47994545102119,48.5));
#80757=CARTESIAN_POINT('Ctrl Pts',(130.474965924397,3.47994545102119,48.35));
#80758=CARTESIAN_POINT('Ctrl Pts',(130.63328778185,3.60900411009789,48.5));
#80759=CARTESIAN_POINT('Ctrl Pts',(130.63328778185,3.60900411009789,48.35));
#80760=CARTESIAN_POINT('Ctrl Pts',(130.873396748677,3.60900411009789,48.5));
#80761=CARTESIAN_POINT('Ctrl Pts',(130.873396748677,3.60900411009789,48.35));
#80762=CARTESIAN_POINT('',(130.474965924397,3.47994545102119,48.5));
#80763=CARTESIAN_POINT('Ctrl Pts',(130.474965924397,3.47994545102119,48.5));
#80764=CARTESIAN_POINT('Ctrl Pts',(130.63328778185,3.60900411009789,48.5));
#80765=CARTESIAN_POINT('Ctrl Pts',(130.873396748677,3.60900411009789,48.5));
#80766=CARTESIAN_POINT('',(130.474965924397,3.47994545102119,48.35));
#80767=CARTESIAN_POINT('',(130.474965924397,3.47994545102119,48.5));
#80768=CARTESIAN_POINT('Ctrl Pts',(130.474965924397,3.47994545102119,48.35));
#80769=CARTESIAN_POINT('Ctrl Pts',(130.63328778185,3.60900411009789,48.35));
#80770=CARTESIAN_POINT('Ctrl Pts',(130.873396748677,3.60900411009789,48.35));
#80771=CARTESIAN_POINT('Ctrl Pts',(130.236357206479,3.11302864551544,48.5));
#80772=CARTESIAN_POINT('Ctrl Pts',(130.236357206479,3.11302864551544,48.35));
#80773=CARTESIAN_POINT('Ctrl Pts',(130.316643768921,3.3508867919445,48.5));
#80774=CARTESIAN_POINT('Ctrl Pts',(130.316643768921,3.3508867919445,48.35));
#80775=CARTESIAN_POINT('Ctrl Pts',(130.474965924397,3.47994545102119,48.5));
#80776=CARTESIAN_POINT('Ctrl Pts',(130.474965924397,3.47994545102119,48.35));
#80777=CARTESIAN_POINT('',(130.236357206479,3.11302864551544,48.5));
#80778=CARTESIAN_POINT('Ctrl Pts',(130.236357206479,3.11302864551544,48.5));
#80779=CARTESIAN_POINT('Ctrl Pts',(130.316643768921,3.3508867919445,48.5));
#80780=CARTESIAN_POINT('Ctrl Pts',(130.474965924397,3.47994545102119,48.5));
#80781=CARTESIAN_POINT('',(130.236357206479,3.11302864551544,48.35));
#80782=CARTESIAN_POINT('',(130.236357206479,3.11302864551544,48.5));
#80783=CARTESIAN_POINT('Ctrl Pts',(130.236357206479,3.11302864551544,48.35));
#80784=CARTESIAN_POINT('Ctrl Pts',(130.316643768921,3.3508867919445,48.35));
#80785=CARTESIAN_POINT('Ctrl Pts',(130.474965924397,3.47994545102119,48.35));
#80786=CARTESIAN_POINT('Ctrl Pts',(130.156070942059,2.48499327898026,48.5));
#80787=CARTESIAN_POINT('Ctrl Pts',(130.156070942059,2.48499327898026,48.35));
#80788=CARTESIAN_POINT('Ctrl Pts',(130.156070942059,2.87517049908638,48.5));
#80789=CARTESIAN_POINT('Ctrl Pts',(130.156070942059,2.87517049908638,48.35));
#80790=CARTESIAN_POINT('Ctrl Pts',(130.236357206479,3.11302864551544,48.5));
#80791=CARTESIAN_POINT('Ctrl Pts',(130.236357206479,3.11302864551544,48.35));
#80792=CARTESIAN_POINT('',(130.156070942059,2.48499327898026,48.5));
#80793=CARTESIAN_POINT('Ctrl Pts',(130.156070942059,2.48499327898026,48.5));
#80794=CARTESIAN_POINT('Ctrl Pts',(130.156070942059,2.87517049908638,48.5));
#80795=CARTESIAN_POINT('Ctrl Pts',(130.236357206479,3.11302864551544,48.5));
#80796=CARTESIAN_POINT('',(130.156070942059,2.48499327898026,48.35));
#80797=CARTESIAN_POINT('',(130.156070942059,2.48499327898026,48.5));
#80798=CARTESIAN_POINT('Ctrl Pts',(130.156070942059,2.48499327898026,48.35));
#80799=CARTESIAN_POINT('Ctrl Pts',(130.156070942059,2.87517049908638,48.35));
#80800=CARTESIAN_POINT('Ctrl Pts',(130.236357206479,3.11302864551544,48.35));
#80801=CARTESIAN_POINT('Ctrl Pts',(130.373669618741,1.59058684110642,48.5));
#80802=CARTESIAN_POINT('Ctrl Pts',(130.373669618741,1.59058684110642,48.35));
#80803=CARTESIAN_POINT('Ctrl Pts',(130.156070942059,1.86521166563034,48.5));
#80804=CARTESIAN_POINT('Ctrl Pts',(130.156070942059,1.86521166563034,48.35));
#80805=CARTESIAN_POINT('Ctrl Pts',(130.156070942059,2.48499327898026,48.5));
#80806=CARTESIAN_POINT('Ctrl Pts',(130.156070942059,2.48499327898026,48.35));
#80807=CARTESIAN_POINT('Ctrl Pts',(130.373669618741,1.59058684110642,48.5));
#80808=CARTESIAN_POINT('Ctrl Pts',(130.156070942059,1.86521166563034,48.5));
#80809=CARTESIAN_POINT('Ctrl Pts',(130.156070942059,2.48499327898026,48.5));
#80810=CARTESIAN_POINT('Ctrl Pts',(130.373669618741,1.59058684110642,48.35));
#80811=CARTESIAN_POINT('Ctrl Pts',(130.156070942059,1.86521166563034,48.35));
#80812=CARTESIAN_POINT('Ctrl Pts',(130.156070942059,2.48499327898026,48.35));
#80813=CARTESIAN_POINT('Origin',(129.999999681488,2.48574362695217,48.35));
#80814=CARTESIAN_POINT('Ctrl Pts',(128.901500606909,1.80593454837799,48.5));
#80815=CARTESIAN_POINT('Ctrl Pts',(128.901500606909,1.80593454837799,48.35));
#80816=CARTESIAN_POINT('Ctrl Pts',(128.83246918954,1.73315161466599,48.5));
#80817=CARTESIAN_POINT('Ctrl Pts',(128.83246918954,1.73315161466599,48.35));
#80818=CARTESIAN_POINT('Ctrl Pts',(128.787448758259,1.65961825847626,48.5));
#80819=CARTESIAN_POINT('Ctrl Pts',(128.787448758259,1.65961825847626,48.35));
#80820=CARTESIAN_POINT('',(128.901500606909,1.80593454837799,48.5));
#80821=CARTESIAN_POINT('',(128.787448758259,1.65961825847626,48.5));
#80822=CARTESIAN_POINT('Ctrl Pts',(128.901500606909,1.80593454837799,48.5));
#80823=CARTESIAN_POINT('Ctrl Pts',(128.83246918954,1.73315161466599,48.5));
#80824=CARTESIAN_POINT('Ctrl Pts',(128.787448758259,1.65961825847626,48.5));
#80825=CARTESIAN_POINT('',(128.901500606909,1.80593454837799,48.35));
#80826=CARTESIAN_POINT('',(128.901500606909,1.80593454837799,48.5));
#80827=CARTESIAN_POINT('',(128.787448758259,1.65961825847626,48.35));
#80828=CARTESIAN_POINT('Ctrl Pts',(128.901500606909,1.80593454837799,48.35));
#80829=CARTESIAN_POINT('Ctrl Pts',(128.83246918954,1.73315161466599,48.35));
#80830=CARTESIAN_POINT('Ctrl Pts',(128.787448758259,1.65961825847626,48.35));
#80831=CARTESIAN_POINT('',(128.787448758259,1.65961825847626,48.5));
#80832=CARTESIAN_POINT('Ctrl Pts',(129.213642532006,2.08281049132347,48.5));
#80833=CARTESIAN_POINT('Ctrl Pts',(129.213642532006,2.08281049132347,48.35));
#80834=CARTESIAN_POINT('Ctrl Pts',(128.970531875268,1.87871778011322,48.5));
#80835=CARTESIAN_POINT('Ctrl Pts',(128.970531875268,1.87871778011322,48.35));
#80836=CARTESIAN_POINT('Ctrl Pts',(128.901500606909,1.80593454837799,48.5));
#80837=CARTESIAN_POINT('Ctrl Pts',(128.901500606909,1.80593454837799,48.35));
#80838=CARTESIAN_POINT('',(129.213642532006,2.08281049132347,48.5));
#80839=CARTESIAN_POINT('Ctrl Pts',(129.213642532006,2.08281049132347,48.5));
#80840=CARTESIAN_POINT('Ctrl Pts',(128.970531875268,1.87871778011322,48.5));
#80841=CARTESIAN_POINT('Ctrl Pts',(128.901500606909,1.80593454837799,48.5));
#80842=CARTESIAN_POINT('',(129.213642532006,2.08281049132347,48.35));
#80843=CARTESIAN_POINT('',(129.213642532006,2.08281049132347,48.5));
#80844=CARTESIAN_POINT('Ctrl Pts',(129.213642532006,2.08281049132347,48.35));
#80845=CARTESIAN_POINT('Ctrl Pts',(128.970531875268,1.87871778011322,48.35));
#80846=CARTESIAN_POINT('Ctrl Pts',(128.901500606909,1.80593454837799,48.35));
#80847=CARTESIAN_POINT('Ctrl Pts',(129.630081707612,2.46998646855354,48.5));
#80848=CARTESIAN_POINT('Ctrl Pts',(129.630081707612,2.46998646855354,48.35));
#80849=CARTESIAN_POINT('Ctrl Pts',(129.5047748629,2.32892239093781,48.5));
#80850=CARTESIAN_POINT('Ctrl Pts',(129.5047748629,2.32892239093781,48.35));
#80851=CARTESIAN_POINT('Ctrl Pts',(129.213642532006,2.08281049132347,48.5));
#80852=CARTESIAN_POINT('Ctrl Pts',(129.213642532006,2.08281049132347,48.35));
#80853=CARTESIAN_POINT('',(129.630081707612,2.46998646855354,48.5));
#80854=CARTESIAN_POINT('Ctrl Pts',(129.630081707612,2.46998646855354,48.5));
#80855=CARTESIAN_POINT('Ctrl Pts',(129.5047748629,2.32892239093781,48.5));
#80856=CARTESIAN_POINT('Ctrl Pts',(129.213642532006,2.08281049132347,48.5));
#80857=CARTESIAN_POINT('',(129.630081707612,2.46998646855354,48.35));
#80858=CARTESIAN_POINT('',(129.630081707612,2.46998646855354,48.5));
#80859=CARTESIAN_POINT('Ctrl Pts',(129.630081707612,2.46998646855354,48.35));
#80860=CARTESIAN_POINT('Ctrl Pts',(129.5047748629,2.32892239093781,48.35));
#80861=CARTESIAN_POINT('Ctrl Pts',(129.213642532006,2.08281049132347,48.35));
#80862=CARTESIAN_POINT('Ctrl Pts',(129.809413308278,2.73860850930214,48.5));
#80863=CARTESIAN_POINT('Ctrl Pts',(129.809413308278,2.73860850930214,48.35));
#80864=CARTESIAN_POINT('Ctrl Pts',(129.755388850346,2.61105054616928,48.5));
#80865=CARTESIAN_POINT('Ctrl Pts',(129.755388850346,2.61105054616928,48.35));
#80866=CARTESIAN_POINT('Ctrl Pts',(129.630081707612,2.46998646855354,48.5));
#80867=CARTESIAN_POINT('Ctrl Pts',(129.630081707612,2.46998646855354,48.35));
#80868=CARTESIAN_POINT('',(129.809413308278,2.73860850930214,48.5));
#80869=CARTESIAN_POINT('Ctrl Pts',(129.809413308278,2.73860850930214,48.5));
#80870=CARTESIAN_POINT('Ctrl Pts',(129.755388850346,2.61105054616928,48.5));
#80871=CARTESIAN_POINT('Ctrl Pts',(129.630081707612,2.46998646855354,48.5));
#80872=CARTESIAN_POINT('',(129.809413308278,2.73860850930214,48.35));
#80873=CARTESIAN_POINT('',(129.809413308278,2.73860850930214,48.5));
#80874=CARTESIAN_POINT('Ctrl Pts',(129.809413308278,2.73860850930214,48.35));
#80875=CARTESIAN_POINT('Ctrl Pts',(129.755388850346,2.61105054616928,48.35));
#80876=CARTESIAN_POINT('Ctrl Pts',(129.630081707612,2.46998646855354,48.35));
#80877=CARTESIAN_POINT('Ctrl Pts',(129.863437766209,2.99822652339935,48.5));
#80878=CARTESIAN_POINT('Ctrl Pts',(129.863437766209,2.99822652339935,48.35));
#80879=CARTESIAN_POINT('Ctrl Pts',(129.863437766209,2.866166472435,48.5));
#80880=CARTESIAN_POINT('Ctrl Pts',(129.863437766209,2.866166472435,48.35));
#80881=CARTESIAN_POINT('Ctrl Pts',(129.809413308278,2.73860850930214,48.5));
#80882=CARTESIAN_POINT('Ctrl Pts',(129.809413308278,2.73860850930214,48.35));
#80883=CARTESIAN_POINT('',(129.863437766209,2.99822652339935,48.5));
#80884=CARTESIAN_POINT('Ctrl Pts',(129.863437766209,2.99822652339935,48.5));
#80885=CARTESIAN_POINT('Ctrl Pts',(129.863437766209,2.866166472435,48.5));
#80886=CARTESIAN_POINT('Ctrl Pts',(129.809413308278,2.73860850930214,48.5));
#80887=CARTESIAN_POINT('',(129.863437766209,2.99822652339935,48.35));
#80888=CARTESIAN_POINT('',(129.863437766209,2.99822652339935,48.5));
#80889=CARTESIAN_POINT('Ctrl Pts',(129.863437766209,2.99822652339935,48.35));
#80890=CARTESIAN_POINT('Ctrl Pts',(129.863437766209,2.866166472435,48.35));
#80891=CARTESIAN_POINT('Ctrl Pts',(129.809413308278,2.73860850930214,48.35));
#80892=CARTESIAN_POINT('Ctrl Pts',(129.678854102269,3.43342432379723,48.5));
#80893=CARTESIAN_POINT('Ctrl Pts',(129.678854102269,3.43342432379723,48.35));
#80894=CARTESIAN_POINT('Ctrl Pts',(129.863437766209,3.25784453749657,48.5));
#80895=CARTESIAN_POINT('Ctrl Pts',(129.863437766209,3.25784453749657,48.35));
#80896=CARTESIAN_POINT('Ctrl Pts',(129.863437766209,2.99822652339935,48.5));
#80897=CARTESIAN_POINT('Ctrl Pts',(129.863437766209,2.99822652339935,48.35));
#80898=CARTESIAN_POINT('',(129.678854102269,3.43342432379723,48.5));
#80899=CARTESIAN_POINT('Ctrl Pts',(129.678854102269,3.43342432379723,48.5));
#80900=CARTESIAN_POINT('Ctrl Pts',(129.863437766209,3.25784453749657,48.5));
#80901=CARTESIAN_POINT('Ctrl Pts',(129.863437766209,2.99822652339935,48.5));
#80902=CARTESIAN_POINT('',(129.678854102269,3.43342432379723,48.35));
#80903=CARTESIAN_POINT('',(129.678854102269,3.43342432379723,48.5));
#80904=CARTESIAN_POINT('Ctrl Pts',(129.678854102269,3.43342432379723,48.35));
#80905=CARTESIAN_POINT('Ctrl Pts',(129.863437766209,3.25784453749657,48.35));
#80906=CARTESIAN_POINT('Ctrl Pts',(129.863437766209,2.99822652339935,48.35));
#80907=CARTESIAN_POINT('Ctrl Pts',(129.177626127377,3.60900411009789,48.5));
#80908=CARTESIAN_POINT('Ctrl Pts',(129.177626127377,3.60900411009789,48.35));
#80909=CARTESIAN_POINT('Ctrl Pts',(129.494270140305,3.60900411009789,48.5));
#80910=CARTESIAN_POINT('Ctrl Pts',(129.494270140305,3.60900411009789,48.35));
#80911=CARTESIAN_POINT('Ctrl Pts',(129.678854102269,3.43342432379723,48.5));
#80912=CARTESIAN_POINT('Ctrl Pts',(129.678854102269,3.43342432379723,48.35));
#80913=CARTESIAN_POINT('',(129.177626127377,3.60900411009789,48.5));
#80914=CARTESIAN_POINT('Ctrl Pts',(129.177626127377,3.60900411009789,48.5));
#80915=CARTESIAN_POINT('Ctrl Pts',(129.494270140305,3.60900411009789,48.5));
#80916=CARTESIAN_POINT('Ctrl Pts',(129.678854102269,3.43342432379723,48.5));
#80917=CARTESIAN_POINT('',(129.177626127377,3.60900411009789,48.35));
#80918=CARTESIAN_POINT('',(129.177626127377,3.60900411009789,48.5));
#80919=CARTESIAN_POINT('Ctrl Pts',(129.177626127377,3.60900411009789,48.35));
#80920=CARTESIAN_POINT('Ctrl Pts',(129.494270140305,3.60900411009789,48.35));
#80921=CARTESIAN_POINT('Ctrl Pts',(129.678854102269,3.43342432379723,48.35));
#80922=CARTESIAN_POINT('Ctrl Pts',(128.677898997441,3.446180164814,48.5));
#80923=CARTESIAN_POINT('Ctrl Pts',(128.677898997441,3.446180164814,48.35));
#80924=CARTESIAN_POINT('Ctrl Pts',(128.863983506337,3.60900411009789,48.5));
#80925=CARTESIAN_POINT('Ctrl Pts',(128.863983506337,3.60900411009789,48.35));
#80926=CARTESIAN_POINT('Ctrl Pts',(129.177626127377,3.60900411009789,48.5));
#80927=CARTESIAN_POINT('Ctrl Pts',(129.177626127377,3.60900411009789,48.35));
#80928=CARTESIAN_POINT('',(128.677898997441,3.446180164814,48.5));
#80929=CARTESIAN_POINT('Ctrl Pts',(128.677898997441,3.446180164814,48.5));
#80930=CARTESIAN_POINT('Ctrl Pts',(128.863983506337,3.60900411009789,48.5));
#80931=CARTESIAN_POINT('Ctrl Pts',(129.177626127377,3.60900411009789,48.5));
#80932=CARTESIAN_POINT('',(128.677898997441,3.446180164814,48.35));
#80933=CARTESIAN_POINT('',(128.677898997441,3.446180164814,48.5));
#80934=CARTESIAN_POINT('Ctrl Pts',(128.677898997441,3.446180164814,48.35));
#80935=CARTESIAN_POINT('Ctrl Pts',(128.863983506337,3.60900411009789,48.35));
#80936=CARTESIAN_POINT('Ctrl Pts',(129.177626127377,3.60900411009789,48.35));
#80937=CARTESIAN_POINT('Ctrl Pts',(128.463301414624,2.97271499037743,48.5));
#80938=CARTESIAN_POINT('Ctrl Pts',(128.463301414624,2.97271499037743,48.35));
#80939=CARTESIAN_POINT('Ctrl Pts',(128.491814339533,3.28335621953011,48.5));
#80940=CARTESIAN_POINT('Ctrl Pts',(128.491814339533,3.28335621953011,48.35));
#80941=CARTESIAN_POINT('Ctrl Pts',(128.677898997441,3.446180164814,48.5));
#80942=CARTESIAN_POINT('Ctrl Pts',(128.677898997441,3.446180164814,48.35));
#80943=CARTESIAN_POINT('',(128.463301414624,2.97271499037743,48.5));
#80944=CARTESIAN_POINT('Ctrl Pts',(128.463301414624,2.97271499037743,48.5));
#80945=CARTESIAN_POINT('Ctrl Pts',(128.491814339533,3.28335621953011,48.5));
#80946=CARTESIAN_POINT('Ctrl Pts',(128.677898997441,3.446180164814,48.5));
#80947=CARTESIAN_POINT('',(128.463301414624,2.97271499037743,48.35));
#80948=CARTESIAN_POINT('',(128.463301414624,2.97271499037743,48.5));
#80949=CARTESIAN_POINT('Ctrl Pts',(128.463301414624,2.97271499037743,48.35));
#80950=CARTESIAN_POINT('Ctrl Pts',(128.491814339533,3.28335621953011,48.35));
#80951=CARTESIAN_POINT('Ctrl Pts',(128.677898997441,3.446180164814,48.35));
#80952=CARTESIAN_POINT('Origin',(128.740927631035,2.94420206546783,48.5));
#80953=CARTESIAN_POINT('',(128.740927631035,2.94420206546783,48.5));
#80954=CARTESIAN_POINT('',(64.7854329665245,9.51259549925474,48.5));
#80955=CARTESIAN_POINT('',(128.740927631035,2.94420206546783,48.35));
#80956=CARTESIAN_POINT('',(128.740927631035,2.94420206546783,48.5));
#80957=CARTESIAN_POINT('',(128.740927631035,2.94420206546783,48.35));
#80958=CARTESIAN_POINT('Ctrl Pts',(128.859481567517,3.26834926009178,48.5));
#80959=CARTESIAN_POINT('Ctrl Pts',(128.859481567517,3.26834926009178,48.35));
#80960=CARTESIAN_POINT('Ctrl Pts',(128.742428326979,3.15129616856575,48.5));
#80961=CARTESIAN_POINT('Ctrl Pts',(128.742428326979,3.15129616856575,48.35));
#80962=CARTESIAN_POINT('Ctrl Pts',(128.740927631035,2.94420206546783,48.5));
#80963=CARTESIAN_POINT('Ctrl Pts',(128.740927631035,2.94420206546783,48.35));
#80964=CARTESIAN_POINT('',(128.859481567517,3.26834926009178,48.5));
#80965=CARTESIAN_POINT('Ctrl Pts',(128.859481567517,3.26834926009178,48.5));
#80966=CARTESIAN_POINT('Ctrl Pts',(128.742428326979,3.15129616856575,48.5));
#80967=CARTESIAN_POINT('Ctrl Pts',(128.740927631035,2.94420206546783,48.5));
#80968=CARTESIAN_POINT('',(128.859481567517,3.26834926009178,48.35));
#80969=CARTESIAN_POINT('',(128.859481567517,3.26834926009178,48.5));
#80970=CARTESIAN_POINT('Ctrl Pts',(128.859481567517,3.26834926009178,48.35));
#80971=CARTESIAN_POINT('Ctrl Pts',(128.742428326979,3.15129616856575,48.35));
#80972=CARTESIAN_POINT('Ctrl Pts',(128.740927631035,2.94420206546783,48.35));
#80973=CARTESIAN_POINT('Ctrl Pts',(129.171623343602,3.38540250062943,48.5));
#80974=CARTESIAN_POINT('Ctrl Pts',(129.171623343602,3.38540250062943,48.35));
#80975=CARTESIAN_POINT('Ctrl Pts',(128.976534659043,3.38540250062943,48.5));
#80976=CARTESIAN_POINT('Ctrl Pts',(128.976534659043,3.38540250062943,48.35));
#80977=CARTESIAN_POINT('Ctrl Pts',(128.859481567517,3.26834926009178,48.5));
#80978=CARTESIAN_POINT('Ctrl Pts',(128.859481567517,3.26834926009178,48.35));
#80979=CARTESIAN_POINT('',(129.171623343602,3.38540250062943,48.5));
#80980=CARTESIAN_POINT('Ctrl Pts',(129.171623343602,3.38540250062943,48.5));
#80981=CARTESIAN_POINT('Ctrl Pts',(128.976534659043,3.38540250062943,48.5));
#80982=CARTESIAN_POINT('Ctrl Pts',(128.859481567517,3.26834926009178,48.5));
#80983=CARTESIAN_POINT('',(129.171623343602,3.38540250062943,48.35));
#80984=CARTESIAN_POINT('',(129.171623343602,3.38540250062943,48.5));
#80985=CARTESIAN_POINT('Ctrl Pts',(129.171623343602,3.38540250062943,48.35));
#80986=CARTESIAN_POINT('Ctrl Pts',(128.976534659043,3.38540250062943,48.35));
#80987=CARTESIAN_POINT('Ctrl Pts',(128.859481567517,3.26834926009178,48.35));
#80988=CARTESIAN_POINT('Ctrl Pts',(129.471009427682,3.27510246634483,48.5));
#80989=CARTESIAN_POINT('Ctrl Pts',(129.471009427682,3.27510246634483,48.35));
#80990=CARTESIAN_POINT('Ctrl Pts',(129.356207305565,3.38540250062943,48.5));
#80991=CARTESIAN_POINT('Ctrl Pts',(129.356207305565,3.38540250062943,48.35));
#80992=CARTESIAN_POINT('Ctrl Pts',(129.171623343602,3.38540250062943,48.5));
#80993=CARTESIAN_POINT('Ctrl Pts',(129.171623343602,3.38540250062943,48.35));
#80994=CARTESIAN_POINT('',(129.471009427682,3.27510246634483,48.5));
#80995=CARTESIAN_POINT('Ctrl Pts',(129.471009427682,3.27510246634483,48.5));
#80996=CARTESIAN_POINT('Ctrl Pts',(129.356207305565,3.38540250062943,48.5));
#80997=CARTESIAN_POINT('Ctrl Pts',(129.171623343602,3.38540250062943,48.5));
#80998=CARTESIAN_POINT('',(129.471009427682,3.27510246634483,48.35));
#80999=CARTESIAN_POINT('',(129.471009427682,3.27510246634483,48.5));
#81000=CARTESIAN_POINT('Ctrl Pts',(129.471009427682,3.27510246634483,48.35));
#81001=CARTESIAN_POINT('Ctrl Pts',(129.356207305565,3.38540250062943,48.35));
#81002=CARTESIAN_POINT('Ctrl Pts',(129.171623343602,3.38540250062943,48.35));
#81003=CARTESIAN_POINT('Ctrl Pts',(129.585811847821,3.00422930717468,48.5));
#81004=CARTESIAN_POINT('Ctrl Pts',(129.585811847821,3.00422930717468,48.35));
#81005=CARTESIAN_POINT('Ctrl Pts',(129.585811847821,3.16480228304863,48.5));
#81006=CARTESIAN_POINT('Ctrl Pts',(129.585811847821,3.16480228304863,48.35));
#81007=CARTESIAN_POINT('Ctrl Pts',(129.471009427682,3.27510246634483,48.5));
#81008=CARTESIAN_POINT('Ctrl Pts',(129.471009427682,3.27510246634483,48.35));
#81009=CARTESIAN_POINT('',(129.585811847821,3.00422930717468,48.5));
#81010=CARTESIAN_POINT('Ctrl Pts',(129.585811847821,3.00422930717468,48.5));
#81011=CARTESIAN_POINT('Ctrl Pts',(129.585811847821,3.16480228304863,48.5));
#81012=CARTESIAN_POINT('Ctrl Pts',(129.471009427682,3.27510246634483,48.5));
#81013=CARTESIAN_POINT('',(129.585811847821,3.00422930717468,48.35));
#81014=CARTESIAN_POINT('',(129.585811847821,3.00422930717468,48.5));
#81015=CARTESIAN_POINT('Ctrl Pts',(129.585811847821,3.00422930717468,48.35));
#81016=CARTESIAN_POINT('Ctrl Pts',(129.585811847821,3.16480228304863,48.35));
#81017=CARTESIAN_POINT('Ctrl Pts',(129.471009427682,3.27510246634483,48.35));
#81018=CARTESIAN_POINT('Ctrl Pts',(129.459754282609,2.6793315410614,48.5));
#81019=CARTESIAN_POINT('Ctrl Pts',(129.459754282609,2.6793315410614,48.35));
#81020=CARTESIAN_POINT('Ctrl Pts',(129.585811847821,2.85115966200829,48.5));
#81021=CARTESIAN_POINT('Ctrl Pts',(129.585811847821,2.85115966200829,48.35));
#81022=CARTESIAN_POINT('Ctrl Pts',(129.585811847821,3.00422930717468,48.5));
#81023=CARTESIAN_POINT('Ctrl Pts',(129.585811847821,3.00422930717468,48.35));
#81024=CARTESIAN_POINT('',(129.459754282609,2.6793315410614,48.5));
#81025=CARTESIAN_POINT('Ctrl Pts',(129.459754282609,2.6793315410614,48.5));
#81026=CARTESIAN_POINT('Ctrl Pts',(129.585811847821,2.85115966200829,48.5));
#81027=CARTESIAN_POINT('Ctrl Pts',(129.585811847821,3.00422930717468,48.5));
#81028=CARTESIAN_POINT('',(129.459754282609,2.6793315410614,48.35));
#81029=CARTESIAN_POINT('',(129.459754282609,2.6793315410614,48.5));
#81030=CARTESIAN_POINT('Ctrl Pts',(129.459754282609,2.6793315410614,48.35));
#81031=CARTESIAN_POINT('Ctrl Pts',(129.585811847821,2.85115966200829,48.35));
#81032=CARTESIAN_POINT('Ctrl Pts',(129.585811847821,3.00422930717468,48.35));
#81033=CARTESIAN_POINT('Ctrl Pts',(128.975034112111,2.21336984634399,48.5));
#81034=CARTESIAN_POINT('Ctrl Pts',(128.975034112111,2.21336984634399,48.35));
#81035=CARTESIAN_POINT('Ctrl Pts',(129.33369701542,2.50750356912613,48.5));
#81036=CARTESIAN_POINT('Ctrl Pts',(129.33369701542,2.50750356912613,48.35));
#81037=CARTESIAN_POINT('Ctrl Pts',(129.459754282609,2.6793315410614,48.5));
#81038=CARTESIAN_POINT('Ctrl Pts',(129.459754282609,2.6793315410614,48.35));
#81039=CARTESIAN_POINT('',(128.975034112111,2.21336984634399,48.5));
#81040=CARTESIAN_POINT('Ctrl Pts',(128.975034112111,2.21336984634399,48.5));
#81041=CARTESIAN_POINT('Ctrl Pts',(129.33369701542,2.50750356912613,48.5));
#81042=CARTESIAN_POINT('Ctrl Pts',(129.459754282609,2.6793315410614,48.5));
#81043=CARTESIAN_POINT('',(128.975034112111,2.21336984634399,48.35));
#81044=CARTESIAN_POINT('',(128.975034112111,2.21336984634399,48.5));
#81045=CARTESIAN_POINT('Ctrl Pts',(128.975034112111,2.21336984634399,48.35));
#81046=CARTESIAN_POINT('Ctrl Pts',(129.33369701542,2.50750356912613,48.35));
#81047=CARTESIAN_POINT('Ctrl Pts',(129.459754282609,2.6793315410614,48.35));
#81048=CARTESIAN_POINT('Ctrl Pts',(128.621623421088,1.88021832704544,48.5));
#81049=CARTESIAN_POINT('Ctrl Pts',(128.621623421088,1.88021832704544,48.35));
#81050=CARTESIAN_POINT('Ctrl Pts',(128.743929022923,2.02428394556046,48.5));
#81051=CARTESIAN_POINT('Ctrl Pts',(128.743929022923,2.02428394556046,48.35));
#81052=CARTESIAN_POINT('Ctrl Pts',(128.975034112111,2.21336984634399,48.5));
#81053=CARTESIAN_POINT('Ctrl Pts',(128.975034112111,2.21336984634399,48.35));
#81054=CARTESIAN_POINT('',(128.621623421088,1.88021832704544,48.5));
#81055=CARTESIAN_POINT('Ctrl Pts',(128.621623421088,1.88021832704544,48.5));
#81056=CARTESIAN_POINT('Ctrl Pts',(128.743929022923,2.02428394556046,48.5));
#81057=CARTESIAN_POINT('Ctrl Pts',(128.975034112111,2.21336984634399,48.5));
#81058=CARTESIAN_POINT('',(128.621623421088,1.88021832704544,48.35));
#81059=CARTESIAN_POINT('',(128.621623421088,1.88021832704544,48.5));
#81060=CARTESIAN_POINT('Ctrl Pts',(128.621623421088,1.88021832704544,48.35));
#81061=CARTESIAN_POINT('Ctrl Pts',(128.743929022923,2.02428394556046,48.35));
#81062=CARTESIAN_POINT('Ctrl Pts',(128.975034112111,2.21336984634399,48.35));
#81063=CARTESIAN_POINT('Ctrl Pts',(128.443792516366,1.58758544921875,48.5));
#81064=CARTESIAN_POINT('Ctrl Pts',(128.443792516366,1.58758544921875,48.35));
#81065=CARTESIAN_POINT('Ctrl Pts',(128.499317819253,1.73615300655365,48.5));
#81066=CARTESIAN_POINT('Ctrl Pts',(128.499317819253,1.73615300655365,48.35));
#81067=CARTESIAN_POINT('Ctrl Pts',(128.621623421088,1.88021832704544,48.5));
#81068=CARTESIAN_POINT('Ctrl Pts',(128.621623421088,1.88021832704544,48.35));
#81069=CARTESIAN_POINT('',(128.443792516366,1.58758544921875,48.5));
#81070=CARTESIAN_POINT('Ctrl Pts',(128.443792516366,1.58758544921875,48.5));
#81071=CARTESIAN_POINT('Ctrl Pts',(128.499317819253,1.73615300655365,48.5));
#81072=CARTESIAN_POINT('Ctrl Pts',(128.621623421088,1.88021832704544,48.5));
#81073=CARTESIAN_POINT('',(128.443792516366,1.58758544921875,48.35));
#81074=CARTESIAN_POINT('',(128.443792516366,1.58758544921875,48.5));
#81075=CARTESIAN_POINT('Ctrl Pts',(128.443792516366,1.58758544921875,48.35));
#81076=CARTESIAN_POINT('Ctrl Pts',(128.499317819253,1.73615300655365,48.35));
#81077=CARTESIAN_POINT('Ctrl Pts',(128.621623421088,1.88021832704544,48.35));
#81078=CARTESIAN_POINT('Ctrl Pts',(128.412278199568,1.40000009536743,48.5));
#81079=CARTESIAN_POINT('Ctrl Pts',(128.412278199568,1.40000009536743,48.35));
#81080=CARTESIAN_POINT('Ctrl Pts',(128.409276807681,1.49754428863525,48.5));
#81081=CARTESIAN_POINT('Ctrl Pts',(128.409276807681,1.49754428863525,48.35));
#81082=CARTESIAN_POINT('Ctrl Pts',(128.443792516366,1.58758544921875,48.5));
#81083=CARTESIAN_POINT('Ctrl Pts',(128.443792516366,1.58758544921875,48.35));
#81084=CARTESIAN_POINT('',(128.412278199568,1.40000009536743,48.5));
#81085=CARTESIAN_POINT('Ctrl Pts',(128.412278199568,1.40000009536743,48.5));
#81086=CARTESIAN_POINT('Ctrl Pts',(128.409276807681,1.49754428863525,48.5));
#81087=CARTESIAN_POINT('Ctrl Pts',(128.443792516366,1.58758544921875,48.5));
#81088=CARTESIAN_POINT('',(128.412278199568,1.40000009536743,48.35));
#81089=CARTESIAN_POINT('',(128.412278199568,1.40000009536743,48.5));
#81090=CARTESIAN_POINT('Ctrl Pts',(128.412278199568,1.40000009536743,48.35));
#81091=CARTESIAN_POINT('Ctrl Pts',(128.409276807681,1.49754428863525,48.35));
#81092=CARTESIAN_POINT('Ctrl Pts',(128.443792516366,1.58758544921875,48.35));
#81093=CARTESIAN_POINT('Origin',(129.866439158097,1.40000009536743,48.5));
#81094=CARTESIAN_POINT('',(129.866439158097,1.40000009536743,48.5));
#81095=CARTESIAN_POINT('',(64.9332195790485,1.40000009536743,48.5));
#81096=CARTESIAN_POINT('',(129.866439158097,1.40000009536743,48.35));
#81097=CARTESIAN_POINT('',(129.866439158097,1.40000009536743,48.5));
#81098=CARTESIAN_POINT('',(129.866439158097,1.40000009536743,48.35));
#81099=CARTESIAN_POINT('Origin',(129.866439158097,1.65961825847626,48.5));
#81100=CARTESIAN_POINT('',(129.866439158097,1.65961825847626,48.5));
#81101=CARTESIAN_POINT('',(129.866439158097,4.82980912923813,48.5));
#81102=CARTESIAN_POINT('',(129.866439158097,1.65961825847626,48.35));
#81103=CARTESIAN_POINT('',(129.866439158097,1.65961825847626,48.5));
#81104=CARTESIAN_POINT('',(129.866439158097,1.65961825847626,48.35));
#81105=CARTESIAN_POINT('Origin',(128.787448758259,1.65961825847626,48.5));
#81106=CARTESIAN_POINT('',(64.3937243791297,1.65961825847626,48.5));
#81107=CARTESIAN_POINT('',(128.787448758259,1.65961825847626,48.35));
#81108=CARTESIAN_POINT('Origin',(129.999999681488,2.48574362695217,48.35));
#81109=CARTESIAN_POINT('Origin',(0.,8.,48.5));
#81110=CARTESIAN_POINT('Ctrl Pts',(120.748090229928,3.38540250062943,48.5));
#81111=CARTESIAN_POINT('Ctrl Pts',(120.748090229928,3.38540250062943,48.35));
#81112=CARTESIAN_POINT('Ctrl Pts',(120.562005423009,3.38540250062943,48.5));
#81113=CARTESIAN_POINT('Ctrl Pts',(120.562005423009,3.38540250062943,48.35));
#81114=CARTESIAN_POINT('Ctrl Pts',(120.450955115259,3.22783091664314,48.5));
#81115=CARTESIAN_POINT('Ctrl Pts',(120.450955115259,3.22783091664314,48.35));
#81116=CARTESIAN_POINT('',(120.748090229928,3.38540250062943,48.5));
#81117=CARTESIAN_POINT('',(120.450955115259,3.22783091664314,48.5));
#81118=CARTESIAN_POINT('Ctrl Pts',(120.748090229928,3.38540250062943,48.5));
#81119=CARTESIAN_POINT('Ctrl Pts',(120.562005423009,3.38540250062943,48.5));
#81120=CARTESIAN_POINT('Ctrl Pts',(120.450955115259,3.22783091664314,48.5));
#81121=CARTESIAN_POINT('',(120.748090229928,3.38540250062943,48.35));
#81122=CARTESIAN_POINT('',(120.748090229928,3.38540250062943,48.5));
#81123=CARTESIAN_POINT('',(120.450955115259,3.22783091664314,48.35));
#81124=CARTESIAN_POINT('Ctrl Pts',(120.748090229928,3.38540250062943,48.35));
#81125=CARTESIAN_POINT('Ctrl Pts',(120.562005423009,3.38540250062943,48.35));
#81126=CARTESIAN_POINT('Ctrl Pts',(120.450955115259,3.22783091664314,48.35));
#81127=CARTESIAN_POINT('',(120.450955115259,3.22783091664314,48.5));
#81128=CARTESIAN_POINT('Ctrl Pts',(121.063983522356,3.2068213224411,48.5));
#81129=CARTESIAN_POINT('Ctrl Pts',(121.063983522356,3.2068213224411,48.35));
#81130=CARTESIAN_POINT('Ctrl Pts',(120.937175832689,3.38540250062943,48.5));
#81131=CARTESIAN_POINT('Ctrl Pts',(120.937175832689,3.38540250062943,48.35));
#81132=CARTESIAN_POINT('Ctrl Pts',(120.748090229928,3.38540250062943,48.5));
#81133=CARTESIAN_POINT('Ctrl Pts',(120.748090229928,3.38540250062943,48.35));
#81134=CARTESIAN_POINT('',(121.063983522356,3.2068213224411,48.5));
#81135=CARTESIAN_POINT('Ctrl Pts',(121.063983522356,3.2068213224411,48.5));
#81136=CARTESIAN_POINT('Ctrl Pts',(120.937175832689,3.38540250062943,48.5));
#81137=CARTESIAN_POINT('Ctrl Pts',(120.748090229928,3.38540250062943,48.5));
#81138=CARTESIAN_POINT('',(121.063983522356,3.2068213224411,48.35));
#81139=CARTESIAN_POINT('',(121.063983522356,3.2068213224411,48.5));
#81140=CARTESIAN_POINT('Ctrl Pts',(121.063983522356,3.2068213224411,48.35));
#81141=CARTESIAN_POINT('Ctrl Pts',(120.937175832689,3.38540250062943,48.35));
#81142=CARTESIAN_POINT('Ctrl Pts',(120.748090229928,3.38540250062943,48.35));
#81143=CARTESIAN_POINT('Ctrl Pts',(121.190791212022,2.48499327898026,48.5));
#81144=CARTESIAN_POINT('Ctrl Pts',(121.190791212022,2.48499327898026,48.35));
#81145=CARTESIAN_POINT('Ctrl Pts',(121.190791212022,3.02824014425278,48.5));
#81146=CARTESIAN_POINT('Ctrl Pts',(121.190791212022,3.02824014425278,48.35));
#81147=CARTESIAN_POINT('Ctrl Pts',(121.063983522356,3.2068213224411,48.5));
#81148=CARTESIAN_POINT('Ctrl Pts',(121.063983522356,3.2068213224411,48.35));
#81149=CARTESIAN_POINT('',(121.190791212022,2.48499327898026,48.5));
#81150=CARTESIAN_POINT('Ctrl Pts',(121.190791212022,2.48499327898026,48.5));
#81151=CARTESIAN_POINT('Ctrl Pts',(121.190791212022,3.02824014425278,48.5));
#81152=CARTESIAN_POINT('Ctrl Pts',(121.063983522356,3.2068213224411,48.5));
#81153=CARTESIAN_POINT('',(121.190791212022,2.48499327898026,48.35));
#81154=CARTESIAN_POINT('',(121.190791212022,2.48499327898026,48.5));
#81155=CARTESIAN_POINT('Ctrl Pts',(121.190791212022,2.48499327898026,48.35));
#81156=CARTESIAN_POINT('Ctrl Pts',(121.190791212022,3.02824014425278,48.35));
#81157=CARTESIAN_POINT('Ctrl Pts',(121.063983522356,3.2068213224411,48.35));
#81158=CARTESIAN_POINT('Ctrl Pts',(121.063983522356,1.76466578245163,48.5));
#81159=CARTESIAN_POINT('Ctrl Pts',(121.063983522356,1.76466578245163,48.35));
#81160=CARTESIAN_POINT('Ctrl Pts',(121.190791212022,1.9447478055954,48.5));
#81161=CARTESIAN_POINT('Ctrl Pts',(121.190791212022,1.9447478055954,48.35));
#81162=CARTESIAN_POINT('Ctrl Pts',(121.190791212022,2.48499327898026,48.5));
#81163=CARTESIAN_POINT('Ctrl Pts',(121.190791212022,2.48499327898026,48.35));
#81164=CARTESIAN_POINT('',(121.063983522356,1.76466578245163,48.5));
#81165=CARTESIAN_POINT('Ctrl Pts',(121.063983522356,1.76466578245163,48.5));
#81166=CARTESIAN_POINT('Ctrl Pts',(121.190791212022,1.9447478055954,48.5));
#81167=CARTESIAN_POINT('Ctrl Pts',(121.190791212022,2.48499327898026,48.5));
#81168=CARTESIAN_POINT('',(121.063983522356,1.76466578245163,48.35));
#81169=CARTESIAN_POINT('',(121.063983522356,1.76466578245163,48.5));
#81170=CARTESIAN_POINT('Ctrl Pts',(121.063983522356,1.76466578245163,48.35));
#81171=CARTESIAN_POINT('Ctrl Pts',(121.190791212022,1.9447478055954,48.35));
#81172=CARTESIAN_POINT('Ctrl Pts',(121.190791212022,2.48499327898026,48.35));
#81173=CARTESIAN_POINT('Ctrl Pts',(120.751091323793,1.58458405733109,48.5));
#81174=CARTESIAN_POINT('Ctrl Pts',(120.751091323793,1.58458405733109,48.35));
#81175=CARTESIAN_POINT('Ctrl Pts',(120.937175832689,1.58458405733109,48.5));
#81176=CARTESIAN_POINT('Ctrl Pts',(120.937175832689,1.58458405733109,48.35));
#81177=CARTESIAN_POINT('Ctrl Pts',(121.063983522356,1.76466578245163,48.5));
#81178=CARTESIAN_POINT('Ctrl Pts',(121.063983522356,1.76466578245163,48.35));
#81179=CARTESIAN_POINT('',(120.751091323793,1.58458405733109,48.5));
#81180=CARTESIAN_POINT('Ctrl Pts',(120.751091323793,1.58458405733109,48.5));
#81181=CARTESIAN_POINT('Ctrl Pts',(120.937175832689,1.58458405733109,48.5));
#81182=CARTESIAN_POINT('Ctrl Pts',(121.063983522356,1.76466578245163,48.5));
#81183=CARTESIAN_POINT('',(120.751091323793,1.58458405733109,48.35));
#81184=CARTESIAN_POINT('',(120.751091323793,1.58458405733109,48.5));
#81185=CARTESIAN_POINT('Ctrl Pts',(120.751091323793,1.58458405733109,48.35));
#81186=CARTESIAN_POINT('Ctrl Pts',(120.937175832689,1.58458405733109,48.35));
#81187=CARTESIAN_POINT('Ctrl Pts',(121.063983522356,1.76466578245163,48.35));
#81188=CARTESIAN_POINT('Ctrl Pts',(120.43819912523,1.76391565799713,48.5));
#81189=CARTESIAN_POINT('Ctrl Pts',(120.43819912523,1.76391565799713,48.35));
#81190=CARTESIAN_POINT('Ctrl Pts',(120.565006814897,1.58458405733109,48.5));
#81191=CARTESIAN_POINT('Ctrl Pts',(120.565006814897,1.58458405733109,48.35));
#81192=CARTESIAN_POINT('Ctrl Pts',(120.751091323793,1.58458405733109,48.5));
#81193=CARTESIAN_POINT('Ctrl Pts',(120.751091323793,1.58458405733109,48.35));
#81194=CARTESIAN_POINT('',(120.43819912523,1.76391565799713,48.5));
#81195=CARTESIAN_POINT('Ctrl Pts',(120.43819912523,1.76391565799713,48.5));
#81196=CARTESIAN_POINT('Ctrl Pts',(120.565006814897,1.58458405733109,48.5));
#81197=CARTESIAN_POINT('Ctrl Pts',(120.751091323793,1.58458405733109,48.5));
#81198=CARTESIAN_POINT('',(120.43819912523,1.76391565799713,48.35));
#81199=CARTESIAN_POINT('',(120.43819912523,1.76391565799713,48.5));
#81200=CARTESIAN_POINT('Ctrl Pts',(120.43819912523,1.76391565799713,48.35));
#81201=CARTESIAN_POINT('Ctrl Pts',(120.565006814897,1.58458405733109,48.35));
#81202=CARTESIAN_POINT('Ctrl Pts',(120.751091323793,1.58458405733109,48.35));
#81203=CARTESIAN_POINT('Ctrl Pts',(120.311391435564,2.48499327898026,48.5));
#81204=CARTESIAN_POINT('Ctrl Pts',(120.311391435564,2.48499327898026,48.35));
#81205=CARTESIAN_POINT('Ctrl Pts',(120.311391435564,1.94324696063995,48.5));
#81206=CARTESIAN_POINT('Ctrl Pts',(120.311391435564,1.94324696063995,48.35));
#81207=CARTESIAN_POINT('Ctrl Pts',(120.43819912523,1.76391565799713,48.5));
#81208=CARTESIAN_POINT('Ctrl Pts',(120.43819912523,1.76391565799713,48.35));
#81209=CARTESIAN_POINT('',(120.311391435564,2.48499327898026,48.5));
#81210=CARTESIAN_POINT('Ctrl Pts',(120.311391435564,2.48499327898026,48.5));
#81211=CARTESIAN_POINT('Ctrl Pts',(120.311391435564,1.94324696063995,48.5));
#81212=CARTESIAN_POINT('Ctrl Pts',(120.43819912523,1.76391565799713,48.5));
#81213=CARTESIAN_POINT('',(120.311391435564,2.48499327898026,48.35));
#81214=CARTESIAN_POINT('',(120.311391435564,2.48499327898026,48.5));
#81215=CARTESIAN_POINT('Ctrl Pts',(120.311391435564,2.48499327898026,48.35));
#81216=CARTESIAN_POINT('Ctrl Pts',(120.311391435564,1.94324696063995,48.35));
#81217=CARTESIAN_POINT('Ctrl Pts',(120.43819912523,1.76391565799713,48.35));
#81218=CARTESIAN_POINT('Ctrl Pts',(120.450955115259,3.22783091664314,48.5));
#81219=CARTESIAN_POINT('Ctrl Pts',(120.450955115259,3.22783091664314,48.35));
#81220=CARTESIAN_POINT('Ctrl Pts',(120.311391435564,3.02673944830894,48.5));
#81221=CARTESIAN_POINT('Ctrl Pts',(120.311391435564,3.02673944830894,48.35));
#81222=CARTESIAN_POINT('Ctrl Pts',(120.311391435564,2.48499327898026,48.5));
#81223=CARTESIAN_POINT('Ctrl Pts',(120.311391435564,2.48499327898026,48.35));
#81224=CARTESIAN_POINT('Ctrl Pts',(120.450955115259,3.22783091664314,48.5));
#81225=CARTESIAN_POINT('Ctrl Pts',(120.311391435564,3.02673944830894,48.5));
#81226=CARTESIAN_POINT('Ctrl Pts',(120.311391435564,2.48499327898026,48.5));
#81227=CARTESIAN_POINT('Ctrl Pts',(120.450955115259,3.22783091664314,48.35));
#81228=CARTESIAN_POINT('Ctrl Pts',(120.311391435564,3.02673944830894,48.35));
#81229=CARTESIAN_POINT('Ctrl Pts',(120.311391435564,2.48499327898026,48.35));
#81230=CARTESIAN_POINT('Ctrl Pts',(120.751091323793,1.36248314380646,48.5));
#81231=CARTESIAN_POINT('Ctrl Pts',(120.751091323793,1.36248314380646,48.35));
#81232=CARTESIAN_POINT('Ctrl Pts',(120.432946763933,1.36248314380646,48.5));
#81233=CARTESIAN_POINT('Ctrl Pts',(120.432946763933,1.36248314380646,48.35));
#81234=CARTESIAN_POINT('Ctrl Pts',(120.251364193857,1.59058684110642,48.5));
#81235=CARTESIAN_POINT('Ctrl Pts',(120.251364193857,1.59058684110642,48.35));
#81236=CARTESIAN_POINT('',(120.751091323793,1.36248314380646,48.5));
#81237=CARTESIAN_POINT('',(120.251364193857,1.59058684110642,48.5));
#81238=CARTESIAN_POINT('Ctrl Pts',(120.751091323793,1.36248314380646,48.5));
#81239=CARTESIAN_POINT('Ctrl Pts',(120.432946763933,1.36248314380646,48.5));
#81240=CARTESIAN_POINT('Ctrl Pts',(120.251364193857,1.59058684110642,48.5));
#81241=CARTESIAN_POINT('',(120.751091323793,1.36248314380646,48.35));
#81242=CARTESIAN_POINT('',(120.751091323793,1.36248314380646,48.5));
#81243=CARTESIAN_POINT('',(120.251364193857,1.59058684110642,48.35));
#81244=CARTESIAN_POINT('Ctrl Pts',(120.751091323793,1.36248314380646,48.35));
#81245=CARTESIAN_POINT('Ctrl Pts',(120.432946763933,1.36248314380646,48.35));
#81246=CARTESIAN_POINT('Ctrl Pts',(120.251364193857,1.59058684110642,48.35));
#81247=CARTESIAN_POINT('',(120.251364193857,1.59058684110642,48.5));
#81248=CARTESIAN_POINT('Ctrl Pts',(121.151022993028,1.49229192733765,48.5));
#81249=CARTESIAN_POINT('Ctrl Pts',(121.151022993028,1.49229192733765,48.35));
#81250=CARTESIAN_POINT('Ctrl Pts',(120.992701135576,1.36248314380646,48.5));
#81251=CARTESIAN_POINT('Ctrl Pts',(120.992701135576,1.36248314380646,48.35));
#81252=CARTESIAN_POINT('Ctrl Pts',(120.751091323793,1.36248314380646,48.5));
#81253=CARTESIAN_POINT('Ctrl Pts',(120.751091323793,1.36248314380646,48.35));
#81254=CARTESIAN_POINT('',(121.151022993028,1.49229192733765,48.5));
#81255=CARTESIAN_POINT('Ctrl Pts',(121.151022993028,1.49229192733765,48.5));
#81256=CARTESIAN_POINT('Ctrl Pts',(120.992701135576,1.36248314380646,48.5));
#81257=CARTESIAN_POINT('Ctrl Pts',(120.751091323793,1.36248314380646,48.5));
#81258=CARTESIAN_POINT('',(121.151022993028,1.49229192733765,48.35));
#81259=CARTESIAN_POINT('',(121.151022993028,1.49229192733765,48.5));
#81260=CARTESIAN_POINT('Ctrl Pts',(121.151022993028,1.49229192733765,48.35));
#81261=CARTESIAN_POINT('Ctrl Pts',(120.992701135576,1.36248314380646,48.35));
#81262=CARTESIAN_POINT('Ctrl Pts',(120.751091323793,1.36248314380646,48.35));
#81263=CARTESIAN_POINT('Ctrl Pts',(121.388881288469,1.85995900630951,48.5));
#81264=CARTESIAN_POINT('Ctrl Pts',(121.388881288469,1.85995900630951,48.35));
#81265=CARTESIAN_POINT('Ctrl Pts',(121.309344850481,1.62210100889206,48.5));
#81266=CARTESIAN_POINT('Ctrl Pts',(121.309344850481,1.62210100889206,48.35));
#81267=CARTESIAN_POINT('Ctrl Pts',(121.151022993028,1.49229192733765,48.5));
#81268=CARTESIAN_POINT('Ctrl Pts',(121.151022993028,1.49229192733765,48.35));
#81269=CARTESIAN_POINT('',(121.388881288469,1.85995900630951,48.5));
#81270=CARTESIAN_POINT('Ctrl Pts',(121.388881288469,1.85995900630951,48.5));
#81271=CARTESIAN_POINT('Ctrl Pts',(121.309344850481,1.62210100889206,48.5));
#81272=CARTESIAN_POINT('Ctrl Pts',(121.151022993028,1.49229192733765,48.5));
#81273=CARTESIAN_POINT('',(121.388881288469,1.85995900630951,48.35));
#81274=CARTESIAN_POINT('',(121.388881288469,1.85995900630951,48.5));
#81275=CARTESIAN_POINT('Ctrl Pts',(121.388881288469,1.85995900630951,48.35));
#81276=CARTESIAN_POINT('Ctrl Pts',(121.309344850481,1.62210100889206,48.35));
#81277=CARTESIAN_POINT('Ctrl Pts',(121.151022993028,1.49229192733765,48.35));
#81278=CARTESIAN_POINT('Ctrl Pts',(121.468417130411,2.48499327898026,48.5));
#81279=CARTESIAN_POINT('Ctrl Pts',(121.468417130411,2.48499327898026,48.35));
#81280=CARTESIAN_POINT('Ctrl Pts',(121.468417130411,2.09781730175018,48.5));
#81281=CARTESIAN_POINT('Ctrl Pts',(121.468417130411,2.09781730175018,48.35));
#81282=CARTESIAN_POINT('Ctrl Pts',(121.388881288469,1.85995900630951,48.5));
#81283=CARTESIAN_POINT('Ctrl Pts',(121.388881288469,1.85995900630951,48.35));
#81284=CARTESIAN_POINT('',(121.468417130411,2.48499327898026,48.5));
#81285=CARTESIAN_POINT('Ctrl Pts',(121.468417130411,2.48499327898026,48.5));
#81286=CARTESIAN_POINT('Ctrl Pts',(121.468417130411,2.09781730175018,48.5));
#81287=CARTESIAN_POINT('Ctrl Pts',(121.388881288469,1.85995900630951,48.5));
#81288=CARTESIAN_POINT('',(121.468417130411,2.48499327898026,48.35));
#81289=CARTESIAN_POINT('',(121.468417130411,2.48499327898026,48.5));
#81290=CARTESIAN_POINT('Ctrl Pts',(121.468417130411,2.48499327898026,48.35));
#81291=CARTESIAN_POINT('Ctrl Pts',(121.468417130411,2.09781730175018,48.35));
#81292=CARTESIAN_POINT('Ctrl Pts',(121.388881288469,1.85995900630951,48.35));
#81293=CARTESIAN_POINT('Ctrl Pts',(121.418894611299,3.00497958064079,48.5));
#81294=CARTESIAN_POINT('Ctrl Pts',(121.418894611299,3.00497958064079,48.35));
#81295=CARTESIAN_POINT('Ctrl Pts',(121.468417130411,2.81214186549187,48.5));
#81296=CARTESIAN_POINT('Ctrl Pts',(121.468417130411,2.81214186549187,48.35));
#81297=CARTESIAN_POINT('Ctrl Pts',(121.468417130411,2.48499327898026,48.5));
#81298=CARTESIAN_POINT('Ctrl Pts',(121.468417130411,2.48499327898026,48.35));
#81299=CARTESIAN_POINT('',(121.418894611299,3.00497958064079,48.5));
#81300=CARTESIAN_POINT('Ctrl Pts',(121.418894611299,3.00497958064079,48.5));
#81301=CARTESIAN_POINT('Ctrl Pts',(121.468417130411,2.81214186549187,48.5));
#81302=CARTESIAN_POINT('Ctrl Pts',(121.468417130411,2.48499327898026,48.5));
#81303=CARTESIAN_POINT('',(121.418894611299,3.00497958064079,48.35));
#81304=CARTESIAN_POINT('',(121.418894611299,3.00497958064079,48.5));
#81305=CARTESIAN_POINT('Ctrl Pts',(121.418894611299,3.00497958064079,48.35));
#81306=CARTESIAN_POINT('Ctrl Pts',(121.468417130411,2.81214186549187,48.35));
#81307=CARTESIAN_POINT('Ctrl Pts',(121.468417130411,2.48499327898026,48.35));
#81308=CARTESIAN_POINT('Ctrl Pts',(121.282332621515,3.33212831616402,48.5));
#81309=CARTESIAN_POINT('Ctrl Pts',(121.282332621515,3.33212831616402,48.35));
#81310=CARTESIAN_POINT('Ctrl Pts',(121.369372092187,3.19781729578972,48.5));
#81311=CARTESIAN_POINT('Ctrl Pts',(121.369372092187,3.19781729578972,48.35));
#81312=CARTESIAN_POINT('Ctrl Pts',(121.418894611299,3.00497958064079,48.5));
#81313=CARTESIAN_POINT('Ctrl Pts',(121.418894611299,3.00497958064079,48.35));
#81314=CARTESIAN_POINT('',(121.282332621515,3.33212831616402,48.5));
#81315=CARTESIAN_POINT('Ctrl Pts',(121.282332621515,3.33212831616402,48.5));
#81316=CARTESIAN_POINT('Ctrl Pts',(121.369372092187,3.19781729578972,48.5));
#81317=CARTESIAN_POINT('Ctrl Pts',(121.418894611299,3.00497958064079,48.5));
#81318=CARTESIAN_POINT('',(121.282332621515,3.33212831616402,48.35));
#81319=CARTESIAN_POINT('',(121.282332621515,3.33212831616402,48.5));
#81320=CARTESIAN_POINT('Ctrl Pts',(121.282332621515,3.33212831616402,48.35));
#81321=CARTESIAN_POINT('Ctrl Pts',(121.369372092187,3.19781729578972,48.35));
#81322=CARTESIAN_POINT('Ctrl Pts',(121.418894611299,3.00497958064079,48.35));
#81323=CARTESIAN_POINT('Ctrl Pts',(121.061732850969,3.5377217233181,48.5));
#81324=CARTESIAN_POINT('Ctrl Pts',(121.061732850969,3.5377217233181,48.35));
#81325=CARTESIAN_POINT('Ctrl Pts',(121.195293150842,3.46643933653831,48.5));
#81326=CARTESIAN_POINT('Ctrl Pts',(121.195293150842,3.46643933653831,48.35));
#81327=CARTESIAN_POINT('Ctrl Pts',(121.282332621515,3.33212831616402,48.5));
#81328=CARTESIAN_POINT('Ctrl Pts',(121.282332621515,3.33212831616402,48.35));
#81329=CARTESIAN_POINT('',(121.061732850969,3.5377217233181,48.5));
#81330=CARTESIAN_POINT('Ctrl Pts',(121.061732850969,3.5377217233181,48.5));
#81331=CARTESIAN_POINT('Ctrl Pts',(121.195293150842,3.46643933653831,48.5));
#81332=CARTESIAN_POINT('Ctrl Pts',(121.282332621515,3.33212831616402,48.5));
#81333=CARTESIAN_POINT('',(121.061732850969,3.5377217233181,48.35));
#81334=CARTESIAN_POINT('',(121.061732850969,3.5377217233181,48.5));
#81335=CARTESIAN_POINT('Ctrl Pts',(121.061732850969,3.5377217233181,48.35));
#81336=CARTESIAN_POINT('Ctrl Pts',(121.195293150842,3.46643933653831,48.35));
#81337=CARTESIAN_POINT('Ctrl Pts',(121.282332621515,3.33212831616402,48.35));
#81338=CARTESIAN_POINT('Ctrl Pts',(120.751091323793,3.60900411009789,48.5));
#81339=CARTESIAN_POINT('Ctrl Pts',(120.751091323793,3.60900411009789,48.35));
#81340=CARTESIAN_POINT('Ctrl Pts',(120.928171955049,3.60900411009789,48.5));
#81341=CARTESIAN_POINT('Ctrl Pts',(120.928171955049,3.60900411009789,48.35));
#81342=CARTESIAN_POINT('Ctrl Pts',(121.061732850969,3.5377217233181,48.5));
#81343=CARTESIAN_POINT('Ctrl Pts',(121.061732850969,3.5377217233181,48.35));
#81344=CARTESIAN_POINT('',(120.751091323793,3.60900411009789,48.5));
#81345=CARTESIAN_POINT('Ctrl Pts',(120.751091323793,3.60900411009789,48.5));
#81346=CARTESIAN_POINT('Ctrl Pts',(120.928171955049,3.60900411009789,48.5));
#81347=CARTESIAN_POINT('Ctrl Pts',(121.061732850969,3.5377217233181,48.5));
#81348=CARTESIAN_POINT('',(120.751091323793,3.60900411009789,48.35));
#81349=CARTESIAN_POINT('',(120.751091323793,3.60900411009789,48.5));
#81350=CARTESIAN_POINT('Ctrl Pts',(120.751091323793,3.60900411009789,48.35));
#81351=CARTESIAN_POINT('Ctrl Pts',(120.928171955049,3.60900411009789,48.35));
#81352=CARTESIAN_POINT('Ctrl Pts',(121.061732850969,3.5377217233181,48.35));
#81353=CARTESIAN_POINT('Ctrl Pts',(120.352660499513,3.47994545102119,48.5));
#81354=CARTESIAN_POINT('Ctrl Pts',(120.352660499513,3.47994545102119,48.35));
#81355=CARTESIAN_POINT('Ctrl Pts',(120.510982356966,3.60900411009789,48.5));
#81356=CARTESIAN_POINT('Ctrl Pts',(120.510982356966,3.60900411009789,48.35));
#81357=CARTESIAN_POINT('Ctrl Pts',(120.751091323793,3.60900411009789,48.5));
#81358=CARTESIAN_POINT('Ctrl Pts',(120.751091323793,3.60900411009789,48.35));
#81359=CARTESIAN_POINT('',(120.352660499513,3.47994545102119,48.5));
#81360=CARTESIAN_POINT('Ctrl Pts',(120.352660499513,3.47994545102119,48.5));
#81361=CARTESIAN_POINT('Ctrl Pts',(120.510982356966,3.60900411009789,48.5));
#81362=CARTESIAN_POINT('Ctrl Pts',(120.751091323793,3.60900411009789,48.5));
#81363=CARTESIAN_POINT('',(120.352660499513,3.47994545102119,48.35));
#81364=CARTESIAN_POINT('',(120.352660499513,3.47994545102119,48.5));
#81365=CARTESIAN_POINT('Ctrl Pts',(120.352660499513,3.47994545102119,48.35));
#81366=CARTESIAN_POINT('Ctrl Pts',(120.510982356966,3.60900411009789,48.35));
#81367=CARTESIAN_POINT('Ctrl Pts',(120.751091323793,3.60900411009789,48.35));
#81368=CARTESIAN_POINT('Ctrl Pts',(120.114051781595,3.11302864551544,48.5));
#81369=CARTESIAN_POINT('Ctrl Pts',(120.114051781595,3.11302864551544,48.35));
#81370=CARTESIAN_POINT('Ctrl Pts',(120.194338344038,3.3508867919445,48.5));
#81371=CARTESIAN_POINT('Ctrl Pts',(120.194338344038,3.3508867919445,48.35));
#81372=CARTESIAN_POINT('Ctrl Pts',(120.352660499513,3.47994545102119,48.5));
#81373=CARTESIAN_POINT('Ctrl Pts',(120.352660499513,3.47994545102119,48.35));
#81374=CARTESIAN_POINT('',(120.114051781595,3.11302864551544,48.5));
#81375=CARTESIAN_POINT('Ctrl Pts',(120.114051781595,3.11302864551544,48.5));
#81376=CARTESIAN_POINT('Ctrl Pts',(120.194338344038,3.3508867919445,48.5));
#81377=CARTESIAN_POINT('Ctrl Pts',(120.352660499513,3.47994545102119,48.5));
#81378=CARTESIAN_POINT('',(120.114051781595,3.11302864551544,48.35));
#81379=CARTESIAN_POINT('',(120.114051781595,3.11302864551544,48.5));
#81380=CARTESIAN_POINT('Ctrl Pts',(120.114051781595,3.11302864551544,48.35));
#81381=CARTESIAN_POINT('Ctrl Pts',(120.194338344038,3.3508867919445,48.35));
#81382=CARTESIAN_POINT('Ctrl Pts',(120.352660499513,3.47994545102119,48.35));
#81383=CARTESIAN_POINT('Ctrl Pts',(120.033765517175,2.48499327898026,48.5));
#81384=CARTESIAN_POINT('Ctrl Pts',(120.033765517175,2.48499327898026,48.35));
#81385=CARTESIAN_POINT('Ctrl Pts',(120.033765517175,2.87517049908638,48.5));
#81386=CARTESIAN_POINT('Ctrl Pts',(120.033765517175,2.87517049908638,48.35));
#81387=CARTESIAN_POINT('Ctrl Pts',(120.114051781595,3.11302864551544,48.5));
#81388=CARTESIAN_POINT('Ctrl Pts',(120.114051781595,3.11302864551544,48.35));
#81389=CARTESIAN_POINT('',(120.033765517175,2.48499327898026,48.5));
#81390=CARTESIAN_POINT('Ctrl Pts',(120.033765517175,2.48499327898026,48.5));
#81391=CARTESIAN_POINT('Ctrl Pts',(120.033765517175,2.87517049908638,48.5));
#81392=CARTESIAN_POINT('Ctrl Pts',(120.114051781595,3.11302864551544,48.5));
#81393=CARTESIAN_POINT('',(120.033765517175,2.48499327898026,48.35));
#81394=CARTESIAN_POINT('',(120.033765517175,2.48499327898026,48.5));
#81395=CARTESIAN_POINT('Ctrl Pts',(120.033765517175,2.48499327898026,48.35));
#81396=CARTESIAN_POINT('Ctrl Pts',(120.033765517175,2.87517049908638,48.35));
#81397=CARTESIAN_POINT('Ctrl Pts',(120.114051781595,3.11302864551544,48.35));
#81398=CARTESIAN_POINT('Ctrl Pts',(120.251364193857,1.59058684110642,48.5));
#81399=CARTESIAN_POINT('Ctrl Pts',(120.251364193857,1.59058684110642,48.35));
#81400=CARTESIAN_POINT('Ctrl Pts',(120.033765517175,1.86521166563034,48.5));
#81401=CARTESIAN_POINT('Ctrl Pts',(120.033765517175,1.86521166563034,48.35));
#81402=CARTESIAN_POINT('Ctrl Pts',(120.033765517175,2.48499327898026,48.5));
#81403=CARTESIAN_POINT('Ctrl Pts',(120.033765517175,2.48499327898026,48.35));
#81404=CARTESIAN_POINT('Ctrl Pts',(120.251364193857,1.59058684110642,48.5));
#81405=CARTESIAN_POINT('Ctrl Pts',(120.033765517175,1.86521166563034,48.5));
#81406=CARTESIAN_POINT('Ctrl Pts',(120.033765517175,2.48499327898026,48.5));
#81407=CARTESIAN_POINT('Ctrl Pts',(120.251364193857,1.59058684110642,48.35));
#81408=CARTESIAN_POINT('Ctrl Pts',(120.033765517175,1.86521166563034,48.35));
#81409=CARTESIAN_POINT('Ctrl Pts',(120.033765517175,2.48499327898026,48.35));
#81410=CARTESIAN_POINT('Origin',(119.999999858439,2.48574362695217,48.35));
#81411=CARTESIAN_POINT('Origin',(119.167871855199,3.60900411009789,48.5));
#81412=CARTESIAN_POINT('',(119.167871855199,3.60900411009789,48.5));
#81413=CARTESIAN_POINT('',(119.341951094568,3.60900411009789,48.5));
#81414=CARTESIAN_POINT('',(59.5839359275997,3.60900411009789,48.5));
#81415=CARTESIAN_POINT('',(119.167871855199,3.60900411009789,48.35));
#81416=CARTESIAN_POINT('',(119.167871855199,3.60900411009789,48.5));
#81417=CARTESIAN_POINT('',(119.341951094568,3.60900411009789,48.35));
#81418=CARTESIAN_POINT('',(119.167871855199,3.60900411009789,48.35));
#81419=CARTESIAN_POINT('',(119.341951094568,3.60900411009789,48.5));
#81420=CARTESIAN_POINT('Ctrl Pts',(118.92776273936,3.31487053632736,48.5));
#81421=CARTESIAN_POINT('Ctrl Pts',(118.92776273936,3.31487053632736,48.35));
#81422=CARTESIAN_POINT('Ctrl Pts',(119.097339741886,3.46643933653831,48.5));
#81423=CARTESIAN_POINT('Ctrl Pts',(119.097339741886,3.46643933653831,48.35));
#81424=CARTESIAN_POINT('Ctrl Pts',(119.167871855199,3.60900411009789,48.5));
#81425=CARTESIAN_POINT('Ctrl Pts',(119.167871855199,3.60900411009789,48.35));
#81426=CARTESIAN_POINT('',(118.92776273936,3.31487053632736,48.5));
#81427=CARTESIAN_POINT('Ctrl Pts',(118.92776273936,3.31487053632736,48.5));
#81428=CARTESIAN_POINT('Ctrl Pts',(119.097339741886,3.46643933653831,48.5));
#81429=CARTESIAN_POINT('Ctrl Pts',(119.167871855199,3.60900411009789,48.5));
#81430=CARTESIAN_POINT('',(118.92776273936,3.31487053632736,48.35));
#81431=CARTESIAN_POINT('',(118.92776273936,3.31487053632736,48.5));
#81432=CARTESIAN_POINT('Ctrl Pts',(118.92776273936,3.31487053632736,48.35));
#81433=CARTESIAN_POINT('Ctrl Pts',(119.097339741886,3.46643933653831,48.35));
#81434=CARTESIAN_POINT('Ctrl Pts',(119.167871855199,3.60900411009789,48.35));
#81435=CARTESIAN_POINT('Ctrl Pts',(118.531582586467,3.05675321817398,48.5));
#81436=CARTESIAN_POINT('Ctrl Pts',(118.531582586467,3.05675321817398,48.35));
#81437=CARTESIAN_POINT('Ctrl Pts',(118.758185587823,3.1633015871048,48.5));
#81438=CARTESIAN_POINT('Ctrl Pts',(118.758185587823,3.1633015871048,48.35));
#81439=CARTESIAN_POINT('Ctrl Pts',(118.92776273936,3.31487053632736,48.5));
#81440=CARTESIAN_POINT('Ctrl Pts',(118.92776273936,3.31487053632736,48.35));
#81441=CARTESIAN_POINT('',(118.531582586467,3.05675321817398,48.5));
#81442=CARTESIAN_POINT('Ctrl Pts',(118.531582586467,3.05675321817398,48.5));
#81443=CARTESIAN_POINT('Ctrl Pts',(118.758185587823,3.1633015871048,48.5));
#81444=CARTESIAN_POINT('Ctrl Pts',(118.92776273936,3.31487053632736,48.5));
#81445=CARTESIAN_POINT('',(118.531582586467,3.05675321817398,48.35));
#81446=CARTESIAN_POINT('',(118.531582586467,3.05675321817398,48.5));
#81447=CARTESIAN_POINT('Ctrl Pts',(118.531582586467,3.05675321817398,48.35));
#81448=CARTESIAN_POINT('Ctrl Pts',(118.758185587823,3.1633015871048,48.35));
#81449=CARTESIAN_POINT('Ctrl Pts',(118.92776273936,3.31487053632736,48.35));
#81450=CARTESIAN_POINT('Origin',(118.531582586467,2.79563450813293,48.5));
#81451=CARTESIAN_POINT('',(118.531582586467,2.79563450813293,48.5));
#81452=CARTESIAN_POINT('',(118.531582586467,5.39781725406647,48.5));
#81453=CARTESIAN_POINT('',(118.531582586467,2.79563450813293,48.35));
#81454=CARTESIAN_POINT('',(118.531582586467,2.79563450813293,48.5));
#81455=CARTESIAN_POINT('',(118.531582586467,2.79563450813293,48.35));
#81456=CARTESIAN_POINT('Ctrl Pts',(118.81596186012,2.93519788980484,48.5));
#81457=CARTESIAN_POINT('Ctrl Pts',(118.81596186012,2.93519788980484,48.35));
#81458=CARTESIAN_POINT('Ctrl Pts',(118.657640002668,2.8421556353569,48.5));
#81459=CARTESIAN_POINT('Ctrl Pts',(118.657640002668,2.8421556353569,48.35));
#81460=CARTESIAN_POINT('Ctrl Pts',(118.531582586467,2.79563450813293,48.5));
#81461=CARTESIAN_POINT('Ctrl Pts',(118.531582586467,2.79563450813293,48.35));
#81462=CARTESIAN_POINT('',(118.81596186012,2.93519788980484,48.5));
#81463=CARTESIAN_POINT('Ctrl Pts',(118.81596186012,2.93519788980484,48.5));
#81464=CARTESIAN_POINT('Ctrl Pts',(118.657640002668,2.8421556353569,48.5));
#81465=CARTESIAN_POINT('Ctrl Pts',(118.531582586467,2.79563450813293,48.5));
#81466=CARTESIAN_POINT('',(118.81596186012,2.93519788980484,48.35));
#81467=CARTESIAN_POINT('',(118.81596186012,2.93519788980484,48.5));
#81468=CARTESIAN_POINT('Ctrl Pts',(118.81596186012,2.93519788980484,48.35));
#81469=CARTESIAN_POINT('Ctrl Pts',(118.657640002668,2.8421556353569,48.35));
#81470=CARTESIAN_POINT('Ctrl Pts',(118.531582586467,2.79563450813293,48.35));
#81471=CARTESIAN_POINT('Ctrl Pts',(119.071828208864,3.12128254771233,48.5));
#81472=CARTESIAN_POINT('Ctrl Pts',(119.071828208864,3.12128254771233,48.35));
#81473=CARTESIAN_POINT('Ctrl Pts',(118.974283866584,3.02824014425278,48.5));
#81474=CARTESIAN_POINT('Ctrl Pts',(118.974283866584,3.02824014425278,48.35));
#81475=CARTESIAN_POINT('Ctrl Pts',(118.81596186012,2.93519788980484,48.5));
#81476=CARTESIAN_POINT('Ctrl Pts',(118.81596186012,2.93519788980484,48.35));
#81477=CARTESIAN_POINT('',(119.071828208864,3.12128254771233,48.5));
#81478=CARTESIAN_POINT('Ctrl Pts',(119.071828208864,3.12128254771233,48.5));
#81479=CARTESIAN_POINT('Ctrl Pts',(118.974283866584,3.02824014425278,48.5));
#81480=CARTESIAN_POINT('Ctrl Pts',(118.81596186012,2.93519788980484,48.5));
#81481=CARTESIAN_POINT('',(119.071828208864,3.12128254771233,48.35));
#81482=CARTESIAN_POINT('',(119.071828208864,3.12128254771233,48.5));
#81483=CARTESIAN_POINT('Ctrl Pts',(119.071828208864,3.12128254771233,48.35));
#81484=CARTESIAN_POINT('Ctrl Pts',(118.974283866584,3.02824014425278,48.35));
#81485=CARTESIAN_POINT('Ctrl Pts',(118.81596186012,2.93519788980484,48.35));
#81486=CARTESIAN_POINT('Origin',(119.071828208864,1.40000009536743,48.5));
#81487=CARTESIAN_POINT('',(119.071828208864,1.40000009536743,48.5));
#81488=CARTESIAN_POINT('',(119.071828208864,4.70000004768372,48.5));
#81489=CARTESIAN_POINT('',(119.071828208864,1.40000009536743,48.35));
#81490=CARTESIAN_POINT('',(119.071828208864,1.40000009536743,48.5));
#81491=CARTESIAN_POINT('',(119.071828208864,1.40000009536743,48.35));
#81492=CARTESIAN_POINT('Origin',(119.341951094568,1.40000009536743,48.5));
#81493=CARTESIAN_POINT('',(119.341951094568,1.40000009536743,48.5));
#81494=CARTESIAN_POINT('',(59.6709755472839,1.40000009536743,48.5));
#81495=CARTESIAN_POINT('',(119.341951094568,1.40000009536743,48.35));
#81496=CARTESIAN_POINT('',(119.341951094568,1.40000009536743,48.5));
#81497=CARTESIAN_POINT('',(119.341951094568,1.40000009536743,48.35));
#81498=CARTESIAN_POINT('Origin',(119.341951094568,3.60900411009789,48.5));
#81499=CARTESIAN_POINT('',(119.341951094568,5.80450205504894,48.5));
#81500=CARTESIAN_POINT('',(119.341951094568,3.60900411009789,48.35));
#81501=CARTESIAN_POINT('Origin',(119.999999858439,2.48574362695217,48.35));
#81502=CARTESIAN_POINT('Origin',(0.,8.,48.5));
#81503=CARTESIAN_POINT('Ctrl Pts',(109.996998559684,3.38540250062943,48.5));
#81504=CARTESIAN_POINT('Ctrl Pts',(109.996998559684,3.38540250062943,48.35));
#81505=CARTESIAN_POINT('Ctrl Pts',(109.810914050788,3.38540250062943,48.5));
#81506=CARTESIAN_POINT('Ctrl Pts',(109.810914050788,3.38540250062943,48.35));
#81507=CARTESIAN_POINT('Ctrl Pts',(109.699863743037,3.22783091664314,48.5));
#81508=CARTESIAN_POINT('Ctrl Pts',(109.699863743037,3.22783091664314,48.35));
#81509=CARTESIAN_POINT('',(109.996998559684,3.38540250062943,48.5));
#81510=CARTESIAN_POINT('',(109.699863743037,3.22783091664314,48.5));
#81511=CARTESIAN_POINT('Ctrl Pts',(109.996998559684,3.38540250062943,48.5));
#81512=CARTESIAN_POINT('Ctrl Pts',(109.810914050788,3.38540250062943,48.5));
#81513=CARTESIAN_POINT('Ctrl Pts',(109.699863743037,3.22783091664314,48.5));
#81514=CARTESIAN_POINT('',(109.996998559684,3.38540250062943,48.35));
#81515=CARTESIAN_POINT('',(109.996998559684,3.38540250062943,48.5));
#81516=CARTESIAN_POINT('',(109.699863743037,3.22783091664314,48.35));
#81517=CARTESIAN_POINT('Ctrl Pts',(109.996998559684,3.38540250062943,48.35));
#81518=CARTESIAN_POINT('Ctrl Pts',(109.810914050788,3.38540250062943,48.35));
#81519=CARTESIAN_POINT('Ctrl Pts',(109.699863743037,3.22783091664314,48.35));
#81520=CARTESIAN_POINT('',(109.699863743037,3.22783091664314,48.5));
#81521=CARTESIAN_POINT('Ctrl Pts',(110.312892448157,3.2068213224411,48.5));
#81522=CARTESIAN_POINT('Ctrl Pts',(110.312892448157,3.2068213224411,48.35));
#81523=CARTESIAN_POINT('Ctrl Pts',(110.18608475849,3.38540250062943,48.5));
#81524=CARTESIAN_POINT('Ctrl Pts',(110.18608475849,3.38540250062943,48.35));
#81525=CARTESIAN_POINT('Ctrl Pts',(109.996998559684,3.38540250062943,48.5));
#81526=CARTESIAN_POINT('Ctrl Pts',(109.996998559684,3.38540250062943,48.35));
#81527=CARTESIAN_POINT('',(110.312892448157,3.2068213224411,48.5));
#81528=CARTESIAN_POINT('Ctrl Pts',(110.312892448157,3.2068213224411,48.5));
#81529=CARTESIAN_POINT('Ctrl Pts',(110.18608475849,3.38540250062943,48.5));
#81530=CARTESIAN_POINT('Ctrl Pts',(109.996998559684,3.38540250062943,48.5));
#81531=CARTESIAN_POINT('',(110.312892448157,3.2068213224411,48.35));
#81532=CARTESIAN_POINT('',(110.312892448157,3.2068213224411,48.5));
#81533=CARTESIAN_POINT('Ctrl Pts',(110.312892448157,3.2068213224411,48.35));
#81534=CARTESIAN_POINT('Ctrl Pts',(110.18608475849,3.38540250062943,48.35));
#81535=CARTESIAN_POINT('Ctrl Pts',(109.996998559684,3.38540250062943,48.35));
#81536=CARTESIAN_POINT('Ctrl Pts',(110.439700137824,2.48499327898026,48.5));
#81537=CARTESIAN_POINT('Ctrl Pts',(110.439700137824,2.48499327898026,48.35));
#81538=CARTESIAN_POINT('Ctrl Pts',(110.439700137824,3.02824014425278,48.5));
#81539=CARTESIAN_POINT('Ctrl Pts',(110.439700137824,3.02824014425278,48.35));
#81540=CARTESIAN_POINT('Ctrl Pts',(110.312892448157,3.2068213224411,48.5));
#81541=CARTESIAN_POINT('Ctrl Pts',(110.312892448157,3.2068213224411,48.35));
#81542=CARTESIAN_POINT('',(110.439700137824,2.48499327898026,48.5));
#81543=CARTESIAN_POINT('Ctrl Pts',(110.439700137824,2.48499327898026,48.5));
#81544=CARTESIAN_POINT('Ctrl Pts',(110.439700137824,3.02824014425278,48.5));
#81545=CARTESIAN_POINT('Ctrl Pts',(110.312892448157,3.2068213224411,48.5));
#81546=CARTESIAN_POINT('',(110.439700137824,2.48499327898026,48.35));
#81547=CARTESIAN_POINT('',(110.439700137824,2.48499327898026,48.5));
#81548=CARTESIAN_POINT('Ctrl Pts',(110.439700137824,2.48499327898026,48.35));
#81549=CARTESIAN_POINT('Ctrl Pts',(110.439700137824,3.02824014425278,48.35));
#81550=CARTESIAN_POINT('Ctrl Pts',(110.312892448157,3.2068213224411,48.35));
#81551=CARTESIAN_POINT('Ctrl Pts',(110.312892448157,1.76466578245163,48.5));
#81552=CARTESIAN_POINT('Ctrl Pts',(110.312892448157,1.76466578245163,48.35));
#81553=CARTESIAN_POINT('Ctrl Pts',(110.439700137824,1.9447478055954,48.5));
#81554=CARTESIAN_POINT('Ctrl Pts',(110.439700137824,1.9447478055954,48.35));
#81555=CARTESIAN_POINT('Ctrl Pts',(110.439700137824,2.48499327898026,48.5));
#81556=CARTESIAN_POINT('Ctrl Pts',(110.439700137824,2.48499327898026,48.35));
#81557=CARTESIAN_POINT('',(110.312892448157,1.76466578245163,48.5));
#81558=CARTESIAN_POINT('Ctrl Pts',(110.312892448157,1.76466578245163,48.5));
#81559=CARTESIAN_POINT('Ctrl Pts',(110.439700137824,1.9447478055954,48.5));
#81560=CARTESIAN_POINT('Ctrl Pts',(110.439700137824,2.48499327898026,48.5));
#81561=CARTESIAN_POINT('',(110.312892448157,1.76466578245163,48.35));
#81562=CARTESIAN_POINT('',(110.312892448157,1.76466578245163,48.5));
#81563=CARTESIAN_POINT('Ctrl Pts',(110.312892448157,1.76466578245163,48.35));
#81564=CARTESIAN_POINT('Ctrl Pts',(110.439700137824,1.9447478055954,48.35));
#81565=CARTESIAN_POINT('Ctrl Pts',(110.439700137824,2.48499327898026,48.35));
#81566=CARTESIAN_POINT('Ctrl Pts',(109.999999951571,1.58458405733109,48.5));
#81567=CARTESIAN_POINT('Ctrl Pts',(109.999999951571,1.58458405733109,48.35));
#81568=CARTESIAN_POINT('Ctrl Pts',(110.18608475849,1.58458405733109,48.5));
#81569=CARTESIAN_POINT('Ctrl Pts',(110.18608475849,1.58458405733109,48.35));
#81570=CARTESIAN_POINT('Ctrl Pts',(110.312892448157,1.76466578245163,48.5));
#81571=CARTESIAN_POINT('Ctrl Pts',(110.312892448157,1.76466578245163,48.35));
#81572=CARTESIAN_POINT('',(109.999999951571,1.58458405733109,48.5));
#81573=CARTESIAN_POINT('Ctrl Pts',(109.999999951571,1.58458405733109,48.5));
#81574=CARTESIAN_POINT('Ctrl Pts',(110.18608475849,1.58458405733109,48.5));
#81575=CARTESIAN_POINT('Ctrl Pts',(110.312892448157,1.76466578245163,48.5));
#81576=CARTESIAN_POINT('',(109.999999951571,1.58458405733109,48.35));
#81577=CARTESIAN_POINT('',(109.999999951571,1.58458405733109,48.5));
#81578=CARTESIAN_POINT('Ctrl Pts',(109.999999951571,1.58458405733109,48.35));
#81579=CARTESIAN_POINT('Ctrl Pts',(110.18608475849,1.58458405733109,48.35));
#81580=CARTESIAN_POINT('Ctrl Pts',(110.312892448157,1.76466578245163,48.35));
#81581=CARTESIAN_POINT('Ctrl Pts',(109.687107753009,1.76391565799713,48.5));
#81582=CARTESIAN_POINT('Ctrl Pts',(109.687107753009,1.76391565799713,48.35));
#81583=CARTESIAN_POINT('Ctrl Pts',(109.813915442675,1.58458405733109,48.5));
#81584=CARTESIAN_POINT('Ctrl Pts',(109.813915442675,1.58458405733109,48.35));
#81585=CARTESIAN_POINT('Ctrl Pts',(109.999999951571,1.58458405733109,48.5));
#81586=CARTESIAN_POINT('Ctrl Pts',(109.999999951571,1.58458405733109,48.35));
#81587=CARTESIAN_POINT('',(109.687107753009,1.76391565799713,48.5));
#81588=CARTESIAN_POINT('Ctrl Pts',(109.687107753009,1.76391565799713,48.5));
#81589=CARTESIAN_POINT('Ctrl Pts',(109.813915442675,1.58458405733109,48.5));
#81590=CARTESIAN_POINT('Ctrl Pts',(109.999999951571,1.58458405733109,48.5));
#81591=CARTESIAN_POINT('',(109.687107753009,1.76391565799713,48.35));
#81592=CARTESIAN_POINT('',(109.687107753009,1.76391565799713,48.5));
#81593=CARTESIAN_POINT('Ctrl Pts',(109.687107753009,1.76391565799713,48.35));
#81594=CARTESIAN_POINT('Ctrl Pts',(109.813915442675,1.58458405733109,48.35));
#81595=CARTESIAN_POINT('Ctrl Pts',(109.999999951571,1.58458405733109,48.35));
#81596=CARTESIAN_POINT('Ctrl Pts',(109.560300361365,2.48499327898026,48.5));
#81597=CARTESIAN_POINT('Ctrl Pts',(109.560300361365,2.48499327898026,48.35));
#81598=CARTESIAN_POINT('Ctrl Pts',(109.560300361365,1.94324696063995,48.5));
#81599=CARTESIAN_POINT('Ctrl Pts',(109.560300361365,1.94324696063995,48.35));
#81600=CARTESIAN_POINT('Ctrl Pts',(109.687107753009,1.76391565799713,48.5));
#81601=CARTESIAN_POINT('Ctrl Pts',(109.687107753009,1.76391565799713,48.35));
#81602=CARTESIAN_POINT('',(109.560300361365,2.48499327898026,48.5));
#81603=CARTESIAN_POINT('Ctrl Pts',(109.560300361365,2.48499327898026,48.5));
#81604=CARTESIAN_POINT('Ctrl Pts',(109.560300361365,1.94324696063995,48.5));
#81605=CARTESIAN_POINT('Ctrl Pts',(109.687107753009,1.76391565799713,48.5));
#81606=CARTESIAN_POINT('',(109.560300361365,2.48499327898026,48.35));
#81607=CARTESIAN_POINT('',(109.560300361365,2.48499327898026,48.5));
#81608=CARTESIAN_POINT('Ctrl Pts',(109.560300361365,2.48499327898026,48.35));
#81609=CARTESIAN_POINT('Ctrl Pts',(109.560300361365,1.94324696063995,48.35));
#81610=CARTESIAN_POINT('Ctrl Pts',(109.687107753009,1.76391565799713,48.35));
#81611=CARTESIAN_POINT('Ctrl Pts',(109.699863743037,3.22783091664314,48.5));
#81612=CARTESIAN_POINT('Ctrl Pts',(109.699863743037,3.22783091664314,48.35));
#81613=CARTESIAN_POINT('Ctrl Pts',(109.560300361365,3.02673944830894,48.5));
#81614=CARTESIAN_POINT('Ctrl Pts',(109.560300361365,3.02673944830894,48.35));
#81615=CARTESIAN_POINT('Ctrl Pts',(109.560300361365,2.48499327898026,48.5));
#81616=CARTESIAN_POINT('Ctrl Pts',(109.560300361365,2.48499327898026,48.35));
#81617=CARTESIAN_POINT('Ctrl Pts',(109.699863743037,3.22783091664314,48.5));
#81618=CARTESIAN_POINT('Ctrl Pts',(109.560300361365,3.02673944830894,48.5));
#81619=CARTESIAN_POINT('Ctrl Pts',(109.560300361365,2.48499327898026,48.5));
#81620=CARTESIAN_POINT('Ctrl Pts',(109.699863743037,3.22783091664314,48.35));
#81621=CARTESIAN_POINT('Ctrl Pts',(109.560300361365,3.02673944830894,48.35));
#81622=CARTESIAN_POINT('Ctrl Pts',(109.560300361365,2.48499327898026,48.35));
#81623=CARTESIAN_POINT('Ctrl Pts',(109.999999951571,1.36248314380646,48.5));
#81624=CARTESIAN_POINT('Ctrl Pts',(109.999999951571,1.36248314380646,48.35));
#81625=CARTESIAN_POINT('Ctrl Pts',(109.681855391711,1.36248314380646,48.5));
#81626=CARTESIAN_POINT('Ctrl Pts',(109.681855391711,1.36248314380646,48.35));
#81627=CARTESIAN_POINT('Ctrl Pts',(109.500272821635,1.59058684110642,48.5));
#81628=CARTESIAN_POINT('Ctrl Pts',(109.500272821635,1.59058684110642,48.35));
#81629=CARTESIAN_POINT('',(109.999999951571,1.36248314380646,48.5));
#81630=CARTESIAN_POINT('',(109.500272821635,1.59058684110642,48.5));
#81631=CARTESIAN_POINT('Ctrl Pts',(109.999999951571,1.36248314380646,48.5));
#81632=CARTESIAN_POINT('Ctrl Pts',(109.681855391711,1.36248314380646,48.5));
#81633=CARTESIAN_POINT('Ctrl Pts',(109.500272821635,1.59058684110642,48.5));
#81634=CARTESIAN_POINT('',(109.999999951571,1.36248314380646,48.35));
#81635=CARTESIAN_POINT('',(109.999999951571,1.36248314380646,48.5));
#81636=CARTESIAN_POINT('',(109.500272821635,1.59058684110642,48.35));
#81637=CARTESIAN_POINT('Ctrl Pts',(109.999999951571,1.36248314380646,48.35));
#81638=CARTESIAN_POINT('Ctrl Pts',(109.681855391711,1.36248314380646,48.35));
#81639=CARTESIAN_POINT('Ctrl Pts',(109.500272821635,1.59058684110642,48.35));
#81640=CARTESIAN_POINT('',(109.500272821635,1.59058684110642,48.5));
#81641=CARTESIAN_POINT('Ctrl Pts',(110.39993191883,1.49229192733765,48.5));
#81642=CARTESIAN_POINT('Ctrl Pts',(110.39993191883,1.49229192733765,48.35));
#81643=CARTESIAN_POINT('Ctrl Pts',(110.241609763354,1.36248314380646,48.5));
#81644=CARTESIAN_POINT('Ctrl Pts',(110.241609763354,1.36248314380646,48.35));
#81645=CARTESIAN_POINT('Ctrl Pts',(109.999999951571,1.36248314380646,48.5));
#81646=CARTESIAN_POINT('Ctrl Pts',(109.999999951571,1.36248314380646,48.35));
#81647=CARTESIAN_POINT('',(110.39993191883,1.49229192733765,48.5));
#81648=CARTESIAN_POINT('Ctrl Pts',(110.39993191883,1.49229192733765,48.5));
#81649=CARTESIAN_POINT('Ctrl Pts',(110.241609763354,1.36248314380646,48.5));
#81650=CARTESIAN_POINT('Ctrl Pts',(109.999999951571,1.36248314380646,48.5));
#81651=CARTESIAN_POINT('',(110.39993191883,1.49229192733765,48.35));
#81652=CARTESIAN_POINT('',(110.39993191883,1.49229192733765,48.5));
#81653=CARTESIAN_POINT('Ctrl Pts',(110.39993191883,1.49229192733765,48.35));
#81654=CARTESIAN_POINT('Ctrl Pts',(110.241609763354,1.36248314380646,48.35));
#81655=CARTESIAN_POINT('Ctrl Pts',(109.999999951571,1.36248314380646,48.35));
#81656=CARTESIAN_POINT('Ctrl Pts',(110.637789916247,1.85995900630951,48.5));
#81657=CARTESIAN_POINT('Ctrl Pts',(110.637789916247,1.85995900630951,48.35));
#81658=CARTESIAN_POINT('Ctrl Pts',(110.558253776282,1.62210100889206,48.5));
#81659=CARTESIAN_POINT('Ctrl Pts',(110.558253776282,1.62210100889206,48.35));
#81660=CARTESIAN_POINT('Ctrl Pts',(110.39993191883,1.49229192733765,48.5));
#81661=CARTESIAN_POINT('Ctrl Pts',(110.39993191883,1.49229192733765,48.35));
#81662=CARTESIAN_POINT('',(110.637789916247,1.85995900630951,48.5));
#81663=CARTESIAN_POINT('Ctrl Pts',(110.637789916247,1.85995900630951,48.5));
#81664=CARTESIAN_POINT('Ctrl Pts',(110.558253776282,1.62210100889206,48.5));
#81665=CARTESIAN_POINT('Ctrl Pts',(110.39993191883,1.49229192733765,48.5));
#81666=CARTESIAN_POINT('',(110.637789916247,1.85995900630951,48.35));
#81667=CARTESIAN_POINT('',(110.637789916247,1.85995900630951,48.5));
#81668=CARTESIAN_POINT('Ctrl Pts',(110.637789916247,1.85995900630951,48.35));
#81669=CARTESIAN_POINT('Ctrl Pts',(110.558253776282,1.62210100889206,48.35));
#81670=CARTESIAN_POINT('Ctrl Pts',(110.39993191883,1.49229192733765,48.35));
#81671=CARTESIAN_POINT('Ctrl Pts',(110.717326056212,2.48499327898026,48.5));
#81672=CARTESIAN_POINT('Ctrl Pts',(110.717326056212,2.48499327898026,48.35));
#81673=CARTESIAN_POINT('Ctrl Pts',(110.717326056212,2.09781730175018,48.5));
#81674=CARTESIAN_POINT('Ctrl Pts',(110.717326056212,2.09781730175018,48.35));
#81675=CARTESIAN_POINT('Ctrl Pts',(110.637789916247,1.85995900630951,48.5));
#81676=CARTESIAN_POINT('Ctrl Pts',(110.637789916247,1.85995900630951,48.35));
#81677=CARTESIAN_POINT('',(110.717326056212,2.48499327898026,48.5));
#81678=CARTESIAN_POINT('Ctrl Pts',(110.717326056212,2.48499327898026,48.5));
#81679=CARTESIAN_POINT('Ctrl Pts',(110.717326056212,2.09781730175018,48.5));
#81680=CARTESIAN_POINT('Ctrl Pts',(110.637789916247,1.85995900630951,48.5));
#81681=CARTESIAN_POINT('',(110.717326056212,2.48499327898026,48.35));
#81682=CARTESIAN_POINT('',(110.717326056212,2.48499327898026,48.5));
#81683=CARTESIAN_POINT('Ctrl Pts',(110.717326056212,2.48499327898026,48.35));
#81684=CARTESIAN_POINT('Ctrl Pts',(110.717326056212,2.09781730175018,48.35));
#81685=CARTESIAN_POINT('Ctrl Pts',(110.637789916247,1.85995900630951,48.35));
#81686=CARTESIAN_POINT('Ctrl Pts',(110.667803537101,3.00497958064079,48.5));
#81687=CARTESIAN_POINT('Ctrl Pts',(110.667803537101,3.00497958064079,48.35));
#81688=CARTESIAN_POINT('Ctrl Pts',(110.717326056212,2.81214186549187,48.5));
#81689=CARTESIAN_POINT('Ctrl Pts',(110.717326056212,2.81214186549187,48.35));
#81690=CARTESIAN_POINT('Ctrl Pts',(110.717326056212,2.48499327898026,48.5));
#81691=CARTESIAN_POINT('Ctrl Pts',(110.717326056212,2.48499327898026,48.35));
#81692=CARTESIAN_POINT('',(110.667803537101,3.00497958064079,48.5));
#81693=CARTESIAN_POINT('Ctrl Pts',(110.667803537101,3.00497958064079,48.5));
#81694=CARTESIAN_POINT('Ctrl Pts',(110.717326056212,2.81214186549187,48.5));
#81695=CARTESIAN_POINT('Ctrl Pts',(110.717326056212,2.48499327898026,48.5));
#81696=CARTESIAN_POINT('',(110.667803537101,3.00497958064079,48.35));
#81697=CARTESIAN_POINT('',(110.667803537101,3.00497958064079,48.5));
#81698=CARTESIAN_POINT('Ctrl Pts',(110.667803537101,3.00497958064079,48.35));
#81699=CARTESIAN_POINT('Ctrl Pts',(110.717326056212,2.81214186549187,48.35));
#81700=CARTESIAN_POINT('Ctrl Pts',(110.717326056212,2.48499327898026,48.35));
#81701=CARTESIAN_POINT('Ctrl Pts',(110.531241547316,3.33212831616402,48.5));
#81702=CARTESIAN_POINT('Ctrl Pts',(110.531241547316,3.33212831616402,48.35));
#81703=CARTESIAN_POINT('Ctrl Pts',(110.618281017989,3.19781729578972,48.5));
#81704=CARTESIAN_POINT('Ctrl Pts',(110.618281017989,3.19781729578972,48.35));
#81705=CARTESIAN_POINT('Ctrl Pts',(110.667803537101,3.00497958064079,48.5));
#81706=CARTESIAN_POINT('Ctrl Pts',(110.667803537101,3.00497958064079,48.35));
#81707=CARTESIAN_POINT('',(110.531241547316,3.33212831616402,48.5));
#81708=CARTESIAN_POINT('Ctrl Pts',(110.531241547316,3.33212831616402,48.5));
#81709=CARTESIAN_POINT('Ctrl Pts',(110.618281017989,3.19781729578972,48.5));
#81710=CARTESIAN_POINT('Ctrl Pts',(110.667803537101,3.00497958064079,48.5));
#81711=CARTESIAN_POINT('',(110.531241547316,3.33212831616402,48.35));
#81712=CARTESIAN_POINT('',(110.531241547316,3.33212831616402,48.5));
#81713=CARTESIAN_POINT('Ctrl Pts',(110.531241547316,3.33212831616402,48.35));
#81714=CARTESIAN_POINT('Ctrl Pts',(110.618281017989,3.19781729578972,48.35));
#81715=CARTESIAN_POINT('Ctrl Pts',(110.667803537101,3.00497958064079,48.35));
#81716=CARTESIAN_POINT('Ctrl Pts',(110.310641180724,3.5377217233181,48.5));
#81717=CARTESIAN_POINT('Ctrl Pts',(110.310641180724,3.5377217233181,48.35));
#81718=CARTESIAN_POINT('Ctrl Pts',(110.444202076644,3.46643933653831,48.5));
#81719=CARTESIAN_POINT('Ctrl Pts',(110.444202076644,3.46643933653831,48.35));
#81720=CARTESIAN_POINT('Ctrl Pts',(110.531241547316,3.33212831616402,48.5));
#81721=CARTESIAN_POINT('Ctrl Pts',(110.531241547316,3.33212831616402,48.35));
#81722=CARTESIAN_POINT('',(110.310641180724,3.5377217233181,48.5));
#81723=CARTESIAN_POINT('Ctrl Pts',(110.310641180724,3.5377217233181,48.5));
#81724=CARTESIAN_POINT('Ctrl Pts',(110.444202076644,3.46643933653831,48.5));
#81725=CARTESIAN_POINT('Ctrl Pts',(110.531241547316,3.33212831616402,48.5));
#81726=CARTESIAN_POINT('',(110.310641180724,3.5377217233181,48.35));
#81727=CARTESIAN_POINT('',(110.310641180724,3.5377217233181,48.5));
#81728=CARTESIAN_POINT('Ctrl Pts',(110.310641180724,3.5377217233181,48.35));
#81729=CARTESIAN_POINT('Ctrl Pts',(110.444202076644,3.46643933653831,48.35));
#81730=CARTESIAN_POINT('Ctrl Pts',(110.531241547316,3.33212831616402,48.35));
#81731=CARTESIAN_POINT('Ctrl Pts',(109.999999951571,3.60900411009789,48.5));
#81732=CARTESIAN_POINT('Ctrl Pts',(109.999999951571,3.60900411009789,48.35));
#81733=CARTESIAN_POINT('Ctrl Pts',(110.177080582827,3.60900411009789,48.5));
#81734=CARTESIAN_POINT('Ctrl Pts',(110.177080582827,3.60900411009789,48.35));
#81735=CARTESIAN_POINT('Ctrl Pts',(110.310641180724,3.5377217233181,48.5));
#81736=CARTESIAN_POINT('Ctrl Pts',(110.310641180724,3.5377217233181,48.35));
#81737=CARTESIAN_POINT('',(109.999999951571,3.60900411009789,48.5));
#81738=CARTESIAN_POINT('Ctrl Pts',(109.999999951571,3.60900411009789,48.5));
#81739=CARTESIAN_POINT('Ctrl Pts',(110.177080582827,3.60900411009789,48.5));
#81740=CARTESIAN_POINT('Ctrl Pts',(110.310641180724,3.5377217233181,48.5));
#81741=CARTESIAN_POINT('',(109.999999951571,3.60900411009789,48.35));
#81742=CARTESIAN_POINT('',(109.999999951571,3.60900411009789,48.5));
#81743=CARTESIAN_POINT('Ctrl Pts',(109.999999951571,3.60900411009789,48.35));
#81744=CARTESIAN_POINT('Ctrl Pts',(110.177080582827,3.60900411009789,48.35));
#81745=CARTESIAN_POINT('Ctrl Pts',(110.310641180724,3.5377217233181,48.35));
#81746=CARTESIAN_POINT('Ctrl Pts',(109.601568829268,3.47994545102119,48.5));
#81747=CARTESIAN_POINT('Ctrl Pts',(109.601568829268,3.47994545102119,48.35));
#81748=CARTESIAN_POINT('Ctrl Pts',(109.759890984744,3.60900411009789,48.5));
#81749=CARTESIAN_POINT('Ctrl Pts',(109.759890984744,3.60900411009789,48.35));
#81750=CARTESIAN_POINT('Ctrl Pts',(109.999999951571,3.60900411009789,48.5));
#81751=CARTESIAN_POINT('Ctrl Pts',(109.999999951571,3.60900411009789,48.35));
#81752=CARTESIAN_POINT('',(109.601568829268,3.47994545102119,48.5));
#81753=CARTESIAN_POINT('Ctrl Pts',(109.601568829268,3.47994545102119,48.5));
#81754=CARTESIAN_POINT('Ctrl Pts',(109.759890984744,3.60900411009789,48.5));
#81755=CARTESIAN_POINT('Ctrl Pts',(109.999999951571,3.60900411009789,48.5));
#81756=CARTESIAN_POINT('',(109.601568829268,3.47994545102119,48.35));
#81757=CARTESIAN_POINT('',(109.601568829268,3.47994545102119,48.5));
#81758=CARTESIAN_POINT('Ctrl Pts',(109.601568829268,3.47994545102119,48.35));
#81759=CARTESIAN_POINT('Ctrl Pts',(109.759890984744,3.60900411009789,48.35));
#81760=CARTESIAN_POINT('Ctrl Pts',(109.999999951571,3.60900411009789,48.35));
#81761=CARTESIAN_POINT('Ctrl Pts',(109.362960558385,3.11302864551544,48.5));
#81762=CARTESIAN_POINT('Ctrl Pts',(109.362960558385,3.11302864551544,48.35));
#81763=CARTESIAN_POINT('Ctrl Pts',(109.443246971816,3.3508867919445,48.5));
#81764=CARTESIAN_POINT('Ctrl Pts',(109.443246971816,3.3508867919445,48.35));
#81765=CARTESIAN_POINT('Ctrl Pts',(109.601568829268,3.47994545102119,48.5));
#81766=CARTESIAN_POINT('Ctrl Pts',(109.601568829268,3.47994545102119,48.35));
#81767=CARTESIAN_POINT('',(109.362960558385,3.11302864551544,48.5));
#81768=CARTESIAN_POINT('Ctrl Pts',(109.362960558385,3.11302864551544,48.5));
#81769=CARTESIAN_POINT('Ctrl Pts',(109.443246971816,3.3508867919445,48.5));
#81770=CARTESIAN_POINT('Ctrl Pts',(109.601568829268,3.47994545102119,48.5));
#81771=CARTESIAN_POINT('',(109.362960558385,3.11302864551544,48.35));
#81772=CARTESIAN_POINT('',(109.362960558385,3.11302864551544,48.5));
#81773=CARTESIAN_POINT('Ctrl Pts',(109.362960558385,3.11302864551544,48.35));
#81774=CARTESIAN_POINT('Ctrl Pts',(109.443246971816,3.3508867919445,48.35));
#81775=CARTESIAN_POINT('Ctrl Pts',(109.601568829268,3.47994545102119,48.35));
#81776=CARTESIAN_POINT('Ctrl Pts',(109.282673995942,2.48499327898026,48.5));
#81777=CARTESIAN_POINT('Ctrl Pts',(109.282673995942,2.48499327898026,48.35));
#81778=CARTESIAN_POINT('Ctrl Pts',(109.282673995942,2.87517049908638,48.5));
#81779=CARTESIAN_POINT('Ctrl Pts',(109.282673995942,2.87517049908638,48.35));
#81780=CARTESIAN_POINT('Ctrl Pts',(109.362960558385,3.11302864551544,48.5));
#81781=CARTESIAN_POINT('Ctrl Pts',(109.362960558385,3.11302864551544,48.35));
#81782=CARTESIAN_POINT('',(109.282673995942,2.48499327898026,48.5));
#81783=CARTESIAN_POINT('Ctrl Pts',(109.282673995942,2.48499327898026,48.5));
#81784=CARTESIAN_POINT('Ctrl Pts',(109.282673995942,2.87517049908638,48.5));
#81785=CARTESIAN_POINT('Ctrl Pts',(109.362960558385,3.11302864551544,48.5));
#81786=CARTESIAN_POINT('',(109.282673995942,2.48499327898026,48.35));
#81787=CARTESIAN_POINT('',(109.282673995942,2.48499327898026,48.5));
#81788=CARTESIAN_POINT('Ctrl Pts',(109.282673995942,2.48499327898026,48.35));
#81789=CARTESIAN_POINT('Ctrl Pts',(109.282673995942,2.87517049908638,48.35));
#81790=CARTESIAN_POINT('Ctrl Pts',(109.362960558385,3.11302864551544,48.35));
#81791=CARTESIAN_POINT('Ctrl Pts',(109.500272821635,1.59058684110642,48.5));
#81792=CARTESIAN_POINT('Ctrl Pts',(109.500272821635,1.59058684110642,48.35));
#81793=CARTESIAN_POINT('Ctrl Pts',(109.282673995942,1.86521166563034,48.5));
#81794=CARTESIAN_POINT('Ctrl Pts',(109.282673995942,1.86521166563034,48.35));
#81795=CARTESIAN_POINT('Ctrl Pts',(109.282673995942,2.48499327898026,48.5));
#81796=CARTESIAN_POINT('Ctrl Pts',(109.282673995942,2.48499327898026,48.35));
#81797=CARTESIAN_POINT('Ctrl Pts',(109.500272821635,1.59058684110642,48.5));
#81798=CARTESIAN_POINT('Ctrl Pts',(109.282673995942,1.86521166563034,48.5));
#81799=CARTESIAN_POINT('Ctrl Pts',(109.282673995942,2.48499327898026,48.5));
#81800=CARTESIAN_POINT('Ctrl Pts',(109.500272821635,1.59058684110642,48.35));
#81801=CARTESIAN_POINT('Ctrl Pts',(109.282673995942,1.86521166563034,48.35));
#81802=CARTESIAN_POINT('Ctrl Pts',(109.282673995942,2.48499327898026,48.35));
#81803=CARTESIAN_POINT('Origin',(110.000000026077,2.48574362695217,48.35));
#81804=CARTESIAN_POINT('Origin',(0.,8.,48.5));
#81805=CARTESIAN_POINT('Ctrl Pts',(100.748090229928,3.38540250062943,48.5));
#81806=CARTESIAN_POINT('Ctrl Pts',(100.748090229928,3.38540250062943,48.35));
#81807=CARTESIAN_POINT('Ctrl Pts',(100.562005423009,3.38540250062943,48.5));
#81808=CARTESIAN_POINT('Ctrl Pts',(100.562005423009,3.38540250062943,48.35));
#81809=CARTESIAN_POINT('Ctrl Pts',(100.450955115259,3.22783091664314,48.5));
#81810=CARTESIAN_POINT('Ctrl Pts',(100.450955115259,3.22783091664314,48.35));
#81811=CARTESIAN_POINT('',(100.748090229928,3.38540250062943,48.5));
#81812=CARTESIAN_POINT('',(100.450955115259,3.22783091664314,48.5));
#81813=CARTESIAN_POINT('Ctrl Pts',(100.748090229928,3.38540250062943,48.5));
#81814=CARTESIAN_POINT('Ctrl Pts',(100.562005423009,3.38540250062943,48.5));
#81815=CARTESIAN_POINT('Ctrl Pts',(100.450955115259,3.22783091664314,48.5));
#81816=CARTESIAN_POINT('',(100.748090229928,3.38540250062943,48.35));
#81817=CARTESIAN_POINT('',(100.748090229928,3.38540250062943,48.5));
#81818=CARTESIAN_POINT('',(100.450955115259,3.22783091664314,48.35));
#81819=CARTESIAN_POINT('Ctrl Pts',(100.748090229928,3.38540250062943,48.35));
#81820=CARTESIAN_POINT('Ctrl Pts',(100.562005423009,3.38540250062943,48.35));
#81821=CARTESIAN_POINT('Ctrl Pts',(100.450955115259,3.22783091664314,48.35));
#81822=CARTESIAN_POINT('',(100.450955115259,3.22783091664314,48.5));
#81823=CARTESIAN_POINT('Ctrl Pts',(101.063983522356,3.2068213224411,48.5));
#81824=CARTESIAN_POINT('Ctrl Pts',(101.063983522356,3.2068213224411,48.35));
#81825=CARTESIAN_POINT('Ctrl Pts',(100.937175832689,3.38540250062943,48.5));
#81826=CARTESIAN_POINT('Ctrl Pts',(100.937175832689,3.38540250062943,48.35));
#81827=CARTESIAN_POINT('Ctrl Pts',(100.748090229928,3.38540250062943,48.5));
#81828=CARTESIAN_POINT('Ctrl Pts',(100.748090229928,3.38540250062943,48.35));
#81829=CARTESIAN_POINT('',(101.063983522356,3.2068213224411,48.5));
#81830=CARTESIAN_POINT('Ctrl Pts',(101.063983522356,3.2068213224411,48.5));
#81831=CARTESIAN_POINT('Ctrl Pts',(100.937175832689,3.38540250062943,48.5));
#81832=CARTESIAN_POINT('Ctrl Pts',(100.748090229928,3.38540250062943,48.5));
#81833=CARTESIAN_POINT('',(101.063983522356,3.2068213224411,48.35));
#81834=CARTESIAN_POINT('',(101.063983522356,3.2068213224411,48.5));
#81835=CARTESIAN_POINT('Ctrl Pts',(101.063983522356,3.2068213224411,48.35));
#81836=CARTESIAN_POINT('Ctrl Pts',(100.937175832689,3.38540250062943,48.35));
#81837=CARTESIAN_POINT('Ctrl Pts',(100.748090229928,3.38540250062943,48.35));
#81838=CARTESIAN_POINT('Ctrl Pts',(101.190791212022,2.48499327898026,48.5));
#81839=CARTESIAN_POINT('Ctrl Pts',(101.190791212022,2.48499327898026,48.35));
#81840=CARTESIAN_POINT('Ctrl Pts',(101.190791212022,3.02824014425278,48.5));
#81841=CARTESIAN_POINT('Ctrl Pts',(101.190791212022,3.02824014425278,48.35));
#81842=CARTESIAN_POINT('Ctrl Pts',(101.063983522356,3.2068213224411,48.5));
#81843=CARTESIAN_POINT('Ctrl Pts',(101.063983522356,3.2068213224411,48.35));
#81844=CARTESIAN_POINT('',(101.190791212022,2.48499327898026,48.5));
#81845=CARTESIAN_POINT('Ctrl Pts',(101.190791212022,2.48499327898026,48.5));
#81846=CARTESIAN_POINT('Ctrl Pts',(101.190791212022,3.02824014425278,48.5));
#81847=CARTESIAN_POINT('Ctrl Pts',(101.063983522356,3.2068213224411,48.5));
#81848=CARTESIAN_POINT('',(101.190791212022,2.48499327898026,48.35));
#81849=CARTESIAN_POINT('',(101.190791212022,2.48499327898026,48.5));
#81850=CARTESIAN_POINT('Ctrl Pts',(101.190791212022,2.48499327898026,48.35));
#81851=CARTESIAN_POINT('Ctrl Pts',(101.190791212022,3.02824014425278,48.35));
#81852=CARTESIAN_POINT('Ctrl Pts',(101.063983522356,3.2068213224411,48.35));
#81853=CARTESIAN_POINT('Ctrl Pts',(101.063983522356,1.76466578245163,48.5));
#81854=CARTESIAN_POINT('Ctrl Pts',(101.063983522356,1.76466578245163,48.35));
#81855=CARTESIAN_POINT('Ctrl Pts',(101.190791212022,1.9447478055954,48.5));
#81856=CARTESIAN_POINT('Ctrl Pts',(101.190791212022,1.9447478055954,48.35));
#81857=CARTESIAN_POINT('Ctrl Pts',(101.190791212022,2.48499327898026,48.5));
#81858=CARTESIAN_POINT('Ctrl Pts',(101.190791212022,2.48499327898026,48.35));
#81859=CARTESIAN_POINT('',(101.063983522356,1.76466578245163,48.5));
#81860=CARTESIAN_POINT('Ctrl Pts',(101.063983522356,1.76466578245163,48.5));
#81861=CARTESIAN_POINT('Ctrl Pts',(101.190791212022,1.9447478055954,48.5));
#81862=CARTESIAN_POINT('Ctrl Pts',(101.190791212022,2.48499327898026,48.5));
#81863=CARTESIAN_POINT('',(101.063983522356,1.76466578245163,48.35));
#81864=CARTESIAN_POINT('',(101.063983522356,1.76466578245163,48.5));
#81865=CARTESIAN_POINT('Ctrl Pts',(101.063983522356,1.76466578245163,48.35));
#81866=CARTESIAN_POINT('Ctrl Pts',(101.190791212022,1.9447478055954,48.35));
#81867=CARTESIAN_POINT('Ctrl Pts',(101.190791212022,2.48499327898026,48.35));
#81868=CARTESIAN_POINT('Ctrl Pts',(100.751091323793,1.58458405733109,48.5));
#81869=CARTESIAN_POINT('Ctrl Pts',(100.751091323793,1.58458405733109,48.35));
#81870=CARTESIAN_POINT('Ctrl Pts',(100.937175832689,1.58458405733109,48.5));
#81871=CARTESIAN_POINT('Ctrl Pts',(100.937175832689,1.58458405733109,48.35));
#81872=CARTESIAN_POINT('Ctrl Pts',(101.063983522356,1.76466578245163,48.5));
#81873=CARTESIAN_POINT('Ctrl Pts',(101.063983522356,1.76466578245163,48.35));
#81874=CARTESIAN_POINT('',(100.751091323793,1.58458405733109,48.5));
#81875=CARTESIAN_POINT('Ctrl Pts',(100.751091323793,1.58458405733109,48.5));
#81876=CARTESIAN_POINT('Ctrl Pts',(100.937175832689,1.58458405733109,48.5));
#81877=CARTESIAN_POINT('Ctrl Pts',(101.063983522356,1.76466578245163,48.5));
#81878=CARTESIAN_POINT('',(100.751091323793,1.58458405733109,48.35));
#81879=CARTESIAN_POINT('',(100.751091323793,1.58458405733109,48.5));
#81880=CARTESIAN_POINT('Ctrl Pts',(100.751091323793,1.58458405733109,48.35));
#81881=CARTESIAN_POINT('Ctrl Pts',(100.937175832689,1.58458405733109,48.35));
#81882=CARTESIAN_POINT('Ctrl Pts',(101.063983522356,1.76466578245163,48.35));
#81883=CARTESIAN_POINT('Ctrl Pts',(100.43819912523,1.76391565799713,48.5));
#81884=CARTESIAN_POINT('Ctrl Pts',(100.43819912523,1.76391565799713,48.35));
#81885=CARTESIAN_POINT('Ctrl Pts',(100.565006814897,1.58458405733109,48.5));
#81886=CARTESIAN_POINT('Ctrl Pts',(100.565006814897,1.58458405733109,48.35));
#81887=CARTESIAN_POINT('Ctrl Pts',(100.751091323793,1.58458405733109,48.5));
#81888=CARTESIAN_POINT('Ctrl Pts',(100.751091323793,1.58458405733109,48.35));
#81889=CARTESIAN_POINT('',(100.43819912523,1.76391565799713,48.5));
#81890=CARTESIAN_POINT('Ctrl Pts',(100.43819912523,1.76391565799713,48.5));
#81891=CARTESIAN_POINT('Ctrl Pts',(100.565006814897,1.58458405733109,48.5));
#81892=CARTESIAN_POINT('Ctrl Pts',(100.751091323793,1.58458405733109,48.5));
#81893=CARTESIAN_POINT('',(100.43819912523,1.76391565799713,48.35));
#81894=CARTESIAN_POINT('',(100.43819912523,1.76391565799713,48.5));
#81895=CARTESIAN_POINT('Ctrl Pts',(100.43819912523,1.76391565799713,48.35));
#81896=CARTESIAN_POINT('Ctrl Pts',(100.565006814897,1.58458405733109,48.35));
#81897=CARTESIAN_POINT('Ctrl Pts',(100.751091323793,1.58458405733109,48.35));
#81898=CARTESIAN_POINT('Ctrl Pts',(100.311391435564,2.48499327898026,48.5));
#81899=CARTESIAN_POINT('Ctrl Pts',(100.311391435564,2.48499327898026,48.35));
#81900=CARTESIAN_POINT('Ctrl Pts',(100.311391435564,1.94324696063995,48.5));
#81901=CARTESIAN_POINT('Ctrl Pts',(100.311391435564,1.94324696063995,48.35));
#81902=CARTESIAN_POINT('Ctrl Pts',(100.43819912523,1.76391565799713,48.5));
#81903=CARTESIAN_POINT('Ctrl Pts',(100.43819912523,1.76391565799713,48.35));
#81904=CARTESIAN_POINT('',(100.311391435564,2.48499327898026,48.5));
#81905=CARTESIAN_POINT('Ctrl Pts',(100.311391435564,2.48499327898026,48.5));
#81906=CARTESIAN_POINT('Ctrl Pts',(100.311391435564,1.94324696063995,48.5));
#81907=CARTESIAN_POINT('Ctrl Pts',(100.43819912523,1.76391565799713,48.5));
#81908=CARTESIAN_POINT('',(100.311391435564,2.48499327898026,48.35));
#81909=CARTESIAN_POINT('',(100.311391435564,2.48499327898026,48.5));
#81910=CARTESIAN_POINT('Ctrl Pts',(100.311391435564,2.48499327898026,48.35));
#81911=CARTESIAN_POINT('Ctrl Pts',(100.311391435564,1.94324696063995,48.35));
#81912=CARTESIAN_POINT('Ctrl Pts',(100.43819912523,1.76391565799713,48.35));
#81913=CARTESIAN_POINT('Ctrl Pts',(100.450955115259,3.22783091664314,48.5));
#81914=CARTESIAN_POINT('Ctrl Pts',(100.450955115259,3.22783091664314,48.35));
#81915=CARTESIAN_POINT('Ctrl Pts',(100.311391435564,3.02673944830894,48.5));
#81916=CARTESIAN_POINT('Ctrl Pts',(100.311391435564,3.02673944830894,48.35));
#81917=CARTESIAN_POINT('Ctrl Pts',(100.311391435564,2.48499327898026,48.5));
#81918=CARTESIAN_POINT('Ctrl Pts',(100.311391435564,2.48499327898026,48.35));
#81919=CARTESIAN_POINT('Ctrl Pts',(100.450955115259,3.22783091664314,48.5));
#81920=CARTESIAN_POINT('Ctrl Pts',(100.311391435564,3.02673944830894,48.5));
#81921=CARTESIAN_POINT('Ctrl Pts',(100.311391435564,2.48499327898026,48.5));
#81922=CARTESIAN_POINT('Ctrl Pts',(100.450955115259,3.22783091664314,48.35));
#81923=CARTESIAN_POINT('Ctrl Pts',(100.311391435564,3.02673944830894,48.35));
#81924=CARTESIAN_POINT('Ctrl Pts',(100.311391435564,2.48499327898026,48.35));
#81925=CARTESIAN_POINT('Ctrl Pts',(100.751091323793,1.36248314380646,48.5));
#81926=CARTESIAN_POINT('Ctrl Pts',(100.751091323793,1.36248314380646,48.35));
#81927=CARTESIAN_POINT('Ctrl Pts',(100.432946763933,1.36248314380646,48.5));
#81928=CARTESIAN_POINT('Ctrl Pts',(100.432946763933,1.36248314380646,48.35));
#81929=CARTESIAN_POINT('Ctrl Pts',(100.251364193857,1.59058684110642,48.5));
#81930=CARTESIAN_POINT('Ctrl Pts',(100.251364193857,1.59058684110642,48.35));
#81931=CARTESIAN_POINT('',(100.751091323793,1.36248314380646,48.5));
#81932=CARTESIAN_POINT('',(100.251364193857,1.59058684110642,48.5));
#81933=CARTESIAN_POINT('Ctrl Pts',(100.751091323793,1.36248314380646,48.5));
#81934=CARTESIAN_POINT('Ctrl Pts',(100.432946763933,1.36248314380646,48.5));
#81935=CARTESIAN_POINT('Ctrl Pts',(100.251364193857,1.59058684110642,48.5));
#81936=CARTESIAN_POINT('',(100.751091323793,1.36248314380646,48.35));
#81937=CARTESIAN_POINT('',(100.751091323793,1.36248314380646,48.5));
#81938=CARTESIAN_POINT('',(100.251364193857,1.59058684110642,48.35));
#81939=CARTESIAN_POINT('Ctrl Pts',(100.751091323793,1.36248314380646,48.35));
#81940=CARTESIAN_POINT('Ctrl Pts',(100.432946763933,1.36248314380646,48.35));
#81941=CARTESIAN_POINT('Ctrl Pts',(100.251364193857,1.59058684110642,48.35));
#81942=CARTESIAN_POINT('',(100.251364193857,1.59058684110642,48.5));
#81943=CARTESIAN_POINT('Ctrl Pts',(101.151022993028,1.49229192733765,48.5));
#81944=CARTESIAN_POINT('Ctrl Pts',(101.151022993028,1.49229192733765,48.35));
#81945=CARTESIAN_POINT('Ctrl Pts',(100.992701135576,1.36248314380646,48.5));
#81946=CARTESIAN_POINT('Ctrl Pts',(100.992701135576,1.36248314380646,48.35));
#81947=CARTESIAN_POINT('Ctrl Pts',(100.751091323793,1.36248314380646,48.5));
#81948=CARTESIAN_POINT('Ctrl Pts',(100.751091323793,1.36248314380646,48.35));
#81949=CARTESIAN_POINT('',(101.151022993028,1.49229192733765,48.5));
#81950=CARTESIAN_POINT('Ctrl Pts',(101.151022993028,1.49229192733765,48.5));
#81951=CARTESIAN_POINT('Ctrl Pts',(100.992701135576,1.36248314380646,48.5));
#81952=CARTESIAN_POINT('Ctrl Pts',(100.751091323793,1.36248314380646,48.5));
#81953=CARTESIAN_POINT('',(101.151022993028,1.49229192733765,48.35));
#81954=CARTESIAN_POINT('',(101.151022993028,1.49229192733765,48.5));
#81955=CARTESIAN_POINT('Ctrl Pts',(101.151022993028,1.49229192733765,48.35));
#81956=CARTESIAN_POINT('Ctrl Pts',(100.992701135576,1.36248314380646,48.35));
#81957=CARTESIAN_POINT('Ctrl Pts',(100.751091323793,1.36248314380646,48.35));
#81958=CARTESIAN_POINT('Ctrl Pts',(101.388881288469,1.85995900630951,48.5));
#81959=CARTESIAN_POINT('Ctrl Pts',(101.388881288469,1.85995900630951,48.35));
#81960=CARTESIAN_POINT('Ctrl Pts',(101.309344850481,1.62210100889206,48.5));
#81961=CARTESIAN_POINT('Ctrl Pts',(101.309344850481,1.62210100889206,48.35));
#81962=CARTESIAN_POINT('Ctrl Pts',(101.151022993028,1.49229192733765,48.5));
#81963=CARTESIAN_POINT('Ctrl Pts',(101.151022993028,1.49229192733765,48.35));
#81964=CARTESIAN_POINT('',(101.388881288469,1.85995900630951,48.5));
#81965=CARTESIAN_POINT('Ctrl Pts',(101.388881288469,1.85995900630951,48.5));
#81966=CARTESIAN_POINT('Ctrl Pts',(101.309344850481,1.62210100889206,48.5));
#81967=CARTESIAN_POINT('Ctrl Pts',(101.151022993028,1.49229192733765,48.5));
#81968=CARTESIAN_POINT('',(101.388881288469,1.85995900630951,48.35));
#81969=CARTESIAN_POINT('',(101.388881288469,1.85995900630951,48.5));
#81970=CARTESIAN_POINT('Ctrl Pts',(101.388881288469,1.85995900630951,48.35));
#81971=CARTESIAN_POINT('Ctrl Pts',(101.309344850481,1.62210100889206,48.35));
#81972=CARTESIAN_POINT('Ctrl Pts',(101.151022993028,1.49229192733765,48.35));
#81973=CARTESIAN_POINT('Ctrl Pts',(101.468417130411,2.48499327898026,48.5));
#81974=CARTESIAN_POINT('Ctrl Pts',(101.468417130411,2.48499327898026,48.35));
#81975=CARTESIAN_POINT('Ctrl Pts',(101.468417130411,2.09781730175018,48.5));
#81976=CARTESIAN_POINT('Ctrl Pts',(101.468417130411,2.09781730175018,48.35));
#81977=CARTESIAN_POINT('Ctrl Pts',(101.388881288469,1.85995900630951,48.5));
#81978=CARTESIAN_POINT('Ctrl Pts',(101.388881288469,1.85995900630951,48.35));
#81979=CARTESIAN_POINT('',(101.468417130411,2.48499327898026,48.5));
#81980=CARTESIAN_POINT('Ctrl Pts',(101.468417130411,2.48499327898026,48.5));
#81981=CARTESIAN_POINT('Ctrl Pts',(101.468417130411,2.09781730175018,48.5));
#81982=CARTESIAN_POINT('Ctrl Pts',(101.388881288469,1.85995900630951,48.5));
#81983=CARTESIAN_POINT('',(101.468417130411,2.48499327898026,48.35));
#81984=CARTESIAN_POINT('',(101.468417130411,2.48499327898026,48.5));
#81985=CARTESIAN_POINT('Ctrl Pts',(101.468417130411,2.48499327898026,48.35));
#81986=CARTESIAN_POINT('Ctrl Pts',(101.468417130411,2.09781730175018,48.35));
#81987=CARTESIAN_POINT('Ctrl Pts',(101.388881288469,1.85995900630951,48.35));
#81988=CARTESIAN_POINT('Ctrl Pts',(101.418894611299,3.00497958064079,48.5));
#81989=CARTESIAN_POINT('Ctrl Pts',(101.418894611299,3.00497958064079,48.35));
#81990=CARTESIAN_POINT('Ctrl Pts',(101.468417130411,2.81214186549187,48.5));
#81991=CARTESIAN_POINT('Ctrl Pts',(101.468417130411,2.81214186549187,48.35));
#81992=CARTESIAN_POINT('Ctrl Pts',(101.468417130411,2.48499327898026,48.5));
#81993=CARTESIAN_POINT('Ctrl Pts',(101.468417130411,2.48499327898026,48.35));
#81994=CARTESIAN_POINT('',(101.418894611299,3.00497958064079,48.5));
#81995=CARTESIAN_POINT('Ctrl Pts',(101.418894611299,3.00497958064079,48.5));
#81996=CARTESIAN_POINT('Ctrl Pts',(101.468417130411,2.81214186549187,48.5));
#81997=CARTESIAN_POINT('Ctrl Pts',(101.468417130411,2.48499327898026,48.5));
#81998=CARTESIAN_POINT('',(101.418894611299,3.00497958064079,48.35));
#81999=CARTESIAN_POINT('',(101.418894611299,3.00497958064079,48.5));
#82000=CARTESIAN_POINT('Ctrl Pts',(101.418894611299,3.00497958064079,48.35));
#82001=CARTESIAN_POINT('Ctrl Pts',(101.468417130411,2.81214186549187,48.35));
#82002=CARTESIAN_POINT('Ctrl Pts',(101.468417130411,2.48499327898026,48.35));
#82003=CARTESIAN_POINT('Ctrl Pts',(101.282332621515,3.33212831616402,48.5));
#82004=CARTESIAN_POINT('Ctrl Pts',(101.282332621515,3.33212831616402,48.35));
#82005=CARTESIAN_POINT('Ctrl Pts',(101.369372092187,3.19781729578972,48.5));
#82006=CARTESIAN_POINT('Ctrl Pts',(101.369372092187,3.19781729578972,48.35));
#82007=CARTESIAN_POINT('Ctrl Pts',(101.418894611299,3.00497958064079,48.5));
#82008=CARTESIAN_POINT('Ctrl Pts',(101.418894611299,3.00497958064079,48.35));
#82009=CARTESIAN_POINT('',(101.282332621515,3.33212831616402,48.5));
#82010=CARTESIAN_POINT('Ctrl Pts',(101.282332621515,3.33212831616402,48.5));
#82011=CARTESIAN_POINT('Ctrl Pts',(101.369372092187,3.19781729578972,48.5));
#82012=CARTESIAN_POINT('Ctrl Pts',(101.418894611299,3.00497958064079,48.5));
#82013=CARTESIAN_POINT('',(101.282332621515,3.33212831616402,48.35));
#82014=CARTESIAN_POINT('',(101.282332621515,3.33212831616402,48.5));
#82015=CARTESIAN_POINT('Ctrl Pts',(101.282332621515,3.33212831616402,48.35));
#82016=CARTESIAN_POINT('Ctrl Pts',(101.369372092187,3.19781729578972,48.35));
#82017=CARTESIAN_POINT('Ctrl Pts',(101.418894611299,3.00497958064079,48.35));
#82018=CARTESIAN_POINT('Ctrl Pts',(101.061732850969,3.5377217233181,48.5));
#82019=CARTESIAN_POINT('Ctrl Pts',(101.061732850969,3.5377217233181,48.35));
#82020=CARTESIAN_POINT('Ctrl Pts',(101.195293150842,3.46643933653831,48.5));
#82021=CARTESIAN_POINT('Ctrl Pts',(101.195293150842,3.46643933653831,48.35));
#82022=CARTESIAN_POINT('Ctrl Pts',(101.282332621515,3.33212831616402,48.5));
#82023=CARTESIAN_POINT('Ctrl Pts',(101.282332621515,3.33212831616402,48.35));
#82024=CARTESIAN_POINT('',(101.061732850969,3.5377217233181,48.5));
#82025=CARTESIAN_POINT('Ctrl Pts',(101.061732850969,3.5377217233181,48.5));
#82026=CARTESIAN_POINT('Ctrl Pts',(101.195293150842,3.46643933653831,48.5));
#82027=CARTESIAN_POINT('Ctrl Pts',(101.282332621515,3.33212831616402,48.5));
#82028=CARTESIAN_POINT('',(101.061732850969,3.5377217233181,48.35));
#82029=CARTESIAN_POINT('',(101.061732850969,3.5377217233181,48.5));
#82030=CARTESIAN_POINT('Ctrl Pts',(101.061732850969,3.5377217233181,48.35));
#82031=CARTESIAN_POINT('Ctrl Pts',(101.195293150842,3.46643933653831,48.35));
#82032=CARTESIAN_POINT('Ctrl Pts',(101.282332621515,3.33212831616402,48.35));
#82033=CARTESIAN_POINT('Ctrl Pts',(100.751091323793,3.60900411009789,48.5));
#82034=CARTESIAN_POINT('Ctrl Pts',(100.751091323793,3.60900411009789,48.35));
#82035=CARTESIAN_POINT('Ctrl Pts',(100.928171955049,3.60900411009789,48.5));
#82036=CARTESIAN_POINT('Ctrl Pts',(100.928171955049,3.60900411009789,48.35));
#82037=CARTESIAN_POINT('Ctrl Pts',(101.061732850969,3.5377217233181,48.5));
#82038=CARTESIAN_POINT('Ctrl Pts',(101.061732850969,3.5377217233181,48.35));
#82039=CARTESIAN_POINT('',(100.751091323793,3.60900411009789,48.5));
#82040=CARTESIAN_POINT('Ctrl Pts',(100.751091323793,3.60900411009789,48.5));
#82041=CARTESIAN_POINT('Ctrl Pts',(100.928171955049,3.60900411009789,48.5));
#82042=CARTESIAN_POINT('Ctrl Pts',(101.061732850969,3.5377217233181,48.5));
#82043=CARTESIAN_POINT('',(100.751091323793,3.60900411009789,48.35));
#82044=CARTESIAN_POINT('',(100.751091323793,3.60900411009789,48.5));
#82045=CARTESIAN_POINT('Ctrl Pts',(100.751091323793,3.60900411009789,48.35));
#82046=CARTESIAN_POINT('Ctrl Pts',(100.928171955049,3.60900411009789,48.35));
#82047=CARTESIAN_POINT('Ctrl Pts',(101.061732850969,3.5377217233181,48.35));
#82048=CARTESIAN_POINT('Ctrl Pts',(100.352660499513,3.47994545102119,48.5));
#82049=CARTESIAN_POINT('Ctrl Pts',(100.352660499513,3.47994545102119,48.35));
#82050=CARTESIAN_POINT('Ctrl Pts',(100.510982356966,3.60900411009789,48.5));
#82051=CARTESIAN_POINT('Ctrl Pts',(100.510982356966,3.60900411009789,48.35));
#82052=CARTESIAN_POINT('Ctrl Pts',(100.751091323793,3.60900411009789,48.5));
#82053=CARTESIAN_POINT('Ctrl Pts',(100.751091323793,3.60900411009789,48.35));
#82054=CARTESIAN_POINT('',(100.352660499513,3.47994545102119,48.5));
#82055=CARTESIAN_POINT('Ctrl Pts',(100.352660499513,3.47994545102119,48.5));
#82056=CARTESIAN_POINT('Ctrl Pts',(100.510982356966,3.60900411009789,48.5));
#82057=CARTESIAN_POINT('Ctrl Pts',(100.751091323793,3.60900411009789,48.5));
#82058=CARTESIAN_POINT('',(100.352660499513,3.47994545102119,48.35));
#82059=CARTESIAN_POINT('',(100.352660499513,3.47994545102119,48.5));
#82060=CARTESIAN_POINT('Ctrl Pts',(100.352660499513,3.47994545102119,48.35));
#82061=CARTESIAN_POINT('Ctrl Pts',(100.510982356966,3.60900411009789,48.35));
#82062=CARTESIAN_POINT('Ctrl Pts',(100.751091323793,3.60900411009789,48.35));
#82063=CARTESIAN_POINT('Ctrl Pts',(100.114051781595,3.11302864551544,48.5));
#82064=CARTESIAN_POINT('Ctrl Pts',(100.114051781595,3.11302864551544,48.35));
#82065=CARTESIAN_POINT('Ctrl Pts',(100.194338344038,3.3508867919445,48.5));
#82066=CARTESIAN_POINT('Ctrl Pts',(100.194338344038,3.3508867919445,48.35));
#82067=CARTESIAN_POINT('Ctrl Pts',(100.352660499513,3.47994545102119,48.5));
#82068=CARTESIAN_POINT('Ctrl Pts',(100.352660499513,3.47994545102119,48.35));
#82069=CARTESIAN_POINT('',(100.114051781595,3.11302864551544,48.5));
#82070=CARTESIAN_POINT('Ctrl Pts',(100.114051781595,3.11302864551544,48.5));
#82071=CARTESIAN_POINT('Ctrl Pts',(100.194338344038,3.3508867919445,48.5));
#82072=CARTESIAN_POINT('Ctrl Pts',(100.352660499513,3.47994545102119,48.5));
#82073=CARTESIAN_POINT('',(100.114051781595,3.11302864551544,48.35));
#82074=CARTESIAN_POINT('',(100.114051781595,3.11302864551544,48.5));
#82075=CARTESIAN_POINT('Ctrl Pts',(100.114051781595,3.11302864551544,48.35));
#82076=CARTESIAN_POINT('Ctrl Pts',(100.194338344038,3.3508867919445,48.35));
#82077=CARTESIAN_POINT('Ctrl Pts',(100.352660499513,3.47994545102119,48.35));
#82078=CARTESIAN_POINT('Ctrl Pts',(100.033765517175,2.48499327898026,48.5));
#82079=CARTESIAN_POINT('Ctrl Pts',(100.033765517175,2.48499327898026,48.35));
#82080=CARTESIAN_POINT('Ctrl Pts',(100.033765517175,2.87517049908638,48.5));
#82081=CARTESIAN_POINT('Ctrl Pts',(100.033765517175,2.87517049908638,48.35));
#82082=CARTESIAN_POINT('Ctrl Pts',(100.114051781595,3.11302864551544,48.5));
#82083=CARTESIAN_POINT('Ctrl Pts',(100.114051781595,3.11302864551544,48.35));
#82084=CARTESIAN_POINT('',(100.033765517175,2.48499327898026,48.5));
#82085=CARTESIAN_POINT('Ctrl Pts',(100.033765517175,2.48499327898026,48.5));
#82086=CARTESIAN_POINT('Ctrl Pts',(100.033765517175,2.87517049908638,48.5));
#82087=CARTESIAN_POINT('Ctrl Pts',(100.114051781595,3.11302864551544,48.5));
#82088=CARTESIAN_POINT('',(100.033765517175,2.48499327898026,48.35));
#82089=CARTESIAN_POINT('',(100.033765517175,2.48499327898026,48.5));
#82090=CARTESIAN_POINT('Ctrl Pts',(100.033765517175,2.48499327898026,48.35));
#82091=CARTESIAN_POINT('Ctrl Pts',(100.033765517175,2.87517049908638,48.35));
#82092=CARTESIAN_POINT('Ctrl Pts',(100.114051781595,3.11302864551544,48.35));
#82093=CARTESIAN_POINT('Ctrl Pts',(100.251364193857,1.59058684110642,48.5));
#82094=CARTESIAN_POINT('Ctrl Pts',(100.251364193857,1.59058684110642,48.35));
#82095=CARTESIAN_POINT('Ctrl Pts',(100.033765517175,1.86521166563034,48.5));
#82096=CARTESIAN_POINT('Ctrl Pts',(100.033765517175,1.86521166563034,48.35));
#82097=CARTESIAN_POINT('Ctrl Pts',(100.033765517175,2.48499327898026,48.5));
#82098=CARTESIAN_POINT('Ctrl Pts',(100.033765517175,2.48499327898026,48.35));
#82099=CARTESIAN_POINT('Ctrl Pts',(100.251364193857,1.59058684110642,48.5));
#82100=CARTESIAN_POINT('Ctrl Pts',(100.033765517175,1.86521166563034,48.5));
#82101=CARTESIAN_POINT('Ctrl Pts',(100.033765517175,2.48499327898026,48.5));
#82102=CARTESIAN_POINT('Ctrl Pts',(100.251364193857,1.59058684110642,48.35));
#82103=CARTESIAN_POINT('Ctrl Pts',(100.033765517175,1.86521166563034,48.35));
#82104=CARTESIAN_POINT('Ctrl Pts',(100.033765517175,2.48499327898026,48.35));
#82105=CARTESIAN_POINT('Origin',(99.999999858439,2.48574362695217,48.35));
#82106=CARTESIAN_POINT('Origin',(99.1678718551993,3.60900411009789,48.5));
#82107=CARTESIAN_POINT('',(99.1678718551993,3.60900411009789,48.5));
#82108=CARTESIAN_POINT('',(99.3419510945678,3.60900411009789,48.5));
#82109=CARTESIAN_POINT('',(49.5839359275997,3.60900411009789,48.5));
#82110=CARTESIAN_POINT('',(99.1678718551993,3.60900411009789,48.35));
#82111=CARTESIAN_POINT('',(99.1678718551993,3.60900411009789,48.5));
#82112=CARTESIAN_POINT('',(99.3419510945678,3.60900411009789,48.35));
#82113=CARTESIAN_POINT('',(99.1678718551993,3.60900411009789,48.35));
#82114=CARTESIAN_POINT('',(99.3419510945678,3.60900411009789,48.5));
#82115=CARTESIAN_POINT('Ctrl Pts',(98.9277627393603,3.31487053632736,48.5));
#82116=CARTESIAN_POINT('Ctrl Pts',(98.9277627393603,3.31487053632736,48.35));
#82117=CARTESIAN_POINT('Ctrl Pts',(99.0973397418857,3.46643933653831,48.5));
#82118=CARTESIAN_POINT('Ctrl Pts',(99.0973397418857,3.46643933653831,48.35));
#82119=CARTESIAN_POINT('Ctrl Pts',(99.1678718551993,3.60900411009789,48.5));
#82120=CARTESIAN_POINT('Ctrl Pts',(99.1678718551993,3.60900411009789,48.35));
#82121=CARTESIAN_POINT('',(98.9277627393603,3.31487053632736,48.5));
#82122=CARTESIAN_POINT('Ctrl Pts',(98.9277627393603,3.31487053632736,48.5));
#82123=CARTESIAN_POINT('Ctrl Pts',(99.0973397418857,3.46643933653831,48.5));
#82124=CARTESIAN_POINT('Ctrl Pts',(99.1678718551993,3.60900411009789,48.5));
#82125=CARTESIAN_POINT('',(98.9277627393603,3.31487053632736,48.35));
#82126=CARTESIAN_POINT('',(98.9277627393603,3.31487053632736,48.5));
#82127=CARTESIAN_POINT('Ctrl Pts',(98.9277627393603,3.31487053632736,48.35));
#82128=CARTESIAN_POINT('Ctrl Pts',(99.0973397418857,3.46643933653831,48.35));
#82129=CARTESIAN_POINT('Ctrl Pts',(99.1678718551993,3.60900411009789,48.35));
#82130=CARTESIAN_POINT('Ctrl Pts',(98.5315825864673,3.05675321817398,48.5));
#82131=CARTESIAN_POINT('Ctrl Pts',(98.5315825864673,3.05675321817398,48.35));
#82132=CARTESIAN_POINT('Ctrl Pts',(98.7581855878234,3.1633015871048,48.5));
#82133=CARTESIAN_POINT('Ctrl Pts',(98.7581855878234,3.1633015871048,48.35));
#82134=CARTESIAN_POINT('Ctrl Pts',(98.9277627393603,3.31487053632736,48.5));
#82135=CARTESIAN_POINT('Ctrl Pts',(98.9277627393603,3.31487053632736,48.35));
#82136=CARTESIAN_POINT('',(98.5315825864673,3.05675321817398,48.5));
#82137=CARTESIAN_POINT('Ctrl Pts',(98.5315825864673,3.05675321817398,48.5));
#82138=CARTESIAN_POINT('Ctrl Pts',(98.7581855878234,3.1633015871048,48.5));
#82139=CARTESIAN_POINT('Ctrl Pts',(98.9277627393603,3.31487053632736,48.5));
#82140=CARTESIAN_POINT('',(98.5315825864673,3.05675321817398,48.35));
#82141=CARTESIAN_POINT('',(98.5315825864673,3.05675321817398,48.5));
#82142=CARTESIAN_POINT('Ctrl Pts',(98.5315825864673,3.05675321817398,48.35));
#82143=CARTESIAN_POINT('Ctrl Pts',(98.7581855878234,3.1633015871048,48.35));
#82144=CARTESIAN_POINT('Ctrl Pts',(98.9277627393603,3.31487053632736,48.35));
#82145=CARTESIAN_POINT('Origin',(98.5315825864673,2.79563450813293,48.5));
#82146=CARTESIAN_POINT('',(98.5315825864673,2.79563450813293,48.5));
#82147=CARTESIAN_POINT('',(98.5315825864673,5.39781725406647,48.5));
#82148=CARTESIAN_POINT('',(98.5315825864673,2.79563450813293,48.35));
#82149=CARTESIAN_POINT('',(98.5315825864673,2.79563450813293,48.5));
#82150=CARTESIAN_POINT('',(98.5315825864673,2.79563450813293,48.35));
#82151=CARTESIAN_POINT('Ctrl Pts',(98.8159618601203,2.93519788980484,48.5));
#82152=CARTESIAN_POINT('Ctrl Pts',(98.8159618601203,2.93519788980484,48.35));
#82153=CARTESIAN_POINT('Ctrl Pts',(98.6576400026679,2.8421556353569,48.5));
#82154=CARTESIAN_POINT('Ctrl Pts',(98.6576400026679,2.8421556353569,48.35));
#82155=CARTESIAN_POINT('Ctrl Pts',(98.5315825864673,2.79563450813293,48.5));
#82156=CARTESIAN_POINT('Ctrl Pts',(98.5315825864673,2.79563450813293,48.35));
#82157=CARTESIAN_POINT('',(98.8159618601203,2.93519788980484,48.5));
#82158=CARTESIAN_POINT('Ctrl Pts',(98.8159618601203,2.93519788980484,48.5));
#82159=CARTESIAN_POINT('Ctrl Pts',(98.6576400026679,2.8421556353569,48.5));
#82160=CARTESIAN_POINT('Ctrl Pts',(98.5315825864673,2.79563450813293,48.5));
#82161=CARTESIAN_POINT('',(98.8159618601203,2.93519788980484,48.35));
#82162=CARTESIAN_POINT('',(98.8159618601203,2.93519788980484,48.5));
#82163=CARTESIAN_POINT('Ctrl Pts',(98.8159618601203,2.93519788980484,48.35));
#82164=CARTESIAN_POINT('Ctrl Pts',(98.6576400026679,2.8421556353569,48.35));
#82165=CARTESIAN_POINT('Ctrl Pts',(98.5315825864673,2.79563450813293,48.35));
#82166=CARTESIAN_POINT('Ctrl Pts',(99.0718282088637,3.12128254771233,48.5));
#82167=CARTESIAN_POINT('Ctrl Pts',(99.0718282088637,3.12128254771233,48.35));
#82168=CARTESIAN_POINT('Ctrl Pts',(98.9742838665843,3.02824014425278,48.5));
#82169=CARTESIAN_POINT('Ctrl Pts',(98.9742838665843,3.02824014425278,48.35));
#82170=CARTESIAN_POINT('Ctrl Pts',(98.8159618601203,2.93519788980484,48.5));
#82171=CARTESIAN_POINT('Ctrl Pts',(98.8159618601203,2.93519788980484,48.35));
#82172=CARTESIAN_POINT('',(99.0718282088637,3.12128254771233,48.5));
#82173=CARTESIAN_POINT('Ctrl Pts',(99.0718282088637,3.12128254771233,48.5));
#82174=CARTESIAN_POINT('Ctrl Pts',(98.9742838665843,3.02824014425278,48.5));
#82175=CARTESIAN_POINT('Ctrl Pts',(98.8159618601203,2.93519788980484,48.5));
#82176=CARTESIAN_POINT('',(99.0718282088637,3.12128254771233,48.35));
#82177=CARTESIAN_POINT('',(99.0718282088637,3.12128254771233,48.5));
#82178=CARTESIAN_POINT('Ctrl Pts',(99.0718282088637,3.12128254771233,48.35));
#82179=CARTESIAN_POINT('Ctrl Pts',(98.9742838665843,3.02824014425278,48.35));
#82180=CARTESIAN_POINT('Ctrl Pts',(98.8159618601203,2.93519788980484,48.35));
#82181=CARTESIAN_POINT('Origin',(99.0718282088637,1.40000009536743,48.5));
#82182=CARTESIAN_POINT('',(99.0718282088637,1.40000009536743,48.5));
#82183=CARTESIAN_POINT('',(99.0718282088637,4.70000004768372,48.5));
#82184=CARTESIAN_POINT('',(99.0718282088637,1.40000009536743,48.35));
#82185=CARTESIAN_POINT('',(99.0718282088637,1.40000009536743,48.5));
#82186=CARTESIAN_POINT('',(99.0718282088637,1.40000009536743,48.35));
#82187=CARTESIAN_POINT('Origin',(99.3419510945678,1.40000009536743,48.5));
#82188=CARTESIAN_POINT('',(99.3419510945678,1.40000009536743,48.5));
#82189=CARTESIAN_POINT('',(49.6709755472839,1.40000009536743,48.5));
#82190=CARTESIAN_POINT('',(99.3419510945678,1.40000009536743,48.35));
#82191=CARTESIAN_POINT('',(99.3419510945678,1.40000009536743,48.5));
#82192=CARTESIAN_POINT('',(99.3419510945678,1.40000009536743,48.35));
#82193=CARTESIAN_POINT('Origin',(99.3419510945678,3.60900411009789,48.5));
#82194=CARTESIAN_POINT('',(99.3419510945678,5.80450205504894,48.5));
#82195=CARTESIAN_POINT('',(99.3419510945678,3.60900411009789,48.35));
#82196=CARTESIAN_POINT('Origin',(99.999999858439,2.48574362695217,48.35));
#82197=CARTESIAN_POINT('Origin',(0.,8.,48.5));
#82198=CARTESIAN_POINT('Ctrl Pts',(90.8703956548125,3.38540250062943,48.5));
#82199=CARTESIAN_POINT('Ctrl Pts',(90.8703956548125,3.38540250062943,48.35));
#82200=CARTESIAN_POINT('Ctrl Pts',(90.6843108478934,3.38540250062943,48.5));
#82201=CARTESIAN_POINT('Ctrl Pts',(90.6843108478934,3.38540250062943,48.35));
#82202=CARTESIAN_POINT('Ctrl Pts',(90.5732605401427,3.22783091664314,48.5));
#82203=CARTESIAN_POINT('Ctrl Pts',(90.5732605401427,3.22783091664314,48.35));
#82204=CARTESIAN_POINT('',(90.8703956548125,3.38540250062943,48.5));
#82205=CARTESIAN_POINT('',(90.5732605401427,3.22783091664314,48.5));
#82206=CARTESIAN_POINT('Ctrl Pts',(90.8703956548125,3.38540250062943,48.5));
#82207=CARTESIAN_POINT('Ctrl Pts',(90.6843108478934,3.38540250062943,48.5));
#82208=CARTESIAN_POINT('Ctrl Pts',(90.5732605401427,3.22783091664314,48.5));
#82209=CARTESIAN_POINT('',(90.8703956548125,3.38540250062943,48.35));
#82210=CARTESIAN_POINT('',(90.8703956548125,3.38540250062943,48.5));
#82211=CARTESIAN_POINT('',(90.5732605401427,3.22783091664314,48.35));
#82212=CARTESIAN_POINT('Ctrl Pts',(90.8703956548125,3.38540250062943,48.35));
#82213=CARTESIAN_POINT('Ctrl Pts',(90.6843108478934,3.38540250062943,48.35));
#82214=CARTESIAN_POINT('Ctrl Pts',(90.5732605401427,3.22783091664314,48.35));
#82215=CARTESIAN_POINT('',(90.5732605401427,3.22783091664314,48.5));
#82216=CARTESIAN_POINT('Ctrl Pts',(91.1862889472395,3.2068213224411,48.5));
#82217=CARTESIAN_POINT('Ctrl Pts',(91.1862889472395,3.2068213224411,48.35));
#82218=CARTESIAN_POINT('Ctrl Pts',(91.0594812575728,3.38540250062943,48.5));
#82219=CARTESIAN_POINT('Ctrl Pts',(91.0594812575728,3.38540250062943,48.35));
#82220=CARTESIAN_POINT('Ctrl Pts',(90.8703956548125,3.38540250062943,48.5));
#82221=CARTESIAN_POINT('Ctrl Pts',(90.8703956548125,3.38540250062943,48.35));
#82222=CARTESIAN_POINT('',(91.1862889472395,3.2068213224411,48.5));
#82223=CARTESIAN_POINT('Ctrl Pts',(91.1862889472395,3.2068213224411,48.5));
#82224=CARTESIAN_POINT('Ctrl Pts',(91.0594812575728,3.38540250062943,48.5));
#82225=CARTESIAN_POINT('Ctrl Pts',(90.8703956548125,3.38540250062943,48.5));
#82226=CARTESIAN_POINT('',(91.1862889472395,3.2068213224411,48.35));
#82227=CARTESIAN_POINT('',(91.1862889472395,3.2068213224411,48.5));
#82228=CARTESIAN_POINT('Ctrl Pts',(91.1862889472395,3.2068213224411,48.35));
#82229=CARTESIAN_POINT('Ctrl Pts',(91.0594812575728,3.38540250062943,48.35));
#82230=CARTESIAN_POINT('Ctrl Pts',(90.8703956548125,3.38540250062943,48.35));
#82231=CARTESIAN_POINT('Ctrl Pts',(91.3130966369063,2.48499327898026,48.5));
#82232=CARTESIAN_POINT('Ctrl Pts',(91.3130966369063,2.48499327898026,48.35));
#82233=CARTESIAN_POINT('Ctrl Pts',(91.3130966369063,3.02824014425278,48.5));
#82234=CARTESIAN_POINT('Ctrl Pts',(91.3130966369063,3.02824014425278,48.35));
#82235=CARTESIAN_POINT('Ctrl Pts',(91.1862889472395,3.2068213224411,48.5));
#82236=CARTESIAN_POINT('Ctrl Pts',(91.1862889472395,3.2068213224411,48.35));
#82237=CARTESIAN_POINT('',(91.3130966369063,2.48499327898026,48.5));
#82238=CARTESIAN_POINT('Ctrl Pts',(91.3130966369063,2.48499327898026,48.5));
#82239=CARTESIAN_POINT('Ctrl Pts',(91.3130966369063,3.02824014425278,48.5));
#82240=CARTESIAN_POINT('Ctrl Pts',(91.1862889472395,3.2068213224411,48.5));
#82241=CARTESIAN_POINT('',(91.3130966369063,2.48499327898026,48.35));
#82242=CARTESIAN_POINT('',(91.3130966369063,2.48499327898026,48.5));
#82243=CARTESIAN_POINT('Ctrl Pts',(91.3130966369063,2.48499327898026,48.35));
#82244=CARTESIAN_POINT('Ctrl Pts',(91.3130966369063,3.02824014425278,48.35));
#82245=CARTESIAN_POINT('Ctrl Pts',(91.1862889472395,3.2068213224411,48.35));
#82246=CARTESIAN_POINT('Ctrl Pts',(91.1862889472395,1.76466578245163,48.5));
#82247=CARTESIAN_POINT('Ctrl Pts',(91.1862889472395,1.76466578245163,48.35));
#82248=CARTESIAN_POINT('Ctrl Pts',(91.3130966369063,1.9447478055954,48.5));
#82249=CARTESIAN_POINT('Ctrl Pts',(91.3130966369063,1.9447478055954,48.35));
#82250=CARTESIAN_POINT('Ctrl Pts',(91.3130966369063,2.48499327898026,48.5));
#82251=CARTESIAN_POINT('Ctrl Pts',(91.3130966369063,2.48499327898026,48.35));
#82252=CARTESIAN_POINT('',(91.1862889472395,1.76466578245163,48.5));
#82253=CARTESIAN_POINT('Ctrl Pts',(91.1862889472395,1.76466578245163,48.5));
#82254=CARTESIAN_POINT('Ctrl Pts',(91.3130966369063,1.9447478055954,48.5));
#82255=CARTESIAN_POINT('Ctrl Pts',(91.3130966369063,2.48499327898026,48.5));
#82256=CARTESIAN_POINT('',(91.1862889472395,1.76466578245163,48.35));
#82257=CARTESIAN_POINT('',(91.1862889472395,1.76466578245163,48.5));
#82258=CARTESIAN_POINT('Ctrl Pts',(91.1862889472395,1.76466578245163,48.35));
#82259=CARTESIAN_POINT('Ctrl Pts',(91.3130966369063,1.9447478055954,48.35));
#82260=CARTESIAN_POINT('Ctrl Pts',(91.3130966369063,2.48499327898026,48.35));
#82261=CARTESIAN_POINT('Ctrl Pts',(90.8733967486769,1.58458405733109,48.5));
#82262=CARTESIAN_POINT('Ctrl Pts',(90.8733967486769,1.58458405733109,48.35));
#82263=CARTESIAN_POINT('Ctrl Pts',(91.0594812575728,1.58458405733109,48.5));
#82264=CARTESIAN_POINT('Ctrl Pts',(91.0594812575728,1.58458405733109,48.35));
#82265=CARTESIAN_POINT('Ctrl Pts',(91.1862889472395,1.76466578245163,48.5));
#82266=CARTESIAN_POINT('Ctrl Pts',(91.1862889472395,1.76466578245163,48.35));
#82267=CARTESIAN_POINT('',(90.8733967486769,1.58458405733109,48.5));
#82268=CARTESIAN_POINT('Ctrl Pts',(90.8733967486769,1.58458405733109,48.5));
#82269=CARTESIAN_POINT('Ctrl Pts',(91.0594812575728,1.58458405733109,48.5));
#82270=CARTESIAN_POINT('Ctrl Pts',(91.1862889472395,1.76466578245163,48.5));
#82271=CARTESIAN_POINT('',(90.8733967486769,1.58458405733109,48.35));
#82272=CARTESIAN_POINT('',(90.8733967486769,1.58458405733109,48.5));
#82273=CARTESIAN_POINT('Ctrl Pts',(90.8733967486769,1.58458405733109,48.35));
#82274=CARTESIAN_POINT('Ctrl Pts',(91.0594812575728,1.58458405733109,48.35));
#82275=CARTESIAN_POINT('Ctrl Pts',(91.1862889472395,1.76466578245163,48.35));
#82276=CARTESIAN_POINT('Ctrl Pts',(90.5605045501143,1.76391565799713,48.5));
#82277=CARTESIAN_POINT('Ctrl Pts',(90.5605045501143,1.76391565799713,48.35));
#82278=CARTESIAN_POINT('Ctrl Pts',(90.687312239781,1.58458405733109,48.5));
#82279=CARTESIAN_POINT('Ctrl Pts',(90.687312239781,1.58458405733109,48.35));
#82280=CARTESIAN_POINT('Ctrl Pts',(90.8733967486769,1.58458405733109,48.5));
#82281=CARTESIAN_POINT('Ctrl Pts',(90.8733967486769,1.58458405733109,48.35));
#82282=CARTESIAN_POINT('',(90.5605045501143,1.76391565799713,48.5));
#82283=CARTESIAN_POINT('Ctrl Pts',(90.5605045501143,1.76391565799713,48.5));
#82284=CARTESIAN_POINT('Ctrl Pts',(90.687312239781,1.58458405733109,48.5));
#82285=CARTESIAN_POINT('Ctrl Pts',(90.8733967486769,1.58458405733109,48.5));
#82286=CARTESIAN_POINT('',(90.5605045501143,1.76391565799713,48.35));
#82287=CARTESIAN_POINT('',(90.5605045501143,1.76391565799713,48.5));
#82288=CARTESIAN_POINT('Ctrl Pts',(90.5605045501143,1.76391565799713,48.35));
#82289=CARTESIAN_POINT('Ctrl Pts',(90.687312239781,1.58458405733109,48.35));
#82290=CARTESIAN_POINT('Ctrl Pts',(90.8733967486769,1.58458405733109,48.35));
#82291=CARTESIAN_POINT('Ctrl Pts',(90.4336968604475,2.48499327898026,48.5));
#82292=CARTESIAN_POINT('Ctrl Pts',(90.4336968604475,2.48499327898026,48.35));
#82293=CARTESIAN_POINT('Ctrl Pts',(90.4336968604475,1.94324696063995,48.5));
#82294=CARTESIAN_POINT('Ctrl Pts',(90.4336968604475,1.94324696063995,48.35));
#82295=CARTESIAN_POINT('Ctrl Pts',(90.5605045501143,1.76391565799713,48.5));
#82296=CARTESIAN_POINT('Ctrl Pts',(90.5605045501143,1.76391565799713,48.35));
#82297=CARTESIAN_POINT('',(90.4336968604475,2.48499327898026,48.5));
#82298=CARTESIAN_POINT('Ctrl Pts',(90.4336968604475,2.48499327898026,48.5));
#82299=CARTESIAN_POINT('Ctrl Pts',(90.4336968604475,1.94324696063995,48.5));
#82300=CARTESIAN_POINT('Ctrl Pts',(90.5605045501143,1.76391565799713,48.5));
#82301=CARTESIAN_POINT('',(90.4336968604475,2.48499327898026,48.35));
#82302=CARTESIAN_POINT('',(90.4336968604475,2.48499327898026,48.5));
#82303=CARTESIAN_POINT('Ctrl Pts',(90.4336968604475,2.48499327898026,48.35));
#82304=CARTESIAN_POINT('Ctrl Pts',(90.4336968604475,1.94324696063995,48.35));
#82305=CARTESIAN_POINT('Ctrl Pts',(90.5605045501143,1.76391565799713,48.35));
#82306=CARTESIAN_POINT('Ctrl Pts',(90.5732605401427,3.22783091664314,48.5));
#82307=CARTESIAN_POINT('Ctrl Pts',(90.5732605401427,3.22783091664314,48.35));
#82308=CARTESIAN_POINT('Ctrl Pts',(90.4336968604475,3.02673944830894,48.5));
#82309=CARTESIAN_POINT('Ctrl Pts',(90.4336968604475,3.02673944830894,48.35));
#82310=CARTESIAN_POINT('Ctrl Pts',(90.4336968604475,2.48499327898026,48.5));
#82311=CARTESIAN_POINT('Ctrl Pts',(90.4336968604475,2.48499327898026,48.35));
#82312=CARTESIAN_POINT('Ctrl Pts',(90.5732605401427,3.22783091664314,48.5));
#82313=CARTESIAN_POINT('Ctrl Pts',(90.4336968604475,3.02673944830894,48.5));
#82314=CARTESIAN_POINT('Ctrl Pts',(90.4336968604475,2.48499327898026,48.5));
#82315=CARTESIAN_POINT('Ctrl Pts',(90.5732605401427,3.22783091664314,48.35));
#82316=CARTESIAN_POINT('Ctrl Pts',(90.4336968604475,3.02673944830894,48.35));
#82317=CARTESIAN_POINT('Ctrl Pts',(90.4336968604475,2.48499327898026,48.35));
#82318=CARTESIAN_POINT('Ctrl Pts',(90.8733967486769,1.36248314380646,48.5));
#82319=CARTESIAN_POINT('Ctrl Pts',(90.8733967486769,1.36248314380646,48.35));
#82320=CARTESIAN_POINT('Ctrl Pts',(90.5552521888167,1.36248314380646,48.5));
#82321=CARTESIAN_POINT('Ctrl Pts',(90.5552521888167,1.36248314380646,48.35));
#82322=CARTESIAN_POINT('Ctrl Pts',(90.3736696187407,1.59058684110642,48.5));
#82323=CARTESIAN_POINT('Ctrl Pts',(90.3736696187407,1.59058684110642,48.35));
#82324=CARTESIAN_POINT('',(90.8733967486769,1.36248314380646,48.5));
#82325=CARTESIAN_POINT('',(90.3736696187407,1.59058684110642,48.5));
#82326=CARTESIAN_POINT('Ctrl Pts',(90.8733967486769,1.36248314380646,48.5));
#82327=CARTESIAN_POINT('Ctrl Pts',(90.5552521888167,1.36248314380646,48.5));
#82328=CARTESIAN_POINT('Ctrl Pts',(90.3736696187407,1.59058684110642,48.5));
#82329=CARTESIAN_POINT('',(90.8733967486769,1.36248314380646,48.35));
#82330=CARTESIAN_POINT('',(90.8733967486769,1.36248314380646,48.5));
#82331=CARTESIAN_POINT('',(90.3736696187407,1.59058684110642,48.35));
#82332=CARTESIAN_POINT('Ctrl Pts',(90.8733967486769,1.36248314380646,48.35));
#82333=CARTESIAN_POINT('Ctrl Pts',(90.5552521888167,1.36248314380646,48.35));
#82334=CARTESIAN_POINT('Ctrl Pts',(90.3736696187407,1.59058684110642,48.35));
#82335=CARTESIAN_POINT('',(90.3736696187407,1.59058684110642,48.5));
#82336=CARTESIAN_POINT('Ctrl Pts',(91.2733284179121,1.49229192733765,48.5));
#82337=CARTESIAN_POINT('Ctrl Pts',(91.2733284179121,1.49229192733765,48.35));
#82338=CARTESIAN_POINT('Ctrl Pts',(91.1150065604597,1.36248314380646,48.5));
#82339=CARTESIAN_POINT('Ctrl Pts',(91.1150065604597,1.36248314380646,48.35));
#82340=CARTESIAN_POINT('Ctrl Pts',(90.8733967486769,1.36248314380646,48.5));
#82341=CARTESIAN_POINT('Ctrl Pts',(90.8733967486769,1.36248314380646,48.35));
#82342=CARTESIAN_POINT('',(91.2733284179121,1.49229192733765,48.5));
#82343=CARTESIAN_POINT('Ctrl Pts',(91.2733284179121,1.49229192733765,48.5));
#82344=CARTESIAN_POINT('Ctrl Pts',(91.1150065604597,1.36248314380646,48.5));
#82345=CARTESIAN_POINT('Ctrl Pts',(90.8733967486769,1.36248314380646,48.5));
#82346=CARTESIAN_POINT('',(91.2733284179121,1.49229192733765,48.35));
#82347=CARTESIAN_POINT('',(91.2733284179121,1.49229192733765,48.5));
#82348=CARTESIAN_POINT('Ctrl Pts',(91.2733284179121,1.49229192733765,48.35));
#82349=CARTESIAN_POINT('Ctrl Pts',(91.1150065604597,1.36248314380646,48.35));
#82350=CARTESIAN_POINT('Ctrl Pts',(90.8733967486769,1.36248314380646,48.35));
#82351=CARTESIAN_POINT('Ctrl Pts',(91.5111867133528,1.85995900630951,48.5));
#82352=CARTESIAN_POINT('Ctrl Pts',(91.5111867133528,1.85995900630951,48.35));
#82353=CARTESIAN_POINT('Ctrl Pts',(91.4316502753645,1.62210100889206,48.5));
#82354=CARTESIAN_POINT('Ctrl Pts',(91.4316502753645,1.62210100889206,48.35));
#82355=CARTESIAN_POINT('Ctrl Pts',(91.2733284179121,1.49229192733765,48.5));
#82356=CARTESIAN_POINT('Ctrl Pts',(91.2733284179121,1.49229192733765,48.35));
#82357=CARTESIAN_POINT('',(91.5111867133528,1.85995900630951,48.5));
#82358=CARTESIAN_POINT('Ctrl Pts',(91.5111867133528,1.85995900630951,48.5));
#82359=CARTESIAN_POINT('Ctrl Pts',(91.4316502753645,1.62210100889206,48.5));
#82360=CARTESIAN_POINT('Ctrl Pts',(91.2733284179121,1.49229192733765,48.5));
#82361=CARTESIAN_POINT('',(91.5111867133528,1.85995900630951,48.35));
#82362=CARTESIAN_POINT('',(91.5111867133528,1.85995900630951,48.5));
#82363=CARTESIAN_POINT('Ctrl Pts',(91.5111867133528,1.85995900630951,48.35));
#82364=CARTESIAN_POINT('Ctrl Pts',(91.4316502753645,1.62210100889206,48.35));
#82365=CARTESIAN_POINT('Ctrl Pts',(91.2733284179121,1.49229192733765,48.35));
#82366=CARTESIAN_POINT('Ctrl Pts',(91.5907225552946,2.48499327898026,48.5));
#82367=CARTESIAN_POINT('Ctrl Pts',(91.5907225552946,2.48499327898026,48.35));
#82368=CARTESIAN_POINT('Ctrl Pts',(91.5907225552946,2.09781730175018,48.5));
#82369=CARTESIAN_POINT('Ctrl Pts',(91.5907225552946,2.09781730175018,48.35));
#82370=CARTESIAN_POINT('Ctrl Pts',(91.5111867133528,1.85995900630951,48.5));
#82371=CARTESIAN_POINT('Ctrl Pts',(91.5111867133528,1.85995900630951,48.35));
#82372=CARTESIAN_POINT('',(91.5907225552946,2.48499327898026,48.5));
#82373=CARTESIAN_POINT('Ctrl Pts',(91.5907225552946,2.48499327898026,48.5));
#82374=CARTESIAN_POINT('Ctrl Pts',(91.5907225552946,2.09781730175018,48.5));
#82375=CARTESIAN_POINT('Ctrl Pts',(91.5111867133528,1.85995900630951,48.5));
#82376=CARTESIAN_POINT('',(91.5907225552946,2.48499327898026,48.35));
#82377=CARTESIAN_POINT('',(91.5907225552946,2.48499327898026,48.5));
#82378=CARTESIAN_POINT('Ctrl Pts',(91.5907225552946,2.48499327898026,48.35));
#82379=CARTESIAN_POINT('Ctrl Pts',(91.5907225552946,2.09781730175018,48.35));
#82380=CARTESIAN_POINT('Ctrl Pts',(91.5111867133528,1.85995900630951,48.35));
#82381=CARTESIAN_POINT('Ctrl Pts',(91.541200036183,3.00497958064079,48.5));
#82382=CARTESIAN_POINT('Ctrl Pts',(91.541200036183,3.00497958064079,48.35));
#82383=CARTESIAN_POINT('Ctrl Pts',(91.5907225552946,2.81214186549187,48.5));
#82384=CARTESIAN_POINT('Ctrl Pts',(91.5907225552946,2.81214186549187,48.35));
#82385=CARTESIAN_POINT('Ctrl Pts',(91.5907225552946,2.48499327898026,48.5));
#82386=CARTESIAN_POINT('Ctrl Pts',(91.5907225552946,2.48499327898026,48.35));
#82387=CARTESIAN_POINT('',(91.541200036183,3.00497958064079,48.5));
#82388=CARTESIAN_POINT('Ctrl Pts',(91.541200036183,3.00497958064079,48.5));
#82389=CARTESIAN_POINT('Ctrl Pts',(91.5907225552946,2.81214186549187,48.5));
#82390=CARTESIAN_POINT('Ctrl Pts',(91.5907225552946,2.48499327898026,48.5));
#82391=CARTESIAN_POINT('',(91.541200036183,3.00497958064079,48.35));
#82392=CARTESIAN_POINT('',(91.541200036183,3.00497958064079,48.5));
#82393=CARTESIAN_POINT('Ctrl Pts',(91.541200036183,3.00497958064079,48.35));
#82394=CARTESIAN_POINT('Ctrl Pts',(91.5907225552946,2.81214186549187,48.35));
#82395=CARTESIAN_POINT('Ctrl Pts',(91.5907225552946,2.48499327898026,48.35));
#82396=CARTESIAN_POINT('Ctrl Pts',(91.4046380463988,3.33212831616402,48.5));
#82397=CARTESIAN_POINT('Ctrl Pts',(91.4046380463988,3.33212831616402,48.35));
#82398=CARTESIAN_POINT('Ctrl Pts',(91.4916775170714,3.19781729578972,48.5));
#82399=CARTESIAN_POINT('Ctrl Pts',(91.4916775170714,3.19781729578972,48.35));
#82400=CARTESIAN_POINT('Ctrl Pts',(91.541200036183,3.00497958064079,48.5));
#82401=CARTESIAN_POINT('Ctrl Pts',(91.541200036183,3.00497958064079,48.35));
#82402=CARTESIAN_POINT('',(91.4046380463988,3.33212831616402,48.5));
#82403=CARTESIAN_POINT('Ctrl Pts',(91.4046380463988,3.33212831616402,48.5));
#82404=CARTESIAN_POINT('Ctrl Pts',(91.4916775170714,3.19781729578972,48.5));
#82405=CARTESIAN_POINT('Ctrl Pts',(91.541200036183,3.00497958064079,48.5));
#82406=CARTESIAN_POINT('',(91.4046380463988,3.33212831616402,48.35));
#82407=CARTESIAN_POINT('',(91.4046380463988,3.33212831616402,48.5));
#82408=CARTESIAN_POINT('Ctrl Pts',(91.4046380463988,3.33212831616402,48.35));
#82409=CARTESIAN_POINT('Ctrl Pts',(91.4916775170714,3.19781729578972,48.35));
#82410=CARTESIAN_POINT('Ctrl Pts',(91.541200036183,3.00497958064079,48.35));
#82411=CARTESIAN_POINT('Ctrl Pts',(91.1840382758528,3.5377217233181,48.5));
#82412=CARTESIAN_POINT('Ctrl Pts',(91.1840382758528,3.5377217233181,48.35));
#82413=CARTESIAN_POINT('Ctrl Pts',(91.3175985757262,3.46643933653831,48.5));
#82414=CARTESIAN_POINT('Ctrl Pts',(91.3175985757262,3.46643933653831,48.35));
#82415=CARTESIAN_POINT('Ctrl Pts',(91.4046380463988,3.33212831616402,48.5));
#82416=CARTESIAN_POINT('Ctrl Pts',(91.4046380463988,3.33212831616402,48.35));
#82417=CARTESIAN_POINT('',(91.1840382758528,3.5377217233181,48.5));
#82418=CARTESIAN_POINT('Ctrl Pts',(91.1840382758528,3.5377217233181,48.5));
#82419=CARTESIAN_POINT('Ctrl Pts',(91.3175985757262,3.46643933653831,48.5));
#82420=CARTESIAN_POINT('Ctrl Pts',(91.4046380463988,3.33212831616402,48.5));
#82421=CARTESIAN_POINT('',(91.1840382758528,3.5377217233181,48.35));
#82422=CARTESIAN_POINT('',(91.1840382758528,3.5377217233181,48.5));
#82423=CARTESIAN_POINT('Ctrl Pts',(91.1840382758528,3.5377217233181,48.35));
#82424=CARTESIAN_POINT('Ctrl Pts',(91.3175985757262,3.46643933653831,48.35));
#82425=CARTESIAN_POINT('Ctrl Pts',(91.4046380463988,3.33212831616402,48.35));
#82426=CARTESIAN_POINT('Ctrl Pts',(90.8733967486769,3.60900411009789,48.5));
#82427=CARTESIAN_POINT('Ctrl Pts',(90.8733967486769,3.60900411009789,48.35));
#82428=CARTESIAN_POINT('Ctrl Pts',(91.050477379933,3.60900411009789,48.5));
#82429=CARTESIAN_POINT('Ctrl Pts',(91.050477379933,3.60900411009789,48.35));
#82430=CARTESIAN_POINT('Ctrl Pts',(91.1840382758528,3.5377217233181,48.5));
#82431=CARTESIAN_POINT('Ctrl Pts',(91.1840382758528,3.5377217233181,48.35));
#82432=CARTESIAN_POINT('',(90.8733967486769,3.60900411009789,48.5));
#82433=CARTESIAN_POINT('Ctrl Pts',(90.8733967486769,3.60900411009789,48.5));
#82434=CARTESIAN_POINT('Ctrl Pts',(91.050477379933,3.60900411009789,48.5));
#82435=CARTESIAN_POINT('Ctrl Pts',(91.1840382758528,3.5377217233181,48.5));
#82436=CARTESIAN_POINT('',(90.8733967486769,3.60900411009789,48.35));
#82437=CARTESIAN_POINT('',(90.8733967486769,3.60900411009789,48.5));
#82438=CARTESIAN_POINT('Ctrl Pts',(90.8733967486769,3.60900411009789,48.35));
#82439=CARTESIAN_POINT('Ctrl Pts',(91.050477379933,3.60900411009789,48.35));
#82440=CARTESIAN_POINT('Ctrl Pts',(91.1840382758528,3.5377217233181,48.35));
#82441=CARTESIAN_POINT('Ctrl Pts',(90.4749659243971,3.47994545102119,48.5));
#82442=CARTESIAN_POINT('Ctrl Pts',(90.4749659243971,3.47994545102119,48.35));
#82443=CARTESIAN_POINT('Ctrl Pts',(90.6332877818495,3.60900411009789,48.5));
#82444=CARTESIAN_POINT('Ctrl Pts',(90.6332877818495,3.60900411009789,48.35));
#82445=CARTESIAN_POINT('Ctrl Pts',(90.8733967486769,3.60900411009789,48.5));
#82446=CARTESIAN_POINT('Ctrl Pts',(90.8733967486769,3.60900411009789,48.35));
#82447=CARTESIAN_POINT('',(90.4749659243971,3.47994545102119,48.5));
#82448=CARTESIAN_POINT('Ctrl Pts',(90.4749659243971,3.47994545102119,48.5));
#82449=CARTESIAN_POINT('Ctrl Pts',(90.6332877818495,3.60900411009789,48.5));
#82450=CARTESIAN_POINT('Ctrl Pts',(90.8733967486769,3.60900411009789,48.5));
#82451=CARTESIAN_POINT('',(90.4749659243971,3.47994545102119,48.35));
#82452=CARTESIAN_POINT('',(90.4749659243971,3.47994545102119,48.5));
#82453=CARTESIAN_POINT('Ctrl Pts',(90.4749659243971,3.47994545102119,48.35));
#82454=CARTESIAN_POINT('Ctrl Pts',(90.6332877818495,3.60900411009789,48.35));
#82455=CARTESIAN_POINT('Ctrl Pts',(90.8733967486769,3.60900411009789,48.35));
#82456=CARTESIAN_POINT('Ctrl Pts',(90.2363572064787,3.11302864551544,48.5));
#82457=CARTESIAN_POINT('Ctrl Pts',(90.2363572064787,3.11302864551544,48.35));
#82458=CARTESIAN_POINT('Ctrl Pts',(90.3166437689215,3.3508867919445,48.5));
#82459=CARTESIAN_POINT('Ctrl Pts',(90.3166437689215,3.3508867919445,48.35));
#82460=CARTESIAN_POINT('Ctrl Pts',(90.4749659243971,3.47994545102119,48.5));
#82461=CARTESIAN_POINT('Ctrl Pts',(90.4749659243971,3.47994545102119,48.35));
#82462=CARTESIAN_POINT('',(90.2363572064787,3.11302864551544,48.5));
#82463=CARTESIAN_POINT('Ctrl Pts',(90.2363572064787,3.11302864551544,48.5));
#82464=CARTESIAN_POINT('Ctrl Pts',(90.3166437689215,3.3508867919445,48.5));
#82465=CARTESIAN_POINT('Ctrl Pts',(90.4749659243971,3.47994545102119,48.5));
#82466=CARTESIAN_POINT('',(90.2363572064787,3.11302864551544,48.35));
#82467=CARTESIAN_POINT('',(90.2363572064787,3.11302864551544,48.5));
#82468=CARTESIAN_POINT('Ctrl Pts',(90.2363572064787,3.11302864551544,48.35));
#82469=CARTESIAN_POINT('Ctrl Pts',(90.3166437689215,3.3508867919445,48.35));
#82470=CARTESIAN_POINT('Ctrl Pts',(90.4749659243971,3.47994545102119,48.35));
#82471=CARTESIAN_POINT('Ctrl Pts',(90.1560709420592,2.48499327898026,48.5));
#82472=CARTESIAN_POINT('Ctrl Pts',(90.1560709420592,2.48499327898026,48.35));
#82473=CARTESIAN_POINT('Ctrl Pts',(90.1560709420592,2.87517049908638,48.5));
#82474=CARTESIAN_POINT('Ctrl Pts',(90.1560709420592,2.87517049908638,48.35));
#82475=CARTESIAN_POINT('Ctrl Pts',(90.2363572064787,3.11302864551544,48.5));
#82476=CARTESIAN_POINT('Ctrl Pts',(90.2363572064787,3.11302864551544,48.35));
#82477=CARTESIAN_POINT('',(90.1560709420592,2.48499327898026,48.5));
#82478=CARTESIAN_POINT('Ctrl Pts',(90.1560709420592,2.48499327898026,48.5));
#82479=CARTESIAN_POINT('Ctrl Pts',(90.1560709420592,2.87517049908638,48.5));
#82480=CARTESIAN_POINT('Ctrl Pts',(90.2363572064787,3.11302864551544,48.5));
#82481=CARTESIAN_POINT('',(90.1560709420592,2.48499327898026,48.35));
#82482=CARTESIAN_POINT('',(90.1560709420592,2.48499327898026,48.5));
#82483=CARTESIAN_POINT('Ctrl Pts',(90.1560709420592,2.48499327898026,48.35));
#82484=CARTESIAN_POINT('Ctrl Pts',(90.1560709420592,2.87517049908638,48.35));
#82485=CARTESIAN_POINT('Ctrl Pts',(90.2363572064787,3.11302864551544,48.35));
#82486=CARTESIAN_POINT('Ctrl Pts',(90.3736696187407,1.59058684110642,48.5));
#82487=CARTESIAN_POINT('Ctrl Pts',(90.3736696187407,1.59058684110642,48.35));
#82488=CARTESIAN_POINT('Ctrl Pts',(90.1560709420592,1.86521166563034,48.5));
#82489=CARTESIAN_POINT('Ctrl Pts',(90.1560709420592,1.86521166563034,48.35));
#82490=CARTESIAN_POINT('Ctrl Pts',(90.1560709420592,2.48499327898026,48.5));
#82491=CARTESIAN_POINT('Ctrl Pts',(90.1560709420592,2.48499327898026,48.35));
#82492=CARTESIAN_POINT('Ctrl Pts',(90.3736696187407,1.59058684110642,48.5));
#82493=CARTESIAN_POINT('Ctrl Pts',(90.1560709420592,1.86521166563034,48.5));
#82494=CARTESIAN_POINT('Ctrl Pts',(90.1560709420592,2.48499327898026,48.5));
#82495=CARTESIAN_POINT('Ctrl Pts',(90.3736696187407,1.59058684110642,48.35));
#82496=CARTESIAN_POINT('Ctrl Pts',(90.1560709420592,1.86521166563034,48.35));
#82497=CARTESIAN_POINT('Ctrl Pts',(90.1560709420592,2.48499327898026,48.35));
#82498=CARTESIAN_POINT('Origin',(89.9999996814877,2.48574362695217,48.35));
#82499=CARTESIAN_POINT('Ctrl Pts',(88.9015006069094,1.80593454837799,48.5));
#82500=CARTESIAN_POINT('Ctrl Pts',(88.9015006069094,1.80593454837799,48.35));
#82501=CARTESIAN_POINT('Ctrl Pts',(88.8324691895396,1.73315161466599,48.5));
#82502=CARTESIAN_POINT('Ctrl Pts',(88.8324691895396,1.73315161466599,48.35));
#82503=CARTESIAN_POINT('Ctrl Pts',(88.7874487582594,1.65961825847626,48.5));
#82504=CARTESIAN_POINT('Ctrl Pts',(88.7874487582594,1.65961825847626,48.35));
#82505=CARTESIAN_POINT('',(88.9015006069094,1.80593454837799,48.5));
#82506=CARTESIAN_POINT('',(88.7874487582594,1.65961825847626,48.5));
#82507=CARTESIAN_POINT('Ctrl Pts',(88.9015006069094,1.80593454837799,48.5));
#82508=CARTESIAN_POINT('Ctrl Pts',(88.8324691895396,1.73315161466599,48.5));
#82509=CARTESIAN_POINT('Ctrl Pts',(88.7874487582594,1.65961825847626,48.5));
#82510=CARTESIAN_POINT('',(88.9015006069094,1.80593454837799,48.35));
#82511=CARTESIAN_POINT('',(88.9015006069094,1.80593454837799,48.5));
#82512=CARTESIAN_POINT('',(88.7874487582594,1.65961825847626,48.35));
#82513=CARTESIAN_POINT('Ctrl Pts',(88.9015006069094,1.80593454837799,48.35));
#82514=CARTESIAN_POINT('Ctrl Pts',(88.8324691895396,1.73315161466599,48.35));
#82515=CARTESIAN_POINT('Ctrl Pts',(88.7874487582594,1.65961825847626,48.35));
#82516=CARTESIAN_POINT('',(88.7874487582594,1.65961825847626,48.5));
#82517=CARTESIAN_POINT('Ctrl Pts',(89.2136425320059,2.08281049132347,48.5));
#82518=CARTESIAN_POINT('Ctrl Pts',(89.2136425320059,2.08281049132347,48.35));
#82519=CARTESIAN_POINT('Ctrl Pts',(88.9705318752676,1.87871778011322,48.5));
#82520=CARTESIAN_POINT('Ctrl Pts',(88.9705318752676,1.87871778011322,48.35));
#82521=CARTESIAN_POINT('Ctrl Pts',(88.9015006069094,1.80593454837799,48.5));
#82522=CARTESIAN_POINT('Ctrl Pts',(88.9015006069094,1.80593454837799,48.35));
#82523=CARTESIAN_POINT('',(89.2136425320059,2.08281049132347,48.5));
#82524=CARTESIAN_POINT('Ctrl Pts',(89.2136425320059,2.08281049132347,48.5));
#82525=CARTESIAN_POINT('Ctrl Pts',(88.9705318752676,1.87871778011322,48.5));
#82526=CARTESIAN_POINT('Ctrl Pts',(88.9015006069094,1.80593454837799,48.5));
#82527=CARTESIAN_POINT('',(89.2136425320059,2.08281049132347,48.35));
#82528=CARTESIAN_POINT('',(89.2136425320059,2.08281049132347,48.5));
#82529=CARTESIAN_POINT('Ctrl Pts',(89.2136425320059,2.08281049132347,48.35));
#82530=CARTESIAN_POINT('Ctrl Pts',(88.9705318752676,1.87871778011322,48.35));
#82531=CARTESIAN_POINT('Ctrl Pts',(88.9015006069094,1.80593454837799,48.35));
#82532=CARTESIAN_POINT('Ctrl Pts',(89.6300817076117,2.46998646855354,48.5));
#82533=CARTESIAN_POINT('Ctrl Pts',(89.6300817076117,2.46998646855354,48.35));
#82534=CARTESIAN_POINT('Ctrl Pts',(89.5047748629004,2.32892239093781,48.5));
#82535=CARTESIAN_POINT('Ctrl Pts',(89.5047748629004,2.32892239093781,48.35));
#82536=CARTESIAN_POINT('Ctrl Pts',(89.2136425320059,2.08281049132347,48.5));
#82537=CARTESIAN_POINT('Ctrl Pts',(89.2136425320059,2.08281049132347,48.35));
#82538=CARTESIAN_POINT('',(89.6300817076117,2.46998646855354,48.5));
#82539=CARTESIAN_POINT('Ctrl Pts',(89.6300817076117,2.46998646855354,48.5));
#82540=CARTESIAN_POINT('Ctrl Pts',(89.5047748629004,2.32892239093781,48.5));
#82541=CARTESIAN_POINT('Ctrl Pts',(89.2136425320059,2.08281049132347,48.5));
#82542=CARTESIAN_POINT('',(89.6300817076117,2.46998646855354,48.35));
#82543=CARTESIAN_POINT('',(89.6300817076117,2.46998646855354,48.5));
#82544=CARTESIAN_POINT('Ctrl Pts',(89.6300817076117,2.46998646855354,48.35));
#82545=CARTESIAN_POINT('Ctrl Pts',(89.5047748629004,2.32892239093781,48.35));
#82546=CARTESIAN_POINT('Ctrl Pts',(89.2136425320059,2.08281049132347,48.35));
#82547=CARTESIAN_POINT('Ctrl Pts',(89.8094133082777,2.73860850930214,48.5));
#82548=CARTESIAN_POINT('Ctrl Pts',(89.8094133082777,2.73860850930214,48.35));
#82549=CARTESIAN_POINT('Ctrl Pts',(89.7553888503462,2.61105054616928,48.5));
#82550=CARTESIAN_POINT('Ctrl Pts',(89.7553888503462,2.61105054616928,48.35));
#82551=CARTESIAN_POINT('Ctrl Pts',(89.6300817076117,2.46998646855354,48.5));
#82552=CARTESIAN_POINT('Ctrl Pts',(89.6300817076117,2.46998646855354,48.35));
#82553=CARTESIAN_POINT('',(89.8094133082777,2.73860850930214,48.5));
#82554=CARTESIAN_POINT('Ctrl Pts',(89.8094133082777,2.73860850930214,48.5));
#82555=CARTESIAN_POINT('Ctrl Pts',(89.7553888503462,2.61105054616928,48.5));
#82556=CARTESIAN_POINT('Ctrl Pts',(89.6300817076117,2.46998646855354,48.5));
#82557=CARTESIAN_POINT('',(89.8094133082777,2.73860850930214,48.35));
#82558=CARTESIAN_POINT('',(89.8094133082777,2.73860850930214,48.5));
#82559=CARTESIAN_POINT('Ctrl Pts',(89.8094133082777,2.73860850930214,48.35));
#82560=CARTESIAN_POINT('Ctrl Pts',(89.7553888503462,2.61105054616928,48.35));
#82561=CARTESIAN_POINT('Ctrl Pts',(89.6300817076117,2.46998646855354,48.35));
#82562=CARTESIAN_POINT('Ctrl Pts',(89.8634377662092,2.99822652339935,48.5));
#82563=CARTESIAN_POINT('Ctrl Pts',(89.8634377662092,2.99822652339935,48.35));
#82564=CARTESIAN_POINT('Ctrl Pts',(89.8634377662092,2.866166472435,48.5));
#82565=CARTESIAN_POINT('Ctrl Pts',(89.8634377662092,2.866166472435,48.35));
#82566=CARTESIAN_POINT('Ctrl Pts',(89.8094133082777,2.73860850930214,48.5));
#82567=CARTESIAN_POINT('Ctrl Pts',(89.8094133082777,2.73860850930214,48.35));
#82568=CARTESIAN_POINT('',(89.8634377662092,2.99822652339935,48.5));
#82569=CARTESIAN_POINT('Ctrl Pts',(89.8634377662092,2.99822652339935,48.5));
#82570=CARTESIAN_POINT('Ctrl Pts',(89.8634377662092,2.866166472435,48.5));
#82571=CARTESIAN_POINT('Ctrl Pts',(89.8094133082777,2.73860850930214,48.5));
#82572=CARTESIAN_POINT('',(89.8634377662092,2.99822652339935,48.35));
#82573=CARTESIAN_POINT('',(89.8634377662092,2.99822652339935,48.5));
#82574=CARTESIAN_POINT('Ctrl Pts',(89.8634377662092,2.99822652339935,48.35));
#82575=CARTESIAN_POINT('Ctrl Pts',(89.8634377662092,2.866166472435,48.35));
#82576=CARTESIAN_POINT('Ctrl Pts',(89.8094133082777,2.73860850930214,48.35));
#82577=CARTESIAN_POINT('Ctrl Pts',(89.6788541022688,3.43342432379723,48.5));
#82578=CARTESIAN_POINT('Ctrl Pts',(89.6788541022688,3.43342432379723,48.35));
#82579=CARTESIAN_POINT('Ctrl Pts',(89.8634377662092,3.25784453749657,48.5));
#82580=CARTESIAN_POINT('Ctrl Pts',(89.8634377662092,3.25784453749657,48.35));
#82581=CARTESIAN_POINT('Ctrl Pts',(89.8634377662092,2.99822652339935,48.5));
#82582=CARTESIAN_POINT('Ctrl Pts',(89.8634377662092,2.99822652339935,48.35));
#82583=CARTESIAN_POINT('',(89.6788541022688,3.43342432379723,48.5));
#82584=CARTESIAN_POINT('Ctrl Pts',(89.6788541022688,3.43342432379723,48.5));
#82585=CARTESIAN_POINT('Ctrl Pts',(89.8634377662092,3.25784453749657,48.5));
#82586=CARTESIAN_POINT('Ctrl Pts',(89.8634377662092,2.99822652339935,48.5));
#82587=CARTESIAN_POINT('',(89.6788541022688,3.43342432379723,48.35));
#82588=CARTESIAN_POINT('',(89.6788541022688,3.43342432379723,48.5));
#82589=CARTESIAN_POINT('Ctrl Pts',(89.6788541022688,3.43342432379723,48.35));
#82590=CARTESIAN_POINT('Ctrl Pts',(89.8634377662092,3.25784453749657,48.35));
#82591=CARTESIAN_POINT('Ctrl Pts',(89.8634377662092,2.99822652339935,48.35));
#82592=CARTESIAN_POINT('Ctrl Pts',(89.1776261273772,3.60900411009789,48.5));
#82593=CARTESIAN_POINT('Ctrl Pts',(89.1776261273772,3.60900411009789,48.35));
#82594=CARTESIAN_POINT('Ctrl Pts',(89.4942701403052,3.60900411009789,48.5));
#82595=CARTESIAN_POINT('Ctrl Pts',(89.4942701403052,3.60900411009789,48.35));
#82596=CARTESIAN_POINT('Ctrl Pts',(89.6788541022688,3.43342432379723,48.5));
#82597=CARTESIAN_POINT('Ctrl Pts',(89.6788541022688,3.43342432379723,48.35));
#82598=CARTESIAN_POINT('',(89.1776261273772,3.60900411009789,48.5));
#82599=CARTESIAN_POINT('Ctrl Pts',(89.1776261273772,3.60900411009789,48.5));
#82600=CARTESIAN_POINT('Ctrl Pts',(89.4942701403052,3.60900411009789,48.5));
#82601=CARTESIAN_POINT('Ctrl Pts',(89.6788541022688,3.43342432379723,48.5));
#82602=CARTESIAN_POINT('',(89.1776261273772,3.60900411009789,48.35));
#82603=CARTESIAN_POINT('',(89.1776261273772,3.60900411009789,48.5));
#82604=CARTESIAN_POINT('Ctrl Pts',(89.1776261273772,3.60900411009789,48.35));
#82605=CARTESIAN_POINT('Ctrl Pts',(89.4942701403052,3.60900411009789,48.35));
#82606=CARTESIAN_POINT('Ctrl Pts',(89.6788541022688,3.43342432379723,48.35));
#82607=CARTESIAN_POINT('Ctrl Pts',(88.6778989974409,3.446180164814,48.5));
#82608=CARTESIAN_POINT('Ctrl Pts',(88.6778989974409,3.446180164814,48.35));
#82609=CARTESIAN_POINT('Ctrl Pts',(88.8639835063368,3.60900411009789,48.5));
#82610=CARTESIAN_POINT('Ctrl Pts',(88.8639835063368,3.60900411009789,48.35));
#82611=CARTESIAN_POINT('Ctrl Pts',(89.1776261273772,3.60900411009789,48.5));
#82612=CARTESIAN_POINT('Ctrl Pts',(89.1776261273772,3.60900411009789,48.35));
#82613=CARTESIAN_POINT('',(88.6778989974409,3.446180164814,48.5));
#82614=CARTESIAN_POINT('Ctrl Pts',(88.6778989974409,3.446180164814,48.5));
#82615=CARTESIAN_POINT('Ctrl Pts',(88.8639835063368,3.60900411009789,48.5));
#82616=CARTESIAN_POINT('Ctrl Pts',(89.1776261273772,3.60900411009789,48.5));
#82617=CARTESIAN_POINT('',(88.6778989974409,3.446180164814,48.35));
#82618=CARTESIAN_POINT('',(88.6778989974409,3.446180164814,48.5));
#82619=CARTESIAN_POINT('Ctrl Pts',(88.6778989974409,3.446180164814,48.35));
#82620=CARTESIAN_POINT('Ctrl Pts',(88.8639835063368,3.60900411009789,48.35));
#82621=CARTESIAN_POINT('Ctrl Pts',(89.1776261273772,3.60900411009789,48.35));
#82622=CARTESIAN_POINT('Ctrl Pts',(88.4633014146239,2.97271499037743,48.5));
#82623=CARTESIAN_POINT('Ctrl Pts',(88.4633014146239,2.97271499037743,48.35));
#82624=CARTESIAN_POINT('Ctrl Pts',(88.4918143395334,3.28335621953011,48.5));
#82625=CARTESIAN_POINT('Ctrl Pts',(88.4918143395334,3.28335621953011,48.35));
#82626=CARTESIAN_POINT('Ctrl Pts',(88.6778989974409,3.446180164814,48.5));
#82627=CARTESIAN_POINT('Ctrl Pts',(88.6778989974409,3.446180164814,48.35));
#82628=CARTESIAN_POINT('',(88.4633014146239,2.97271499037743,48.5));
#82629=CARTESIAN_POINT('Ctrl Pts',(88.4633014146239,2.97271499037743,48.5));
#82630=CARTESIAN_POINT('Ctrl Pts',(88.4918143395334,3.28335621953011,48.5));
#82631=CARTESIAN_POINT('Ctrl Pts',(88.6778989974409,3.446180164814,48.5));
#82632=CARTESIAN_POINT('',(88.4633014146239,2.97271499037743,48.35));
#82633=CARTESIAN_POINT('',(88.4633014146239,2.97271499037743,48.5));
#82634=CARTESIAN_POINT('Ctrl Pts',(88.4633014146239,2.97271499037743,48.35));
#82635=CARTESIAN_POINT('Ctrl Pts',(88.4918143395334,3.28335621953011,48.35));
#82636=CARTESIAN_POINT('Ctrl Pts',(88.6778989974409,3.446180164814,48.35));
#82637=CARTESIAN_POINT('Origin',(88.7409276310354,2.94420206546783,48.5));
#82638=CARTESIAN_POINT('',(88.7409276310354,2.94420206546783,48.5));
#82639=CARTESIAN_POINT('',(44.5766785275039,7.47998378901591,48.5));
#82640=CARTESIAN_POINT('',(88.7409276310354,2.94420206546783,48.35));
#82641=CARTESIAN_POINT('',(88.7409276310354,2.94420206546783,48.5));
#82642=CARTESIAN_POINT('',(88.7409276310354,2.94420206546783,48.35));
#82643=CARTESIAN_POINT('Ctrl Pts',(88.8594815675169,3.26834926009178,48.5));
#82644=CARTESIAN_POINT('Ctrl Pts',(88.8594815675169,3.26834926009178,48.35));
#82645=CARTESIAN_POINT('Ctrl Pts',(88.7424283269793,3.15129616856575,48.5));
#82646=CARTESIAN_POINT('Ctrl Pts',(88.7424283269793,3.15129616856575,48.35));
#82647=CARTESIAN_POINT('Ctrl Pts',(88.7409276310354,2.94420206546783,48.5));
#82648=CARTESIAN_POINT('Ctrl Pts',(88.7409276310354,2.94420206546783,48.35));
#82649=CARTESIAN_POINT('',(88.8594815675169,3.26834926009178,48.5));
#82650=CARTESIAN_POINT('Ctrl Pts',(88.8594815675169,3.26834926009178,48.5));
#82651=CARTESIAN_POINT('Ctrl Pts',(88.7424283269793,3.15129616856575,48.5));
#82652=CARTESIAN_POINT('Ctrl Pts',(88.7409276310354,2.94420206546783,48.5));
#82653=CARTESIAN_POINT('',(88.8594815675169,3.26834926009178,48.35));
#82654=CARTESIAN_POINT('',(88.8594815675169,3.26834926009178,48.5));
#82655=CARTESIAN_POINT('Ctrl Pts',(88.8594815675169,3.26834926009178,48.35));
#82656=CARTESIAN_POINT('Ctrl Pts',(88.7424283269793,3.15129616856575,48.35));
#82657=CARTESIAN_POINT('Ctrl Pts',(88.7409276310354,2.94420206546783,48.35));
#82658=CARTESIAN_POINT('Ctrl Pts',(89.1716233436018,3.38540250062943,48.5));
#82659=CARTESIAN_POINT('Ctrl Pts',(89.1716233436018,3.38540250062943,48.35));
#82660=CARTESIAN_POINT('Ctrl Pts',(88.976534659043,3.38540250062943,48.5));
#82661=CARTESIAN_POINT('Ctrl Pts',(88.976534659043,3.38540250062943,48.35));
#82662=CARTESIAN_POINT('Ctrl Pts',(88.8594815675169,3.26834926009178,48.5));
#82663=CARTESIAN_POINT('Ctrl Pts',(88.8594815675169,3.26834926009178,48.35));
#82664=CARTESIAN_POINT('',(89.1716233436018,3.38540250062943,48.5));
#82665=CARTESIAN_POINT('Ctrl Pts',(89.1716233436018,3.38540250062943,48.5));
#82666=CARTESIAN_POINT('Ctrl Pts',(88.976534659043,3.38540250062943,48.5));
#82667=CARTESIAN_POINT('Ctrl Pts',(88.8594815675169,3.26834926009178,48.5));
#82668=CARTESIAN_POINT('',(89.1716233436018,3.38540250062943,48.35));
#82669=CARTESIAN_POINT('',(89.1716233436018,3.38540250062943,48.5));
#82670=CARTESIAN_POINT('Ctrl Pts',(89.1716233436018,3.38540250062943,48.35));
#82671=CARTESIAN_POINT('Ctrl Pts',(88.976534659043,3.38540250062943,48.35));
#82672=CARTESIAN_POINT('Ctrl Pts',(88.8594815675169,3.26834926009178,48.35));
#82673=CARTESIAN_POINT('Ctrl Pts',(89.4710094276816,3.27510246634483,48.5));
#82674=CARTESIAN_POINT('Ctrl Pts',(89.4710094276816,3.27510246634483,48.35));
#82675=CARTESIAN_POINT('Ctrl Pts',(89.3562073055655,3.38540250062943,48.5));
#82676=CARTESIAN_POINT('Ctrl Pts',(89.3562073055655,3.38540250062943,48.35));
#82677=CARTESIAN_POINT('Ctrl Pts',(89.1716233436018,3.38540250062943,48.5));
#82678=CARTESIAN_POINT('Ctrl Pts',(89.1716233436018,3.38540250062943,48.35));
#82679=CARTESIAN_POINT('',(89.4710094276816,3.27510246634483,48.5));
#82680=CARTESIAN_POINT('Ctrl Pts',(89.4710094276816,3.27510246634483,48.5));
#82681=CARTESIAN_POINT('Ctrl Pts',(89.3562073055655,3.38540250062943,48.5));
#82682=CARTESIAN_POINT('Ctrl Pts',(89.1716233436018,3.38540250062943,48.5));
#82683=CARTESIAN_POINT('',(89.4710094276816,3.27510246634483,48.35));
#82684=CARTESIAN_POINT('',(89.4710094276816,3.27510246634483,48.5));
#82685=CARTESIAN_POINT('Ctrl Pts',(89.4710094276816,3.27510246634483,48.35));
#82686=CARTESIAN_POINT('Ctrl Pts',(89.3562073055655,3.38540250062943,48.35));
#82687=CARTESIAN_POINT('Ctrl Pts',(89.1716233436018,3.38540250062943,48.35));
#82688=CARTESIAN_POINT('Ctrl Pts',(89.5858118478209,3.00422930717468,48.5));
#82689=CARTESIAN_POINT('Ctrl Pts',(89.5858118478209,3.00422930717468,48.35));
#82690=CARTESIAN_POINT('Ctrl Pts',(89.5858118478209,3.16480228304863,48.5));
#82691=CARTESIAN_POINT('Ctrl Pts',(89.5858118478209,3.16480228304863,48.35));
#82692=CARTESIAN_POINT('Ctrl Pts',(89.4710094276816,3.27510246634483,48.5));
#82693=CARTESIAN_POINT('Ctrl Pts',(89.4710094276816,3.27510246634483,48.35));
#82694=CARTESIAN_POINT('',(89.5858118478209,3.00422930717468,48.5));
#82695=CARTESIAN_POINT('Ctrl Pts',(89.5858118478209,3.00422930717468,48.5));
#82696=CARTESIAN_POINT('Ctrl Pts',(89.5858118478209,3.16480228304863,48.5));
#82697=CARTESIAN_POINT('Ctrl Pts',(89.4710094276816,3.27510246634483,48.5));
#82698=CARTESIAN_POINT('',(89.5858118478209,3.00422930717468,48.35));
#82699=CARTESIAN_POINT('',(89.5858118478209,3.00422930717468,48.5));
#82700=CARTESIAN_POINT('Ctrl Pts',(89.5858118478209,3.00422930717468,48.35));
#82701=CARTESIAN_POINT('Ctrl Pts',(89.5858118478209,3.16480228304863,48.35));
#82702=CARTESIAN_POINT('Ctrl Pts',(89.4710094276816,3.27510246634483,48.35));
#82703=CARTESIAN_POINT('Ctrl Pts',(89.4597542826086,2.6793315410614,48.5));
#82704=CARTESIAN_POINT('Ctrl Pts',(89.4597542826086,2.6793315410614,48.35));
#82705=CARTESIAN_POINT('Ctrl Pts',(89.5858118478209,2.85115966200829,48.5));
#82706=CARTESIAN_POINT('Ctrl Pts',(89.5858118478209,2.85115966200829,48.35));
#82707=CARTESIAN_POINT('Ctrl Pts',(89.5858118478209,3.00422930717468,48.5));
#82708=CARTESIAN_POINT('Ctrl Pts',(89.5858118478209,3.00422930717468,48.35));
#82709=CARTESIAN_POINT('',(89.4597542826086,2.6793315410614,48.5));
#82710=CARTESIAN_POINT('Ctrl Pts',(89.4597542826086,2.6793315410614,48.5));
#82711=CARTESIAN_POINT('Ctrl Pts',(89.5858118478209,2.85115966200829,48.5));
#82712=CARTESIAN_POINT('Ctrl Pts',(89.5858118478209,3.00422930717468,48.5));
#82713=CARTESIAN_POINT('',(89.4597542826086,2.6793315410614,48.35));
#82714=CARTESIAN_POINT('',(89.4597542826086,2.6793315410614,48.5));
#82715=CARTESIAN_POINT('Ctrl Pts',(89.4597542826086,2.6793315410614,48.35));
#82716=CARTESIAN_POINT('Ctrl Pts',(89.5858118478209,2.85115966200829,48.35));
#82717=CARTESIAN_POINT('Ctrl Pts',(89.5858118478209,3.00422930717468,48.35));
#82718=CARTESIAN_POINT('Ctrl Pts',(88.9750341121107,2.21336984634399,48.5));
#82719=CARTESIAN_POINT('Ctrl Pts',(88.9750341121107,2.21336984634399,48.35));
#82720=CARTESIAN_POINT('Ctrl Pts',(89.3336970154196,2.50750356912613,48.5));
#82721=CARTESIAN_POINT('Ctrl Pts',(89.3336970154196,2.50750356912613,48.35));
#82722=CARTESIAN_POINT('Ctrl Pts',(89.4597542826086,2.6793315410614,48.5));
#82723=CARTESIAN_POINT('Ctrl Pts',(89.4597542826086,2.6793315410614,48.35));
#82724=CARTESIAN_POINT('',(88.9750341121107,2.21336984634399,48.5));
#82725=CARTESIAN_POINT('Ctrl Pts',(88.9750341121107,2.21336984634399,48.5));
#82726=CARTESIAN_POINT('Ctrl Pts',(89.3336970154196,2.50750356912613,48.5));
#82727=CARTESIAN_POINT('Ctrl Pts',(89.4597542826086,2.6793315410614,48.5));
#82728=CARTESIAN_POINT('',(88.9750341121107,2.21336984634399,48.35));
#82729=CARTESIAN_POINT('',(88.9750341121107,2.21336984634399,48.5));
#82730=CARTESIAN_POINT('Ctrl Pts',(88.9750341121107,2.21336984634399,48.35));
#82731=CARTESIAN_POINT('Ctrl Pts',(89.3336970154196,2.50750356912613,48.35));
#82732=CARTESIAN_POINT('Ctrl Pts',(89.4597542826086,2.6793315410614,48.35));
#82733=CARTESIAN_POINT('Ctrl Pts',(88.6216234210879,1.88021832704544,48.5));
#82734=CARTESIAN_POINT('Ctrl Pts',(88.6216234210879,1.88021832704544,48.35));
#82735=CARTESIAN_POINT('Ctrl Pts',(88.7439290229231,2.02428394556046,48.5));
#82736=CARTESIAN_POINT('Ctrl Pts',(88.7439290229231,2.02428394556046,48.35));
#82737=CARTESIAN_POINT('Ctrl Pts',(88.9750341121107,2.21336984634399,48.5));
#82738=CARTESIAN_POINT('Ctrl Pts',(88.9750341121107,2.21336984634399,48.35));
#82739=CARTESIAN_POINT('',(88.6216234210879,1.88021832704544,48.5));
#82740=CARTESIAN_POINT('Ctrl Pts',(88.6216234210879,1.88021832704544,48.5));
#82741=CARTESIAN_POINT('Ctrl Pts',(88.7439290229231,2.02428394556046,48.5));
#82742=CARTESIAN_POINT('Ctrl Pts',(88.9750341121107,2.21336984634399,48.5));
#82743=CARTESIAN_POINT('',(88.6216234210879,1.88021832704544,48.35));
#82744=CARTESIAN_POINT('',(88.6216234210879,1.88021832704544,48.5));
#82745=CARTESIAN_POINT('Ctrl Pts',(88.6216234210879,1.88021832704544,48.35));
#82746=CARTESIAN_POINT('Ctrl Pts',(88.7439290229231,2.02428394556046,48.35));
#82747=CARTESIAN_POINT('Ctrl Pts',(88.9750341121107,2.21336984634399,48.35));
#82748=CARTESIAN_POINT('Ctrl Pts',(88.4437925163656,1.58758544921875,48.5));
#82749=CARTESIAN_POINT('Ctrl Pts',(88.4437925163656,1.58758544921875,48.35));
#82750=CARTESIAN_POINT('Ctrl Pts',(88.4993178192526,1.73615300655365,48.5));
#82751=CARTESIAN_POINT('Ctrl Pts',(88.4993178192526,1.73615300655365,48.35));
#82752=CARTESIAN_POINT('Ctrl Pts',(88.6216234210879,1.88021832704544,48.5));
#82753=CARTESIAN_POINT('Ctrl Pts',(88.6216234210879,1.88021832704544,48.35));
#82754=CARTESIAN_POINT('',(88.4437925163656,1.58758544921875,48.5));
#82755=CARTESIAN_POINT('Ctrl Pts',(88.4437925163656,1.58758544921875,48.5));
#82756=CARTESIAN_POINT('Ctrl Pts',(88.4993178192526,1.73615300655365,48.5));
#82757=CARTESIAN_POINT('Ctrl Pts',(88.6216234210879,1.88021832704544,48.5));
#82758=CARTESIAN_POINT('',(88.4437925163656,1.58758544921875,48.35));
#82759=CARTESIAN_POINT('',(88.4437925163656,1.58758544921875,48.5));
#82760=CARTESIAN_POINT('Ctrl Pts',(88.4437925163656,1.58758544921875,48.35));
#82761=CARTESIAN_POINT('Ctrl Pts',(88.4993178192526,1.73615300655365,48.35));
#82762=CARTESIAN_POINT('Ctrl Pts',(88.6216234210879,1.88021832704544,48.35));
#82763=CARTESIAN_POINT('Ctrl Pts',(88.4122781995684,1.40000009536743,48.5));
#82764=CARTESIAN_POINT('Ctrl Pts',(88.4122781995684,1.40000009536743,48.35));
#82765=CARTESIAN_POINT('Ctrl Pts',(88.4092768076807,1.49754428863525,48.5));
#82766=CARTESIAN_POINT('Ctrl Pts',(88.4092768076807,1.49754428863525,48.35));
#82767=CARTESIAN_POINT('Ctrl Pts',(88.4437925163656,1.58758544921875,48.5));
#82768=CARTESIAN_POINT('Ctrl Pts',(88.4437925163656,1.58758544921875,48.35));
#82769=CARTESIAN_POINT('',(88.4122781995684,1.40000009536743,48.5));
#82770=CARTESIAN_POINT('Ctrl Pts',(88.4122781995684,1.40000009536743,48.5));
#82771=CARTESIAN_POINT('Ctrl Pts',(88.4092768076807,1.49754428863525,48.5));
#82772=CARTESIAN_POINT('Ctrl Pts',(88.4437925163656,1.58758544921875,48.5));
#82773=CARTESIAN_POINT('',(88.4122781995684,1.40000009536743,48.35));
#82774=CARTESIAN_POINT('',(88.4122781995684,1.40000009536743,48.5));
#82775=CARTESIAN_POINT('Ctrl Pts',(88.4122781995684,1.40000009536743,48.35));
#82776=CARTESIAN_POINT('Ctrl Pts',(88.4092768076807,1.49754428863525,48.35));
#82777=CARTESIAN_POINT('Ctrl Pts',(88.4437925163656,1.58758544921875,48.35));
#82778=CARTESIAN_POINT('Origin',(89.8664391580969,1.40000009536743,48.5));
#82779=CARTESIAN_POINT('',(89.8664391580969,1.40000009536743,48.5));
#82780=CARTESIAN_POINT('',(44.9332195790485,1.40000009536743,48.5));
#82781=CARTESIAN_POINT('',(89.8664391580969,1.40000009536743,48.35));
#82782=CARTESIAN_POINT('',(89.8664391580969,1.40000009536743,48.5));
#82783=CARTESIAN_POINT('',(89.8664391580969,1.40000009536743,48.35));
#82784=CARTESIAN_POINT('Origin',(89.8664391580969,1.65961825847626,48.5));
#82785=CARTESIAN_POINT('',(89.8664391580969,1.65961825847626,48.5));
#82786=CARTESIAN_POINT('',(89.8664391580969,4.82980912923813,48.5));
#82787=CARTESIAN_POINT('',(89.8664391580969,1.65961825847626,48.35));
#82788=CARTESIAN_POINT('',(89.8664391580969,1.65961825847626,48.5));
#82789=CARTESIAN_POINT('',(89.8664391580969,1.65961825847626,48.35));
#82790=CARTESIAN_POINT('Origin',(88.7874487582594,1.65961825847626,48.5));
#82791=CARTESIAN_POINT('',(44.3937243791297,1.65961825847626,48.5));
#82792=CARTESIAN_POINT('',(88.7874487582594,1.65961825847626,48.35));
#82793=CARTESIAN_POINT('Origin',(89.9999996814877,2.48574362695217,48.35));
#82794=CARTESIAN_POINT('Origin',(0.,8.,48.5));
#82795=CARTESIAN_POINT('Ctrl Pts',(80.8508865237236,3.38540250062943,48.5));
#82796=CARTESIAN_POINT('Ctrl Pts',(80.8508865237236,3.38540250062943,48.35));
#82797=CARTESIAN_POINT('Ctrl Pts',(80.6648020148277,3.38540250062943,48.5));
#82798=CARTESIAN_POINT('Ctrl Pts',(80.6648020148277,3.38540250062943,48.35));
#82799=CARTESIAN_POINT('Ctrl Pts',(80.5537514090538,3.22783091664314,48.5));
#82800=CARTESIAN_POINT('Ctrl Pts',(80.5537514090538,3.22783091664314,48.35));
#82801=CARTESIAN_POINT('',(80.8508865237236,3.38540250062943,48.5));
#82802=CARTESIAN_POINT('',(80.5537514090538,3.22783091664314,48.5));
#82803=CARTESIAN_POINT('Ctrl Pts',(80.8508865237236,3.38540250062943,48.5));
#82804=CARTESIAN_POINT('Ctrl Pts',(80.6648020148277,3.38540250062943,48.5));
#82805=CARTESIAN_POINT('Ctrl Pts',(80.5537514090538,3.22783091664314,48.5));
#82806=CARTESIAN_POINT('',(80.8508865237236,3.38540250062943,48.35));
#82807=CARTESIAN_POINT('',(80.8508865237236,3.38540250062943,48.5));
#82808=CARTESIAN_POINT('',(80.5537514090538,3.22783091664314,48.35));
#82809=CARTESIAN_POINT('Ctrl Pts',(80.8508865237236,3.38540250062943,48.35));
#82810=CARTESIAN_POINT('Ctrl Pts',(80.6648020148277,3.38540250062943,48.35));
#82811=CARTESIAN_POINT('Ctrl Pts',(80.5537514090538,3.22783091664314,48.35));
#82812=CARTESIAN_POINT('',(80.5537514090538,3.22783091664314,48.5));
#82813=CARTESIAN_POINT('Ctrl Pts',(81.1667804121971,3.2068213224411,48.5));
#82814=CARTESIAN_POINT('Ctrl Pts',(81.1667804121971,3.2068213224411,48.35));
#82815=CARTESIAN_POINT('Ctrl Pts',(81.0399727225304,3.38540250062943,48.5));
#82816=CARTESIAN_POINT('Ctrl Pts',(81.0399727225304,3.38540250062943,48.35));
#82817=CARTESIAN_POINT('Ctrl Pts',(80.8508865237236,3.38540250062943,48.5));
#82818=CARTESIAN_POINT('Ctrl Pts',(80.8508865237236,3.38540250062943,48.35));
#82819=CARTESIAN_POINT('',(81.1667804121971,3.2068213224411,48.5));
#82820=CARTESIAN_POINT('Ctrl Pts',(81.1667804121971,3.2068213224411,48.5));
#82821=CARTESIAN_POINT('Ctrl Pts',(81.0399727225304,3.38540250062943,48.5));
#82822=CARTESIAN_POINT('Ctrl Pts',(80.8508865237236,3.38540250062943,48.5));
#82823=CARTESIAN_POINT('',(81.1667804121971,3.2068213224411,48.35));
#82824=CARTESIAN_POINT('',(81.1667804121971,3.2068213224411,48.5));
#82825=CARTESIAN_POINT('Ctrl Pts',(81.1667804121971,3.2068213224411,48.35));
#82826=CARTESIAN_POINT('Ctrl Pts',(81.0399727225304,3.38540250062943,48.35));
#82827=CARTESIAN_POINT('Ctrl Pts',(80.8508865237236,3.38540250062943,48.35));
#82828=CARTESIAN_POINT('Ctrl Pts',(81.2935881018639,2.48499327898026,48.5));
#82829=CARTESIAN_POINT('Ctrl Pts',(81.2935881018639,2.48499327898026,48.35));
#82830=CARTESIAN_POINT('Ctrl Pts',(81.2935881018639,3.02824014425278,48.5));
#82831=CARTESIAN_POINT('Ctrl Pts',(81.2935881018639,3.02824014425278,48.35));
#82832=CARTESIAN_POINT('Ctrl Pts',(81.1667804121971,3.2068213224411,48.5));
#82833=CARTESIAN_POINT('Ctrl Pts',(81.1667804121971,3.2068213224411,48.35));
#82834=CARTESIAN_POINT('',(81.2935881018639,2.48499327898026,48.5));
#82835=CARTESIAN_POINT('Ctrl Pts',(81.2935881018639,2.48499327898026,48.5));
#82836=CARTESIAN_POINT('Ctrl Pts',(81.2935881018639,3.02824014425278,48.5));
#82837=CARTESIAN_POINT('Ctrl Pts',(81.1667804121971,3.2068213224411,48.5));
#82838=CARTESIAN_POINT('',(81.2935881018639,2.48499327898026,48.35));
#82839=CARTESIAN_POINT('',(81.2935881018639,2.48499327898026,48.5));
#82840=CARTESIAN_POINT('Ctrl Pts',(81.2935881018639,2.48499327898026,48.35));
#82841=CARTESIAN_POINT('Ctrl Pts',(81.2935881018639,3.02824014425278,48.35));
#82842=CARTESIAN_POINT('Ctrl Pts',(81.1667804121971,3.2068213224411,48.35));
#82843=CARTESIAN_POINT('Ctrl Pts',(81.1667804121971,1.76466578245163,48.5));
#82844=CARTESIAN_POINT('Ctrl Pts',(81.1667804121971,1.76466578245163,48.35));
#82845=CARTESIAN_POINT('Ctrl Pts',(81.2935881018639,1.9447478055954,48.5));
#82846=CARTESIAN_POINT('Ctrl Pts',(81.2935881018639,1.9447478055954,48.35));
#82847=CARTESIAN_POINT('Ctrl Pts',(81.2935881018639,2.48499327898026,48.5));
#82848=CARTESIAN_POINT('Ctrl Pts',(81.2935881018639,2.48499327898026,48.35));
#82849=CARTESIAN_POINT('',(81.1667804121971,1.76466578245163,48.5));
#82850=CARTESIAN_POINT('Ctrl Pts',(81.1667804121971,1.76466578245163,48.5));
#82851=CARTESIAN_POINT('Ctrl Pts',(81.2935881018639,1.9447478055954,48.5));
#82852=CARTESIAN_POINT('Ctrl Pts',(81.2935881018639,2.48499327898026,48.5));
#82853=CARTESIAN_POINT('',(81.1667804121971,1.76466578245163,48.35));
#82854=CARTESIAN_POINT('',(81.1667804121971,1.76466578245163,48.5));
#82855=CARTESIAN_POINT('Ctrl Pts',(81.1667804121971,1.76466578245163,48.35));
#82856=CARTESIAN_POINT('Ctrl Pts',(81.2935881018639,1.9447478055954,48.35));
#82857=CARTESIAN_POINT('Ctrl Pts',(81.2935881018639,2.48499327898026,48.35));
#82858=CARTESIAN_POINT('Ctrl Pts',(80.8538882136345,1.58458405733109,48.5));
#82859=CARTESIAN_POINT('Ctrl Pts',(80.8538882136345,1.58458405733109,48.35));
#82860=CARTESIAN_POINT('Ctrl Pts',(81.0399727225304,1.58458405733109,48.5));
#82861=CARTESIAN_POINT('Ctrl Pts',(81.0399727225304,1.58458405733109,48.35));
#82862=CARTESIAN_POINT('Ctrl Pts',(81.1667804121971,1.76466578245163,48.5));
#82863=CARTESIAN_POINT('Ctrl Pts',(81.1667804121971,1.76466578245163,48.35));
#82864=CARTESIAN_POINT('',(80.8538882136345,1.58458405733109,48.5));
#82865=CARTESIAN_POINT('Ctrl Pts',(80.8538882136345,1.58458405733109,48.5));
#82866=CARTESIAN_POINT('Ctrl Pts',(81.0399727225304,1.58458405733109,48.5));
#82867=CARTESIAN_POINT('Ctrl Pts',(81.1667804121971,1.76466578245163,48.5));
#82868=CARTESIAN_POINT('',(80.8538882136345,1.58458405733109,48.35));
#82869=CARTESIAN_POINT('',(80.8538882136345,1.58458405733109,48.5));
#82870=CARTESIAN_POINT('Ctrl Pts',(80.8538882136345,1.58458405733109,48.35));
#82871=CARTESIAN_POINT('Ctrl Pts',(81.0399727225304,1.58458405733109,48.35));
#82872=CARTESIAN_POINT('Ctrl Pts',(81.1667804121971,1.76466578245163,48.35));
#82873=CARTESIAN_POINT('Ctrl Pts',(80.5409960150719,1.76391565799713,48.5));
#82874=CARTESIAN_POINT('Ctrl Pts',(80.5409960150719,1.76391565799713,48.35));
#82875=CARTESIAN_POINT('Ctrl Pts',(80.6678034067154,1.58458405733109,48.5));
#82876=CARTESIAN_POINT('Ctrl Pts',(80.6678034067154,1.58458405733109,48.35));
#82877=CARTESIAN_POINT('Ctrl Pts',(80.8538882136345,1.58458405733109,48.5));
#82878=CARTESIAN_POINT('Ctrl Pts',(80.8538882136345,1.58458405733109,48.35));
#82879=CARTESIAN_POINT('',(80.5409960150719,1.76391565799713,48.5));
#82880=CARTESIAN_POINT('Ctrl Pts',(80.5409960150719,1.76391565799713,48.5));
#82881=CARTESIAN_POINT('Ctrl Pts',(80.6678034067154,1.58458405733109,48.5));
#82882=CARTESIAN_POINT('Ctrl Pts',(80.8538882136345,1.58458405733109,48.5));
#82883=CARTESIAN_POINT('',(80.5409960150719,1.76391565799713,48.35));
#82884=CARTESIAN_POINT('',(80.5409960150719,1.76391565799713,48.5));
#82885=CARTESIAN_POINT('Ctrl Pts',(80.5409960150719,1.76391565799713,48.35));
#82886=CARTESIAN_POINT('Ctrl Pts',(80.6678034067154,1.58458405733109,48.35));
#82887=CARTESIAN_POINT('Ctrl Pts',(80.8538882136345,1.58458405733109,48.35));
#82888=CARTESIAN_POINT('Ctrl Pts',(80.4141883254051,2.48499327898026,48.5));
#82889=CARTESIAN_POINT('Ctrl Pts',(80.4141883254051,2.48499327898026,48.35));
#82890=CARTESIAN_POINT('Ctrl Pts',(80.4141883254051,1.94324696063995,48.5));
#82891=CARTESIAN_POINT('Ctrl Pts',(80.4141883254051,1.94324696063995,48.35));
#82892=CARTESIAN_POINT('Ctrl Pts',(80.5409960150719,1.76391565799713,48.5));
#82893=CARTESIAN_POINT('Ctrl Pts',(80.5409960150719,1.76391565799713,48.35));
#82894=CARTESIAN_POINT('',(80.4141883254051,2.48499327898026,48.5));
#82895=CARTESIAN_POINT('Ctrl Pts',(80.4141883254051,2.48499327898026,48.5));
#82896=CARTESIAN_POINT('Ctrl Pts',(80.4141883254051,1.94324696063995,48.5));
#82897=CARTESIAN_POINT('Ctrl Pts',(80.5409960150719,1.76391565799713,48.5));
#82898=CARTESIAN_POINT('',(80.4141883254051,2.48499327898026,48.35));
#82899=CARTESIAN_POINT('',(80.4141883254051,2.48499327898026,48.5));
#82900=CARTESIAN_POINT('Ctrl Pts',(80.4141883254051,2.48499327898026,48.35));
#82901=CARTESIAN_POINT('Ctrl Pts',(80.4141883254051,1.94324696063995,48.35));
#82902=CARTESIAN_POINT('Ctrl Pts',(80.5409960150719,1.76391565799713,48.35));
#82903=CARTESIAN_POINT('Ctrl Pts',(80.5537514090538,3.22783091664314,48.5));
#82904=CARTESIAN_POINT('Ctrl Pts',(80.5537514090538,3.22783091664314,48.35));
#82905=CARTESIAN_POINT('Ctrl Pts',(80.4141883254051,3.02673944830894,48.5));
#82906=CARTESIAN_POINT('Ctrl Pts',(80.4141883254051,3.02673944830894,48.35));
#82907=CARTESIAN_POINT('Ctrl Pts',(80.4141883254051,2.48499327898026,48.5));
#82908=CARTESIAN_POINT('Ctrl Pts',(80.4141883254051,2.48499327898026,48.35));
#82909=CARTESIAN_POINT('Ctrl Pts',(80.5537514090538,3.22783091664314,48.5));
#82910=CARTESIAN_POINT('Ctrl Pts',(80.4141883254051,3.02673944830894,48.5));
#82911=CARTESIAN_POINT('Ctrl Pts',(80.4141883254051,2.48499327898026,48.5));
#82912=CARTESIAN_POINT('Ctrl Pts',(80.5537514090538,3.22783091664314,48.35));
#82913=CARTESIAN_POINT('Ctrl Pts',(80.4141883254051,3.02673944830894,48.35));
#82914=CARTESIAN_POINT('Ctrl Pts',(80.4141883254051,2.48499327898026,48.35));
#82915=CARTESIAN_POINT('Ctrl Pts',(80.8538882136345,1.36248314380646,48.5));
#82916=CARTESIAN_POINT('Ctrl Pts',(80.8538882136345,1.36248314380646,48.35));
#82917=CARTESIAN_POINT('Ctrl Pts',(80.535743355751,1.36248314380646,48.5));
#82918=CARTESIAN_POINT('Ctrl Pts',(80.535743355751,1.36248314380646,48.35));
#82919=CARTESIAN_POINT('Ctrl Pts',(80.3541610836983,1.59058684110642,48.5));
#82920=CARTESIAN_POINT('Ctrl Pts',(80.3541610836983,1.59058684110642,48.35));
#82921=CARTESIAN_POINT('',(80.8538882136345,1.36248314380646,48.5));
#82922=CARTESIAN_POINT('',(80.3541610836983,1.59058684110642,48.5));
#82923=CARTESIAN_POINT('Ctrl Pts',(80.8538882136345,1.36248314380646,48.5));
#82924=CARTESIAN_POINT('Ctrl Pts',(80.535743355751,1.36248314380646,48.5));
#82925=CARTESIAN_POINT('Ctrl Pts',(80.3541610836983,1.59058684110642,48.5));
#82926=CARTESIAN_POINT('',(80.8538882136345,1.36248314380646,48.35));
#82927=CARTESIAN_POINT('',(80.8538882136345,1.36248314380646,48.5));
#82928=CARTESIAN_POINT('',(80.3541610836983,1.59058684110642,48.35));
#82929=CARTESIAN_POINT('Ctrl Pts',(80.8538882136345,1.36248314380646,48.35));
#82930=CARTESIAN_POINT('Ctrl Pts',(80.535743355751,1.36248314380646,48.35));
#82931=CARTESIAN_POINT('Ctrl Pts',(80.3541610836983,1.59058684110642,48.35));
#82932=CARTESIAN_POINT('',(80.3541610836983,1.59058684110642,48.5));
#82933=CARTESIAN_POINT('Ctrl Pts',(81.2538198828697,1.49229192733765,48.5));
#82934=CARTESIAN_POINT('Ctrl Pts',(81.2538198828697,1.49229192733765,48.35));
#82935=CARTESIAN_POINT('Ctrl Pts',(81.0954980254173,1.36248314380646,48.5));
#82936=CARTESIAN_POINT('Ctrl Pts',(81.0954980254173,1.36248314380646,48.35));
#82937=CARTESIAN_POINT('Ctrl Pts',(80.8538882136345,1.36248314380646,48.5));
#82938=CARTESIAN_POINT('Ctrl Pts',(80.8538882136345,1.36248314380646,48.35));
#82939=CARTESIAN_POINT('',(81.2538198828697,1.49229192733765,48.5));
#82940=CARTESIAN_POINT('Ctrl Pts',(81.2538198828697,1.49229192733765,48.5));
#82941=CARTESIAN_POINT('Ctrl Pts',(81.0954980254173,1.36248314380646,48.5));
#82942=CARTESIAN_POINT('Ctrl Pts',(80.8538882136345,1.36248314380646,48.5));
#82943=CARTESIAN_POINT('',(81.2538198828697,1.49229192733765,48.35));
#82944=CARTESIAN_POINT('',(81.2538198828697,1.49229192733765,48.5));
#82945=CARTESIAN_POINT('Ctrl Pts',(81.2538198828697,1.49229192733765,48.35));
#82946=CARTESIAN_POINT('Ctrl Pts',(81.0954980254173,1.36248314380646,48.35));
#82947=CARTESIAN_POINT('Ctrl Pts',(80.8538882136345,1.36248314380646,48.35));
#82948=CARTESIAN_POINT('Ctrl Pts',(81.4916781783104,1.85995900630951,48.5));
#82949=CARTESIAN_POINT('Ctrl Pts',(81.4916781783104,1.85995900630951,48.35));
#82950=CARTESIAN_POINT('Ctrl Pts',(81.4121417403221,1.62210100889206,48.5));
#82951=CARTESIAN_POINT('Ctrl Pts',(81.4121417403221,1.62210100889206,48.35));
#82952=CARTESIAN_POINT('Ctrl Pts',(81.2538198828697,1.49229192733765,48.5));
#82953=CARTESIAN_POINT('Ctrl Pts',(81.2538198828697,1.49229192733765,48.35));
#82954=CARTESIAN_POINT('',(81.4916781783104,1.85995900630951,48.5));
#82955=CARTESIAN_POINT('Ctrl Pts',(81.4916781783104,1.85995900630951,48.5));
#82956=CARTESIAN_POINT('Ctrl Pts',(81.4121417403221,1.62210100889206,48.5));
#82957=CARTESIAN_POINT('Ctrl Pts',(81.2538198828697,1.49229192733765,48.5));
#82958=CARTESIAN_POINT('',(81.4916781783104,1.85995900630951,48.35));
#82959=CARTESIAN_POINT('',(81.4916781783104,1.85995900630951,48.5));
#82960=CARTESIAN_POINT('Ctrl Pts',(81.4916781783104,1.85995900630951,48.35));
#82961=CARTESIAN_POINT('Ctrl Pts',(81.4121417403221,1.62210100889206,48.35));
#82962=CARTESIAN_POINT('Ctrl Pts',(81.2538198828697,1.49229192733765,48.35));
#82963=CARTESIAN_POINT('Ctrl Pts',(81.5712140202522,2.48499327898026,48.5));
#82964=CARTESIAN_POINT('Ctrl Pts',(81.5712140202522,2.48499327898026,48.35));
#82965=CARTESIAN_POINT('Ctrl Pts',(81.5712140202522,2.09781730175018,48.5));
#82966=CARTESIAN_POINT('Ctrl Pts',(81.5712140202522,2.09781730175018,48.35));
#82967=CARTESIAN_POINT('Ctrl Pts',(81.4916781783104,1.85995900630951,48.5));
#82968=CARTESIAN_POINT('Ctrl Pts',(81.4916781783104,1.85995900630951,48.35));
#82969=CARTESIAN_POINT('',(81.5712140202522,2.48499327898026,48.5));
#82970=CARTESIAN_POINT('Ctrl Pts',(81.5712140202522,2.48499327898026,48.5));
#82971=CARTESIAN_POINT('Ctrl Pts',(81.5712140202522,2.09781730175018,48.5));
#82972=CARTESIAN_POINT('Ctrl Pts',(81.4916781783104,1.85995900630951,48.5));
#82973=CARTESIAN_POINT('',(81.5712140202522,2.48499327898026,48.35));
#82974=CARTESIAN_POINT('',(81.5712140202522,2.48499327898026,48.5));
#82975=CARTESIAN_POINT('Ctrl Pts',(81.5712140202522,2.48499327898026,48.35));
#82976=CARTESIAN_POINT('Ctrl Pts',(81.5712140202522,2.09781730175018,48.35));
#82977=CARTESIAN_POINT('Ctrl Pts',(81.4916781783104,1.85995900630951,48.35));
#82978=CARTESIAN_POINT('Ctrl Pts',(81.5216915011406,3.00497958064079,48.5));
#82979=CARTESIAN_POINT('Ctrl Pts',(81.5216915011406,3.00497958064079,48.35));
#82980=CARTESIAN_POINT('Ctrl Pts',(81.5712140202522,2.81214186549187,48.5));
#82981=CARTESIAN_POINT('Ctrl Pts',(81.5712140202522,2.81214186549187,48.35));
#82982=CARTESIAN_POINT('Ctrl Pts',(81.5712140202522,2.48499327898026,48.5));
#82983=CARTESIAN_POINT('Ctrl Pts',(81.5712140202522,2.48499327898026,48.35));
#82984=CARTESIAN_POINT('',(81.5216915011406,3.00497958064079,48.5));
#82985=CARTESIAN_POINT('Ctrl Pts',(81.5216915011406,3.00497958064079,48.5));
#82986=CARTESIAN_POINT('Ctrl Pts',(81.5712140202522,2.81214186549187,48.5));
#82987=CARTESIAN_POINT('Ctrl Pts',(81.5712140202522,2.48499327898026,48.5));
#82988=CARTESIAN_POINT('',(81.5216915011406,3.00497958064079,48.35));
#82989=CARTESIAN_POINT('',(81.5216915011406,3.00497958064079,48.5));
#82990=CARTESIAN_POINT('Ctrl Pts',(81.5216915011406,3.00497958064079,48.35));
#82991=CARTESIAN_POINT('Ctrl Pts',(81.5712140202522,2.81214186549187,48.35));
#82992=CARTESIAN_POINT('Ctrl Pts',(81.5712140202522,2.48499327898026,48.35));
#82993=CARTESIAN_POINT('Ctrl Pts',(81.3851295113564,3.33212831616402,48.5));
#82994=CARTESIAN_POINT('Ctrl Pts',(81.3851295113564,3.33212831616402,48.35));
#82995=CARTESIAN_POINT('Ctrl Pts',(81.472168982029,3.19781729578972,48.5));
#82996=CARTESIAN_POINT('Ctrl Pts',(81.472168982029,3.19781729578972,48.35));
#82997=CARTESIAN_POINT('Ctrl Pts',(81.5216915011406,3.00497958064079,48.5));
#82998=CARTESIAN_POINT('Ctrl Pts',(81.5216915011406,3.00497958064079,48.35));
#82999=CARTESIAN_POINT('',(81.3851295113564,3.33212831616402,48.5));
#83000=CARTESIAN_POINT('Ctrl Pts',(81.3851295113564,3.33212831616402,48.5));
#83001=CARTESIAN_POINT('Ctrl Pts',(81.472168982029,3.19781729578972,48.5));
#83002=CARTESIAN_POINT('Ctrl Pts',(81.5216915011406,3.00497958064079,48.5));
#83003=CARTESIAN_POINT('',(81.3851295113564,3.33212831616402,48.35));
#83004=CARTESIAN_POINT('',(81.3851295113564,3.33212831616402,48.5));
#83005=CARTESIAN_POINT('Ctrl Pts',(81.3851295113564,3.33212831616402,48.35));
#83006=CARTESIAN_POINT('Ctrl Pts',(81.472168982029,3.19781729578972,48.35));
#83007=CARTESIAN_POINT('Ctrl Pts',(81.5216915011406,3.00497958064079,48.35));
#83008=CARTESIAN_POINT('Ctrl Pts',(81.1645291447639,3.5377217233181,48.5));
#83009=CARTESIAN_POINT('Ctrl Pts',(81.1645291447639,3.5377217233181,48.35));
#83010=CARTESIAN_POINT('Ctrl Pts',(81.2980900406837,3.46643933653831,48.5));
#83011=CARTESIAN_POINT('Ctrl Pts',(81.2980900406837,3.46643933653831,48.35));
#83012=CARTESIAN_POINT('Ctrl Pts',(81.3851295113564,3.33212831616402,48.5));
#83013=CARTESIAN_POINT('Ctrl Pts',(81.3851295113564,3.33212831616402,48.35));
#83014=CARTESIAN_POINT('',(81.1645291447639,3.5377217233181,48.5));
#83015=CARTESIAN_POINT('Ctrl Pts',(81.1645291447639,3.5377217233181,48.5));
#83016=CARTESIAN_POINT('Ctrl Pts',(81.2980900406837,3.46643933653831,48.5));
#83017=CARTESIAN_POINT('Ctrl Pts',(81.3851295113564,3.33212831616402,48.5));
#83018=CARTESIAN_POINT('',(81.1645291447639,3.5377217233181,48.35));
#83019=CARTESIAN_POINT('',(81.1645291447639,3.5377217233181,48.5));
#83020=CARTESIAN_POINT('Ctrl Pts',(81.1645291447639,3.5377217233181,48.35));
#83021=CARTESIAN_POINT('Ctrl Pts',(81.2980900406837,3.46643933653831,48.35));
#83022=CARTESIAN_POINT('Ctrl Pts',(81.3851295113564,3.33212831616402,48.35));
#83023=CARTESIAN_POINT('Ctrl Pts',(80.8538882136345,3.60900411009789,48.5));
#83024=CARTESIAN_POINT('Ctrl Pts',(80.8538882136345,3.60900411009789,48.35));
#83025=CARTESIAN_POINT('Ctrl Pts',(81.0309682488441,3.60900411009789,48.5));
#83026=CARTESIAN_POINT('Ctrl Pts',(81.0309682488441,3.60900411009789,48.35));
#83027=CARTESIAN_POINT('Ctrl Pts',(81.1645291447639,3.5377217233181,48.5));
#83028=CARTESIAN_POINT('Ctrl Pts',(81.1645291447639,3.5377217233181,48.35));
#83029=CARTESIAN_POINT('',(80.8538882136345,3.60900411009789,48.5));
#83030=CARTESIAN_POINT('Ctrl Pts',(80.8538882136345,3.60900411009789,48.5));
#83031=CARTESIAN_POINT('Ctrl Pts',(81.0309682488441,3.60900411009789,48.5));
#83032=CARTESIAN_POINT('Ctrl Pts',(81.1645291447639,3.5377217233181,48.5));
#83033=CARTESIAN_POINT('',(80.8538882136345,3.60900411009789,48.35));
#83034=CARTESIAN_POINT('',(80.8538882136345,3.60900411009789,48.5));
#83035=CARTESIAN_POINT('Ctrl Pts',(80.8538882136345,3.60900411009789,48.35));
#83036=CARTESIAN_POINT('Ctrl Pts',(81.0309682488441,3.60900411009789,48.35));
#83037=CARTESIAN_POINT('Ctrl Pts',(81.1645291447639,3.5377217233181,48.35));
#83038=CARTESIAN_POINT('Ctrl Pts',(80.4554567933083,3.47994545102119,48.5));
#83039=CARTESIAN_POINT('Ctrl Pts',(80.4554567933083,3.47994545102119,48.35));
#83040=CARTESIAN_POINT('Ctrl Pts',(80.6137786507607,3.60900411009789,48.5));
#83041=CARTESIAN_POINT('Ctrl Pts',(80.6137786507607,3.60900411009789,48.35));
#83042=CARTESIAN_POINT('Ctrl Pts',(80.8538882136345,3.60900411009789,48.5));
#83043=CARTESIAN_POINT('Ctrl Pts',(80.8538882136345,3.60900411009789,48.35));
#83044=CARTESIAN_POINT('',(80.4554567933083,3.47994545102119,48.5));
#83045=CARTESIAN_POINT('Ctrl Pts',(80.4554567933083,3.47994545102119,48.5));
#83046=CARTESIAN_POINT('Ctrl Pts',(80.6137786507607,3.60900411009789,48.5));
#83047=CARTESIAN_POINT('Ctrl Pts',(80.8538882136345,3.60900411009789,48.5));
#83048=CARTESIAN_POINT('',(80.4554567933083,3.47994545102119,48.35));
#83049=CARTESIAN_POINT('',(80.4554567933083,3.47994545102119,48.5));
#83050=CARTESIAN_POINT('Ctrl Pts',(80.4554567933083,3.47994545102119,48.35));
#83051=CARTESIAN_POINT('Ctrl Pts',(80.6137786507607,3.60900411009789,48.35));
#83052=CARTESIAN_POINT('Ctrl Pts',(80.8538882136345,3.60900411009789,48.35));
#83053=CARTESIAN_POINT('Ctrl Pts',(80.2168486714363,3.11302864551544,48.5));
#83054=CARTESIAN_POINT('Ctrl Pts',(80.2168486714363,3.11302864551544,48.35));
#83055=CARTESIAN_POINT('Ctrl Pts',(80.2971349358559,3.3508867919445,48.5));
#83056=CARTESIAN_POINT('Ctrl Pts',(80.2971349358559,3.3508867919445,48.35));
#83057=CARTESIAN_POINT('Ctrl Pts',(80.4554567933083,3.47994545102119,48.5));
#83058=CARTESIAN_POINT('Ctrl Pts',(80.4554567933083,3.47994545102119,48.35));
#83059=CARTESIAN_POINT('',(80.2168486714363,3.11302864551544,48.5));
#83060=CARTESIAN_POINT('Ctrl Pts',(80.2168486714363,3.11302864551544,48.5));
#83061=CARTESIAN_POINT('Ctrl Pts',(80.2971349358559,3.3508867919445,48.5));
#83062=CARTESIAN_POINT('Ctrl Pts',(80.4554567933083,3.47994545102119,48.5));
#83063=CARTESIAN_POINT('',(80.2168486714363,3.11302864551544,48.35));
#83064=CARTESIAN_POINT('',(80.2168486714363,3.11302864551544,48.5));
#83065=CARTESIAN_POINT('Ctrl Pts',(80.2168486714363,3.11302864551544,48.35));
#83066=CARTESIAN_POINT('Ctrl Pts',(80.2971349358559,3.3508867919445,48.35));
#83067=CARTESIAN_POINT('Ctrl Pts',(80.4554567933083,3.47994545102119,48.35));
#83068=CARTESIAN_POINT('Ctrl Pts',(80.1365618109703,2.48499327898026,48.5));
#83069=CARTESIAN_POINT('Ctrl Pts',(80.1365618109703,2.48499327898026,48.35));
#83070=CARTESIAN_POINT('Ctrl Pts',(80.1365618109703,2.87517049908638,48.5));
#83071=CARTESIAN_POINT('Ctrl Pts',(80.1365618109703,2.87517049908638,48.35));
#83072=CARTESIAN_POINT('Ctrl Pts',(80.2168486714363,3.11302864551544,48.5));
#83073=CARTESIAN_POINT('Ctrl Pts',(80.2168486714363,3.11302864551544,48.35));
#83074=CARTESIAN_POINT('',(80.1365618109703,2.48499327898026,48.5));
#83075=CARTESIAN_POINT('Ctrl Pts',(80.1365618109703,2.48499327898026,48.5));
#83076=CARTESIAN_POINT('Ctrl Pts',(80.1365618109703,2.87517049908638,48.5));
#83077=CARTESIAN_POINT('Ctrl Pts',(80.2168486714363,3.11302864551544,48.5));
#83078=CARTESIAN_POINT('',(80.1365618109703,2.48499327898026,48.35));
#83079=CARTESIAN_POINT('',(80.1365618109703,2.48499327898026,48.5));
#83080=CARTESIAN_POINT('Ctrl Pts',(80.1365618109703,2.48499327898026,48.35));
#83081=CARTESIAN_POINT('Ctrl Pts',(80.1365618109703,2.87517049908638,48.35));
#83082=CARTESIAN_POINT('Ctrl Pts',(80.2168486714363,3.11302864551544,48.35));
#83083=CARTESIAN_POINT('Ctrl Pts',(80.3541610836983,1.59058684110642,48.5));
#83084=CARTESIAN_POINT('Ctrl Pts',(80.3541610836983,1.59058684110642,48.35));
#83085=CARTESIAN_POINT('Ctrl Pts',(80.1365618109703,1.86521166563034,48.5));
#83086=CARTESIAN_POINT('Ctrl Pts',(80.1365618109703,1.86521166563034,48.35));
#83087=CARTESIAN_POINT('Ctrl Pts',(80.1365618109703,2.48499327898026,48.5));
#83088=CARTESIAN_POINT('Ctrl Pts',(80.1365618109703,2.48499327898026,48.35));
#83089=CARTESIAN_POINT('Ctrl Pts',(80.3541610836983,1.59058684110642,48.5));
#83090=CARTESIAN_POINT('Ctrl Pts',(80.1365618109703,1.86521166563034,48.5));
#83091=CARTESIAN_POINT('Ctrl Pts',(80.1365618109703,2.48499327898026,48.5));
#83092=CARTESIAN_POINT('Ctrl Pts',(80.3541610836983,1.59058684110642,48.35));
#83093=CARTESIAN_POINT('Ctrl Pts',(80.1365618109703,1.86521166563034,48.35));
#83094=CARTESIAN_POINT('Ctrl Pts',(80.1365618109703,2.48499327898026,48.35));
#83095=CARTESIAN_POINT('Origin',(79.9999998956919,2.48499320447445,48.35));
#83096=CARTESIAN_POINT('Ctrl Pts',(79.1281036734581,1.36098229885101,48.5));
#83097=CARTESIAN_POINT('Ctrl Pts',(79.1281036734581,1.36098229885101,48.35));
#83098=CARTESIAN_POINT('Ctrl Pts',(78.8384720385075,1.36098229885101,48.5));
#83099=CARTESIAN_POINT('Ctrl Pts',(78.8384720385075,1.36098229885101,48.35));
#83100=CARTESIAN_POINT('Ctrl Pts',(78.6471350193024,1.53356069326401,48.5));
#83101=CARTESIAN_POINT('Ctrl Pts',(78.6471350193024,1.53356069326401,48.35));
#83102=CARTESIAN_POINT('',(79.1281036734581,1.36098229885101,48.5));
#83103=CARTESIAN_POINT('',(78.6471350193024,1.53356069326401,48.5));
#83104=CARTESIAN_POINT('Ctrl Pts',(79.1281036734581,1.36098229885101,48.5));
#83105=CARTESIAN_POINT('Ctrl Pts',(78.8384720385075,1.36098229885101,48.5));
#83106=CARTESIAN_POINT('Ctrl Pts',(78.6471350193024,1.53356069326401,48.5));
#83107=CARTESIAN_POINT('',(79.1281036734581,1.36098229885101,48.35));
#83108=CARTESIAN_POINT('',(79.1281036734581,1.36098229885101,48.5));
#83109=CARTESIAN_POINT('',(78.6471350193024,1.53356069326401,48.35));
#83110=CARTESIAN_POINT('Ctrl Pts',(79.1281036734581,1.36098229885101,48.35));
#83111=CARTESIAN_POINT('Ctrl Pts',(78.8384720385075,1.36098229885101,48.35));
#83112=CARTESIAN_POINT('Ctrl Pts',(78.6471350193024,1.53356069326401,48.35));
#83113=CARTESIAN_POINT('',(78.6471350193024,1.53356069326401,48.5));
#83114=CARTESIAN_POINT('Ctrl Pts',(79.65934497118,1.56132334470749,48.5));
#83115=CARTESIAN_POINT('Ctrl Pts',(79.65934497118,1.56132334470749,48.35));
#83116=CARTESIAN_POINT('Ctrl Pts',(79.449249625206,1.36098229885101,48.5));
#83117=CARTESIAN_POINT('Ctrl Pts',(79.449249625206,1.36098229885101,48.35));
#83118=CARTESIAN_POINT('Ctrl Pts',(79.1281036734581,1.36098229885101,48.5));
#83119=CARTESIAN_POINT('Ctrl Pts',(79.1281036734581,1.36098229885101,48.35));
#83120=CARTESIAN_POINT('',(79.65934497118,1.56132334470749,48.5));
#83121=CARTESIAN_POINT('Ctrl Pts',(79.65934497118,1.56132334470749,48.5));
#83122=CARTESIAN_POINT('Ctrl Pts',(79.449249625206,1.36098229885101,48.5));
#83123=CARTESIAN_POINT('Ctrl Pts',(79.1281036734581,1.36098229885101,48.5));
#83124=CARTESIAN_POINT('',(79.65934497118,1.56132334470749,48.35));
#83125=CARTESIAN_POINT('',(79.65934497118,1.56132334470749,48.5));
#83126=CARTESIAN_POINT('Ctrl Pts',(79.65934497118,1.56132334470749,48.35));
#83127=CARTESIAN_POINT('Ctrl Pts',(79.449249625206,1.36098229885101,48.35));
#83128=CARTESIAN_POINT('Ctrl Pts',(79.1281036734581,1.36098229885101,48.35));
#83129=CARTESIAN_POINT('Ctrl Pts',(79.8694406151772,2.04979562759399,48.5));
#83130=CARTESIAN_POINT('Ctrl Pts',(79.8694406151772,2.04979562759399,48.35));
#83131=CARTESIAN_POINT('Ctrl Pts',(79.8694406151772,1.76166439056397,48.5));
#83132=CARTESIAN_POINT('Ctrl Pts',(79.8694406151772,1.76166439056397,48.35));
#83133=CARTESIAN_POINT('Ctrl Pts',(79.65934497118,1.56132334470749,48.5));
#83134=CARTESIAN_POINT('Ctrl Pts',(79.65934497118,1.56132334470749,48.35));
#83135=CARTESIAN_POINT('',(79.8694406151772,2.04979562759399,48.5));
#83136=CARTESIAN_POINT('Ctrl Pts',(79.8694406151772,2.04979562759399,48.5));
#83137=CARTESIAN_POINT('Ctrl Pts',(79.8694406151772,1.76166439056397,48.5));
#83138=CARTESIAN_POINT('Ctrl Pts',(79.65934497118,1.56132334470749,48.5));
#83139=CARTESIAN_POINT('',(79.8694406151772,2.04979562759399,48.35));
#83140=CARTESIAN_POINT('',(79.8694406151772,2.04979562759399,48.5));
#83141=CARTESIAN_POINT('Ctrl Pts',(79.8694406151772,2.04979562759399,48.35));
#83142=CARTESIAN_POINT('Ctrl Pts',(79.8694406151772,1.76166439056397,48.35));
#83143=CARTESIAN_POINT('Ctrl Pts',(79.65934497118,1.56132334470749,48.35));
#83144=CARTESIAN_POINT('Ctrl Pts',(79.7613916993141,2.40470671653748,48.5));
#83145=CARTESIAN_POINT('Ctrl Pts',(79.7613916993141,2.40470671653748,48.35));
#83146=CARTESIAN_POINT('Ctrl Pts',(79.8694406151772,2.26289236545563,48.5));
#83147=CARTESIAN_POINT('Ctrl Pts',(79.8694406151772,2.26289236545563,48.35));
#83148=CARTESIAN_POINT('Ctrl Pts',(79.8694406151772,2.04979562759399,48.5));
#83149=CARTESIAN_POINT('Ctrl Pts',(79.8694406151772,2.04979562759399,48.35));
#83150=CARTESIAN_POINT('',(79.7613916993141,2.40470671653748,48.5));
#83151=CARTESIAN_POINT('Ctrl Pts',(79.7613916993141,2.40470671653748,48.5));
#83152=CARTESIAN_POINT('Ctrl Pts',(79.8694406151772,2.26289236545563,48.5));
#83153=CARTESIAN_POINT('Ctrl Pts',(79.8694406151772,2.04979562759399,48.5));
#83154=CARTESIAN_POINT('',(79.7613916993141,2.40470671653748,48.35));
#83155=CARTESIAN_POINT('',(79.7613916993141,2.40470671653748,48.5));
#83156=CARTESIAN_POINT('Ctrl Pts',(79.7613916993141,2.40470671653748,48.35));
#83157=CARTESIAN_POINT('Ctrl Pts',(79.8694406151772,2.26289236545563,48.35));
#83158=CARTESIAN_POINT('Ctrl Pts',(79.8694406151772,2.04979562759399,48.35));
#83159=CARTESIAN_POINT('Ctrl Pts',(79.458253800869,2.59154164791107,48.5));
#83160=CARTESIAN_POINT('Ctrl Pts',(79.458253800869,2.59154164791107,48.35));
#83161=CARTESIAN_POINT('Ctrl Pts',(79.6533421874046,2.54652121663094,48.5));
#83162=CARTESIAN_POINT('Ctrl Pts',(79.6533421874046,2.54652121663094,48.35));
#83163=CARTESIAN_POINT('Ctrl Pts',(79.7613916993141,2.40470671653748,48.5));
#83164=CARTESIAN_POINT('Ctrl Pts',(79.7613916993141,2.40470671653748,48.35));
#83165=CARTESIAN_POINT('',(79.458253800869,2.59154164791107,48.5));
#83166=CARTESIAN_POINT('Ctrl Pts',(79.458253800869,2.59154164791107,48.5));
#83167=CARTESIAN_POINT('Ctrl Pts',(79.6533421874046,2.54652121663094,48.5));
#83168=CARTESIAN_POINT('Ctrl Pts',(79.7613916993141,2.40470671653748,48.5));
#83169=CARTESIAN_POINT('',(79.458253800869,2.59154164791107,48.35));
#83170=CARTESIAN_POINT('',(79.458253800869,2.59154164791107,48.5));
#83171=CARTESIAN_POINT('Ctrl Pts',(79.458253800869,2.59154164791107,48.35));
#83172=CARTESIAN_POINT('Ctrl Pts',(79.6533421874046,2.54652121663094,48.35));
#83173=CARTESIAN_POINT('Ctrl Pts',(79.7613916993141,2.40470671653748,48.35));
#83174=CARTESIAN_POINT('Ctrl Pts',(79.6848566532135,2.77762615680695,48.5));
#83175=CARTESIAN_POINT('Ctrl Pts',(79.6848566532135,2.77762615680695,48.35));
#83176=CARTESIAN_POINT('Ctrl Pts',(79.6083219051361,2.66057306528091,48.5));
#83177=CARTESIAN_POINT('Ctrl Pts',(79.6083219051361,2.66057306528091,48.35));
#83178=CARTESIAN_POINT('Ctrl Pts',(79.458253800869,2.59154164791107,48.5));
#83179=CARTESIAN_POINT('Ctrl Pts',(79.458253800869,2.59154164791107,48.35));
#83180=CARTESIAN_POINT('',(79.6848566532135,2.77762615680695,48.5));
#83181=CARTESIAN_POINT('Ctrl Pts',(79.6848566532135,2.77762615680695,48.5));
#83182=CARTESIAN_POINT('Ctrl Pts',(79.6083219051361,2.66057306528091,48.5));
#83183=CARTESIAN_POINT('Ctrl Pts',(79.458253800869,2.59154164791107,48.5));
#83184=CARTESIAN_POINT('',(79.6848566532135,2.77762615680695,48.35));
#83185=CARTESIAN_POINT('',(79.6848566532135,2.77762615680695,48.5));
#83186=CARTESIAN_POINT('Ctrl Pts',(79.6848566532135,2.77762615680695,48.35));
#83187=CARTESIAN_POINT('Ctrl Pts',(79.6083219051361,2.66057306528091,48.35));
#83188=CARTESIAN_POINT('Ctrl Pts',(79.458253800869,2.59154164791107,48.35));
#83189=CARTESIAN_POINT('Ctrl Pts',(79.7613916993141,3.03724417090416,48.5));
#83190=CARTESIAN_POINT('Ctrl Pts',(79.7613916993141,3.03724417090416,48.35));
#83191=CARTESIAN_POINT('Ctrl Pts',(79.7613916993141,2.89467939734459,48.5));
#83192=CARTESIAN_POINT('Ctrl Pts',(79.7613916993141,2.89467939734459,48.35));
#83193=CARTESIAN_POINT('Ctrl Pts',(79.6848566532135,2.77762615680695,48.5));
#83194=CARTESIAN_POINT('Ctrl Pts',(79.6848566532135,2.77762615680695,48.35));
#83195=CARTESIAN_POINT('',(79.7613916993141,3.03724417090416,48.5));
#83196=CARTESIAN_POINT('Ctrl Pts',(79.7613916993141,3.03724417090416,48.5));
#83197=CARTESIAN_POINT('Ctrl Pts',(79.7613916993141,2.89467939734459,48.5));
#83198=CARTESIAN_POINT('Ctrl Pts',(79.6848566532135,2.77762615680695,48.5));
#83199=CARTESIAN_POINT('',(79.7613916993141,3.03724417090416,48.35));
#83200=CARTESIAN_POINT('',(79.7613916993141,3.03724417090416,48.5));
#83201=CARTESIAN_POINT('Ctrl Pts',(79.7613916993141,3.03724417090416,48.35));
#83202=CARTESIAN_POINT('Ctrl Pts',(79.7613916993141,2.89467939734459,48.35));
#83203=CARTESIAN_POINT('Ctrl Pts',(79.6848566532135,2.77762615680695,48.35));
#83204=CARTESIAN_POINT('Ctrl Pts',(79.6811048388481,3.32087317109108,48.5));
#83205=CARTESIAN_POINT('Ctrl Pts',(79.6811048388481,3.32087317109108,48.35));
#83206=CARTESIAN_POINT('Ctrl Pts',(79.7613916993141,3.18731242418289,48.5));
#83207=CARTESIAN_POINT('Ctrl Pts',(79.7613916993141,3.18731242418289,48.35));
#83208=CARTESIAN_POINT('Ctrl Pts',(79.7613916993141,3.03724417090416,48.5));
#83209=CARTESIAN_POINT('Ctrl Pts',(79.7613916993141,3.03724417090416,48.35));
#83210=CARTESIAN_POINT('',(79.6811048388481,3.32087317109108,48.5));
#83211=CARTESIAN_POINT('Ctrl Pts',(79.6811048388481,3.32087317109108,48.5));
#83212=CARTESIAN_POINT('Ctrl Pts',(79.7613916993141,3.18731242418289,48.5));
#83213=CARTESIAN_POINT('Ctrl Pts',(79.7613916993141,3.03724417090416,48.5));
#83214=CARTESIAN_POINT('',(79.6811048388481,3.32087317109108,48.35));
#83215=CARTESIAN_POINT('',(79.6811048388481,3.32087317109108,48.5));
#83216=CARTESIAN_POINT('Ctrl Pts',(79.6811048388481,3.32087317109108,48.35));
#83217=CARTESIAN_POINT('Ctrl Pts',(79.7613916993141,3.18731242418289,48.35));
#83218=CARTESIAN_POINT('Ctrl Pts',(79.7613916993141,3.03724417090416,48.35));
#83219=CARTESIAN_POINT('Ctrl Pts',(79.449249625206,3.53171893954277,48.5));
#83220=CARTESIAN_POINT('Ctrl Pts',(79.449249625206,3.53171893954277,48.35));
#83221=CARTESIAN_POINT('Ctrl Pts',(79.6008185744286,3.45443391799927,48.5));
#83222=CARTESIAN_POINT('Ctrl Pts',(79.6008185744286,3.45443391799927,48.35));
#83223=CARTESIAN_POINT('Ctrl Pts',(79.6811048388481,3.32087317109108,48.5));
#83224=CARTESIAN_POINT('Ctrl Pts',(79.6811048388481,3.32087317109108,48.35));
#83225=CARTESIAN_POINT('',(79.449249625206,3.53171893954277,48.5));
#83226=CARTESIAN_POINT('Ctrl Pts',(79.449249625206,3.53171893954277,48.5));
#83227=CARTESIAN_POINT('Ctrl Pts',(79.6008185744286,3.45443391799927,48.5));
#83228=CARTESIAN_POINT('Ctrl Pts',(79.6811048388481,3.32087317109108,48.5));
#83229=CARTESIAN_POINT('',(79.449249625206,3.53171893954277,48.35));
#83230=CARTESIAN_POINT('',(79.449249625206,3.53171893954277,48.5));
#83231=CARTESIAN_POINT('Ctrl Pts',(79.449249625206,3.53171893954277,48.35));
#83232=CARTESIAN_POINT('Ctrl Pts',(79.6008185744286,3.45443391799927,48.35));
#83233=CARTESIAN_POINT('Ctrl Pts',(79.6811048388481,3.32087317109108,48.35));
#83234=CARTESIAN_POINT('Ctrl Pts',(79.1175989508629,3.60900411009789,48.5));
#83235=CARTESIAN_POINT('Ctrl Pts',(79.1175989508629,3.60900411009789,48.35));
#83236=CARTESIAN_POINT('Ctrl Pts',(79.2976806759834,3.60900411009789,48.5));
#83237=CARTESIAN_POINT('Ctrl Pts',(79.2976806759834,3.60900411009789,48.35));
#83238=CARTESIAN_POINT('Ctrl Pts',(79.449249625206,3.53171893954277,48.5));
#83239=CARTESIAN_POINT('Ctrl Pts',(79.449249625206,3.53171893954277,48.35));
#83240=CARTESIAN_POINT('',(79.1175989508629,3.60900411009789,48.5));
#83241=CARTESIAN_POINT('Ctrl Pts',(79.1175989508629,3.60900411009789,48.5));
#83242=CARTESIAN_POINT('Ctrl Pts',(79.2976806759834,3.60900411009789,48.5));
#83243=CARTESIAN_POINT('Ctrl Pts',(79.449249625206,3.53171893954277,48.5));
#83244=CARTESIAN_POINT('',(79.1175989508629,3.60900411009789,48.35));
#83245=CARTESIAN_POINT('',(79.1175989508629,3.60900411009789,48.5));
#83246=CARTESIAN_POINT('Ctrl Pts',(79.1175989508629,3.60900411009789,48.35));
#83247=CARTESIAN_POINT('Ctrl Pts',(79.2976806759834,3.60900411009789,48.35));
#83248=CARTESIAN_POINT('Ctrl Pts',(79.449249625206,3.53171893954277,48.35));
#83249=CARTESIAN_POINT('Ctrl Pts',(78.6809004545212,3.45968627929688,48.5));
#83250=CARTESIAN_POINT('Ctrl Pts',(78.6809004545212,3.45968627929688,48.35));
#83251=CARTESIAN_POINT('Ctrl Pts',(78.8564802408218,3.60900411009789,48.5));
#83252=CARTESIAN_POINT('Ctrl Pts',(78.8564802408218,3.60900411009789,48.35));
#83253=CARTESIAN_POINT('Ctrl Pts',(79.1175989508629,3.60900411009789,48.5));
#83254=CARTESIAN_POINT('Ctrl Pts',(79.1175989508629,3.60900411009789,48.35));
#83255=CARTESIAN_POINT('',(78.6809004545212,3.45968627929688,48.5));
#83256=CARTESIAN_POINT('Ctrl Pts',(78.6809004545212,3.45968627929688,48.5));
#83257=CARTESIAN_POINT('Ctrl Pts',(78.8564802408218,3.60900411009789,48.5));
#83258=CARTESIAN_POINT('Ctrl Pts',(79.1175989508629,3.60900411009789,48.5));
#83259=CARTESIAN_POINT('',(78.6809004545212,3.45968627929688,48.35));
#83260=CARTESIAN_POINT('',(78.6809004545212,3.45968627929688,48.5));
#83261=CARTESIAN_POINT('Ctrl Pts',(78.6809004545212,3.45968627929688,48.35));
#83262=CARTESIAN_POINT('Ctrl Pts',(78.8564802408218,3.60900411009789,48.35));
#83263=CARTESIAN_POINT('Ctrl Pts',(79.1175989508629,3.60900411009789,48.35));
#83264=CARTESIAN_POINT('Ctrl Pts',(78.4557980000973,3.03874486684799,48.5));
#83265=CARTESIAN_POINT('Ctrl Pts',(78.4557980000973,3.03874486684799,48.35));
#83266=CARTESIAN_POINT('Ctrl Pts',(78.5053205192089,3.31036829948425,48.5));
#83267=CARTESIAN_POINT('Ctrl Pts',(78.5053205192089,3.31036829948425,48.35));
#83268=CARTESIAN_POINT('Ctrl Pts',(78.6809004545212,3.45968627929688,48.5));
#83269=CARTESIAN_POINT('Ctrl Pts',(78.6809004545212,3.45968627929688,48.35));
#83270=CARTESIAN_POINT('',(78.4557980000973,3.03874486684799,48.5));
#83271=CARTESIAN_POINT('Ctrl Pts',(78.4557980000973,3.03874486684799,48.5));
#83272=CARTESIAN_POINT('Ctrl Pts',(78.5053205192089,3.31036829948425,48.5));
#83273=CARTESIAN_POINT('Ctrl Pts',(78.6809004545212,3.45968627929688,48.5));
#83274=CARTESIAN_POINT('',(78.4557980000973,3.03874486684799,48.35));
#83275=CARTESIAN_POINT('',(78.4557980000973,3.03874486684799,48.5));
#83276=CARTESIAN_POINT('Ctrl Pts',(78.4557980000973,3.03874486684799,48.35));
#83277=CARTESIAN_POINT('Ctrl Pts',(78.5053205192089,3.31036829948425,48.35));
#83278=CARTESIAN_POINT('Ctrl Pts',(78.6809004545212,3.45968627929688,48.35));
#83279=CARTESIAN_POINT('Origin',(78.7259207367897,2.99072304368019,48.5));
#83280=CARTESIAN_POINT('',(78.7259207367897,2.99072304368019,48.5));
#83281=CARTESIAN_POINT('',(40.1372829580836,9.85092578849893,48.5));
#83282=CARTESIAN_POINT('',(78.7259207367897,2.99072304368019,48.35));
#83283=CARTESIAN_POINT('',(78.7259207367897,2.99072304368019,48.5));
#83284=CARTESIAN_POINT('',(78.7259207367897,2.99072304368019,48.35));
#83285=CARTESIAN_POINT('Ctrl Pts',(78.8609821796417,3.28785815834999,48.5));
#83286=CARTESIAN_POINT('Ctrl Pts',(78.8609821796417,3.28785815834999,48.35));
#83287=CARTESIAN_POINT('Ctrl Pts',(78.7559345066547,3.18881312012672,48.5));
#83288=CARTESIAN_POINT('Ctrl Pts',(78.7559345066547,3.18881312012672,48.35));
#83289=CARTESIAN_POINT('Ctrl Pts',(78.7259207367897,2.99072304368019,48.5));
#83290=CARTESIAN_POINT('Ctrl Pts',(78.7259207367897,2.99072304368019,48.35));
#83291=CARTESIAN_POINT('',(78.8609821796417,3.28785815834999,48.5));
#83292=CARTESIAN_POINT('Ctrl Pts',(78.8609821796417,3.28785815834999,48.5));
#83293=CARTESIAN_POINT('Ctrl Pts',(78.7559345066547,3.18881312012672,48.5));
#83294=CARTESIAN_POINT('Ctrl Pts',(78.7259207367897,2.99072304368019,48.5));
#83295=CARTESIAN_POINT('',(78.8609821796417,3.28785815834999,48.35));
#83296=CARTESIAN_POINT('',(78.8609821796417,3.28785815834999,48.5));
#83297=CARTESIAN_POINT('Ctrl Pts',(78.8609821796417,3.28785815834999,48.35));
#83298=CARTESIAN_POINT('Ctrl Pts',(78.7559345066547,3.18881312012672,48.35));
#83299=CARTESIAN_POINT('Ctrl Pts',(78.7259207367897,2.99072304368019,48.35));
#83300=CARTESIAN_POINT('Ctrl Pts',(79.1236015856266,3.38690319657326,48.5));
#83301=CARTESIAN_POINT('Ctrl Pts',(79.1236015856266,3.38690319657326,48.35));
#83302=CARTESIAN_POINT('Ctrl Pts',(78.9660300016403,3.38690319657326,48.5));
#83303=CARTESIAN_POINT('Ctrl Pts',(78.9660300016403,3.38690319657326,48.35));
#83304=CARTESIAN_POINT('Ctrl Pts',(78.8609821796417,3.28785815834999,48.5));
#83305=CARTESIAN_POINT('Ctrl Pts',(78.8609821796417,3.28785815834999,48.35));
#83306=CARTESIAN_POINT('',(79.1236015856266,3.38690319657326,48.5));
#83307=CARTESIAN_POINT('Ctrl Pts',(79.1236015856266,3.38690319657326,48.5));
#83308=CARTESIAN_POINT('Ctrl Pts',(78.9660300016403,3.38690319657326,48.5));
#83309=CARTESIAN_POINT('Ctrl Pts',(78.8609821796417,3.28785815834999,48.5));
#83310=CARTESIAN_POINT('',(79.1236015856266,3.38690319657326,48.35));
#83311=CARTESIAN_POINT('',(79.1236015856266,3.38690319657326,48.5));
#83312=CARTESIAN_POINT('Ctrl Pts',(79.1236015856266,3.38690319657326,48.35));
#83313=CARTESIAN_POINT('Ctrl Pts',(78.9660300016403,3.38690319657326,48.35));
#83314=CARTESIAN_POINT('Ctrl Pts',(78.8609821796417,3.28785815834999,48.35));
#83315=CARTESIAN_POINT('Ctrl Pts',(79.3832195997238,3.28935885429382,48.5));
#83316=CARTESIAN_POINT('Ctrl Pts',(79.3832195997238,3.28935885429382,48.35));
#83317=CARTESIAN_POINT('Ctrl Pts',(79.2826738655567,3.38690319657326,48.5));
#83318=CARTESIAN_POINT('Ctrl Pts',(79.2826738655567,3.38690319657326,48.35));
#83319=CARTESIAN_POINT('Ctrl Pts',(79.1236015856266,3.38690319657326,48.5));
#83320=CARTESIAN_POINT('Ctrl Pts',(79.1236015856266,3.38690319657326,48.35));
#83321=CARTESIAN_POINT('',(79.3832195997238,3.28935885429382,48.5));
#83322=CARTESIAN_POINT('Ctrl Pts',(79.3832195997238,3.28935885429382,48.5));
#83323=CARTESIAN_POINT('Ctrl Pts',(79.2826738655567,3.38690319657326,48.5));
#83324=CARTESIAN_POINT('Ctrl Pts',(79.1236015856266,3.38690319657326,48.5));
#83325=CARTESIAN_POINT('',(79.3832195997238,3.28935885429382,48.35));
#83326=CARTESIAN_POINT('',(79.3832195997238,3.28935885429382,48.5));
#83327=CARTESIAN_POINT('Ctrl Pts',(79.3832195997238,3.28935885429382,48.35));
#83328=CARTESIAN_POINT('Ctrl Pts',(79.2826738655567,3.38690319657326,48.35));
#83329=CARTESIAN_POINT('Ctrl Pts',(79.1236015856266,3.38690319657326,48.35));
#83330=CARTESIAN_POINT('Ctrl Pts',(79.4837651848793,3.04324695467949,48.5));
#83331=CARTESIAN_POINT('Ctrl Pts',(79.4837651848793,3.04324695467949,48.35));
#83332=CARTESIAN_POINT('Ctrl Pts',(79.4837651848793,3.19181451201439,48.5));
#83333=CARTESIAN_POINT('Ctrl Pts',(79.4837651848793,3.19181451201439,48.35));
#83334=CARTESIAN_POINT('Ctrl Pts',(79.3832195997238,3.28935885429382,48.5));
#83335=CARTESIAN_POINT('Ctrl Pts',(79.3832195997238,3.28935885429382,48.35));
#83336=CARTESIAN_POINT('',(79.4837651848793,3.04324695467949,48.5));
#83337=CARTESIAN_POINT('Ctrl Pts',(79.4837651848793,3.04324695467949,48.5));
#83338=CARTESIAN_POINT('Ctrl Pts',(79.4837651848793,3.19181451201439,48.5));
#83339=CARTESIAN_POINT('Ctrl Pts',(79.3832195997238,3.28935885429382,48.5));
#83340=CARTESIAN_POINT('',(79.4837651848793,3.04324695467949,48.35));
#83341=CARTESIAN_POINT('',(79.4837651848793,3.04324695467949,48.5));
#83342=CARTESIAN_POINT('Ctrl Pts',(79.4837651848793,3.04324695467949,48.35));
#83343=CARTESIAN_POINT('Ctrl Pts',(79.4837651848793,3.19181451201439,48.35));
#83344=CARTESIAN_POINT('Ctrl Pts',(79.3832195997238,3.28935885429382,48.35));
#83345=CARTESIAN_POINT('Ctrl Pts',(79.3457026481628,2.7656207382679,48.5));
#83346=CARTESIAN_POINT('Ctrl Pts',(79.3457026481628,2.7656207382679,48.35));
#83347=CARTESIAN_POINT('Ctrl Pts',(79.4837651848793,2.85566174983978,48.5));
#83348=CARTESIAN_POINT('Ctrl Pts',(79.4837651848793,2.85566174983978,48.35));
#83349=CARTESIAN_POINT('Ctrl Pts',(79.4837651848793,3.04324695467949,48.5));
#83350=CARTESIAN_POINT('Ctrl Pts',(79.4837651848793,3.04324695467949,48.35));
#83351=CARTESIAN_POINT('',(79.3457026481628,2.7656207382679,48.5));
#83352=CARTESIAN_POINT('Ctrl Pts',(79.3457026481628,2.7656207382679,48.5));
#83353=CARTESIAN_POINT('Ctrl Pts',(79.4837651848793,2.85566174983978,48.5));
#83354=CARTESIAN_POINT('Ctrl Pts',(79.4837651848793,3.04324695467949,48.5));
#83355=CARTESIAN_POINT('',(79.3457026481628,2.7656207382679,48.35));
#83356=CARTESIAN_POINT('',(79.3457026481628,2.7656207382679,48.5));
#83357=CARTESIAN_POINT('Ctrl Pts',(79.3457026481628,2.7656207382679,48.35));
#83358=CARTESIAN_POINT('Ctrl Pts',(79.4837651848793,2.85566174983978,48.35));
#83359=CARTESIAN_POINT('Ctrl Pts',(79.4837651848793,3.04324695467949,48.35));
#83360=CARTESIAN_POINT('Ctrl Pts',(79.0350614190102,2.67557987570763,48.5));
#83361=CARTESIAN_POINT('Ctrl Pts',(79.0350614190102,2.67557987570763,48.35));
#83362=CARTESIAN_POINT('Ctrl Pts',(79.2076398134232,2.67557987570763,48.5));
#83363=CARTESIAN_POINT('Ctrl Pts',(79.2076398134232,2.67557987570763,48.35));
#83364=CARTESIAN_POINT('Ctrl Pts',(79.3457026481628,2.7656207382679,48.5));
#83365=CARTESIAN_POINT('Ctrl Pts',(79.3457026481628,2.7656207382679,48.35));
#83366=CARTESIAN_POINT('',(79.0350614190102,2.67557987570763,48.5));
#83367=CARTESIAN_POINT('Ctrl Pts',(79.0350614190102,2.67557987570763,48.5));
#83368=CARTESIAN_POINT('Ctrl Pts',(79.2076398134232,2.67557987570763,48.5));
#83369=CARTESIAN_POINT('Ctrl Pts',(79.3457026481628,2.7656207382679,48.5));
#83370=CARTESIAN_POINT('',(79.0350614190102,2.67557987570763,48.35));
#83371=CARTESIAN_POINT('',(79.0350614190102,2.67557987570763,48.5));
#83372=CARTESIAN_POINT('Ctrl Pts',(79.0350614190102,2.67557987570763,48.35));
#83373=CARTESIAN_POINT('Ctrl Pts',(79.2076398134232,2.67557987570763,48.35));
#83374=CARTESIAN_POINT('Ctrl Pts',(79.3457026481628,2.7656207382679,48.35));
#83375=CARTESIAN_POINT('Ctrl Pts',(78.9915415346622,2.67858126759529,48.5));
#83376=CARTESIAN_POINT('Ctrl Pts',(78.9915415346622,2.67858126759529,48.35));
#83377=CARTESIAN_POINT('Ctrl Pts',(79.0185539126396,2.67557987570763,48.5));
#83378=CARTESIAN_POINT('Ctrl Pts',(79.0185539126396,2.67557987570763,48.35));
#83379=CARTESIAN_POINT('Ctrl Pts',(79.0350614190102,2.67557987570763,48.5));
#83380=CARTESIAN_POINT('Ctrl Pts',(79.0350614190102,2.67557987570763,48.35));
#83381=CARTESIAN_POINT('',(78.9915415346622,2.67858126759529,48.5));
#83382=CARTESIAN_POINT('Ctrl Pts',(78.9915415346622,2.67858126759529,48.5));
#83383=CARTESIAN_POINT('Ctrl Pts',(79.0185539126396,2.67557987570763,48.5));
#83384=CARTESIAN_POINT('Ctrl Pts',(79.0350614190102,2.67557987570763,48.5));
#83385=CARTESIAN_POINT('',(78.9915415346622,2.67858126759529,48.35));
#83386=CARTESIAN_POINT('',(78.9915415346622,2.67858126759529,48.5));
#83387=CARTESIAN_POINT('Ctrl Pts',(78.9915415346622,2.67858126759529,48.35));
#83388=CARTESIAN_POINT('Ctrl Pts',(79.0185539126396,2.67557987570763,48.35));
#83389=CARTESIAN_POINT('Ctrl Pts',(79.0350614190102,2.67557987570763,48.35));
#83390=CARTESIAN_POINT('Origin',(78.9615279138088,2.44147354364395,48.5));
#83391=CARTESIAN_POINT('',(78.9615279138088,2.44147354364395,48.5));
#83392=CARTESIAN_POINT('',(78.6851589487883,0.258157622288407,48.5));
#83393=CARTESIAN_POINT('',(78.9615279138088,2.44147354364395,48.35));
#83394=CARTESIAN_POINT('',(78.9615279138088,2.44147354364395,48.5));
#83395=CARTESIAN_POINT('',(78.9615279138088,2.44147354364395,48.35));
#83396=CARTESIAN_POINT('Ctrl Pts',(79.1521145105362,2.47148716449738,48.5));
#83397=CARTESIAN_POINT('Ctrl Pts',(79.1521145105362,2.47148716449738,48.35));
#83398=CARTESIAN_POINT('Ctrl Pts',(79.0755797624588,2.47148716449738,48.5));
#83399=CARTESIAN_POINT('Ctrl Pts',(79.0755797624588,2.47148716449738,48.35));
#83400=CARTESIAN_POINT('Ctrl Pts',(78.9615279138088,2.44147354364395,48.5));
#83401=CARTESIAN_POINT('Ctrl Pts',(78.9615279138088,2.44147354364395,48.35));
#83402=CARTESIAN_POINT('',(79.1521145105362,2.47148716449738,48.5));
#83403=CARTESIAN_POINT('Ctrl Pts',(79.1521145105362,2.47148716449738,48.5));
#83404=CARTESIAN_POINT('Ctrl Pts',(79.0755797624588,2.47148716449738,48.5));
#83405=CARTESIAN_POINT('Ctrl Pts',(78.9615279138088,2.44147354364395,48.5));
#83406=CARTESIAN_POINT('',(79.1521145105362,2.47148716449738,48.35));
#83407=CARTESIAN_POINT('',(79.1521145105362,2.47148716449738,48.5));
#83408=CARTESIAN_POINT('Ctrl Pts',(79.1521145105362,2.47148716449738,48.35));
#83409=CARTESIAN_POINT('Ctrl Pts',(79.0755797624588,2.47148716449738,48.35));
#83410=CARTESIAN_POINT('Ctrl Pts',(78.9615279138088,2.44147354364395,48.35));
#83411=CARTESIAN_POINT('Ctrl Pts',(79.4612548947334,2.35068225860596,48.5));
#83412=CARTESIAN_POINT('Ctrl Pts',(79.4612548947334,2.35068225860596,48.35));
#83413=CARTESIAN_POINT('Ctrl Pts',(79.3396998643875,2.47148716449738,48.5));
#83414=CARTESIAN_POINT('Ctrl Pts',(79.3396998643875,2.47148716449738,48.35));
#83415=CARTESIAN_POINT('Ctrl Pts',(79.1521145105362,2.47148716449738,48.5));
#83416=CARTESIAN_POINT('Ctrl Pts',(79.1521145105362,2.47148716449738,48.35));
#83417=CARTESIAN_POINT('',(79.4612548947334,2.35068225860596,48.5));
#83418=CARTESIAN_POINT('Ctrl Pts',(79.4612548947334,2.35068225860596,48.5));
#83419=CARTESIAN_POINT('Ctrl Pts',(79.3396998643875,2.47148716449738,48.5));
#83420=CARTESIAN_POINT('Ctrl Pts',(79.1521145105362,2.47148716449738,48.5));
#83421=CARTESIAN_POINT('',(79.4612548947334,2.35068225860596,48.35));
#83422=CARTESIAN_POINT('',(79.4612548947334,2.35068225860596,48.5));
#83423=CARTESIAN_POINT('Ctrl Pts',(79.4612548947334,2.35068225860596,48.35));
#83424=CARTESIAN_POINT('Ctrl Pts',(79.3396998643875,2.47148716449738,48.35));
#83425=CARTESIAN_POINT('Ctrl Pts',(79.1521145105362,2.47148716449738,48.35));
#83426=CARTESIAN_POINT('Ctrl Pts',(79.5828102231026,2.04379284381866,48.5));
#83427=CARTESIAN_POINT('Ctrl Pts',(79.5828102231026,2.04379284381866,48.35));
#83428=CARTESIAN_POINT('Ctrl Pts',(79.5828102231026,2.22987735271454,48.5));
#83429=CARTESIAN_POINT('Ctrl Pts',(79.5828102231026,2.22987735271454,48.35));
#83430=CARTESIAN_POINT('Ctrl Pts',(79.4612548947334,2.35068225860596,48.5));
#83431=CARTESIAN_POINT('Ctrl Pts',(79.4612548947334,2.35068225860596,48.35));
#83432=CARTESIAN_POINT('',(79.5828102231026,2.04379284381866,48.5));
#83433=CARTESIAN_POINT('Ctrl Pts',(79.5828102231026,2.04379284381866,48.5));
#83434=CARTESIAN_POINT('Ctrl Pts',(79.5828102231026,2.22987735271454,48.5));
#83435=CARTESIAN_POINT('Ctrl Pts',(79.4612548947334,2.35068225860596,48.5));
#83436=CARTESIAN_POINT('',(79.5828102231026,2.04379284381866,48.35));
#83437=CARTESIAN_POINT('',(79.5828102231026,2.04379284381866,48.5));
#83438=CARTESIAN_POINT('Ctrl Pts',(79.5828102231026,2.04379284381866,48.35));
#83439=CARTESIAN_POINT('Ctrl Pts',(79.5828102231026,2.22987735271454,48.35));
#83440=CARTESIAN_POINT('Ctrl Pts',(79.4612548947334,2.35068225860596,48.35));
#83441=CARTESIAN_POINT('Ctrl Pts',(79.4515005946159,1.71664410829544,48.5));
#83442=CARTESIAN_POINT('Ctrl Pts',(79.4515005946159,1.71664410829544,48.35));
#83443=CARTESIAN_POINT('Ctrl Pts',(79.5828102231026,1.8487041592598,48.5));
#83444=CARTESIAN_POINT('Ctrl Pts',(79.5828102231026,1.8487041592598,48.35));
#83445=CARTESIAN_POINT('Ctrl Pts',(79.5828102231026,2.04379284381866,48.5));
#83446=CARTESIAN_POINT('Ctrl Pts',(79.5828102231026,2.04379284381866,48.35));
#83447=CARTESIAN_POINT('',(79.4515005946159,1.71664410829544,48.5));
#83448=CARTESIAN_POINT('Ctrl Pts',(79.4515005946159,1.71664410829544,48.5));
#83449=CARTESIAN_POINT('Ctrl Pts',(79.5828102231026,1.8487041592598,48.5));
#83450=CARTESIAN_POINT('Ctrl Pts',(79.5828102231026,2.04379284381866,48.5));
#83451=CARTESIAN_POINT('',(79.4515005946159,1.71664410829544,48.35));
#83452=CARTESIAN_POINT('',(79.4515005946159,1.71664410829544,48.5));
#83453=CARTESIAN_POINT('Ctrl Pts',(79.4515005946159,1.71664410829544,48.35));
#83454=CARTESIAN_POINT('Ctrl Pts',(79.5828102231026,1.8487041592598,48.35));
#83455=CARTESIAN_POINT('Ctrl Pts',(79.5828102231026,2.04379284381866,48.35));
#83456=CARTESIAN_POINT('Ctrl Pts',(79.1296042203903,1.58458405733109,48.5));
#83457=CARTESIAN_POINT('Ctrl Pts',(79.1296042203903,1.58458405733109,48.35));
#83458=CARTESIAN_POINT('Ctrl Pts',(79.3201909661293,1.58458405733109,48.5));
#83459=CARTESIAN_POINT('Ctrl Pts',(79.3201909661293,1.58458405733109,48.35));
#83460=CARTESIAN_POINT('Ctrl Pts',(79.4515005946159,1.71664410829544,48.5));
#83461=CARTESIAN_POINT('Ctrl Pts',(79.4515005946159,1.71664410829544,48.35));
#83462=CARTESIAN_POINT('',(79.1296042203903,1.58458405733109,48.5));
#83463=CARTESIAN_POINT('Ctrl Pts',(79.1296042203903,1.58458405733109,48.5));
#83464=CARTESIAN_POINT('Ctrl Pts',(79.3201909661293,1.58458405733109,48.5));
#83465=CARTESIAN_POINT('Ctrl Pts',(79.4515005946159,1.71664410829544,48.5));
#83466=CARTESIAN_POINT('',(79.1296042203903,1.58458405733109,48.35));
#83467=CARTESIAN_POINT('',(79.1296042203903,1.58458405733109,48.5));
#83468=CARTESIAN_POINT('Ctrl Pts',(79.1296042203903,1.58458405733109,48.35));
#83469=CARTESIAN_POINT('Ctrl Pts',(79.3201909661293,1.58458405733109,48.35));
#83470=CARTESIAN_POINT('Ctrl Pts',(79.4515005946159,1.71664410829544,48.35));
#83471=CARTESIAN_POINT('Ctrl Pts',(78.8572305142879,1.68588006496429,48.5));
#83472=CARTESIAN_POINT('Ctrl Pts',(78.8572305142879,1.68588006496429,48.35));
#83473=CARTESIAN_POINT('Ctrl Pts',(78.969031393528,1.58458405733109,48.5));
#83474=CARTESIAN_POINT('Ctrl Pts',(78.969031393528,1.58458405733109,48.35));
#83475=CARTESIAN_POINT('Ctrl Pts',(79.1296042203903,1.58458405733109,48.5));
#83476=CARTESIAN_POINT('Ctrl Pts',(79.1296042203903,1.58458405733109,48.35));
#83477=CARTESIAN_POINT('',(78.8572305142879,1.68588006496429,48.5));
#83478=CARTESIAN_POINT('Ctrl Pts',(78.8572305142879,1.68588006496429,48.5));
#83479=CARTESIAN_POINT('Ctrl Pts',(78.969031393528,1.58458405733109,48.5));
#83480=CARTESIAN_POINT('Ctrl Pts',(79.1296042203903,1.58458405733109,48.5));
#83481=CARTESIAN_POINT('',(78.8572305142879,1.68588006496429,48.35));
#83482=CARTESIAN_POINT('',(78.8572305142879,1.68588006496429,48.5));
#83483=CARTESIAN_POINT('Ctrl Pts',(78.8572305142879,1.68588006496429,48.35));
#83484=CARTESIAN_POINT('Ctrl Pts',(78.969031393528,1.58458405733109,48.35));
#83485=CARTESIAN_POINT('Ctrl Pts',(79.1296042203903,1.58458405733109,48.35));
#83486=CARTESIAN_POINT('Ctrl Pts',(78.6989085078239,2.01678061485291,48.5));
#83487=CARTESIAN_POINT('Ctrl Pts',(78.6989085078239,2.01678061485291,48.35));
#83488=CARTESIAN_POINT('Ctrl Pts',(78.7454296350479,1.7871760725975,48.5));
#83489=CARTESIAN_POINT('Ctrl Pts',(78.7454296350479,1.7871760725975,48.35));
#83490=CARTESIAN_POINT('Ctrl Pts',(78.8572305142879,1.68588006496429,48.5));
#83491=CARTESIAN_POINT('Ctrl Pts',(78.8572305142879,1.68588006496429,48.35));
#83492=CARTESIAN_POINT('',(78.6989085078239,2.01678061485291,48.5));
#83493=CARTESIAN_POINT('Ctrl Pts',(78.6989085078239,2.01678061485291,48.5));
#83494=CARTESIAN_POINT('Ctrl Pts',(78.7454296350479,1.7871760725975,48.5));
#83495=CARTESIAN_POINT('Ctrl Pts',(78.8572305142879,1.68588006496429,48.5));
#83496=CARTESIAN_POINT('',(78.6989085078239,2.01678061485291,48.35));
#83497=CARTESIAN_POINT('',(78.6989085078239,2.01678061485291,48.5));
#83498=CARTESIAN_POINT('Ctrl Pts',(78.6989085078239,2.01678061485291,48.35));
#83499=CARTESIAN_POINT('Ctrl Pts',(78.7454296350479,1.7871760725975,48.35));
#83500=CARTESIAN_POINT('Ctrl Pts',(78.8572305142879,1.68588006496429,48.35));
#83501=CARTESIAN_POINT('Origin',(78.4287857711315,1.98076421022415,48.5));
#83502=CARTESIAN_POINT('',(78.4287857711315,1.98076421022415,48.5));
#83503=CARTESIAN_POINT('',(40.2936354383861,-3.10392811068335,48.5));
#83504=CARTESIAN_POINT('',(78.4287857711315,1.98076421022415,48.35));
#83505=CARTESIAN_POINT('',(78.4287857711315,1.98076421022415,48.5));
#83506=CARTESIAN_POINT('',(78.4287857711315,1.98076421022415,48.35));
#83507=CARTESIAN_POINT('Ctrl Pts',(78.6471350193024,1.53356069326401,48.5));
#83508=CARTESIAN_POINT('Ctrl Pts',(78.6471350193024,1.53356069326401,48.35));
#83509=CARTESIAN_POINT('Ctrl Pts',(78.4557980000973,1.70613938570023,48.5));
#83510=CARTESIAN_POINT('Ctrl Pts',(78.4557980000973,1.70613938570023,48.35));
#83511=CARTESIAN_POINT('Ctrl Pts',(78.4287857711315,1.98076421022415,48.5));
#83512=CARTESIAN_POINT('Ctrl Pts',(78.4287857711315,1.98076421022415,48.35));
#83513=CARTESIAN_POINT('Ctrl Pts',(78.6471350193024,1.53356069326401,48.5));
#83514=CARTESIAN_POINT('Ctrl Pts',(78.4557980000973,1.70613938570023,48.5));
#83515=CARTESIAN_POINT('Ctrl Pts',(78.4287857711315,1.98076421022415,48.5));
#83516=CARTESIAN_POINT('Ctrl Pts',(78.6471350193024,1.53356069326401,48.35));
#83517=CARTESIAN_POINT('Ctrl Pts',(78.4557980000973,1.70613938570023,48.35));
#83518=CARTESIAN_POINT('Ctrl Pts',(78.4287857711315,1.98076421022415,48.35));
#83519=CARTESIAN_POINT('Origin',(79.9999998956919,2.48499320447445,48.35));
#83520=CARTESIAN_POINT('Origin',(0.,8.,48.5));
#83521=CARTESIAN_POINT('Ctrl Pts',(70.8959074625745,3.38540250062943,48.5));
#83522=CARTESIAN_POINT('Ctrl Pts',(70.8959074625745,3.38540250062943,48.35));
#83523=CARTESIAN_POINT('Ctrl Pts',(70.7098226556554,3.38540250062943,48.5));
#83524=CARTESIAN_POINT('Ctrl Pts',(70.7098226556554,3.38540250062943,48.35));
#83525=CARTESIAN_POINT('Ctrl Pts',(70.5987723479047,3.22783091664314,48.5));
#83526=CARTESIAN_POINT('Ctrl Pts',(70.5987723479047,3.22783091664314,48.35));
#83527=CARTESIAN_POINT('',(70.8959074625745,3.38540250062943,48.5));
#83528=CARTESIAN_POINT('',(70.5987723479047,3.22783091664314,48.5));
#83529=CARTESIAN_POINT('Ctrl Pts',(70.8959074625745,3.38540250062943,48.5));
#83530=CARTESIAN_POINT('Ctrl Pts',(70.7098226556554,3.38540250062943,48.5));
#83531=CARTESIAN_POINT('Ctrl Pts',(70.5987723479047,3.22783091664314,48.5));
#83532=CARTESIAN_POINT('',(70.8959074625745,3.38540250062943,48.35));
#83533=CARTESIAN_POINT('',(70.8959074625745,3.38540250062943,48.5));
#83534=CARTESIAN_POINT('',(70.5987723479047,3.22783091664314,48.35));
#83535=CARTESIAN_POINT('Ctrl Pts',(70.8959074625745,3.38540250062943,48.35));
#83536=CARTESIAN_POINT('Ctrl Pts',(70.7098226556554,3.38540250062943,48.35));
#83537=CARTESIAN_POINT('Ctrl Pts',(70.5987723479047,3.22783091664314,48.35));
#83538=CARTESIAN_POINT('',(70.5987723479047,3.22783091664314,48.5));
#83539=CARTESIAN_POINT('Ctrl Pts',(71.2118007550016,3.2068213224411,48.5));
#83540=CARTESIAN_POINT('Ctrl Pts',(71.2118007550016,3.2068213224411,48.35));
#83541=CARTESIAN_POINT('Ctrl Pts',(71.0849930653349,3.38540250062943,48.5));
#83542=CARTESIAN_POINT('Ctrl Pts',(71.0849930653349,3.38540250062943,48.35));
#83543=CARTESIAN_POINT('Ctrl Pts',(70.8959074625745,3.38540250062943,48.5));
#83544=CARTESIAN_POINT('Ctrl Pts',(70.8959074625745,3.38540250062943,48.35));
#83545=CARTESIAN_POINT('',(71.2118007550016,3.2068213224411,48.5));
#83546=CARTESIAN_POINT('Ctrl Pts',(71.2118007550016,3.2068213224411,48.5));
#83547=CARTESIAN_POINT('Ctrl Pts',(71.0849930653349,3.38540250062943,48.5));
#83548=CARTESIAN_POINT('Ctrl Pts',(70.8959074625745,3.38540250062943,48.5));
#83549=CARTESIAN_POINT('',(71.2118007550016,3.2068213224411,48.35));
#83550=CARTESIAN_POINT('',(71.2118007550016,3.2068213224411,48.5));
#83551=CARTESIAN_POINT('Ctrl Pts',(71.2118007550016,3.2068213224411,48.35));
#83552=CARTESIAN_POINT('Ctrl Pts',(71.0849930653349,3.38540250062943,48.35));
#83553=CARTESIAN_POINT('Ctrl Pts',(70.8959074625745,3.38540250062943,48.35));
#83554=CARTESIAN_POINT('Ctrl Pts',(71.3386084446684,2.48499327898026,48.5));
#83555=CARTESIAN_POINT('Ctrl Pts',(71.3386084446684,2.48499327898026,48.35));
#83556=CARTESIAN_POINT('Ctrl Pts',(71.3386084446684,3.02824014425278,48.5));
#83557=CARTESIAN_POINT('Ctrl Pts',(71.3386084446684,3.02824014425278,48.35));
#83558=CARTESIAN_POINT('Ctrl Pts',(71.2118007550016,3.2068213224411,48.5));
#83559=CARTESIAN_POINT('Ctrl Pts',(71.2118007550016,3.2068213224411,48.35));
#83560=CARTESIAN_POINT('',(71.3386084446684,2.48499327898026,48.5));
#83561=CARTESIAN_POINT('Ctrl Pts',(71.3386084446684,2.48499327898026,48.5));
#83562=CARTESIAN_POINT('Ctrl Pts',(71.3386084446684,3.02824014425278,48.5));
#83563=CARTESIAN_POINT('Ctrl Pts',(71.2118007550016,3.2068213224411,48.5));
#83564=CARTESIAN_POINT('',(71.3386084446684,2.48499327898026,48.35));
#83565=CARTESIAN_POINT('',(71.3386084446684,2.48499327898026,48.5));
#83566=CARTESIAN_POINT('Ctrl Pts',(71.3386084446684,2.48499327898026,48.35));
#83567=CARTESIAN_POINT('Ctrl Pts',(71.3386084446684,3.02824014425278,48.35));
#83568=CARTESIAN_POINT('Ctrl Pts',(71.2118007550016,3.2068213224411,48.35));
#83569=CARTESIAN_POINT('Ctrl Pts',(71.2118007550016,1.76466578245163,48.5));
#83570=CARTESIAN_POINT('Ctrl Pts',(71.2118007550016,1.76466578245163,48.35));
#83571=CARTESIAN_POINT('Ctrl Pts',(71.3386084446684,1.9447478055954,48.5));
#83572=CARTESIAN_POINT('Ctrl Pts',(71.3386084446684,1.9447478055954,48.35));
#83573=CARTESIAN_POINT('Ctrl Pts',(71.3386084446684,2.48499327898026,48.5));
#83574=CARTESIAN_POINT('Ctrl Pts',(71.3386084446684,2.48499327898026,48.35));
#83575=CARTESIAN_POINT('',(71.2118007550016,1.76466578245163,48.5));
#83576=CARTESIAN_POINT('Ctrl Pts',(71.2118007550016,1.76466578245163,48.5));
#83577=CARTESIAN_POINT('Ctrl Pts',(71.3386084446684,1.9447478055954,48.5));
#83578=CARTESIAN_POINT('Ctrl Pts',(71.3386084446684,2.48499327898026,48.5));
#83579=CARTESIAN_POINT('',(71.2118007550016,1.76466578245163,48.35));
#83580=CARTESIAN_POINT('',(71.2118007550016,1.76466578245163,48.5));
#83581=CARTESIAN_POINT('Ctrl Pts',(71.2118007550016,1.76466578245163,48.35));
#83582=CARTESIAN_POINT('Ctrl Pts',(71.3386084446684,1.9447478055954,48.35));
#83583=CARTESIAN_POINT('Ctrl Pts',(71.3386084446684,2.48499327898026,48.35));
#83584=CARTESIAN_POINT('Ctrl Pts',(70.898908556439,1.58458405733109,48.5));
#83585=CARTESIAN_POINT('Ctrl Pts',(70.898908556439,1.58458405733109,48.35));
#83586=CARTESIAN_POINT('Ctrl Pts',(71.0849930653349,1.58458405733109,48.5));
#83587=CARTESIAN_POINT('Ctrl Pts',(71.0849930653349,1.58458405733109,48.35));
#83588=CARTESIAN_POINT('Ctrl Pts',(71.2118007550016,1.76466578245163,48.5));
#83589=CARTESIAN_POINT('Ctrl Pts',(71.2118007550016,1.76466578245163,48.35));
#83590=CARTESIAN_POINT('',(70.898908556439,1.58458405733109,48.5));
#83591=CARTESIAN_POINT('Ctrl Pts',(70.898908556439,1.58458405733109,48.5));
#83592=CARTESIAN_POINT('Ctrl Pts',(71.0849930653349,1.58458405733109,48.5));
#83593=CARTESIAN_POINT('Ctrl Pts',(71.2118007550016,1.76466578245163,48.5));
#83594=CARTESIAN_POINT('',(70.898908556439,1.58458405733109,48.35));
#83595=CARTESIAN_POINT('',(70.898908556439,1.58458405733109,48.5));
#83596=CARTESIAN_POINT('Ctrl Pts',(70.898908556439,1.58458405733109,48.35));
#83597=CARTESIAN_POINT('Ctrl Pts',(71.0849930653349,1.58458405733109,48.35));
#83598=CARTESIAN_POINT('Ctrl Pts',(71.2118007550016,1.76466578245163,48.35));
#83599=CARTESIAN_POINT('Ctrl Pts',(70.5860163578764,1.76391565799713,48.5));
#83600=CARTESIAN_POINT('Ctrl Pts',(70.5860163578764,1.76391565799713,48.35));
#83601=CARTESIAN_POINT('Ctrl Pts',(70.7128240475431,1.58458405733109,48.5));
#83602=CARTESIAN_POINT('Ctrl Pts',(70.7128240475431,1.58458405733109,48.35));
#83603=CARTESIAN_POINT('Ctrl Pts',(70.898908556439,1.58458405733109,48.5));
#83604=CARTESIAN_POINT('Ctrl Pts',(70.898908556439,1.58458405733109,48.35));
#83605=CARTESIAN_POINT('',(70.5860163578764,1.76391565799713,48.5));
#83606=CARTESIAN_POINT('Ctrl Pts',(70.5860163578764,1.76391565799713,48.5));
#83607=CARTESIAN_POINT('Ctrl Pts',(70.7128240475431,1.58458405733109,48.5));
#83608=CARTESIAN_POINT('Ctrl Pts',(70.898908556439,1.58458405733109,48.5));
#83609=CARTESIAN_POINT('',(70.5860163578764,1.76391565799713,48.35));
#83610=CARTESIAN_POINT('',(70.5860163578764,1.76391565799713,48.5));
#83611=CARTESIAN_POINT('Ctrl Pts',(70.5860163578764,1.76391565799713,48.35));
#83612=CARTESIAN_POINT('Ctrl Pts',(70.7128240475431,1.58458405733109,48.35));
#83613=CARTESIAN_POINT('Ctrl Pts',(70.898908556439,1.58458405733109,48.35));
#83614=CARTESIAN_POINT('Ctrl Pts',(70.4592086682096,2.48499327898026,48.5));
#83615=CARTESIAN_POINT('Ctrl Pts',(70.4592086682096,2.48499327898026,48.35));
#83616=CARTESIAN_POINT('Ctrl Pts',(70.4592086682096,1.94324696063995,48.5));
#83617=CARTESIAN_POINT('Ctrl Pts',(70.4592086682096,1.94324696063995,48.35));
#83618=CARTESIAN_POINT('Ctrl Pts',(70.5860163578764,1.76391565799713,48.5));
#83619=CARTESIAN_POINT('Ctrl Pts',(70.5860163578764,1.76391565799713,48.35));
#83620=CARTESIAN_POINT('',(70.4592086682096,2.48499327898026,48.5));
#83621=CARTESIAN_POINT('Ctrl Pts',(70.4592086682096,2.48499327898026,48.5));
#83622=CARTESIAN_POINT('Ctrl Pts',(70.4592086682096,1.94324696063995,48.5));
#83623=CARTESIAN_POINT('Ctrl Pts',(70.5860163578764,1.76391565799713,48.5));
#83624=CARTESIAN_POINT('',(70.4592086682096,2.48499327898026,48.35));
#83625=CARTESIAN_POINT('',(70.4592086682096,2.48499327898026,48.5));
#83626=CARTESIAN_POINT('Ctrl Pts',(70.4592086682096,2.48499327898026,48.35));
#83627=CARTESIAN_POINT('Ctrl Pts',(70.4592086682096,1.94324696063995,48.35));
#83628=CARTESIAN_POINT('Ctrl Pts',(70.5860163578764,1.76391565799713,48.35));
#83629=CARTESIAN_POINT('Ctrl Pts',(70.5987723479047,3.22783091664314,48.5));
#83630=CARTESIAN_POINT('Ctrl Pts',(70.5987723479047,3.22783091664314,48.35));
#83631=CARTESIAN_POINT('Ctrl Pts',(70.4592086682096,3.02673944830894,48.5));
#83632=CARTESIAN_POINT('Ctrl Pts',(70.4592086682096,3.02673944830894,48.35));
#83633=CARTESIAN_POINT('Ctrl Pts',(70.4592086682096,2.48499327898026,48.5));
#83634=CARTESIAN_POINT('Ctrl Pts',(70.4592086682096,2.48499327898026,48.35));
#83635=CARTESIAN_POINT('Ctrl Pts',(70.5987723479047,3.22783091664314,48.5));
#83636=CARTESIAN_POINT('Ctrl Pts',(70.4592086682096,3.02673944830894,48.5));
#83637=CARTESIAN_POINT('Ctrl Pts',(70.4592086682096,2.48499327898026,48.5));
#83638=CARTESIAN_POINT('Ctrl Pts',(70.5987723479047,3.22783091664314,48.35));
#83639=CARTESIAN_POINT('Ctrl Pts',(70.4592086682096,3.02673944830894,48.35));
#83640=CARTESIAN_POINT('Ctrl Pts',(70.4592086682096,2.48499327898026,48.35));
#83641=CARTESIAN_POINT('Ctrl Pts',(70.898908556439,1.36248314380646,48.5));
#83642=CARTESIAN_POINT('Ctrl Pts',(70.898908556439,1.36248314380646,48.35));
#83643=CARTESIAN_POINT('Ctrl Pts',(70.5807639965788,1.36248314380646,48.5));
#83644=CARTESIAN_POINT('Ctrl Pts',(70.5807639965788,1.36248314380646,48.35));
#83645=CARTESIAN_POINT('Ctrl Pts',(70.3991814265028,1.59058684110642,48.5));
#83646=CARTESIAN_POINT('Ctrl Pts',(70.3991814265028,1.59058684110642,48.35));
#83647=CARTESIAN_POINT('',(70.898908556439,1.36248314380646,48.5));
#83648=CARTESIAN_POINT('',(70.3991814265028,1.59058684110642,48.5));
#83649=CARTESIAN_POINT('Ctrl Pts',(70.898908556439,1.36248314380646,48.5));
#83650=CARTESIAN_POINT('Ctrl Pts',(70.5807639965788,1.36248314380646,48.5));
#83651=CARTESIAN_POINT('Ctrl Pts',(70.3991814265028,1.59058684110642,48.5));
#83652=CARTESIAN_POINT('',(70.898908556439,1.36248314380646,48.35));
#83653=CARTESIAN_POINT('',(70.898908556439,1.36248314380646,48.5));
#83654=CARTESIAN_POINT('',(70.3991814265028,1.59058684110642,48.35));
#83655=CARTESIAN_POINT('Ctrl Pts',(70.898908556439,1.36248314380646,48.35));
#83656=CARTESIAN_POINT('Ctrl Pts',(70.5807639965788,1.36248314380646,48.35));
#83657=CARTESIAN_POINT('Ctrl Pts',(70.3991814265028,1.59058684110642,48.35));
#83658=CARTESIAN_POINT('',(70.3991814265028,1.59058684110642,48.5));
#83659=CARTESIAN_POINT('Ctrl Pts',(71.2988402256742,1.49229192733765,48.5));
#83660=CARTESIAN_POINT('Ctrl Pts',(71.2988402256742,1.49229192733765,48.35));
#83661=CARTESIAN_POINT('Ctrl Pts',(71.1405183682218,1.36248314380646,48.5));
#83662=CARTESIAN_POINT('Ctrl Pts',(71.1405183682218,1.36248314380646,48.35));
#83663=CARTESIAN_POINT('Ctrl Pts',(70.898908556439,1.36248314380646,48.5));
#83664=CARTESIAN_POINT('Ctrl Pts',(70.898908556439,1.36248314380646,48.35));
#83665=CARTESIAN_POINT('',(71.2988402256742,1.49229192733765,48.5));
#83666=CARTESIAN_POINT('Ctrl Pts',(71.2988402256742,1.49229192733765,48.5));
#83667=CARTESIAN_POINT('Ctrl Pts',(71.1405183682218,1.36248314380646,48.5));
#83668=CARTESIAN_POINT('Ctrl Pts',(70.898908556439,1.36248314380646,48.5));
#83669=CARTESIAN_POINT('',(71.2988402256742,1.49229192733765,48.35));
#83670=CARTESIAN_POINT('',(71.2988402256742,1.49229192733765,48.5));
#83671=CARTESIAN_POINT('Ctrl Pts',(71.2988402256742,1.49229192733765,48.35));
#83672=CARTESIAN_POINT('Ctrl Pts',(71.1405183682218,1.36248314380646,48.35));
#83673=CARTESIAN_POINT('Ctrl Pts',(70.898908556439,1.36248314380646,48.35));
#83674=CARTESIAN_POINT('Ctrl Pts',(71.5366985211149,1.85995900630951,48.5));
#83675=CARTESIAN_POINT('Ctrl Pts',(71.5366985211149,1.85995900630951,48.35));
#83676=CARTESIAN_POINT('Ctrl Pts',(71.4571620831266,1.62210100889206,48.5));
#83677=CARTESIAN_POINT('Ctrl Pts',(71.4571620831266,1.62210100889206,48.35));
#83678=CARTESIAN_POINT('Ctrl Pts',(71.2988402256742,1.49229192733765,48.5));
#83679=CARTESIAN_POINT('Ctrl Pts',(71.2988402256742,1.49229192733765,48.35));
#83680=CARTESIAN_POINT('',(71.5366985211149,1.85995900630951,48.5));
#83681=CARTESIAN_POINT('Ctrl Pts',(71.5366985211149,1.85995900630951,48.5));
#83682=CARTESIAN_POINT('Ctrl Pts',(71.4571620831266,1.62210100889206,48.5));
#83683=CARTESIAN_POINT('Ctrl Pts',(71.2988402256742,1.49229192733765,48.5));
#83684=CARTESIAN_POINT('',(71.5366985211149,1.85995900630951,48.35));
#83685=CARTESIAN_POINT('',(71.5366985211149,1.85995900630951,48.5));
#83686=CARTESIAN_POINT('Ctrl Pts',(71.5366985211149,1.85995900630951,48.35));
#83687=CARTESIAN_POINT('Ctrl Pts',(71.4571620831266,1.62210100889206,48.35));
#83688=CARTESIAN_POINT('Ctrl Pts',(71.2988402256742,1.49229192733765,48.35));
#83689=CARTESIAN_POINT('Ctrl Pts',(71.6162343630567,2.48499327898026,48.5));
#83690=CARTESIAN_POINT('Ctrl Pts',(71.6162343630567,2.48499327898026,48.35));
#83691=CARTESIAN_POINT('Ctrl Pts',(71.6162343630567,2.09781730175018,48.5));
#83692=CARTESIAN_POINT('Ctrl Pts',(71.6162343630567,2.09781730175018,48.35));
#83693=CARTESIAN_POINT('Ctrl Pts',(71.5366985211149,1.85995900630951,48.5));
#83694=CARTESIAN_POINT('Ctrl Pts',(71.5366985211149,1.85995900630951,48.35));
#83695=CARTESIAN_POINT('',(71.6162343630567,2.48499327898026,48.5));
#83696=CARTESIAN_POINT('Ctrl Pts',(71.6162343630567,2.48499327898026,48.5));
#83697=CARTESIAN_POINT('Ctrl Pts',(71.6162343630567,2.09781730175018,48.5));
#83698=CARTESIAN_POINT('Ctrl Pts',(71.5366985211149,1.85995900630951,48.5));
#83699=CARTESIAN_POINT('',(71.6162343630567,2.48499327898026,48.35));
#83700=CARTESIAN_POINT('',(71.6162343630567,2.48499327898026,48.5));
#83701=CARTESIAN_POINT('Ctrl Pts',(71.6162343630567,2.48499327898026,48.35));
#83702=CARTESIAN_POINT('Ctrl Pts',(71.6162343630567,2.09781730175018,48.35));
#83703=CARTESIAN_POINT('Ctrl Pts',(71.5366985211149,1.85995900630951,48.35));
#83704=CARTESIAN_POINT('Ctrl Pts',(71.5667118439451,3.00497958064079,48.5));
#83705=CARTESIAN_POINT('Ctrl Pts',(71.5667118439451,3.00497958064079,48.35));
#83706=CARTESIAN_POINT('Ctrl Pts',(71.6162343630567,2.81214186549187,48.5));
#83707=CARTESIAN_POINT('Ctrl Pts',(71.6162343630567,2.81214186549187,48.35));
#83708=CARTESIAN_POINT('Ctrl Pts',(71.6162343630567,2.48499327898026,48.5));
#83709=CARTESIAN_POINT('Ctrl Pts',(71.6162343630567,2.48499327898026,48.35));
#83710=CARTESIAN_POINT('',(71.5667118439451,3.00497958064079,48.5));
#83711=CARTESIAN_POINT('Ctrl Pts',(71.5667118439451,3.00497958064079,48.5));
#83712=CARTESIAN_POINT('Ctrl Pts',(71.6162343630567,2.81214186549187,48.5));
#83713=CARTESIAN_POINT('Ctrl Pts',(71.6162343630567,2.48499327898026,48.5));
#83714=CARTESIAN_POINT('',(71.5667118439451,3.00497958064079,48.35));
#83715=CARTESIAN_POINT('',(71.5667118439451,3.00497958064079,48.5));
#83716=CARTESIAN_POINT('Ctrl Pts',(71.5667118439451,3.00497958064079,48.35));
#83717=CARTESIAN_POINT('Ctrl Pts',(71.6162343630567,2.81214186549187,48.35));
#83718=CARTESIAN_POINT('Ctrl Pts',(71.6162343630567,2.48499327898026,48.35));
#83719=CARTESIAN_POINT('Ctrl Pts',(71.4301498541608,3.33212831616402,48.5));
#83720=CARTESIAN_POINT('Ctrl Pts',(71.4301498541608,3.33212831616402,48.35));
#83721=CARTESIAN_POINT('Ctrl Pts',(71.5171893248335,3.19781729578972,48.5));
#83722=CARTESIAN_POINT('Ctrl Pts',(71.5171893248335,3.19781729578972,48.35));
#83723=CARTESIAN_POINT('Ctrl Pts',(71.5667118439451,3.00497958064079,48.5));
#83724=CARTESIAN_POINT('Ctrl Pts',(71.5667118439451,3.00497958064079,48.35));
#83725=CARTESIAN_POINT('',(71.4301498541608,3.33212831616402,48.5));
#83726=CARTESIAN_POINT('Ctrl Pts',(71.4301498541608,3.33212831616402,48.5));
#83727=CARTESIAN_POINT('Ctrl Pts',(71.5171893248335,3.19781729578972,48.5));
#83728=CARTESIAN_POINT('Ctrl Pts',(71.5667118439451,3.00497958064079,48.5));
#83729=CARTESIAN_POINT('',(71.4301498541608,3.33212831616402,48.35));
#83730=CARTESIAN_POINT('',(71.4301498541608,3.33212831616402,48.5));
#83731=CARTESIAN_POINT('Ctrl Pts',(71.4301498541608,3.33212831616402,48.35));
#83732=CARTESIAN_POINT('Ctrl Pts',(71.5171893248335,3.19781729578972,48.35));
#83733=CARTESIAN_POINT('Ctrl Pts',(71.5667118439451,3.00497958064079,48.35));
#83734=CARTESIAN_POINT('Ctrl Pts',(71.2095500836149,3.5377217233181,48.5));
#83735=CARTESIAN_POINT('Ctrl Pts',(71.2095500836149,3.5377217233181,48.35));
#83736=CARTESIAN_POINT('Ctrl Pts',(71.3431103834882,3.46643933653831,48.5));
#83737=CARTESIAN_POINT('Ctrl Pts',(71.3431103834882,3.46643933653831,48.35));
#83738=CARTESIAN_POINT('Ctrl Pts',(71.4301498541608,3.33212831616402,48.5));
#83739=CARTESIAN_POINT('Ctrl Pts',(71.4301498541608,3.33212831616402,48.35));
#83740=CARTESIAN_POINT('',(71.2095500836149,3.5377217233181,48.5));
#83741=CARTESIAN_POINT('Ctrl Pts',(71.2095500836149,3.5377217233181,48.5));
#83742=CARTESIAN_POINT('Ctrl Pts',(71.3431103834882,3.46643933653831,48.5));
#83743=CARTESIAN_POINT('Ctrl Pts',(71.4301498541608,3.33212831616402,48.5));
#83744=CARTESIAN_POINT('',(71.2095500836149,3.5377217233181,48.35));
#83745=CARTESIAN_POINT('',(71.2095500836149,3.5377217233181,48.5));
#83746=CARTESIAN_POINT('Ctrl Pts',(71.2095500836149,3.5377217233181,48.35));
#83747=CARTESIAN_POINT('Ctrl Pts',(71.3431103834882,3.46643933653831,48.35));
#83748=CARTESIAN_POINT('Ctrl Pts',(71.4301498541608,3.33212831616402,48.35));
#83749=CARTESIAN_POINT('Ctrl Pts',(70.898908556439,3.60900411009789,48.5));
#83750=CARTESIAN_POINT('Ctrl Pts',(70.898908556439,3.60900411009789,48.35));
#83751=CARTESIAN_POINT('Ctrl Pts',(71.0759891876951,3.60900411009789,48.5));
#83752=CARTESIAN_POINT('Ctrl Pts',(71.0759891876951,3.60900411009789,48.35));
#83753=CARTESIAN_POINT('Ctrl Pts',(71.2095500836149,3.5377217233181,48.5));
#83754=CARTESIAN_POINT('Ctrl Pts',(71.2095500836149,3.5377217233181,48.35));
#83755=CARTESIAN_POINT('',(70.898908556439,3.60900411009789,48.5));
#83756=CARTESIAN_POINT('Ctrl Pts',(70.898908556439,3.60900411009789,48.5));
#83757=CARTESIAN_POINT('Ctrl Pts',(71.0759891876951,3.60900411009789,48.5));
#83758=CARTESIAN_POINT('Ctrl Pts',(71.2095500836149,3.5377217233181,48.5));
#83759=CARTESIAN_POINT('',(70.898908556439,3.60900411009789,48.35));
#83760=CARTESIAN_POINT('',(70.898908556439,3.60900411009789,48.5));
#83761=CARTESIAN_POINT('Ctrl Pts',(70.898908556439,3.60900411009789,48.35));
#83762=CARTESIAN_POINT('Ctrl Pts',(71.0759891876951,3.60900411009789,48.35));
#83763=CARTESIAN_POINT('Ctrl Pts',(71.2095500836149,3.5377217233181,48.35));
#83764=CARTESIAN_POINT('Ctrl Pts',(70.5004777321592,3.47994545102119,48.5));
#83765=CARTESIAN_POINT('Ctrl Pts',(70.5004777321592,3.47994545102119,48.35));
#83766=CARTESIAN_POINT('Ctrl Pts',(70.6587995896116,3.60900411009789,48.5));
#83767=CARTESIAN_POINT('Ctrl Pts',(70.6587995896116,3.60900411009789,48.35));
#83768=CARTESIAN_POINT('Ctrl Pts',(70.898908556439,3.60900411009789,48.5));
#83769=CARTESIAN_POINT('Ctrl Pts',(70.898908556439,3.60900411009789,48.35));
#83770=CARTESIAN_POINT('',(70.5004777321592,3.47994545102119,48.5));
#83771=CARTESIAN_POINT('Ctrl Pts',(70.5004777321592,3.47994545102119,48.5));
#83772=CARTESIAN_POINT('Ctrl Pts',(70.6587995896116,3.60900411009789,48.5));
#83773=CARTESIAN_POINT('Ctrl Pts',(70.898908556439,3.60900411009789,48.5));
#83774=CARTESIAN_POINT('',(70.5004777321592,3.47994545102119,48.35));
#83775=CARTESIAN_POINT('',(70.5004777321592,3.47994545102119,48.5));
#83776=CARTESIAN_POINT('Ctrl Pts',(70.5004777321592,3.47994545102119,48.35));
#83777=CARTESIAN_POINT('Ctrl Pts',(70.6587995896116,3.60900411009789,48.35));
#83778=CARTESIAN_POINT('Ctrl Pts',(70.898908556439,3.60900411009789,48.35));
#83779=CARTESIAN_POINT('Ctrl Pts',(70.2618690142408,3.11302864551544,48.5));
#83780=CARTESIAN_POINT('Ctrl Pts',(70.2618690142408,3.11302864551544,48.35));
#83781=CARTESIAN_POINT('Ctrl Pts',(70.3421555766836,3.3508867919445,48.5));
#83782=CARTESIAN_POINT('Ctrl Pts',(70.3421555766836,3.3508867919445,48.35));
#83783=CARTESIAN_POINT('Ctrl Pts',(70.5004777321592,3.47994545102119,48.5));
#83784=CARTESIAN_POINT('Ctrl Pts',(70.5004777321592,3.47994545102119,48.35));
#83785=CARTESIAN_POINT('',(70.2618690142408,3.11302864551544,48.5));
#83786=CARTESIAN_POINT('Ctrl Pts',(70.2618690142408,3.11302864551544,48.5));
#83787=CARTESIAN_POINT('Ctrl Pts',(70.3421555766836,3.3508867919445,48.5));
#83788=CARTESIAN_POINT('Ctrl Pts',(70.5004777321592,3.47994545102119,48.5));
#83789=CARTESIAN_POINT('',(70.2618690142408,3.11302864551544,48.35));
#83790=CARTESIAN_POINT('',(70.2618690142408,3.11302864551544,48.5));
#83791=CARTESIAN_POINT('Ctrl Pts',(70.2618690142408,3.11302864551544,48.35));
#83792=CARTESIAN_POINT('Ctrl Pts',(70.3421555766836,3.3508867919445,48.35));
#83793=CARTESIAN_POINT('Ctrl Pts',(70.5004777321592,3.47994545102119,48.35));
#83794=CARTESIAN_POINT('Ctrl Pts',(70.1815827498212,2.48499327898026,48.5));
#83795=CARTESIAN_POINT('Ctrl Pts',(70.1815827498212,2.48499327898026,48.35));
#83796=CARTESIAN_POINT('Ctrl Pts',(70.1815827498212,2.87517049908638,48.5));
#83797=CARTESIAN_POINT('Ctrl Pts',(70.1815827498212,2.87517049908638,48.35));
#83798=CARTESIAN_POINT('Ctrl Pts',(70.2618690142408,3.11302864551544,48.5));
#83799=CARTESIAN_POINT('Ctrl Pts',(70.2618690142408,3.11302864551544,48.35));
#83800=CARTESIAN_POINT('',(70.1815827498212,2.48499327898026,48.5));
#83801=CARTESIAN_POINT('Ctrl Pts',(70.1815827498212,2.48499327898026,48.5));
#83802=CARTESIAN_POINT('Ctrl Pts',(70.1815827498212,2.87517049908638,48.5));
#83803=CARTESIAN_POINT('Ctrl Pts',(70.2618690142408,3.11302864551544,48.5));
#83804=CARTESIAN_POINT('',(70.1815827498212,2.48499327898026,48.35));
#83805=CARTESIAN_POINT('',(70.1815827498212,2.48499327898026,48.5));
#83806=CARTESIAN_POINT('Ctrl Pts',(70.1815827498212,2.48499327898026,48.35));
#83807=CARTESIAN_POINT('Ctrl Pts',(70.1815827498212,2.87517049908638,48.35));
#83808=CARTESIAN_POINT('Ctrl Pts',(70.2618690142408,3.11302864551544,48.35));
#83809=CARTESIAN_POINT('Ctrl Pts',(70.3991814265028,1.59058684110642,48.5));
#83810=CARTESIAN_POINT('Ctrl Pts',(70.3991814265028,1.59058684110642,48.35));
#83811=CARTESIAN_POINT('Ctrl Pts',(70.1815827498212,1.86521166563034,48.5));
#83812=CARTESIAN_POINT('Ctrl Pts',(70.1815827498212,1.86521166563034,48.35));
#83813=CARTESIAN_POINT('Ctrl Pts',(70.1815827498212,2.48499327898026,48.5));
#83814=CARTESIAN_POINT('Ctrl Pts',(70.1815827498212,2.48499327898026,48.35));
#83815=CARTESIAN_POINT('Ctrl Pts',(70.3991814265028,1.59058684110642,48.5));
#83816=CARTESIAN_POINT('Ctrl Pts',(70.1815827498212,1.86521166563034,48.5));
#83817=CARTESIAN_POINT('Ctrl Pts',(70.1815827498212,2.48499327898026,48.5));
#83818=CARTESIAN_POINT('Ctrl Pts',(70.3991814265028,1.59058684110642,48.35));
#83819=CARTESIAN_POINT('Ctrl Pts',(70.1815827498212,1.86521166563034,48.35));
#83820=CARTESIAN_POINT('Ctrl Pts',(70.1815827498212,2.48499327898026,48.35));
#83821=CARTESIAN_POINT('Origin',(69.9999999562278,2.48574362695217,48.35));
#83822=CARTESIAN_POINT('Origin',(69.3381993779913,3.16630297899246,48.5));
#83823=CARTESIAN_POINT('',(69.3381993779913,3.16630297899246,48.5));
#83824=CARTESIAN_POINT('',(68.6493861982599,2.17435204982758,48.5));
#83825=CARTESIAN_POINT('',(59.1917638899362,-11.4454472114045,48.5));
#83826=CARTESIAN_POINT('',(69.3381993779913,3.16630297899246,48.35));
#83827=CARTESIAN_POINT('',(69.3381993779913,3.16630297899246,48.5));
#83828=CARTESIAN_POINT('',(68.6493861982599,2.17435204982758,48.35));
#83829=CARTESIAN_POINT('',(69.3381993779913,3.16630297899246,48.35));
#83830=CARTESIAN_POINT('',(68.6493861982599,2.17435204982758,48.5));
#83831=CARTESIAN_POINT('Origin',(69.3381993779913,2.17435204982758,48.5));
#83832=CARTESIAN_POINT('',(69.3381993779913,2.17435204982758,48.5));
#83833=CARTESIAN_POINT('',(69.3381993779913,5.08717602491379,48.5));
#83834=CARTESIAN_POINT('',(69.3381993779913,2.17435204982758,48.35));
#83835=CARTESIAN_POINT('',(69.3381993779913,2.17435204982758,48.5));
#83836=CARTESIAN_POINT('',(69.3381993779913,2.17435204982758,48.35));
#83837=CARTESIAN_POINT('Origin',(68.6493861982599,2.17435204982758,48.5));
#83838=CARTESIAN_POINT('',(34.3246930991299,2.17435204982758,48.5));
#83839=CARTESIAN_POINT('',(68.6493861982599,2.17435204982758,48.35));
#83840=CARTESIAN_POINT('Origin',(69.6083219656721,1.92673945426941,48.5));
#83841=CARTESIAN_POINT('',(69.6083219656721,1.92673945426941,48.5));
#83842=CARTESIAN_POINT('',(69.6083219656721,1.40000009536743,48.5));
#83843=CARTESIAN_POINT('',(69.6083219656721,4.9633697271347,48.5));
#83844=CARTESIAN_POINT('',(69.6083219656721,1.92673945426941,48.35));
#83845=CARTESIAN_POINT('',(69.6083219656721,1.92673945426941,48.5));
#83846=CARTESIAN_POINT('',(69.6083219656721,1.40000009536743,48.35));
#83847=CARTESIAN_POINT('',(69.6083219656721,1.92673945426941,48.35));
#83848=CARTESIAN_POINT('',(69.6083219656721,1.40000009536743,48.5));
#83849=CARTESIAN_POINT('Origin',(69.9054570803419,1.92673945426941,48.5));
#83850=CARTESIAN_POINT('',(69.9054570803419,1.92673945426941,48.5));
#83851=CARTESIAN_POINT('',(34.9527285401709,1.92673945426941,48.5));
#83852=CARTESIAN_POINT('',(69.9054570803419,1.92673945426941,48.35));
#83853=CARTESIAN_POINT('',(69.9054570803419,1.92673945426941,48.5));
#83854=CARTESIAN_POINT('',(69.9054570803419,1.92673945426941,48.35));
#83855=CARTESIAN_POINT('Origin',(69.9054570803419,2.17435204982758,48.5));
#83856=CARTESIAN_POINT('',(69.9054570803419,2.17435204982758,48.5));
#83857=CARTESIAN_POINT('',(69.9054570803419,5.08717602491379,48.5));
#83858=CARTESIAN_POINT('',(69.9054570803419,2.17435204982758,48.35));
#83859=CARTESIAN_POINT('',(69.9054570803419,2.17435204982758,48.5));
#83860=CARTESIAN_POINT('',(69.9054570803419,2.17435204982758,48.35));
#83861=CARTESIAN_POINT('Origin',(69.6083219656721,2.17435204982758,48.5));
#83862=CARTESIAN_POINT('',(69.6083219656721,2.17435204982758,48.5));
#83863=CARTESIAN_POINT('',(34.804160982836,2.17435204982758,48.5));
#83864=CARTESIAN_POINT('',(69.6083219656721,2.17435204982758,48.35));
#83865=CARTESIAN_POINT('',(69.6083219656721,2.17435204982758,48.5));
#83866=CARTESIAN_POINT('',(69.6083219656721,2.17435204982758,48.35));
#83867=CARTESIAN_POINT('Origin',(69.6083219656721,3.6000000834465,48.5));
#83868=CARTESIAN_POINT('',(69.6083219656721,3.6000000834465,48.5));
#83869=CARTESIAN_POINT('',(69.6083219656721,5.80000004172325,48.5));
#83870=CARTESIAN_POINT('',(69.6083219656721,3.6000000834465,48.35));
#83871=CARTESIAN_POINT('',(69.6083219656721,3.6000000834465,48.5));
#83872=CARTESIAN_POINT('',(69.6083219656721,3.6000000834465,48.35));
#83873=CARTESIAN_POINT('Origin',(69.3877218971029,3.6000000834465,48.5));
#83874=CARTESIAN_POINT('',(69.3877218971029,3.6000000834465,48.5));
#83875=CARTESIAN_POINT('',(34.6938609485514,3.6000000834465,48.5));
#83876=CARTESIAN_POINT('',(69.3877218971029,3.6000000834465,48.35));
#83877=CARTESIAN_POINT('',(69.3877218971029,3.6000000834465,48.5));
#83878=CARTESIAN_POINT('',(69.3877218971029,3.6000000834465,48.35));
#83879=CARTESIAN_POINT('Origin',(68.383765549399,2.17435204982758,48.5));
#83880=CARTESIAN_POINT('',(68.383765549399,2.17435204982758,48.5));
#83881=CARTESIAN_POINT('',(58.4199877035187,-11.9745104240059,48.5));
#83882=CARTESIAN_POINT('',(68.383765549399,2.17435204982758,48.35));
#83883=CARTESIAN_POINT('',(68.383765549399,2.17435204982758,48.5));
#83884=CARTESIAN_POINT('',(68.383765549399,2.17435204982758,48.35));
#83885=CARTESIAN_POINT('Origin',(68.383765549399,1.92673945426941,48.5));
#83886=CARTESIAN_POINT('',(68.383765549399,1.92673945426941,48.5));
#83887=CARTESIAN_POINT('',(68.383765549399,4.9633697271347,48.5));
#83888=CARTESIAN_POINT('',(68.383765549399,1.92673945426941,48.35));
#83889=CARTESIAN_POINT('',(68.383765549399,1.92673945426941,48.5));
#83890=CARTESIAN_POINT('',(68.383765549399,1.92673945426941,48.35));
#83891=CARTESIAN_POINT('Origin',(69.3381993779913,1.92673945426941,48.5));
#83892=CARTESIAN_POINT('',(69.3381993779913,1.92673945426941,48.5));
#83893=CARTESIAN_POINT('',(34.6690996889956,1.92673945426941,48.5));
#83894=CARTESIAN_POINT('',(69.3381993779913,1.92673945426941,48.35));
#83895=CARTESIAN_POINT('',(69.3381993779913,1.92673945426941,48.5));
#83896=CARTESIAN_POINT('',(69.3381993779913,1.92673945426941,48.35));
#83897=CARTESIAN_POINT('Origin',(69.3381993779913,1.40000009536743,48.5));
#83898=CARTESIAN_POINT('',(69.3381993779913,1.40000009536743,48.5));
#83899=CARTESIAN_POINT('',(69.3381993779913,4.70000004768372,48.5));
#83900=CARTESIAN_POINT('',(69.3381993779913,1.40000009536743,48.35));
#83901=CARTESIAN_POINT('',(69.3381993779913,1.40000009536743,48.5));
#83902=CARTESIAN_POINT('',(69.3381993779913,1.40000009536743,48.35));
#83903=CARTESIAN_POINT('Origin',(69.6083219656721,1.40000009536743,48.5));
#83904=CARTESIAN_POINT('',(34.804160982836,1.40000009536743,48.5));
#83905=CARTESIAN_POINT('',(69.6083219656721,1.40000009536743,48.35));
#83906=CARTESIAN_POINT('Origin',(69.9999999562278,2.48574362695217,48.35));
#83907=CARTESIAN_POINT('Origin',(0.,8.,48.5));
#83908=CARTESIAN_POINT('Origin',(0.,8.,48.5));
#83909=CARTESIAN_POINT('Ctrl Pts',(60.8516373746097,3.38540250062943,48.5));
#83910=CARTESIAN_POINT('Ctrl Pts',(60.8516373746097,3.38540250062943,48.35));
#83911=CARTESIAN_POINT('Ctrl Pts',(60.6655525676906,3.38540250062943,48.5));
#83912=CARTESIAN_POINT('Ctrl Pts',(60.6655525676906,3.38540250062943,48.35));
#83913=CARTESIAN_POINT('Ctrl Pts',(60.5545022599399,3.22783091664314,48.5));
#83914=CARTESIAN_POINT('Ctrl Pts',(60.5545022599399,3.22783091664314,48.35));
#83915=CARTESIAN_POINT('',(60.8516373746097,3.38540250062943,48.5));
#83916=CARTESIAN_POINT('',(60.5545022599399,3.22783091664314,48.5));
#83917=CARTESIAN_POINT('Ctrl Pts',(60.8516373746097,3.38540250062943,48.5));
#83918=CARTESIAN_POINT('Ctrl Pts',(60.6655525676906,3.38540250062943,48.5));
#83919=CARTESIAN_POINT('Ctrl Pts',(60.5545022599399,3.22783091664314,48.5));
#83920=CARTESIAN_POINT('',(60.8516373746097,3.38540250062943,48.35));
#83921=CARTESIAN_POINT('',(60.8516373746097,3.38540250062943,48.5));
#83922=CARTESIAN_POINT('',(60.5545022599399,3.22783091664314,48.35));
#83923=CARTESIAN_POINT('Ctrl Pts',(60.8516373746097,3.38540250062943,48.35));
#83924=CARTESIAN_POINT('Ctrl Pts',(60.6655525676906,3.38540250062943,48.35));
#83925=CARTESIAN_POINT('Ctrl Pts',(60.5545022599399,3.22783091664314,48.35));
#83926=CARTESIAN_POINT('',(60.5545022599399,3.22783091664314,48.5));
#83927=CARTESIAN_POINT('Ctrl Pts',(61.1675306670368,3.2068213224411,48.5));
#83928=CARTESIAN_POINT('Ctrl Pts',(61.1675306670368,3.2068213224411,48.35));
#83929=CARTESIAN_POINT('Ctrl Pts',(61.04072297737,3.38540250062943,48.5));
#83930=CARTESIAN_POINT('Ctrl Pts',(61.04072297737,3.38540250062943,48.35));
#83931=CARTESIAN_POINT('Ctrl Pts',(60.8516373746097,3.38540250062943,48.5));
#83932=CARTESIAN_POINT('Ctrl Pts',(60.8516373746097,3.38540250062943,48.35));
#83933=CARTESIAN_POINT('',(61.1675306670368,3.2068213224411,48.5));
#83934=CARTESIAN_POINT('Ctrl Pts',(61.1675306670368,3.2068213224411,48.5));
#83935=CARTESIAN_POINT('Ctrl Pts',(61.04072297737,3.38540250062943,48.5));
#83936=CARTESIAN_POINT('Ctrl Pts',(60.8516373746097,3.38540250062943,48.5));
#83937=CARTESIAN_POINT('',(61.1675306670368,3.2068213224411,48.35));
#83938=CARTESIAN_POINT('',(61.1675306670368,3.2068213224411,48.5));
#83939=CARTESIAN_POINT('Ctrl Pts',(61.1675306670368,3.2068213224411,48.35));
#83940=CARTESIAN_POINT('Ctrl Pts',(61.04072297737,3.38540250062943,48.35));
#83941=CARTESIAN_POINT('Ctrl Pts',(60.8516373746097,3.38540250062943,48.35));
#83942=CARTESIAN_POINT('Ctrl Pts',(61.2943383567035,2.48499327898026,48.5));
#83943=CARTESIAN_POINT('Ctrl Pts',(61.2943383567035,2.48499327898026,48.35));
#83944=CARTESIAN_POINT('Ctrl Pts',(61.2943383567035,3.02824014425278,48.5));
#83945=CARTESIAN_POINT('Ctrl Pts',(61.2943383567035,3.02824014425278,48.35));
#83946=CARTESIAN_POINT('Ctrl Pts',(61.1675306670368,3.2068213224411,48.5));
#83947=CARTESIAN_POINT('Ctrl Pts',(61.1675306670368,3.2068213224411,48.35));
#83948=CARTESIAN_POINT('',(61.2943383567035,2.48499327898026,48.5));
#83949=CARTESIAN_POINT('Ctrl Pts',(61.2943383567035,2.48499327898026,48.5));
#83950=CARTESIAN_POINT('Ctrl Pts',(61.2943383567035,3.02824014425278,48.5));
#83951=CARTESIAN_POINT('Ctrl Pts',(61.1675306670368,3.2068213224411,48.5));
#83952=CARTESIAN_POINT('',(61.2943383567035,2.48499327898026,48.35));
#83953=CARTESIAN_POINT('',(61.2943383567035,2.48499327898026,48.5));
#83954=CARTESIAN_POINT('Ctrl Pts',(61.2943383567035,2.48499327898026,48.35));
#83955=CARTESIAN_POINT('Ctrl Pts',(61.2943383567035,3.02824014425278,48.35));
#83956=CARTESIAN_POINT('Ctrl Pts',(61.1675306670368,3.2068213224411,48.35));
#83957=CARTESIAN_POINT('Ctrl Pts',(61.1675306670368,1.76466578245163,48.5));
#83958=CARTESIAN_POINT('Ctrl Pts',(61.1675306670368,1.76466578245163,48.35));
#83959=CARTESIAN_POINT('Ctrl Pts',(61.2943383567035,1.9447478055954,48.5));
#83960=CARTESIAN_POINT('Ctrl Pts',(61.2943383567035,1.9447478055954,48.35));
#83961=CARTESIAN_POINT('Ctrl Pts',(61.2943383567035,2.48499327898026,48.5));
#83962=CARTESIAN_POINT('Ctrl Pts',(61.2943383567035,2.48499327898026,48.35));
#83963=CARTESIAN_POINT('',(61.1675306670368,1.76466578245163,48.5));
#83964=CARTESIAN_POINT('Ctrl Pts',(61.1675306670368,1.76466578245163,48.5));
#83965=CARTESIAN_POINT('Ctrl Pts',(61.2943383567035,1.9447478055954,48.5));
#83966=CARTESIAN_POINT('Ctrl Pts',(61.2943383567035,2.48499327898026,48.5));
#83967=CARTESIAN_POINT('',(61.1675306670368,1.76466578245163,48.35));
#83968=CARTESIAN_POINT('',(61.1675306670368,1.76466578245163,48.5));
#83969=CARTESIAN_POINT('Ctrl Pts',(61.1675306670368,1.76466578245163,48.35));
#83970=CARTESIAN_POINT('Ctrl Pts',(61.2943383567035,1.9447478055954,48.35));
#83971=CARTESIAN_POINT('Ctrl Pts',(61.2943383567035,2.48499327898026,48.35));
#83972=CARTESIAN_POINT('Ctrl Pts',(60.8546384684741,1.58458405733109,48.5));
#83973=CARTESIAN_POINT('Ctrl Pts',(60.8546384684741,1.58458405733109,48.35));
#83974=CARTESIAN_POINT('Ctrl Pts',(61.04072297737,1.58458405733109,48.5));
#83975=CARTESIAN_POINT('Ctrl Pts',(61.04072297737,1.58458405733109,48.35));
#83976=CARTESIAN_POINT('Ctrl Pts',(61.1675306670368,1.76466578245163,48.5));
#83977=CARTESIAN_POINT('Ctrl Pts',(61.1675306670368,1.76466578245163,48.35));
#83978=CARTESIAN_POINT('',(60.8546384684741,1.58458405733109,48.5));
#83979=CARTESIAN_POINT('Ctrl Pts',(60.8546384684741,1.58458405733109,48.5));
#83980=CARTESIAN_POINT('Ctrl Pts',(61.04072297737,1.58458405733109,48.5));
#83981=CARTESIAN_POINT('Ctrl Pts',(61.1675306670368,1.76466578245163,48.5));
#83982=CARTESIAN_POINT('',(60.8546384684741,1.58458405733109,48.35));
#83983=CARTESIAN_POINT('',(60.8546384684741,1.58458405733109,48.5));
#83984=CARTESIAN_POINT('Ctrl Pts',(60.8546384684741,1.58458405733109,48.35));
#83985=CARTESIAN_POINT('Ctrl Pts',(61.04072297737,1.58458405733109,48.35));
#83986=CARTESIAN_POINT('Ctrl Pts',(61.1675306670368,1.76466578245163,48.35));
#83987=CARTESIAN_POINT('Ctrl Pts',(60.5417462699115,1.76391565799713,48.5));
#83988=CARTESIAN_POINT('Ctrl Pts',(60.5417462699115,1.76391565799713,48.35));
#83989=CARTESIAN_POINT('Ctrl Pts',(60.6685539595783,1.58458405733109,48.5));
#83990=CARTESIAN_POINT('Ctrl Pts',(60.6685539595783,1.58458405733109,48.35));
#83991=CARTESIAN_POINT('Ctrl Pts',(60.8546384684741,1.58458405733109,48.5));
#83992=CARTESIAN_POINT('Ctrl Pts',(60.8546384684741,1.58458405733109,48.35));
#83993=CARTESIAN_POINT('',(60.5417462699115,1.76391565799713,48.5));
#83994=CARTESIAN_POINT('Ctrl Pts',(60.5417462699115,1.76391565799713,48.5));
#83995=CARTESIAN_POINT('Ctrl Pts',(60.6685539595783,1.58458405733109,48.5));
#83996=CARTESIAN_POINT('Ctrl Pts',(60.8546384684741,1.58458405733109,48.5));
#83997=CARTESIAN_POINT('',(60.5417462699115,1.76391565799713,48.35));
#83998=CARTESIAN_POINT('',(60.5417462699115,1.76391565799713,48.5));
#83999=CARTESIAN_POINT('Ctrl Pts',(60.5417462699115,1.76391565799713,48.35));
#84000=CARTESIAN_POINT('Ctrl Pts',(60.6685539595783,1.58458405733109,48.35));
#84001=CARTESIAN_POINT('Ctrl Pts',(60.8546384684741,1.58458405733109,48.35));
#84002=CARTESIAN_POINT('Ctrl Pts',(60.4149385802448,2.48499327898026,48.5));
#84003=CARTESIAN_POINT('Ctrl Pts',(60.4149385802448,2.48499327898026,48.35));
#84004=CARTESIAN_POINT('Ctrl Pts',(60.4149385802448,1.94324696063995,48.5));
#84005=CARTESIAN_POINT('Ctrl Pts',(60.4149385802448,1.94324696063995,48.35));
#84006=CARTESIAN_POINT('Ctrl Pts',(60.5417462699115,1.76391565799713,48.5));
#84007=CARTESIAN_POINT('Ctrl Pts',(60.5417462699115,1.76391565799713,48.35));
#84008=CARTESIAN_POINT('',(60.4149385802448,2.48499327898026,48.5));
#84009=CARTESIAN_POINT('Ctrl Pts',(60.4149385802448,2.48499327898026,48.5));
#84010=CARTESIAN_POINT('Ctrl Pts',(60.4149385802448,1.94324696063995,48.5));
#84011=CARTESIAN_POINT('Ctrl Pts',(60.5417462699115,1.76391565799713,48.5));
#84012=CARTESIAN_POINT('',(60.4149385802448,2.48499327898026,48.35));
#84013=CARTESIAN_POINT('',(60.4149385802448,2.48499327898026,48.5));
#84014=CARTESIAN_POINT('Ctrl Pts',(60.4149385802448,2.48499327898026,48.35));
#84015=CARTESIAN_POINT('Ctrl Pts',(60.4149385802448,1.94324696063995,48.35));
#84016=CARTESIAN_POINT('Ctrl Pts',(60.5417462699115,1.76391565799713,48.35));
#84017=CARTESIAN_POINT('Ctrl Pts',(60.5545022599399,3.22783091664314,48.5));
#84018=CARTESIAN_POINT('Ctrl Pts',(60.5545022599399,3.22783091664314,48.35));
#84019=CARTESIAN_POINT('Ctrl Pts',(60.4149385802448,3.02673944830894,48.5));
#84020=CARTESIAN_POINT('Ctrl Pts',(60.4149385802448,3.02673944830894,48.35));
#84021=CARTESIAN_POINT('Ctrl Pts',(60.4149385802448,2.48499327898026,48.5));
#84022=CARTESIAN_POINT('Ctrl Pts',(60.4149385802448,2.48499327898026,48.35));
#84023=CARTESIAN_POINT('Ctrl Pts',(60.5545022599399,3.22783091664314,48.5));
#84024=CARTESIAN_POINT('Ctrl Pts',(60.4149385802448,3.02673944830894,48.5));
#84025=CARTESIAN_POINT('Ctrl Pts',(60.4149385802448,2.48499327898026,48.5));
#84026=CARTESIAN_POINT('Ctrl Pts',(60.5545022599399,3.22783091664314,48.35));
#84027=CARTESIAN_POINT('Ctrl Pts',(60.4149385802448,3.02673944830894,48.35));
#84028=CARTESIAN_POINT('Ctrl Pts',(60.4149385802448,2.48499327898026,48.35));
#84029=CARTESIAN_POINT('Ctrl Pts',(60.8546384684741,1.36248314380646,48.5));
#84030=CARTESIAN_POINT('Ctrl Pts',(60.8546384684741,1.36248314380646,48.35));
#84031=CARTESIAN_POINT('Ctrl Pts',(60.5364939086139,1.36248314380646,48.5));
#84032=CARTESIAN_POINT('Ctrl Pts',(60.5364939086139,1.36248314380646,48.35));
#84033=CARTESIAN_POINT('Ctrl Pts',(60.3549113385379,1.59058684110642,48.5));
#84034=CARTESIAN_POINT('Ctrl Pts',(60.3549113385379,1.59058684110642,48.35));
#84035=CARTESIAN_POINT('',(60.8546384684741,1.36248314380646,48.5));
#84036=CARTESIAN_POINT('',(60.3549113385379,1.59058684110642,48.5));
#84037=CARTESIAN_POINT('Ctrl Pts',(60.8546384684741,1.36248314380646,48.5));
#84038=CARTESIAN_POINT('Ctrl Pts',(60.5364939086139,1.36248314380646,48.5));
#84039=CARTESIAN_POINT('Ctrl Pts',(60.3549113385379,1.59058684110642,48.5));
#84040=CARTESIAN_POINT('',(60.8546384684741,1.36248314380646,48.35));
#84041=CARTESIAN_POINT('',(60.8546384684741,1.36248314380646,48.5));
#84042=CARTESIAN_POINT('',(60.3549113385379,1.59058684110642,48.35));
#84043=CARTESIAN_POINT('Ctrl Pts',(60.8546384684741,1.36248314380646,48.35));
#84044=CARTESIAN_POINT('Ctrl Pts',(60.5364939086139,1.36248314380646,48.35));
#84045=CARTESIAN_POINT('Ctrl Pts',(60.3549113385379,1.59058684110642,48.35));
#84046=CARTESIAN_POINT('',(60.3549113385379,1.59058684110642,48.5));
#84047=CARTESIAN_POINT('Ctrl Pts',(61.2545701377094,1.49229192733765,48.5));
#84048=CARTESIAN_POINT('Ctrl Pts',(61.2545701377094,1.49229192733765,48.35));
#84049=CARTESIAN_POINT('Ctrl Pts',(61.096248280257,1.36248314380646,48.5));
#84050=CARTESIAN_POINT('Ctrl Pts',(61.096248280257,1.36248314380646,48.35));
#84051=CARTESIAN_POINT('Ctrl Pts',(60.8546384684741,1.36248314380646,48.5));
#84052=CARTESIAN_POINT('Ctrl Pts',(60.8546384684741,1.36248314380646,48.35));
#84053=CARTESIAN_POINT('',(61.2545701377094,1.49229192733765,48.5));
#84054=CARTESIAN_POINT('Ctrl Pts',(61.2545701377094,1.49229192733765,48.5));
#84055=CARTESIAN_POINT('Ctrl Pts',(61.096248280257,1.36248314380646,48.5));
#84056=CARTESIAN_POINT('Ctrl Pts',(60.8546384684741,1.36248314380646,48.5));
#84057=CARTESIAN_POINT('',(61.2545701377094,1.49229192733765,48.35));
#84058=CARTESIAN_POINT('',(61.2545701377094,1.49229192733765,48.5));
#84059=CARTESIAN_POINT('Ctrl Pts',(61.2545701377094,1.49229192733765,48.35));
#84060=CARTESIAN_POINT('Ctrl Pts',(61.096248280257,1.36248314380646,48.35));
#84061=CARTESIAN_POINT('Ctrl Pts',(60.8546384684741,1.36248314380646,48.35));
#84062=CARTESIAN_POINT('Ctrl Pts',(61.4924284331501,1.85995900630951,48.5));
#84063=CARTESIAN_POINT('Ctrl Pts',(61.4924284331501,1.85995900630951,48.35));
#84064=CARTESIAN_POINT('Ctrl Pts',(61.4128919951618,1.62210100889206,48.5));
#84065=CARTESIAN_POINT('Ctrl Pts',(61.4128919951618,1.62210100889206,48.35));
#84066=CARTESIAN_POINT('Ctrl Pts',(61.2545701377094,1.49229192733765,48.5));
#84067=CARTESIAN_POINT('Ctrl Pts',(61.2545701377094,1.49229192733765,48.35));
#84068=CARTESIAN_POINT('',(61.4924284331501,1.85995900630951,48.5));
#84069=CARTESIAN_POINT('Ctrl Pts',(61.4924284331501,1.85995900630951,48.5));
#84070=CARTESIAN_POINT('Ctrl Pts',(61.4128919951618,1.62210100889206,48.5));
#84071=CARTESIAN_POINT('Ctrl Pts',(61.2545701377094,1.49229192733765,48.5));
#84072=CARTESIAN_POINT('',(61.4924284331501,1.85995900630951,48.35));
#84073=CARTESIAN_POINT('',(61.4924284331501,1.85995900630951,48.5));
#84074=CARTESIAN_POINT('Ctrl Pts',(61.4924284331501,1.85995900630951,48.35));
#84075=CARTESIAN_POINT('Ctrl Pts',(61.4128919951618,1.62210100889206,48.35));
#84076=CARTESIAN_POINT('Ctrl Pts',(61.2545701377094,1.49229192733765,48.35));
#84077=CARTESIAN_POINT('Ctrl Pts',(61.5719642750919,2.48499327898026,48.5));
#84078=CARTESIAN_POINT('Ctrl Pts',(61.5719642750919,2.48499327898026,48.35));
#84079=CARTESIAN_POINT('Ctrl Pts',(61.5719642750919,2.09781730175018,48.5));
#84080=CARTESIAN_POINT('Ctrl Pts',(61.5719642750919,2.09781730175018,48.35));
#84081=CARTESIAN_POINT('Ctrl Pts',(61.4924284331501,1.85995900630951,48.5));
#84082=CARTESIAN_POINT('Ctrl Pts',(61.4924284331501,1.85995900630951,48.35));
#84083=CARTESIAN_POINT('',(61.5719642750919,2.48499327898026,48.5));
#84084=CARTESIAN_POINT('Ctrl Pts',(61.5719642750919,2.48499327898026,48.5));
#84085=CARTESIAN_POINT('Ctrl Pts',(61.5719642750919,2.09781730175018,48.5));
#84086=CARTESIAN_POINT('Ctrl Pts',(61.4924284331501,1.85995900630951,48.5));
#84087=CARTESIAN_POINT('',(61.5719642750919,2.48499327898026,48.35));
#84088=CARTESIAN_POINT('',(61.5719642750919,2.48499327898026,48.5));
#84089=CARTESIAN_POINT('Ctrl Pts',(61.5719642750919,2.48499327898026,48.35));
#84090=CARTESIAN_POINT('Ctrl Pts',(61.5719642750919,2.09781730175018,48.35));
#84091=CARTESIAN_POINT('Ctrl Pts',(61.4924284331501,1.85995900630951,48.35));
#84092=CARTESIAN_POINT('Ctrl Pts',(61.5224417559803,3.00497958064079,48.5));
#84093=CARTESIAN_POINT('Ctrl Pts',(61.5224417559803,3.00497958064079,48.35));
#84094=CARTESIAN_POINT('Ctrl Pts',(61.5719642750919,2.81214186549187,48.5));
#84095=CARTESIAN_POINT('Ctrl Pts',(61.5719642750919,2.81214186549187,48.35));
#84096=CARTESIAN_POINT('Ctrl Pts',(61.5719642750919,2.48499327898026,48.5));
#84097=CARTESIAN_POINT('Ctrl Pts',(61.5719642750919,2.48499327898026,48.35));
#84098=CARTESIAN_POINT('',(61.5224417559803,3.00497958064079,48.5));
#84099=CARTESIAN_POINT('Ctrl Pts',(61.5224417559803,3.00497958064079,48.5));
#84100=CARTESIAN_POINT('Ctrl Pts',(61.5719642750919,2.81214186549187,48.5));
#84101=CARTESIAN_POINT('Ctrl Pts',(61.5719642750919,2.48499327898026,48.5));
#84102=CARTESIAN_POINT('',(61.5224417559803,3.00497958064079,48.35));
#84103=CARTESIAN_POINT('',(61.5224417559803,3.00497958064079,48.5));
#84104=CARTESIAN_POINT('Ctrl Pts',(61.5224417559803,3.00497958064079,48.35));
#84105=CARTESIAN_POINT('Ctrl Pts',(61.5719642750919,2.81214186549187,48.35));
#84106=CARTESIAN_POINT('Ctrl Pts',(61.5719642750919,2.48499327898026,48.35));
#84107=CARTESIAN_POINT('Ctrl Pts',(61.385879766196,3.33212831616402,48.5));
#84108=CARTESIAN_POINT('Ctrl Pts',(61.385879766196,3.33212831616402,48.35));
#84109=CARTESIAN_POINT('Ctrl Pts',(61.4729192368686,3.19781729578972,48.5));
#84110=CARTESIAN_POINT('Ctrl Pts',(61.4729192368686,3.19781729578972,48.35));
#84111=CARTESIAN_POINT('Ctrl Pts',(61.5224417559803,3.00497958064079,48.5));
#84112=CARTESIAN_POINT('Ctrl Pts',(61.5224417559803,3.00497958064079,48.35));
#84113=CARTESIAN_POINT('',(61.385879766196,3.33212831616402,48.5));
#84114=CARTESIAN_POINT('Ctrl Pts',(61.385879766196,3.33212831616402,48.5));
#84115=CARTESIAN_POINT('Ctrl Pts',(61.4729192368686,3.19781729578972,48.5));
#84116=CARTESIAN_POINT('Ctrl Pts',(61.5224417559803,3.00497958064079,48.5));
#84117=CARTESIAN_POINT('',(61.385879766196,3.33212831616402,48.35));
#84118=CARTESIAN_POINT('',(61.385879766196,3.33212831616402,48.5));
#84119=CARTESIAN_POINT('Ctrl Pts',(61.385879766196,3.33212831616402,48.35));
#84120=CARTESIAN_POINT('Ctrl Pts',(61.4729192368686,3.19781729578972,48.35));
#84121=CARTESIAN_POINT('Ctrl Pts',(61.5224417559803,3.00497958064079,48.35));
#84122=CARTESIAN_POINT('Ctrl Pts',(61.1652799956501,3.5377217233181,48.5));
#84123=CARTESIAN_POINT('Ctrl Pts',(61.1652799956501,3.5377217233181,48.35));
#84124=CARTESIAN_POINT('Ctrl Pts',(61.2988402955234,3.46643933653831,48.5));
#84125=CARTESIAN_POINT('Ctrl Pts',(61.2988402955234,3.46643933653831,48.35));
#84126=CARTESIAN_POINT('Ctrl Pts',(61.385879766196,3.33212831616402,48.5));
#84127=CARTESIAN_POINT('Ctrl Pts',(61.385879766196,3.33212831616402,48.35));
#84128=CARTESIAN_POINT('',(61.1652799956501,3.5377217233181,48.5));
#84129=CARTESIAN_POINT('Ctrl Pts',(61.1652799956501,3.5377217233181,48.5));
#84130=CARTESIAN_POINT('Ctrl Pts',(61.2988402955234,3.46643933653831,48.5));
#84131=CARTESIAN_POINT('Ctrl Pts',(61.385879766196,3.33212831616402,48.5));
#84132=CARTESIAN_POINT('',(61.1652799956501,3.5377217233181,48.35));
#84133=CARTESIAN_POINT('',(61.1652799956501,3.5377217233181,48.5));
#84134=CARTESIAN_POINT('Ctrl Pts',(61.1652799956501,3.5377217233181,48.35));
#84135=CARTESIAN_POINT('Ctrl Pts',(61.2988402955234,3.46643933653831,48.35));
#84136=CARTESIAN_POINT('Ctrl Pts',(61.385879766196,3.33212831616402,48.35));
#84137=CARTESIAN_POINT('Ctrl Pts',(60.8546384684741,3.60900411009789,48.5));
#84138=CARTESIAN_POINT('Ctrl Pts',(60.8546384684741,3.60900411009789,48.35));
#84139=CARTESIAN_POINT('Ctrl Pts',(61.0317190997303,3.60900411009789,48.5));
#84140=CARTESIAN_POINT('Ctrl Pts',(61.0317190997303,3.60900411009789,48.35));
#84141=CARTESIAN_POINT('Ctrl Pts',(61.1652799956501,3.5377217233181,48.5));
#84142=CARTESIAN_POINT('Ctrl Pts',(61.1652799956501,3.5377217233181,48.35));
#84143=CARTESIAN_POINT('',(60.8546384684741,3.60900411009789,48.5));
#84144=CARTESIAN_POINT('Ctrl Pts',(60.8546384684741,3.60900411009789,48.5));
#84145=CARTESIAN_POINT('Ctrl Pts',(61.0317190997303,3.60900411009789,48.5));
#84146=CARTESIAN_POINT('Ctrl Pts',(61.1652799956501,3.5377217233181,48.5));
#84147=CARTESIAN_POINT('',(60.8546384684741,3.60900411009789,48.35));
#84148=CARTESIAN_POINT('',(60.8546384684741,3.60900411009789,48.5));
#84149=CARTESIAN_POINT('Ctrl Pts',(60.8546384684741,3.60900411009789,48.35));
#84150=CARTESIAN_POINT('Ctrl Pts',(61.0317190997303,3.60900411009789,48.35));
#84151=CARTESIAN_POINT('Ctrl Pts',(61.1652799956501,3.5377217233181,48.35));
#84152=CARTESIAN_POINT('Ctrl Pts',(60.4562076441944,3.47994545102119,48.5));
#84153=CARTESIAN_POINT('Ctrl Pts',(60.4562076441944,3.47994545102119,48.35));
#84154=CARTESIAN_POINT('Ctrl Pts',(60.6145295016468,3.60900411009789,48.5));
#84155=CARTESIAN_POINT('Ctrl Pts',(60.6145295016468,3.60900411009789,48.35));
#84156=CARTESIAN_POINT('Ctrl Pts',(60.8546384684741,3.60900411009789,48.5));
#84157=CARTESIAN_POINT('Ctrl Pts',(60.8546384684741,3.60900411009789,48.35));
#84158=CARTESIAN_POINT('',(60.4562076441944,3.47994545102119,48.5));
#84159=CARTESIAN_POINT('Ctrl Pts',(60.4562076441944,3.47994545102119,48.5));
#84160=CARTESIAN_POINT('Ctrl Pts',(60.6145295016468,3.60900411009789,48.5));
#84161=CARTESIAN_POINT('Ctrl Pts',(60.8546384684741,3.60900411009789,48.5));
#84162=CARTESIAN_POINT('',(60.4562076441944,3.47994545102119,48.35));
#84163=CARTESIAN_POINT('',(60.4562076441944,3.47994545102119,48.5));
#84164=CARTESIAN_POINT('Ctrl Pts',(60.4562076441944,3.47994545102119,48.35));
#84165=CARTESIAN_POINT('Ctrl Pts',(60.6145295016468,3.60900411009789,48.35));
#84166=CARTESIAN_POINT('Ctrl Pts',(60.8546384684741,3.60900411009789,48.35));
#84167=CARTESIAN_POINT('Ctrl Pts',(60.217598926276,3.11302864551544,48.5));
#84168=CARTESIAN_POINT('Ctrl Pts',(60.217598926276,3.11302864551544,48.35));
#84169=CARTESIAN_POINT('Ctrl Pts',(60.2978854887187,3.3508867919445,48.5));
#84170=CARTESIAN_POINT('Ctrl Pts',(60.2978854887187,3.3508867919445,48.35));
#84171=CARTESIAN_POINT('Ctrl Pts',(60.4562076441944,3.47994545102119,48.5));
#84172=CARTESIAN_POINT('Ctrl Pts',(60.4562076441944,3.47994545102119,48.35));
#84173=CARTESIAN_POINT('',(60.217598926276,3.11302864551544,48.5));
#84174=CARTESIAN_POINT('Ctrl Pts',(60.217598926276,3.11302864551544,48.5));
#84175=CARTESIAN_POINT('Ctrl Pts',(60.2978854887187,3.3508867919445,48.5));
#84176=CARTESIAN_POINT('Ctrl Pts',(60.4562076441944,3.47994545102119,48.5));
#84177=CARTESIAN_POINT('',(60.217598926276,3.11302864551544,48.35));
#84178=CARTESIAN_POINT('',(60.217598926276,3.11302864551544,48.5));
#84179=CARTESIAN_POINT('Ctrl Pts',(60.217598926276,3.11302864551544,48.35));
#84180=CARTESIAN_POINT('Ctrl Pts',(60.2978854887187,3.3508867919445,48.35));
#84181=CARTESIAN_POINT('Ctrl Pts',(60.4562076441944,3.47994545102119,48.35));
#84182=CARTESIAN_POINT('Ctrl Pts',(60.1373126618564,2.48499327898026,48.5));
#84183=CARTESIAN_POINT('Ctrl Pts',(60.1373126618564,2.48499327898026,48.35));
#84184=CARTESIAN_POINT('Ctrl Pts',(60.1373126618564,2.87517049908638,48.5));
#84185=CARTESIAN_POINT('Ctrl Pts',(60.1373126618564,2.87517049908638,48.35));
#84186=CARTESIAN_POINT('Ctrl Pts',(60.217598926276,3.11302864551544,48.5));
#84187=CARTESIAN_POINT('Ctrl Pts',(60.217598926276,3.11302864551544,48.35));
#84188=CARTESIAN_POINT('',(60.1373126618564,2.48499327898026,48.5));
#84189=CARTESIAN_POINT('Ctrl Pts',(60.1373126618564,2.48499327898026,48.5));
#84190=CARTESIAN_POINT('Ctrl Pts',(60.1373126618564,2.87517049908638,48.5));
#84191=CARTESIAN_POINT('Ctrl Pts',(60.217598926276,3.11302864551544,48.5));
#84192=CARTESIAN_POINT('',(60.1373126618564,2.48499327898026,48.35));
#84193=CARTESIAN_POINT('',(60.1373126618564,2.48499327898026,48.5));
#84194=CARTESIAN_POINT('Ctrl Pts',(60.1373126618564,2.48499327898026,48.35));
#84195=CARTESIAN_POINT('Ctrl Pts',(60.1373126618564,2.87517049908638,48.35));
#84196=CARTESIAN_POINT('Ctrl Pts',(60.217598926276,3.11302864551544,48.35));
#84197=CARTESIAN_POINT('Ctrl Pts',(60.3549113385379,1.59058684110642,48.5));
#84198=CARTESIAN_POINT('Ctrl Pts',(60.3549113385379,1.59058684110642,48.35));
#84199=CARTESIAN_POINT('Ctrl Pts',(60.1373126618564,1.86521166563034,48.5));
#84200=CARTESIAN_POINT('Ctrl Pts',(60.1373126618564,1.86521166563034,48.35));
#84201=CARTESIAN_POINT('Ctrl Pts',(60.1373126618564,2.48499327898026,48.5));
#84202=CARTESIAN_POINT('Ctrl Pts',(60.1373126618564,2.48499327898026,48.35));
#84203=CARTESIAN_POINT('Ctrl Pts',(60.3549113385379,1.59058684110642,48.5));
#84204=CARTESIAN_POINT('Ctrl Pts',(60.1373126618564,1.86521166563034,48.5));
#84205=CARTESIAN_POINT('Ctrl Pts',(60.1373126618564,2.48499327898026,48.5));
#84206=CARTESIAN_POINT('Ctrl Pts',(60.3549113385379,1.59058684110642,48.35));
#84207=CARTESIAN_POINT('Ctrl Pts',(60.1373126618564,1.86521166563034,48.35));
#84208=CARTESIAN_POINT('Ctrl Pts',(60.1373126618564,2.48499327898026,48.35));
#84209=CARTESIAN_POINT('Origin',(59.9999999515712,2.48574362695217,48.35));
#84210=CARTESIAN_POINT('Ctrl Pts',(59.1348570100963,1.36248314380646,48.5));
#84211=CARTESIAN_POINT('Ctrl Pts',(59.1348570100963,1.36248314380646,48.35));
#84212=CARTESIAN_POINT('Ctrl Pts',(58.8347205035388,1.36248314380646,48.5));
#84213=CARTESIAN_POINT('Ctrl Pts',(58.8347205035388,1.36248314380646,48.35));
#84214=CARTESIAN_POINT('Ctrl Pts',(58.6448841802776,1.53055930137634,48.5));
#84215=CARTESIAN_POINT('Ctrl Pts',(58.6448841802776,1.53055930137634,48.35));
#84216=CARTESIAN_POINT('',(59.1348570100963,1.36248314380646,48.5));
#84217=CARTESIAN_POINT('',(58.6448841802776,1.53055930137634,48.5));
#84218=CARTESIAN_POINT('Ctrl Pts',(59.1348570100963,1.36248314380646,48.5));
#84219=CARTESIAN_POINT('Ctrl Pts',(58.8347205035388,1.36248314380646,48.5));
#84220=CARTESIAN_POINT('Ctrl Pts',(58.6448841802776,1.53055930137634,48.5));
#84221=CARTESIAN_POINT('',(59.1348570100963,1.36248314380646,48.35));
#84222=CARTESIAN_POINT('',(59.1348570100963,1.36248314380646,48.5));
#84223=CARTESIAN_POINT('',(58.6448841802776,1.53055930137634,48.35));
#84224=CARTESIAN_POINT('Ctrl Pts',(59.1348570100963,1.36248314380646,48.35));
#84225=CARTESIAN_POINT('Ctrl Pts',(58.8347205035388,1.36248314380646,48.35));
#84226=CARTESIAN_POINT('Ctrl Pts',(58.6448841802776,1.53055930137634,48.35));
#84227=CARTESIAN_POINT('',(58.6448841802776,1.53055930137634,48.5));
#84228=CARTESIAN_POINT('Ctrl Pts',(59.7126194350421,1.62960433959961,48.5));
#84229=CARTESIAN_POINT('Ctrl Pts',(59.7126194350421,1.62960433959961,48.35));
#84230=CARTESIAN_POINT('Ctrl Pts',(59.5010232441127,1.36248314380646,48.5));
#84231=CARTESIAN_POINT('Ctrl Pts',(59.5010232441127,1.36248314380646,48.35));
#84232=CARTESIAN_POINT('Ctrl Pts',(59.1348570100963,1.36248314380646,48.5));
#84233=CARTESIAN_POINT('Ctrl Pts',(59.1348570100963,1.36248314380646,48.35));
#84234=CARTESIAN_POINT('',(59.7126194350421,1.62960433959961,48.5));
#84235=CARTESIAN_POINT('Ctrl Pts',(59.7126194350421,1.62960433959961,48.5));
#84236=CARTESIAN_POINT('Ctrl Pts',(59.5010232441127,1.36248314380646,48.5));
#84237=CARTESIAN_POINT('Ctrl Pts',(59.1348570100963,1.36248314380646,48.5));
#84238=CARTESIAN_POINT('',(59.7126194350421,1.62960433959961,48.35));
#84239=CARTESIAN_POINT('',(59.7126194350421,1.62960433959961,48.5));
#84240=CARTESIAN_POINT('Ctrl Pts',(59.7126194350421,1.62960433959961,48.35));
#84241=CARTESIAN_POINT('Ctrl Pts',(59.5010232441127,1.36248314380646,48.35));
#84242=CARTESIAN_POINT('Ctrl Pts',(59.1348570100963,1.36248314380646,48.35));
#84243=CARTESIAN_POINT('Ctrl Pts',(59.8866986744106,2.14583912491798,48.5));
#84244=CARTESIAN_POINT('Ctrl Pts',(59.8866986744106,2.14583912491798,48.35));
#84245=CARTESIAN_POINT('Ctrl Pts',(59.8866986744106,1.84720331430435,48.5));
#84246=CARTESIAN_POINT('Ctrl Pts',(59.8866986744106,1.84720331430435,48.35));
#84247=CARTESIAN_POINT('Ctrl Pts',(59.7126194350421,1.62960433959961,48.5));
#84248=CARTESIAN_POINT('Ctrl Pts',(59.7126194350421,1.62960433959961,48.35));
#84249=CARTESIAN_POINT('',(59.8866986744106,2.14583912491798,48.5));
#84250=CARTESIAN_POINT('Ctrl Pts',(59.8866986744106,2.14583912491798,48.5));
#84251=CARTESIAN_POINT('Ctrl Pts',(59.8866986744106,1.84720331430435,48.5));
#84252=CARTESIAN_POINT('Ctrl Pts',(59.7126194350421,1.62960433959961,48.5));
#84253=CARTESIAN_POINT('',(59.8866986744106,2.14583912491798,48.35));
#84254=CARTESIAN_POINT('',(59.8866986744106,2.14583912491798,48.5));
#84255=CARTESIAN_POINT('Ctrl Pts',(59.8866986744106,2.14583912491798,48.35));
#84256=CARTESIAN_POINT('Ctrl Pts',(59.8866986744106,1.84720331430435,48.35));
#84257=CARTESIAN_POINT('Ctrl Pts',(59.7126194350421,1.62960433959961,48.35));
#84258=CARTESIAN_POINT('Ctrl Pts',(59.688608597964,2.65907236933708,48.5));
#84259=CARTESIAN_POINT('Ctrl Pts',(59.688608597964,2.65907236933708,48.35));
#84260=CARTESIAN_POINT('Ctrl Pts',(59.8866986744106,2.45948159694672,48.5));
#84261=CARTESIAN_POINT('Ctrl Pts',(59.8866986744106,2.45948159694672,48.35));
#84262=CARTESIAN_POINT('Ctrl Pts',(59.8866986744106,2.14583912491798,48.5));
#84263=CARTESIAN_POINT('Ctrl Pts',(59.8866986744106,2.14583912491798,48.35));
#84264=CARTESIAN_POINT('',(59.688608597964,2.65907236933708,48.5));
#84265=CARTESIAN_POINT('Ctrl Pts',(59.688608597964,2.65907236933708,48.5));
#84266=CARTESIAN_POINT('Ctrl Pts',(59.8866986744106,2.45948159694672,48.5));
#84267=CARTESIAN_POINT('Ctrl Pts',(59.8866986744106,2.14583912491798,48.5));
#84268=CARTESIAN_POINT('',(59.688608597964,2.65907236933708,48.35));
#84269=CARTESIAN_POINT('',(59.688608597964,2.65907236933708,48.5));
#84270=CARTESIAN_POINT('Ctrl Pts',(59.688608597964,2.65907236933708,48.35));
#84271=CARTESIAN_POINT('Ctrl Pts',(59.8866986744106,2.45948159694672,48.35));
#84272=CARTESIAN_POINT('Ctrl Pts',(59.8866986744106,2.14583912491798,48.35));
#84273=CARTESIAN_POINT('Ctrl Pts',(59.2023875825107,2.85866314172745,48.5));
#84274=CARTESIAN_POINT('Ctrl Pts',(59.2023875825107,2.85866314172745,48.35));
#84275=CARTESIAN_POINT('Ctrl Pts',(59.4905185215175,2.85866314172745,48.5));
#84276=CARTESIAN_POINT('Ctrl Pts',(59.4905185215175,2.85866314172745,48.35));
#84277=CARTESIAN_POINT('Ctrl Pts',(59.688608597964,2.65907236933708,48.5));
#84278=CARTESIAN_POINT('Ctrl Pts',(59.688608597964,2.65907236933708,48.35));
#84279=CARTESIAN_POINT('',(59.2023875825107,2.85866314172745,48.5));
#84280=CARTESIAN_POINT('Ctrl Pts',(59.2023875825107,2.85866314172745,48.5));
#84281=CARTESIAN_POINT('Ctrl Pts',(59.4905185215175,2.85866314172745,48.5));
#84282=CARTESIAN_POINT('Ctrl Pts',(59.688608597964,2.65907236933708,48.5));
#84283=CARTESIAN_POINT('',(59.2023875825107,2.85866314172745,48.35));
#84284=CARTESIAN_POINT('',(59.2023875825107,2.85866314172745,48.5));
#84285=CARTESIAN_POINT('Ctrl Pts',(59.2023875825107,2.85866314172745,48.35));
#84286=CARTESIAN_POINT('Ctrl Pts',(59.4905185215175,2.85866314172745,48.35));
#84287=CARTESIAN_POINT('Ctrl Pts',(59.688608597964,2.65907236933708,48.35));
#84288=CARTESIAN_POINT('Ctrl Pts',(58.786698680371,2.72060030698776,48.5));
#84289=CARTESIAN_POINT('Ctrl Pts',(58.786698680371,2.72060030698776,48.35));
#84290=CARTESIAN_POINT('Ctrl Pts',(58.984788607806,2.85866314172745,48.5));
#84291=CARTESIAN_POINT('Ctrl Pts',(58.984788607806,2.85866314172745,48.35));
#84292=CARTESIAN_POINT('Ctrl Pts',(59.2023875825107,2.85866314172745,48.5));
#84293=CARTESIAN_POINT('Ctrl Pts',(59.2023875825107,2.85866314172745,48.35));
#84294=CARTESIAN_POINT('',(58.786698680371,2.72060030698776,48.5));
#84295=CARTESIAN_POINT('Ctrl Pts',(58.786698680371,2.72060030698776,48.5));
#84296=CARTESIAN_POINT('Ctrl Pts',(58.984788607806,2.85866314172745,48.5));
#84297=CARTESIAN_POINT('Ctrl Pts',(59.2023875825107,2.85866314172745,48.5));
#84298=CARTESIAN_POINT('',(58.786698680371,2.72060030698776,48.35));
#84299=CARTESIAN_POINT('',(58.786698680371,2.72060030698776,48.5));
#84300=CARTESIAN_POINT('Ctrl Pts',(58.786698680371,2.72060030698776,48.35));
#84301=CARTESIAN_POINT('Ctrl Pts',(58.984788607806,2.85866314172745,48.35));
#84302=CARTESIAN_POINT('Ctrl Pts',(59.2023875825107,2.85866314172745,48.35));
#84303=CARTESIAN_POINT('Origin',(58.9052524678409,3.31186899542809,48.5));
#84304=CARTESIAN_POINT('',(58.9052524678409,3.31186899542809,48.5));
#84305=CARTESIAN_POINT('',(58.2187630699928,-0.111890755790727,48.5));
#84306=CARTESIAN_POINT('',(58.9052524678409,3.31186899542809,48.35));
#84307=CARTESIAN_POINT('',(58.9052524678409,3.31186899542809,48.5));
#84308=CARTESIAN_POINT('',(58.9052524678409,3.31186899542809,48.35));
#84309=CARTESIAN_POINT('Origin',(59.7831513993442,3.31186899542809,48.5));
#84310=CARTESIAN_POINT('',(59.7831513993442,3.31186899542809,48.5));
#84311=CARTESIAN_POINT('',(29.8915756996721,3.31186899542809,48.5));
#84312=CARTESIAN_POINT('',(59.7831513993442,3.31186899542809,48.35));
#84313=CARTESIAN_POINT('',(59.7831513993442,3.31186899542809,48.5));
#84314=CARTESIAN_POINT('',(59.7831513993442,3.31186899542809,48.35));
#84315=CARTESIAN_POINT('Origin',(59.7831513993442,3.56998646259308,48.5));
#84316=CARTESIAN_POINT('',(59.7831513993442,3.56998646259308,48.5));
#84317=CARTESIAN_POINT('',(59.7831513993442,5.78499323129654,48.5));
#84318=CARTESIAN_POINT('',(59.7831513993442,3.56998646259308,48.35));
#84319=CARTESIAN_POINT('',(59.7831513993442,3.56998646259308,48.5));
#84320=CARTESIAN_POINT('',(59.7831513993442,3.56998646259308,48.35));
#84321=CARTESIAN_POINT('Origin',(58.6891543380916,3.56998646259308,48.5));
#84322=CARTESIAN_POINT('',(58.6891543380916,3.56998646259308,48.5));
#84323=CARTESIAN_POINT('',(29.3445771690458,3.56998646259308,48.5));
#84324=CARTESIAN_POINT('',(58.6891543380916,3.56998646259308,48.35));
#84325=CARTESIAN_POINT('',(58.6891543380916,3.56998646259308,48.5));
#84326=CARTESIAN_POINT('',(58.6891543380916,3.56998646259308,48.35));
#84327=CARTESIAN_POINT('Origin',(58.4760574512184,2.43997284770012,48.5));
#84328=CARTESIAN_POINT('',(58.4760574512184,2.43997284770012,48.5));
#84329=CARTESIAN_POINT('',(57.9782484572375,-0.199816729090836,48.5));
#84330=CARTESIAN_POINT('',(58.4760574512184,2.43997284770012,48.35));
#84331=CARTESIAN_POINT('',(58.4760574512184,2.43997284770012,48.5));
#84332=CARTESIAN_POINT('',(58.4760574512184,2.43997284770012,48.35));
#84333=CARTESIAN_POINT('Origin',(58.7296726815403,2.40695783495903,48.5));
#84334=CARTESIAN_POINT('',(58.7296726815403,2.40695783495903,48.5));
#84335=CARTESIAN_POINT('',(29.4961884529084,6.21250158345456,48.5));
#84336=CARTESIAN_POINT('',(58.7296726815403,2.40695783495903,48.35));
#84337=CARTESIAN_POINT('',(58.7296726815403,2.40695783495903,48.5));
#84338=CARTESIAN_POINT('',(58.7296726815403,2.40695783495903,48.35));
#84339=CARTESIAN_POINT('Ctrl Pts',(58.8947477452457,2.56077775359154,48.5));
#84340=CARTESIAN_POINT('Ctrl Pts',(58.8947477452457,2.56077775359154,48.35));
#84341=CARTESIAN_POINT('Ctrl Pts',(58.7897000722587,2.5015007853508,48.5));
#84342=CARTESIAN_POINT('Ctrl Pts',(58.7897000722587,2.5015007853508,48.35));
#84343=CARTESIAN_POINT('Ctrl Pts',(58.7296726815403,2.40695783495903,48.5));
#84344=CARTESIAN_POINT('Ctrl Pts',(58.7296726815403,2.40695783495903,48.35));
#84345=CARTESIAN_POINT('',(58.8947477452457,2.56077775359154,48.5));
#84346=CARTESIAN_POINT('Ctrl Pts',(58.8947477452457,2.56077775359154,48.5));
#84347=CARTESIAN_POINT('Ctrl Pts',(58.7897000722587,2.5015007853508,48.5));
#84348=CARTESIAN_POINT('Ctrl Pts',(58.7296726815403,2.40695783495903,48.5));
#84349=CARTESIAN_POINT('',(58.8947477452457,2.56077775359154,48.35));
#84350=CARTESIAN_POINT('',(58.8947477452457,2.56077775359154,48.5));
#84351=CARTESIAN_POINT('Ctrl Pts',(58.8947477452457,2.56077775359154,48.35));
#84352=CARTESIAN_POINT('Ctrl Pts',(58.7897000722587,2.5015007853508,48.35));
#84353=CARTESIAN_POINT('Ctrl Pts',(58.7296726815403,2.40695783495903,48.35));
#84354=CARTESIAN_POINT('Ctrl Pts',(59.1303547732532,2.62005472183228,48.5));
#84355=CARTESIAN_POINT('Ctrl Pts',(59.1303547732532,2.62005472183228,48.35));
#84356=CARTESIAN_POINT('Ctrl Pts',(58.9997955672443,2.62005472183228,48.5));
#84357=CARTESIAN_POINT('Ctrl Pts',(58.9997955672443,2.62005472183228,48.35));
#84358=CARTESIAN_POINT('Ctrl Pts',(58.8947477452457,2.56077775359154,48.5));
#84359=CARTESIAN_POINT('Ctrl Pts',(58.8947477452457,2.56077775359154,48.35));
#84360=CARTESIAN_POINT('',(59.1303547732532,2.62005472183228,48.5));
#84361=CARTESIAN_POINT('Ctrl Pts',(59.1303547732532,2.62005472183228,48.5));
#84362=CARTESIAN_POINT('Ctrl Pts',(58.9997955672443,2.62005472183228,48.5));
#84363=CARTESIAN_POINT('Ctrl Pts',(58.8947477452457,2.56077775359154,48.5));
#84364=CARTESIAN_POINT('',(59.1303547732532,2.62005472183228,48.35));
#84365=CARTESIAN_POINT('',(59.1303547732532,2.62005472183228,48.5));
#84366=CARTESIAN_POINT('Ctrl Pts',(59.1303547732532,2.62005472183228,48.35));
#84367=CARTESIAN_POINT('Ctrl Pts',(58.9997955672443,2.62005472183228,48.35));
#84368=CARTESIAN_POINT('Ctrl Pts',(58.8947477452457,2.56077775359154,48.35));
#84369=CARTESIAN_POINT('Ctrl Pts',(59.4702592007816,2.48649397492409,48.5));
#84370=CARTESIAN_POINT('Ctrl Pts',(59.4702592007816,2.48649397492409,48.35));
#84371=CARTESIAN_POINT('Ctrl Pts',(59.3404504172504,2.62005472183228,48.5));
#84372=CARTESIAN_POINT('Ctrl Pts',(59.3404504172504,2.62005472183228,48.35));
#84373=CARTESIAN_POINT('Ctrl Pts',(59.1303547732532,2.62005472183228,48.5));
#84374=CARTESIAN_POINT('Ctrl Pts',(59.1303547732532,2.62005472183228,48.35));
#84375=CARTESIAN_POINT('',(59.4702592007816,2.48649397492409,48.5));
#84376=CARTESIAN_POINT('Ctrl Pts',(59.4702592007816,2.48649397492409,48.5));
#84377=CARTESIAN_POINT('Ctrl Pts',(59.3404504172504,2.62005472183228,48.5));
#84378=CARTESIAN_POINT('Ctrl Pts',(59.1303547732532,2.62005472183228,48.5));
#84379=CARTESIAN_POINT('',(59.4702592007816,2.48649397492409,48.35));
#84380=CARTESIAN_POINT('',(59.4702592007816,2.48649397492409,48.5));
#84381=CARTESIAN_POINT('Ctrl Pts',(59.4702592007816,2.48649397492409,48.35));
#84382=CARTESIAN_POINT('Ctrl Pts',(59.3404504172504,2.62005472183228,48.35));
#84383=CARTESIAN_POINT('Ctrl Pts',(59.1303547732532,2.62005472183228,48.35));
#84384=CARTESIAN_POINT('Ctrl Pts',(59.6000685803592,2.12182813882828,48.5));
#84385=CARTESIAN_POINT('Ctrl Pts',(59.6000685803592,2.12182813882828,48.35));
#84386=CARTESIAN_POINT('Ctrl Pts',(59.6000685803592,2.3529332280159,48.5));
#84387=CARTESIAN_POINT('Ctrl Pts',(59.6000685803592,2.3529332280159,48.35));
#84388=CARTESIAN_POINT('Ctrl Pts',(59.4702592007816,2.48649397492409,48.5));
#84389=CARTESIAN_POINT('Ctrl Pts',(59.4702592007816,2.48649397492409,48.35));
#84390=CARTESIAN_POINT('',(59.6000685803592,2.12182813882828,48.5));
#84391=CARTESIAN_POINT('Ctrl Pts',(59.6000685803592,2.12182813882828,48.5));
#84392=CARTESIAN_POINT('Ctrl Pts',(59.6000685803592,2.3529332280159,48.5));
#84393=CARTESIAN_POINT('Ctrl Pts',(59.4702592007816,2.48649397492409,48.5));
#84394=CARTESIAN_POINT('',(59.6000685803592,2.12182813882828,48.35));
#84395=CARTESIAN_POINT('',(59.6000685803592,2.12182813882828,48.5));
#84396=CARTESIAN_POINT('Ctrl Pts',(59.6000685803592,2.12182813882828,48.35));
#84397=CARTESIAN_POINT('Ctrl Pts',(59.6000685803592,2.3529332280159,48.35));
#84398=CARTESIAN_POINT('Ctrl Pts',(59.4702592007816,2.48649397492409,48.35));
#84399=CARTESIAN_POINT('Ctrl Pts',(59.465006839484,1.73165076971054,48.5));
#84400=CARTESIAN_POINT('Ctrl Pts',(59.465006839484,1.73165076971054,48.35));
#84401=CARTESIAN_POINT('Ctrl Pts',(59.6000685803592,1.87871778011322,48.5));
#84402=CARTESIAN_POINT('Ctrl Pts',(59.6000685803592,1.87871778011322,48.35));
#84403=CARTESIAN_POINT('Ctrl Pts',(59.6000685803592,2.12182813882828,48.5));
#84404=CARTESIAN_POINT('Ctrl Pts',(59.6000685803592,2.12182813882828,48.35));
#84405=CARTESIAN_POINT('',(59.465006839484,1.73165076971054,48.5));
#84406=CARTESIAN_POINT('Ctrl Pts',(59.465006839484,1.73165076971054,48.5));
#84407=CARTESIAN_POINT('Ctrl Pts',(59.6000685803592,1.87871778011322,48.5));
#84408=CARTESIAN_POINT('Ctrl Pts',(59.6000685803592,2.12182813882828,48.5));
#84409=CARTESIAN_POINT('',(59.465006839484,1.73165076971054,48.35));
#84410=CARTESIAN_POINT('',(59.465006839484,1.73165076971054,48.5));
#84411=CARTESIAN_POINT('Ctrl Pts',(59.465006839484,1.73165076971054,48.35));
#84412=CARTESIAN_POINT('Ctrl Pts',(59.6000685803592,1.87871778011322,48.35));
#84413=CARTESIAN_POINT('Ctrl Pts',(59.6000685803592,2.12182813882828,48.35));
#84414=CARTESIAN_POINT('Ctrl Pts',(59.1348570100963,1.58458405733109,48.5));
#84415=CARTESIAN_POINT('Ctrl Pts',(59.1348570100963,1.58458405733109,48.35));
#84416=CARTESIAN_POINT('Ctrl Pts',(59.3299455456436,1.58458405733109,48.5));
#84417=CARTESIAN_POINT('Ctrl Pts',(59.3299455456436,1.58458405733109,48.35));
#84418=CARTESIAN_POINT('Ctrl Pts',(59.465006839484,1.73165076971054,48.5));
#84419=CARTESIAN_POINT('Ctrl Pts',(59.465006839484,1.73165076971054,48.35));
#84420=CARTESIAN_POINT('',(59.1348570100963,1.58458405733109,48.5));
#84421=CARTESIAN_POINT('Ctrl Pts',(59.1348570100963,1.58458405733109,48.5));
#84422=CARTESIAN_POINT('Ctrl Pts',(59.3299455456436,1.58458405733109,48.5));
#84423=CARTESIAN_POINT('Ctrl Pts',(59.465006839484,1.73165076971054,48.5));
#84424=CARTESIAN_POINT('',(59.1348570100963,1.58458405733109,48.35));
#84425=CARTESIAN_POINT('',(59.1348570100963,1.58458405733109,48.5));
#84426=CARTESIAN_POINT('Ctrl Pts',(59.1348570100963,1.58458405733109,48.35));
#84427=CARTESIAN_POINT('Ctrl Pts',(59.3299455456436,1.58458405733109,48.35));
#84428=CARTESIAN_POINT('Ctrl Pts',(59.465006839484,1.73165076971054,48.35));
#84429=CARTESIAN_POINT('Ctrl Pts',(58.8579810671508,1.68888145685196,48.5));
#84430=CARTESIAN_POINT('Ctrl Pts',(58.8579810671508,1.68888145685196,48.35));
#84431=CARTESIAN_POINT('Ctrl Pts',(58.9727833382785,1.58458405733109,48.5));
#84432=CARTESIAN_POINT('Ctrl Pts',(58.9727833382785,1.58458405733109,48.35));
#84433=CARTESIAN_POINT('Ctrl Pts',(59.1348570100963,1.58458405733109,48.5));
#84434=CARTESIAN_POINT('Ctrl Pts',(59.1348570100963,1.58458405733109,48.35));
#84435=CARTESIAN_POINT('',(58.8579810671508,1.68888145685196,48.5));
#84436=CARTESIAN_POINT('Ctrl Pts',(58.8579810671508,1.68888145685196,48.5));
#84437=CARTESIAN_POINT('Ctrl Pts',(58.9727833382785,1.58458405733109,48.5));
#84438=CARTESIAN_POINT('Ctrl Pts',(59.1348570100963,1.58458405733109,48.5));
#84439=CARTESIAN_POINT('',(58.8579810671508,1.68888145685196,48.35));
#84440=CARTESIAN_POINT('',(58.8579810671508,1.68888145685196,48.5));
#84441=CARTESIAN_POINT('Ctrl Pts',(58.8579810671508,1.68888145685196,48.35));
#84442=CARTESIAN_POINT('Ctrl Pts',(58.9727833382785,1.58458405733109,48.35));
#84443=CARTESIAN_POINT('Ctrl Pts',(59.1348570100963,1.58458405733109,48.35));
#84444=CARTESIAN_POINT('Ctrl Pts',(58.7116646282375,2.00027281045914,48.5));
#84445=CARTESIAN_POINT('Ctrl Pts',(58.7116646282375,2.00027281045914,48.35));
#84446=CARTESIAN_POINT('Ctrl Pts',(58.7431787960231,1.79317885637283,48.5));
#84447=CARTESIAN_POINT('Ctrl Pts',(58.7431787960231,1.79317885637283,48.35));
#84448=CARTESIAN_POINT('Ctrl Pts',(58.8579810671508,1.68888145685196,48.5));
#84449=CARTESIAN_POINT('Ctrl Pts',(58.8579810671508,1.68888145685196,48.35));
#84450=CARTESIAN_POINT('',(58.7116646282375,2.00027281045914,48.5));
#84451=CARTESIAN_POINT('Ctrl Pts',(58.7116646282375,2.00027281045914,48.5));
#84452=CARTESIAN_POINT('Ctrl Pts',(58.7431787960231,1.79317885637283,48.5));
#84453=CARTESIAN_POINT('Ctrl Pts',(58.8579810671508,1.68888145685196,48.5));
#84454=CARTESIAN_POINT('',(58.7116646282375,2.00027281045914,48.35));
#84455=CARTESIAN_POINT('',(58.7116646282375,2.00027281045914,48.5));
#84456=CARTESIAN_POINT('Ctrl Pts',(58.7116646282375,2.00027281045914,48.35));
#84457=CARTESIAN_POINT('Ctrl Pts',(58.7431787960231,1.79317885637283,48.35));
#84458=CARTESIAN_POINT('Ctrl Pts',(58.8579810671508,1.68888145685196,48.35));
#84459=CARTESIAN_POINT('Origin',(58.4280356280506,1.97626197338104,48.5));
#84460=CARTESIAN_POINT('',(58.4280356280506,1.97626197338104,48.5));
#84461=CARTESIAN_POINT('',(29.6750511830058,-0.457844639708494,48.5));
#84462=CARTESIAN_POINT('',(58.4280356280506,1.97626197338104,48.35));
#84463=CARTESIAN_POINT('',(58.4280356280506,1.97626197338104,48.5));
#84464=CARTESIAN_POINT('',(58.4280356280506,1.97626197338104,48.35));
#84465=CARTESIAN_POINT('Ctrl Pts',(58.6448841802776,1.53055930137634,48.5));
#84466=CARTESIAN_POINT('Ctrl Pts',(58.6448841802776,1.53055930137634,48.35));
#84467=CARTESIAN_POINT('Ctrl Pts',(58.4550478570163,1.69863575696945,48.5));
#84468=CARTESIAN_POINT('Ctrl Pts',(58.4550478570163,1.69863575696945,48.35));
#84469=CARTESIAN_POINT('Ctrl Pts',(58.4280356280506,1.97626197338104,48.5));
#84470=CARTESIAN_POINT('Ctrl Pts',(58.4280356280506,1.97626197338104,48.35));
#84471=CARTESIAN_POINT('Ctrl Pts',(58.6448841802776,1.53055930137634,48.5));
#84472=CARTESIAN_POINT('Ctrl Pts',(58.4550478570163,1.69863575696945,48.5));
#84473=CARTESIAN_POINT('Ctrl Pts',(58.4280356280506,1.97626197338104,48.5));
#84474=CARTESIAN_POINT('Ctrl Pts',(58.6448841802776,1.53055930137634,48.35));
#84475=CARTESIAN_POINT('Ctrl Pts',(58.4550478570163,1.69863575696945,48.35));
#84476=CARTESIAN_POINT('Ctrl Pts',(58.4280356280506,1.97626197338104,48.35));
#84477=CARTESIAN_POINT('Origin',(59.9999999515712,2.48574362695217,48.35));
#84478=CARTESIAN_POINT('Origin',(0.,8.,48.5));
#84479=CARTESIAN_POINT('Ctrl Pts',(50.8576400466263,3.38540250062943,48.5));
#84480=CARTESIAN_POINT('Ctrl Pts',(50.8576400466263,3.38540250062943,48.35));
#84481=CARTESIAN_POINT('Ctrl Pts',(50.6715552397072,3.38540250062943,48.5));
#84482=CARTESIAN_POINT('Ctrl Pts',(50.6715552397072,3.38540250062943,48.35));
#84483=CARTESIAN_POINT('Ctrl Pts',(50.5605049319565,3.22783091664314,48.5));
#84484=CARTESIAN_POINT('Ctrl Pts',(50.5605049319565,3.22783091664314,48.35));
#84485=CARTESIAN_POINT('',(50.8576400466263,3.38540250062943,48.5));
#84486=CARTESIAN_POINT('',(50.5605049319565,3.22783091664314,48.5));
#84487=CARTESIAN_POINT('Ctrl Pts',(50.8576400466263,3.38540250062943,48.5));
#84488=CARTESIAN_POINT('Ctrl Pts',(50.6715552397072,3.38540250062943,48.5));
#84489=CARTESIAN_POINT('Ctrl Pts',(50.5605049319565,3.22783091664314,48.5));
#84490=CARTESIAN_POINT('',(50.8576400466263,3.38540250062943,48.35));
#84491=CARTESIAN_POINT('',(50.8576400466263,3.38540250062943,48.5));
#84492=CARTESIAN_POINT('',(50.5605049319565,3.22783091664314,48.35));
#84493=CARTESIAN_POINT('Ctrl Pts',(50.8576400466263,3.38540250062943,48.35));
#84494=CARTESIAN_POINT('Ctrl Pts',(50.6715552397072,3.38540250062943,48.35));
#84495=CARTESIAN_POINT('Ctrl Pts',(50.5605049319565,3.22783091664314,48.35));
#84496=CARTESIAN_POINT('',(50.5605049319565,3.22783091664314,48.5));
#84497=CARTESIAN_POINT('Ctrl Pts',(51.1735333390534,3.2068213224411,48.5));
#84498=CARTESIAN_POINT('Ctrl Pts',(51.1735333390534,3.2068213224411,48.35));
#84499=CARTESIAN_POINT('Ctrl Pts',(51.0467256493866,3.38540250062943,48.5));
#84500=CARTESIAN_POINT('Ctrl Pts',(51.0467256493866,3.38540250062943,48.35));
#84501=CARTESIAN_POINT('Ctrl Pts',(50.8576400466263,3.38540250062943,48.5));
#84502=CARTESIAN_POINT('Ctrl Pts',(50.8576400466263,3.38540250062943,48.35));
#84503=CARTESIAN_POINT('',(51.1735333390534,3.2068213224411,48.5));
#84504=CARTESIAN_POINT('Ctrl Pts',(51.1735333390534,3.2068213224411,48.5));
#84505=CARTESIAN_POINT('Ctrl Pts',(51.0467256493866,3.38540250062943,48.5));
#84506=CARTESIAN_POINT('Ctrl Pts',(50.8576400466263,3.38540250062943,48.5));
#84507=CARTESIAN_POINT('',(51.1735333390534,3.2068213224411,48.35));
#84508=CARTESIAN_POINT('',(51.1735333390534,3.2068213224411,48.5));
#84509=CARTESIAN_POINT('Ctrl Pts',(51.1735333390534,3.2068213224411,48.35));
#84510=CARTESIAN_POINT('Ctrl Pts',(51.0467256493866,3.38540250062943,48.35));
#84511=CARTESIAN_POINT('Ctrl Pts',(50.8576400466263,3.38540250062943,48.35));
#84512=CARTESIAN_POINT('Ctrl Pts',(51.3003410287201,2.48499327898026,48.5));
#84513=CARTESIAN_POINT('Ctrl Pts',(51.3003410287201,2.48499327898026,48.35));
#84514=CARTESIAN_POINT('Ctrl Pts',(51.3003410287201,3.02824014425278,48.5));
#84515=CARTESIAN_POINT('Ctrl Pts',(51.3003410287201,3.02824014425278,48.35));
#84516=CARTESIAN_POINT('Ctrl Pts',(51.1735333390534,3.2068213224411,48.5));
#84517=CARTESIAN_POINT('Ctrl Pts',(51.1735333390534,3.2068213224411,48.35));
#84518=CARTESIAN_POINT('',(51.3003410287201,2.48499327898026,48.5));
#84519=CARTESIAN_POINT('Ctrl Pts',(51.3003410287201,2.48499327898026,48.5));
#84520=CARTESIAN_POINT('Ctrl Pts',(51.3003410287201,3.02824014425278,48.5));
#84521=CARTESIAN_POINT('Ctrl Pts',(51.1735333390534,3.2068213224411,48.5));
#84522=CARTESIAN_POINT('',(51.3003410287201,2.48499327898026,48.35));
#84523=CARTESIAN_POINT('',(51.3003410287201,2.48499327898026,48.5));
#84524=CARTESIAN_POINT('Ctrl Pts',(51.3003410287201,2.48499327898026,48.35));
#84525=CARTESIAN_POINT('Ctrl Pts',(51.3003410287201,3.02824014425278,48.35));
#84526=CARTESIAN_POINT('Ctrl Pts',(51.1735333390534,3.2068213224411,48.35));
#84527=CARTESIAN_POINT('Ctrl Pts',(51.1735333390534,1.76466578245163,48.5));
#84528=CARTESIAN_POINT('Ctrl Pts',(51.1735333390534,1.76466578245163,48.35));
#84529=CARTESIAN_POINT('Ctrl Pts',(51.3003410287201,1.9447478055954,48.5));
#84530=CARTESIAN_POINT('Ctrl Pts',(51.3003410287201,1.9447478055954,48.35));
#84531=CARTESIAN_POINT('Ctrl Pts',(51.3003410287201,2.48499327898026,48.5));
#84532=CARTESIAN_POINT('Ctrl Pts',(51.3003410287201,2.48499327898026,48.35));
#84533=CARTESIAN_POINT('',(51.1735333390534,1.76466578245163,48.5));
#84534=CARTESIAN_POINT('Ctrl Pts',(51.1735333390534,1.76466578245163,48.5));
#84535=CARTESIAN_POINT('Ctrl Pts',(51.3003410287201,1.9447478055954,48.5));
#84536=CARTESIAN_POINT('Ctrl Pts',(51.3003410287201,2.48499327898026,48.5));
#84537=CARTESIAN_POINT('',(51.1735333390534,1.76466578245163,48.35));
#84538=CARTESIAN_POINT('',(51.1735333390534,1.76466578245163,48.5));
#84539=CARTESIAN_POINT('Ctrl Pts',(51.1735333390534,1.76466578245163,48.35));
#84540=CARTESIAN_POINT('Ctrl Pts',(51.3003410287201,1.9447478055954,48.35));
#84541=CARTESIAN_POINT('Ctrl Pts',(51.3003410287201,2.48499327898026,48.35));
#84542=CARTESIAN_POINT('Ctrl Pts',(50.8606411404908,1.58458405733109,48.5));
#84543=CARTESIAN_POINT('Ctrl Pts',(50.8606411404908,1.58458405733109,48.35));
#84544=CARTESIAN_POINT('Ctrl Pts',(51.0467256493866,1.58458405733109,48.5));
#84545=CARTESIAN_POINT('Ctrl Pts',(51.0467256493866,1.58458405733109,48.35));
#84546=CARTESIAN_POINT('Ctrl Pts',(51.1735333390534,1.76466578245163,48.5));
#84547=CARTESIAN_POINT('Ctrl Pts',(51.1735333390534,1.76466578245163,48.35));
#84548=CARTESIAN_POINT('',(50.8606411404908,1.58458405733109,48.5));
#84549=CARTESIAN_POINT('Ctrl Pts',(50.8606411404908,1.58458405733109,48.5));
#84550=CARTESIAN_POINT('Ctrl Pts',(51.0467256493866,1.58458405733109,48.5));
#84551=CARTESIAN_POINT('Ctrl Pts',(51.1735333390534,1.76466578245163,48.5));
#84552=CARTESIAN_POINT('',(50.8606411404908,1.58458405733109,48.35));
#84553=CARTESIAN_POINT('',(50.8606411404908,1.58458405733109,48.5));
#84554=CARTESIAN_POINT('Ctrl Pts',(50.8606411404908,1.58458405733109,48.35));
#84555=CARTESIAN_POINT('Ctrl Pts',(51.0467256493866,1.58458405733109,48.35));
#84556=CARTESIAN_POINT('Ctrl Pts',(51.1735333390534,1.76466578245163,48.35));
#84557=CARTESIAN_POINT('Ctrl Pts',(50.5477489419281,1.76391565799713,48.5));
#84558=CARTESIAN_POINT('Ctrl Pts',(50.5477489419281,1.76391565799713,48.35));
#84559=CARTESIAN_POINT('Ctrl Pts',(50.6745566315949,1.58458405733109,48.5));
#84560=CARTESIAN_POINT('Ctrl Pts',(50.6745566315949,1.58458405733109,48.35));
#84561=CARTESIAN_POINT('Ctrl Pts',(50.8606411404908,1.58458405733109,48.5));
#84562=CARTESIAN_POINT('Ctrl Pts',(50.8606411404908,1.58458405733109,48.35));
#84563=CARTESIAN_POINT('',(50.5477489419281,1.76391565799713,48.5));
#84564=CARTESIAN_POINT('Ctrl Pts',(50.5477489419281,1.76391565799713,48.5));
#84565=CARTESIAN_POINT('Ctrl Pts',(50.6745566315949,1.58458405733109,48.5));
#84566=CARTESIAN_POINT('Ctrl Pts',(50.8606411404908,1.58458405733109,48.5));
#84567=CARTESIAN_POINT('',(50.5477489419281,1.76391565799713,48.35));
#84568=CARTESIAN_POINT('',(50.5477489419281,1.76391565799713,48.5));
#84569=CARTESIAN_POINT('Ctrl Pts',(50.5477489419281,1.76391565799713,48.35));
#84570=CARTESIAN_POINT('Ctrl Pts',(50.6745566315949,1.58458405733109,48.35));
#84571=CARTESIAN_POINT('Ctrl Pts',(50.8606411404908,1.58458405733109,48.35));
#84572=CARTESIAN_POINT('Ctrl Pts',(50.4209412522614,2.48499327898026,48.5));
#84573=CARTESIAN_POINT('Ctrl Pts',(50.4209412522614,2.48499327898026,48.35));
#84574=CARTESIAN_POINT('Ctrl Pts',(50.4209412522614,1.94324696063995,48.5));
#84575=CARTESIAN_POINT('Ctrl Pts',(50.4209412522614,1.94324696063995,48.35));
#84576=CARTESIAN_POINT('Ctrl Pts',(50.5477489419281,1.76391565799713,48.5));
#84577=CARTESIAN_POINT('Ctrl Pts',(50.5477489419281,1.76391565799713,48.35));
#84578=CARTESIAN_POINT('',(50.4209412522614,2.48499327898026,48.5));
#84579=CARTESIAN_POINT('Ctrl Pts',(50.4209412522614,2.48499327898026,48.5));
#84580=CARTESIAN_POINT('Ctrl Pts',(50.4209412522614,1.94324696063995,48.5));
#84581=CARTESIAN_POINT('Ctrl Pts',(50.5477489419281,1.76391565799713,48.5));
#84582=CARTESIAN_POINT('',(50.4209412522614,2.48499327898026,48.35));
#84583=CARTESIAN_POINT('',(50.4209412522614,2.48499327898026,48.5));
#84584=CARTESIAN_POINT('Ctrl Pts',(50.4209412522614,2.48499327898026,48.35));
#84585=CARTESIAN_POINT('Ctrl Pts',(50.4209412522614,1.94324696063995,48.35));
#84586=CARTESIAN_POINT('Ctrl Pts',(50.5477489419281,1.76391565799713,48.35));
#84587=CARTESIAN_POINT('Ctrl Pts',(50.5605049319565,3.22783091664314,48.5));
#84588=CARTESIAN_POINT('Ctrl Pts',(50.5605049319565,3.22783091664314,48.35));
#84589=CARTESIAN_POINT('Ctrl Pts',(50.4209412522614,3.02673944830894,48.5));
#84590=CARTESIAN_POINT('Ctrl Pts',(50.4209412522614,3.02673944830894,48.35));
#84591=CARTESIAN_POINT('Ctrl Pts',(50.4209412522614,2.48499327898026,48.5));
#84592=CARTESIAN_POINT('Ctrl Pts',(50.4209412522614,2.48499327898026,48.35));
#84593=CARTESIAN_POINT('Ctrl Pts',(50.5605049319565,3.22783091664314,48.5));
#84594=CARTESIAN_POINT('Ctrl Pts',(50.4209412522614,3.02673944830894,48.5));
#84595=CARTESIAN_POINT('Ctrl Pts',(50.4209412522614,2.48499327898026,48.5));
#84596=CARTESIAN_POINT('Ctrl Pts',(50.5605049319565,3.22783091664314,48.35));
#84597=CARTESIAN_POINT('Ctrl Pts',(50.4209412522614,3.02673944830894,48.35));
#84598=CARTESIAN_POINT('Ctrl Pts',(50.4209412522614,2.48499327898026,48.35));
#84599=CARTESIAN_POINT('Ctrl Pts',(50.8606411404908,1.36248314380646,48.5));
#84600=CARTESIAN_POINT('Ctrl Pts',(50.8606411404908,1.36248314380646,48.35));
#84601=CARTESIAN_POINT('Ctrl Pts',(50.5424965806305,1.36248314380646,48.5));
#84602=CARTESIAN_POINT('Ctrl Pts',(50.5424965806305,1.36248314380646,48.35));
#84603=CARTESIAN_POINT('Ctrl Pts',(50.3609140105546,1.59058684110642,48.5));
#84604=CARTESIAN_POINT('Ctrl Pts',(50.3609140105546,1.59058684110642,48.35));
#84605=CARTESIAN_POINT('',(50.8606411404908,1.36248314380646,48.5));
#84606=CARTESIAN_POINT('',(50.3609140105546,1.59058684110642,48.5));
#84607=CARTESIAN_POINT('Ctrl Pts',(50.8606411404908,1.36248314380646,48.5));
#84608=CARTESIAN_POINT('Ctrl Pts',(50.5424965806305,1.36248314380646,48.5));
#84609=CARTESIAN_POINT('Ctrl Pts',(50.3609140105546,1.59058684110642,48.5));
#84610=CARTESIAN_POINT('',(50.8606411404908,1.36248314380646,48.35));
#84611=CARTESIAN_POINT('',(50.8606411404908,1.36248314380646,48.5));
#84612=CARTESIAN_POINT('',(50.3609140105546,1.59058684110642,48.35));
#84613=CARTESIAN_POINT('Ctrl Pts',(50.8606411404908,1.36248314380646,48.35));
#84614=CARTESIAN_POINT('Ctrl Pts',(50.5424965806305,1.36248314380646,48.35));
#84615=CARTESIAN_POINT('Ctrl Pts',(50.3609140105546,1.59058684110642,48.35));
#84616=CARTESIAN_POINT('',(50.3609140105546,1.59058684110642,48.5));
#84617=CARTESIAN_POINT('Ctrl Pts',(51.260572809726,1.49229192733765,48.5));
#84618=CARTESIAN_POINT('Ctrl Pts',(51.260572809726,1.49229192733765,48.35));
#84619=CARTESIAN_POINT('Ctrl Pts',(51.1022509522736,1.36248314380646,48.5));
#84620=CARTESIAN_POINT('Ctrl Pts',(51.1022509522736,1.36248314380646,48.35));
#84621=CARTESIAN_POINT('Ctrl Pts',(50.8606411404908,1.36248314380646,48.5));
#84622=CARTESIAN_POINT('Ctrl Pts',(50.8606411404908,1.36248314380646,48.35));
#84623=CARTESIAN_POINT('',(51.260572809726,1.49229192733765,48.5));
#84624=CARTESIAN_POINT('Ctrl Pts',(51.260572809726,1.49229192733765,48.5));
#84625=CARTESIAN_POINT('Ctrl Pts',(51.1022509522736,1.36248314380646,48.5));
#84626=CARTESIAN_POINT('Ctrl Pts',(50.8606411404908,1.36248314380646,48.5));
#84627=CARTESIAN_POINT('',(51.260572809726,1.49229192733765,48.35));
#84628=CARTESIAN_POINT('',(51.260572809726,1.49229192733765,48.5));
#84629=CARTESIAN_POINT('Ctrl Pts',(51.260572809726,1.49229192733765,48.35));
#84630=CARTESIAN_POINT('Ctrl Pts',(51.1022509522736,1.36248314380646,48.35));
#84631=CARTESIAN_POINT('Ctrl Pts',(50.8606411404908,1.36248314380646,48.35));
#84632=CARTESIAN_POINT('Ctrl Pts',(51.4984311051667,1.85995900630951,48.5));
#84633=CARTESIAN_POINT('Ctrl Pts',(51.4984311051667,1.85995900630951,48.35));
#84634=CARTESIAN_POINT('Ctrl Pts',(51.4188946671784,1.62210100889206,48.5));
#84635=CARTESIAN_POINT('Ctrl Pts',(51.4188946671784,1.62210100889206,48.35));
#84636=CARTESIAN_POINT('Ctrl Pts',(51.260572809726,1.49229192733765,48.5));
#84637=CARTESIAN_POINT('Ctrl Pts',(51.260572809726,1.49229192733765,48.35));
#84638=CARTESIAN_POINT('',(51.4984311051667,1.85995900630951,48.5));
#84639=CARTESIAN_POINT('Ctrl Pts',(51.4984311051667,1.85995900630951,48.5));
#84640=CARTESIAN_POINT('Ctrl Pts',(51.4188946671784,1.62210100889206,48.5));
#84641=CARTESIAN_POINT('Ctrl Pts',(51.260572809726,1.49229192733765,48.5));
#84642=CARTESIAN_POINT('',(51.4984311051667,1.85995900630951,48.35));
#84643=CARTESIAN_POINT('',(51.4984311051667,1.85995900630951,48.5));
#84644=CARTESIAN_POINT('Ctrl Pts',(51.4984311051667,1.85995900630951,48.35));
#84645=CARTESIAN_POINT('Ctrl Pts',(51.4188946671784,1.62210100889206,48.35));
#84646=CARTESIAN_POINT('Ctrl Pts',(51.260572809726,1.49229192733765,48.35));
#84647=CARTESIAN_POINT('Ctrl Pts',(51.5779669471085,2.48499327898026,48.5));
#84648=CARTESIAN_POINT('Ctrl Pts',(51.5779669471085,2.48499327898026,48.35));
#84649=CARTESIAN_POINT('Ctrl Pts',(51.5779669471085,2.09781730175018,48.5));
#84650=CARTESIAN_POINT('Ctrl Pts',(51.5779669471085,2.09781730175018,48.35));
#84651=CARTESIAN_POINT('Ctrl Pts',(51.4984311051667,1.85995900630951,48.5));
#84652=CARTESIAN_POINT('Ctrl Pts',(51.4984311051667,1.85995900630951,48.35));
#84653=CARTESIAN_POINT('',(51.5779669471085,2.48499327898026,48.5));
#84654=CARTESIAN_POINT('Ctrl Pts',(51.5779669471085,2.48499327898026,48.5));
#84655=CARTESIAN_POINT('Ctrl Pts',(51.5779669471085,2.09781730175018,48.5));
#84656=CARTESIAN_POINT('Ctrl Pts',(51.4984311051667,1.85995900630951,48.5));
#84657=CARTESIAN_POINT('',(51.5779669471085,2.48499327898026,48.35));
#84658=CARTESIAN_POINT('',(51.5779669471085,2.48499327898026,48.5));
#84659=CARTESIAN_POINT('Ctrl Pts',(51.5779669471085,2.48499327898026,48.35));
#84660=CARTESIAN_POINT('Ctrl Pts',(51.5779669471085,2.09781730175018,48.35));
#84661=CARTESIAN_POINT('Ctrl Pts',(51.4984311051667,1.85995900630951,48.35));
#84662=CARTESIAN_POINT('Ctrl Pts',(51.5284444279969,3.00497958064079,48.5));
#84663=CARTESIAN_POINT('Ctrl Pts',(51.5284444279969,3.00497958064079,48.35));
#84664=CARTESIAN_POINT('Ctrl Pts',(51.5779669471085,2.81214186549187,48.5));
#84665=CARTESIAN_POINT('Ctrl Pts',(51.5779669471085,2.81214186549187,48.35));
#84666=CARTESIAN_POINT('Ctrl Pts',(51.5779669471085,2.48499327898026,48.5));
#84667=CARTESIAN_POINT('Ctrl Pts',(51.5779669471085,2.48499327898026,48.35));
#84668=CARTESIAN_POINT('',(51.5284444279969,3.00497958064079,48.5));
#84669=CARTESIAN_POINT('Ctrl Pts',(51.5284444279969,3.00497958064079,48.5));
#84670=CARTESIAN_POINT('Ctrl Pts',(51.5779669471085,2.81214186549187,48.5));
#84671=CARTESIAN_POINT('Ctrl Pts',(51.5779669471085,2.48499327898026,48.5));
#84672=CARTESIAN_POINT('',(51.5284444279969,3.00497958064079,48.35));
#84673=CARTESIAN_POINT('',(51.5284444279969,3.00497958064079,48.5));
#84674=CARTESIAN_POINT('Ctrl Pts',(51.5284444279969,3.00497958064079,48.35));
#84675=CARTESIAN_POINT('Ctrl Pts',(51.5779669471085,2.81214186549187,48.35));
#84676=CARTESIAN_POINT('Ctrl Pts',(51.5779669471085,2.48499327898026,48.35));
#84677=CARTESIAN_POINT('Ctrl Pts',(51.3918824382126,3.33212831616402,48.5));
#84678=CARTESIAN_POINT('Ctrl Pts',(51.3918824382126,3.33212831616402,48.35));
#84679=CARTESIAN_POINT('Ctrl Pts',(51.4789219088852,3.19781729578972,48.5));
#84680=CARTESIAN_POINT('Ctrl Pts',(51.4789219088852,3.19781729578972,48.35));
#84681=CARTESIAN_POINT('Ctrl Pts',(51.5284444279969,3.00497958064079,48.5));
#84682=CARTESIAN_POINT('Ctrl Pts',(51.5284444279969,3.00497958064079,48.35));
#84683=CARTESIAN_POINT('',(51.3918824382126,3.33212831616402,48.5));
#84684=CARTESIAN_POINT('Ctrl Pts',(51.3918824382126,3.33212831616402,48.5));
#84685=CARTESIAN_POINT('Ctrl Pts',(51.4789219088852,3.19781729578972,48.5));
#84686=CARTESIAN_POINT('Ctrl Pts',(51.5284444279969,3.00497958064079,48.5));
#84687=CARTESIAN_POINT('',(51.3918824382126,3.33212831616402,48.35));
#84688=CARTESIAN_POINT('',(51.3918824382126,3.33212831616402,48.5));
#84689=CARTESIAN_POINT('Ctrl Pts',(51.3918824382126,3.33212831616402,48.35));
#84690=CARTESIAN_POINT('Ctrl Pts',(51.4789219088852,3.19781729578972,48.35));
#84691=CARTESIAN_POINT('Ctrl Pts',(51.5284444279969,3.00497958064079,48.35));
#84692=CARTESIAN_POINT('Ctrl Pts',(51.1712826676667,3.5377217233181,48.5));
#84693=CARTESIAN_POINT('Ctrl Pts',(51.1712826676667,3.5377217233181,48.35));
#84694=CARTESIAN_POINT('Ctrl Pts',(51.30484296754,3.46643933653831,48.5));
#84695=CARTESIAN_POINT('Ctrl Pts',(51.30484296754,3.46643933653831,48.35));
#84696=CARTESIAN_POINT('Ctrl Pts',(51.3918824382126,3.33212831616402,48.5));
#84697=CARTESIAN_POINT('Ctrl Pts',(51.3918824382126,3.33212831616402,48.35));
#84698=CARTESIAN_POINT('',(51.1712826676667,3.5377217233181,48.5));
#84699=CARTESIAN_POINT('Ctrl Pts',(51.1712826676667,3.5377217233181,48.5));
#84700=CARTESIAN_POINT('Ctrl Pts',(51.30484296754,3.46643933653831,48.5));
#84701=CARTESIAN_POINT('Ctrl Pts',(51.3918824382126,3.33212831616402,48.5));
#84702=CARTESIAN_POINT('',(51.1712826676667,3.5377217233181,48.35));
#84703=CARTESIAN_POINT('',(51.1712826676667,3.5377217233181,48.5));
#84704=CARTESIAN_POINT('Ctrl Pts',(51.1712826676667,3.5377217233181,48.35));
#84705=CARTESIAN_POINT('Ctrl Pts',(51.30484296754,3.46643933653831,48.35));
#84706=CARTESIAN_POINT('Ctrl Pts',(51.3918824382126,3.33212831616402,48.35));
#84707=CARTESIAN_POINT('Ctrl Pts',(50.8606411404908,3.60900411009789,48.5));
#84708=CARTESIAN_POINT('Ctrl Pts',(50.8606411404908,3.60900411009789,48.35));
#84709=CARTESIAN_POINT('Ctrl Pts',(51.0377217717469,3.60900411009789,48.5));
#84710=CARTESIAN_POINT('Ctrl Pts',(51.0377217717469,3.60900411009789,48.35));
#84711=CARTESIAN_POINT('Ctrl Pts',(51.1712826676667,3.5377217233181,48.5));
#84712=CARTESIAN_POINT('Ctrl Pts',(51.1712826676667,3.5377217233181,48.35));
#84713=CARTESIAN_POINT('',(50.8606411404908,3.60900411009789,48.5));
#84714=CARTESIAN_POINT('Ctrl Pts',(50.8606411404908,3.60900411009789,48.5));
#84715=CARTESIAN_POINT('Ctrl Pts',(51.0377217717469,3.60900411009789,48.5));
#84716=CARTESIAN_POINT('Ctrl Pts',(51.1712826676667,3.5377217233181,48.5));
#84717=CARTESIAN_POINT('',(50.8606411404908,3.60900411009789,48.35));
#84718=CARTESIAN_POINT('',(50.8606411404908,3.60900411009789,48.5));
#84719=CARTESIAN_POINT('Ctrl Pts',(50.8606411404908,3.60900411009789,48.35));
#84720=CARTESIAN_POINT('Ctrl Pts',(51.0377217717469,3.60900411009789,48.35));
#84721=CARTESIAN_POINT('Ctrl Pts',(51.1712826676667,3.5377217233181,48.35));
#84722=CARTESIAN_POINT('Ctrl Pts',(50.462210316211,3.47994545102119,48.5));
#84723=CARTESIAN_POINT('Ctrl Pts',(50.462210316211,3.47994545102119,48.35));
#84724=CARTESIAN_POINT('Ctrl Pts',(50.6205321736634,3.60900411009789,48.5));
#84725=CARTESIAN_POINT('Ctrl Pts',(50.6205321736634,3.60900411009789,48.35));
#84726=CARTESIAN_POINT('Ctrl Pts',(50.8606411404908,3.60900411009789,48.5));
#84727=CARTESIAN_POINT('Ctrl Pts',(50.8606411404908,3.60900411009789,48.35));
#84728=CARTESIAN_POINT('',(50.462210316211,3.47994545102119,48.5));
#84729=CARTESIAN_POINT('Ctrl Pts',(50.462210316211,3.47994545102119,48.5));
#84730=CARTESIAN_POINT('Ctrl Pts',(50.6205321736634,3.60900411009789,48.5));
#84731=CARTESIAN_POINT('Ctrl Pts',(50.8606411404908,3.60900411009789,48.5));
#84732=CARTESIAN_POINT('',(50.462210316211,3.47994545102119,48.35));
#84733=CARTESIAN_POINT('',(50.462210316211,3.47994545102119,48.5));
#84734=CARTESIAN_POINT('Ctrl Pts',(50.462210316211,3.47994545102119,48.35));
#84735=CARTESIAN_POINT('Ctrl Pts',(50.6205321736634,3.60900411009789,48.35));
#84736=CARTESIAN_POINT('Ctrl Pts',(50.8606411404908,3.60900411009789,48.35));
#84737=CARTESIAN_POINT('Ctrl Pts',(50.2236015982926,3.11302864551544,48.5));
#84738=CARTESIAN_POINT('Ctrl Pts',(50.2236015982926,3.11302864551544,48.35));
#84739=CARTESIAN_POINT('Ctrl Pts',(50.3038881607354,3.3508867919445,48.5));
#84740=CARTESIAN_POINT('Ctrl Pts',(50.3038881607354,3.3508867919445,48.35));
#84741=CARTESIAN_POINT('Ctrl Pts',(50.462210316211,3.47994545102119,48.5));
#84742=CARTESIAN_POINT('Ctrl Pts',(50.462210316211,3.47994545102119,48.35));
#84743=CARTESIAN_POINT('',(50.2236015982926,3.11302864551544,48.5));
#84744=CARTESIAN_POINT('Ctrl Pts',(50.2236015982926,3.11302864551544,48.5));
#84745=CARTESIAN_POINT('Ctrl Pts',(50.3038881607354,3.3508867919445,48.5));
#84746=CARTESIAN_POINT('Ctrl Pts',(50.462210316211,3.47994545102119,48.5));
#84747=CARTESIAN_POINT('',(50.2236015982926,3.11302864551544,48.35));
#84748=CARTESIAN_POINT('',(50.2236015982926,3.11302864551544,48.5));
#84749=CARTESIAN_POINT('Ctrl Pts',(50.2236015982926,3.11302864551544,48.35));
#84750=CARTESIAN_POINT('Ctrl Pts',(50.3038881607354,3.3508867919445,48.35));
#84751=CARTESIAN_POINT('Ctrl Pts',(50.462210316211,3.47994545102119,48.35));
#84752=CARTESIAN_POINT('Ctrl Pts',(50.143315333873,2.48499327898026,48.5));
#84753=CARTESIAN_POINT('Ctrl Pts',(50.143315333873,2.48499327898026,48.35));
#84754=CARTESIAN_POINT('Ctrl Pts',(50.143315333873,2.87517049908638,48.5));
#84755=CARTESIAN_POINT('Ctrl Pts',(50.143315333873,2.87517049908638,48.35));
#84756=CARTESIAN_POINT('Ctrl Pts',(50.2236015982926,3.11302864551544,48.5));
#84757=CARTESIAN_POINT('Ctrl Pts',(50.2236015982926,3.11302864551544,48.35));
#84758=CARTESIAN_POINT('',(50.143315333873,2.48499327898026,48.5));
#84759=CARTESIAN_POINT('Ctrl Pts',(50.143315333873,2.48499327898026,48.5));
#84760=CARTESIAN_POINT('Ctrl Pts',(50.143315333873,2.87517049908638,48.5));
#84761=CARTESIAN_POINT('Ctrl Pts',(50.2236015982926,3.11302864551544,48.5));
#84762=CARTESIAN_POINT('',(50.143315333873,2.48499327898026,48.35));
#84763=CARTESIAN_POINT('',(50.143315333873,2.48499327898026,48.5));
#84764=CARTESIAN_POINT('Ctrl Pts',(50.143315333873,2.48499327898026,48.35));
#84765=CARTESIAN_POINT('Ctrl Pts',(50.143315333873,2.87517049908638,48.35));
#84766=CARTESIAN_POINT('Ctrl Pts',(50.2236015982926,3.11302864551544,48.35));
#84767=CARTESIAN_POINT('Ctrl Pts',(50.3609140105546,1.59058684110642,48.5));
#84768=CARTESIAN_POINT('Ctrl Pts',(50.3609140105546,1.59058684110642,48.35));
#84769=CARTESIAN_POINT('Ctrl Pts',(50.143315333873,1.86521166563034,48.5));
#84770=CARTESIAN_POINT('Ctrl Pts',(50.143315333873,1.86521166563034,48.35));
#84771=CARTESIAN_POINT('Ctrl Pts',(50.143315333873,2.48499327898026,48.5));
#84772=CARTESIAN_POINT('Ctrl Pts',(50.143315333873,2.48499327898026,48.35));
#84773=CARTESIAN_POINT('Ctrl Pts',(50.3609140105546,1.59058684110642,48.5));
#84774=CARTESIAN_POINT('Ctrl Pts',(50.143315333873,1.86521166563034,48.5));
#84775=CARTESIAN_POINT('Ctrl Pts',(50.143315333873,2.48499327898026,48.5));
#84776=CARTESIAN_POINT('Ctrl Pts',(50.3609140105546,1.59058684110642,48.35));
#84777=CARTESIAN_POINT('Ctrl Pts',(50.143315333873,1.86521166563034,48.35));
#84778=CARTESIAN_POINT('Ctrl Pts',(50.143315333873,2.48499327898026,48.35));
#84779=CARTESIAN_POINT('Origin',(49.9999999143183,2.48574362695217,48.35));
#84780=CARTESIAN_POINT('Ctrl Pts',(49.1708733029664,2.58854025602341,48.5));
#84781=CARTESIAN_POINT('Ctrl Pts',(49.1708733029664,2.58854025602341,48.35));
#84782=CARTESIAN_POINT('Ctrl Pts',(48.9877900369465,2.58854025602341,48.5));
#84783=CARTESIAN_POINT('Ctrl Pts',(48.9877900369465,2.58854025602341,48.35));
#84784=CARTESIAN_POINT('Ctrl Pts',(48.8602320738137,2.45723062753677,48.5));
#84785=CARTESIAN_POINT('Ctrl Pts',(48.8602320738137,2.45723062753677,48.35));
#84786=CARTESIAN_POINT('',(49.1708733029664,2.58854025602341,48.5));
#84787=CARTESIAN_POINT('',(48.8602320738137,2.45723062753677,48.5));
#84788=CARTESIAN_POINT('Ctrl Pts',(49.1708733029664,2.58854025602341,48.5));
#84789=CARTESIAN_POINT('Ctrl Pts',(48.9877900369465,2.58854025602341,48.5));
#84790=CARTESIAN_POINT('Ctrl Pts',(48.8602320738137,2.45723062753677,48.5));
#84791=CARTESIAN_POINT('',(49.1708733029664,2.58854025602341,48.35));
#84792=CARTESIAN_POINT('',(49.1708733029664,2.58854025602341,48.5));
#84793=CARTESIAN_POINT('',(48.8602320738137,2.45723062753677,48.35));
#84794=CARTESIAN_POINT('Ctrl Pts',(49.1708733029664,2.58854025602341,48.35));
#84795=CARTESIAN_POINT('Ctrl Pts',(48.9877900369465,2.58854025602341,48.35));
#84796=CARTESIAN_POINT('Ctrl Pts',(48.8602320738137,2.45723062753677,48.35));
#84797=CARTESIAN_POINT('',(48.8602320738137,2.45723062753677,48.5));
#84798=CARTESIAN_POINT('Ctrl Pts',(49.4770122952759,2.45723062753677,48.5));
#84799=CARTESIAN_POINT('Ctrl Pts',(49.4770122952759,2.45723062753677,48.35));
#84800=CARTESIAN_POINT('Ctrl Pts',(49.35545726493,2.58854025602341,48.5));
#84801=CARTESIAN_POINT('Ctrl Pts',(49.35545726493,2.58854025602341,48.35));
#84802=CARTESIAN_POINT('Ctrl Pts',(49.1708733029664,2.58854025602341,48.5));
#84803=CARTESIAN_POINT('Ctrl Pts',(49.1708733029664,2.58854025602341,48.35));
#84804=CARTESIAN_POINT('',(49.4770122952759,2.45723062753677,48.5));
#84805=CARTESIAN_POINT('Ctrl Pts',(49.4770122952759,2.45723062753677,48.5));
#84806=CARTESIAN_POINT('Ctrl Pts',(49.35545726493,2.58854025602341,48.5));
#84807=CARTESIAN_POINT('Ctrl Pts',(49.1708733029664,2.58854025602341,48.5));
#84808=CARTESIAN_POINT('',(49.4770122952759,2.45723062753677,48.35));
#84809=CARTESIAN_POINT('',(49.4770122952759,2.45723062753677,48.5));
#84810=CARTESIAN_POINT('Ctrl Pts',(49.4770122952759,2.45723062753677,48.35));
#84811=CARTESIAN_POINT('Ctrl Pts',(49.35545726493,2.58854025602341,48.35));
#84812=CARTESIAN_POINT('Ctrl Pts',(49.1708733029664,2.58854025602341,48.35));
#84813=CARTESIAN_POINT('Ctrl Pts',(49.5985676236451,2.09781730175018,48.5));
#84814=CARTESIAN_POINT('Ctrl Pts',(49.5985676236451,2.09781730175018,48.35));
#84815=CARTESIAN_POINT('Ctrl Pts',(49.5985676236451,2.32592099905014,48.5));
#84816=CARTESIAN_POINT('Ctrl Pts',(49.5985676236451,2.32592099905014,48.35));
#84817=CARTESIAN_POINT('Ctrl Pts',(49.4770122952759,2.45723062753677,48.5));
#84818=CARTESIAN_POINT('Ctrl Pts',(49.4770122952759,2.45723062753677,48.35));
#84819=CARTESIAN_POINT('',(49.5985676236451,2.09781730175018,48.5));
#84820=CARTESIAN_POINT('Ctrl Pts',(49.5985676236451,2.09781730175018,48.5));
#84821=CARTESIAN_POINT('Ctrl Pts',(49.5985676236451,2.32592099905014,48.5));
#84822=CARTESIAN_POINT('Ctrl Pts',(49.4770122952759,2.45723062753677,48.5));
#84823=CARTESIAN_POINT('',(49.5985676236451,2.09781730175018,48.35));
#84824=CARTESIAN_POINT('',(49.5985676236451,2.09781730175018,48.5));
#84825=CARTESIAN_POINT('Ctrl Pts',(49.5985676236451,2.09781730175018,48.35));
#84826=CARTESIAN_POINT('Ctrl Pts',(49.5985676236451,2.32592099905014,48.35));
#84827=CARTESIAN_POINT('Ctrl Pts',(49.4770122952759,2.45723062753677,48.35));
#84828=CARTESIAN_POINT('Ctrl Pts',(49.4755117483437,1.72264659404755,48.5));
#84829=CARTESIAN_POINT('Ctrl Pts',(49.4755117483437,1.72264659404755,48.35));
#84830=CARTESIAN_POINT('Ctrl Pts',(49.5985676236451,1.86070942878723,48.5));
#84831=CARTESIAN_POINT('Ctrl Pts',(49.5985676236451,1.86070942878723,48.35));
#84832=CARTESIAN_POINT('Ctrl Pts',(49.5985676236451,2.09781730175018,48.5));
#84833=CARTESIAN_POINT('Ctrl Pts',(49.5985676236451,2.09781730175018,48.35));
#84834=CARTESIAN_POINT('',(49.4755117483437,1.72264659404755,48.5));
#84835=CARTESIAN_POINT('Ctrl Pts',(49.4755117483437,1.72264659404755,48.5));
#84836=CARTESIAN_POINT('Ctrl Pts',(49.5985676236451,1.86070942878723,48.5));
#84837=CARTESIAN_POINT('Ctrl Pts',(49.5985676236451,2.09781730175018,48.5));
#84838=CARTESIAN_POINT('',(49.4755117483437,1.72264659404755,48.35));
#84839=CARTESIAN_POINT('',(49.4755117483437,1.72264659404755,48.5));
#84840=CARTESIAN_POINT('Ctrl Pts',(49.4755117483437,1.72264659404755,48.35));
#84841=CARTESIAN_POINT('Ctrl Pts',(49.5985676236451,1.86070942878723,48.35));
#84842=CARTESIAN_POINT('Ctrl Pts',(49.5985676236451,2.09781730175018,48.35));
#84843=CARTESIAN_POINT('Ctrl Pts',(49.1813780255616,1.58458405733109,48.5));
#84844=CARTESIAN_POINT('Ctrl Pts',(49.1813780255616,1.58458405733109,48.35));
#84845=CARTESIAN_POINT('Ctrl Pts',(49.3524558730423,1.58458405733109,48.5));
#84846=CARTESIAN_POINT('Ctrl Pts',(49.3524558730423,1.58458405733109,48.35));
#84847=CARTESIAN_POINT('Ctrl Pts',(49.4755117483437,1.72264659404755,48.5));
#84848=CARTESIAN_POINT('Ctrl Pts',(49.4755117483437,1.72264659404755,48.35));
#84849=CARTESIAN_POINT('',(49.1813780255616,1.58458405733109,48.5));
#84850=CARTESIAN_POINT('Ctrl Pts',(49.1813780255616,1.58458405733109,48.5));
#84851=CARTESIAN_POINT('Ctrl Pts',(49.3524558730423,1.58458405733109,48.5));
#84852=CARTESIAN_POINT('Ctrl Pts',(49.4755117483437,1.72264659404755,48.5));
#84853=CARTESIAN_POINT('',(49.1813780255616,1.58458405733109,48.35));
#84854=CARTESIAN_POINT('',(49.1813780255616,1.58458405733109,48.5));
#84855=CARTESIAN_POINT('Ctrl Pts',(49.1813780255616,1.58458405733109,48.35));
#84856=CARTESIAN_POINT('Ctrl Pts',(49.3524558730423,1.58458405733109,48.35));
#84857=CARTESIAN_POINT('Ctrl Pts',(49.4755117483437,1.72264659404755,48.35));
#84858=CARTESIAN_POINT('Ctrl Pts',(48.9577764160931,1.65136420726776,48.5));
#84859=CARTESIAN_POINT('Ctrl Pts',(48.9577764160931,1.65136420726776,48.35));
#84860=CARTESIAN_POINT('Ctrl Pts',(49.0643249340355,1.58458405733109,48.5));
#84861=CARTESIAN_POINT('Ctrl Pts',(49.0643249340355,1.58458405733109,48.35));
#84862=CARTESIAN_POINT('Ctrl Pts',(49.1813780255616,1.58458405733109,48.5));
#84863=CARTESIAN_POINT('Ctrl Pts',(49.1813780255616,1.58458405733109,48.35));
#84864=CARTESIAN_POINT('',(48.9577764160931,1.65136420726776,48.5));
#84865=CARTESIAN_POINT('Ctrl Pts',(48.9577764160931,1.65136420726776,48.5));
#84866=CARTESIAN_POINT('Ctrl Pts',(49.0643249340355,1.58458405733109,48.5));
#84867=CARTESIAN_POINT('Ctrl Pts',(49.1813780255616,1.58458405733109,48.5));
#84868=CARTESIAN_POINT('',(48.9577764160931,1.65136420726776,48.35));
#84869=CARTESIAN_POINT('',(48.9577764160931,1.65136420726776,48.5));
#84870=CARTESIAN_POINT('Ctrl Pts',(48.9577764160931,1.65136420726776,48.35));
#84871=CARTESIAN_POINT('Ctrl Pts',(49.0643249340355,1.58458405733109,48.35));
#84872=CARTESIAN_POINT('Ctrl Pts',(49.1813780255616,1.58458405733109,48.35));
#84873=CARTESIAN_POINT('Ctrl Pts',(48.7919510789216,1.84570276737213,48.5));
#84874=CARTESIAN_POINT('Ctrl Pts',(48.7919510789216,1.84570276737213,48.35));
#84875=CARTESIAN_POINT('Ctrl Pts',(48.8512278981507,1.71814465522766,48.5));
#84876=CARTESIAN_POINT('Ctrl Pts',(48.8512278981507,1.71814465522766,48.35));
#84877=CARTESIAN_POINT('Ctrl Pts',(48.9577764160931,1.65136420726776,48.5));
#84878=CARTESIAN_POINT('Ctrl Pts',(48.9577764160931,1.65136420726776,48.35));
#84879=CARTESIAN_POINT('',(48.7919510789216,1.84570276737213,48.5));
#84880=CARTESIAN_POINT('Ctrl Pts',(48.7919510789216,1.84570276737213,48.5));
#84881=CARTESIAN_POINT('Ctrl Pts',(48.8512278981507,1.71814465522766,48.5));
#84882=CARTESIAN_POINT('Ctrl Pts',(48.9577764160931,1.65136420726776,48.5));
#84883=CARTESIAN_POINT('',(48.7919510789216,1.84570276737213,48.35));
#84884=CARTESIAN_POINT('',(48.7919510789216,1.84570276737213,48.5));
#84885=CARTESIAN_POINT('Ctrl Pts',(48.7919510789216,1.84570276737213,48.35));
#84886=CARTESIAN_POINT('Ctrl Pts',(48.8512278981507,1.71814465522766,48.35));
#84887=CARTESIAN_POINT('Ctrl Pts',(48.9577764160931,1.65136420726776,48.35));
#84888=CARTESIAN_POINT('Ctrl Pts',(48.7326739616692,2.1128241121769,48.5));
#84889=CARTESIAN_POINT('Ctrl Pts',(48.7326739616692,2.1128241121769,48.35));
#84890=CARTESIAN_POINT('Ctrl Pts',(48.7326739616692,1.97326058149338,48.5));
#84891=CARTESIAN_POINT('Ctrl Pts',(48.7326739616692,1.97326058149338,48.35));
#84892=CARTESIAN_POINT('Ctrl Pts',(48.7919510789216,1.84570276737213,48.5));
#84893=CARTESIAN_POINT('Ctrl Pts',(48.7919510789216,1.84570276737213,48.35));
#84894=CARTESIAN_POINT('',(48.7326739616692,2.1128241121769,48.5));
#84895=CARTESIAN_POINT('Ctrl Pts',(48.7326739616692,2.1128241121769,48.5));
#84896=CARTESIAN_POINT('Ctrl Pts',(48.7326739616692,1.97326058149338,48.5));
#84897=CARTESIAN_POINT('Ctrl Pts',(48.7919510789216,1.84570276737213,48.5));
#84898=CARTESIAN_POINT('',(48.7326739616692,2.1128241121769,48.35));
#84899=CARTESIAN_POINT('',(48.7326739616692,2.1128241121769,48.5));
#84900=CARTESIAN_POINT('Ctrl Pts',(48.7326739616692,2.1128241121769,48.35));
#84901=CARTESIAN_POINT('Ctrl Pts',(48.7326739616692,1.97326058149338,48.35));
#84902=CARTESIAN_POINT('Ctrl Pts',(48.7919510789216,1.84570276737213,48.35));
#84903=CARTESIAN_POINT('Ctrl Pts',(48.8602320738137,2.45723062753677,48.5));
#84904=CARTESIAN_POINT('Ctrl Pts',(48.8602320738137,2.45723062753677,48.35));
#84905=CARTESIAN_POINT('Ctrl Pts',(48.7326739616692,2.32592099905014,48.5));
#84906=CARTESIAN_POINT('Ctrl Pts',(48.7326739616692,2.32592099905014,48.35));
#84907=CARTESIAN_POINT('Ctrl Pts',(48.7326739616692,2.1128241121769,48.5));
#84908=CARTESIAN_POINT('Ctrl Pts',(48.7326739616692,2.1128241121769,48.35));
#84909=CARTESIAN_POINT('Ctrl Pts',(48.8602320738137,2.45723062753677,48.5));
#84910=CARTESIAN_POINT('Ctrl Pts',(48.7326739616692,2.32592099905014,48.5));
#84911=CARTESIAN_POINT('Ctrl Pts',(48.7326739616692,2.1128241121769,48.5));
#84912=CARTESIAN_POINT('Ctrl Pts',(48.8602320738137,2.45723062753677,48.35));
#84913=CARTESIAN_POINT('Ctrl Pts',(48.7326739616692,2.32592099905014,48.35));
#84914=CARTESIAN_POINT('Ctrl Pts',(48.7326739616692,2.1128241121769,48.35));
#84915=CARTESIAN_POINT('Ctrl Pts',(49.211391646415,3.60900411009789,48.5));
#84916=CARTESIAN_POINT('Ctrl Pts',(49.211391646415,3.60900411009789,48.35));
#84917=CARTESIAN_POINT('Ctrl Pts',(49.4710095115006,3.60900411009789,48.5));
#84918=CARTESIAN_POINT('Ctrl Pts',(49.4710095115006,3.60900411009789,48.35));
#84919=CARTESIAN_POINT('Ctrl Pts',(49.6368349976838,3.46343794465065,48.5));
#84920=CARTESIAN_POINT('Ctrl Pts',(49.6368349976838,3.46343794465065,48.35));
#84921=CARTESIAN_POINT('',(49.211391646415,3.60900411009789,48.5));
#84922=CARTESIAN_POINT('',(49.6368349976838,3.46343794465065,48.5));
#84923=CARTESIAN_POINT('Ctrl Pts',(49.211391646415,3.60900411009789,48.5));
#84924=CARTESIAN_POINT('Ctrl Pts',(49.4710095115006,3.60900411009789,48.5));
#84925=CARTESIAN_POINT('Ctrl Pts',(49.6368349976838,3.46343794465065,48.5));
#84926=CARTESIAN_POINT('',(49.211391646415,3.60900411009789,48.35));
#84927=CARTESIAN_POINT('',(49.211391646415,3.60900411009789,48.5));
#84928=CARTESIAN_POINT('',(49.6368349976838,3.46343794465065,48.35));
#84929=CARTESIAN_POINT('Ctrl Pts',(49.211391646415,3.60900411009789,48.35));
#84930=CARTESIAN_POINT('Ctrl Pts',(49.4710095115006,3.60900411009789,48.35));
#84931=CARTESIAN_POINT('Ctrl Pts',(49.6368349976838,3.46343794465065,48.35));
#84932=CARTESIAN_POINT('',(49.6368349976838,3.46343794465065,48.5));
#84933=CARTESIAN_POINT('Ctrl Pts',(48.6576399095356,3.35688957571983,48.5));
#84934=CARTESIAN_POINT('Ctrl Pts',(48.6576399095356,3.35688957571983,48.35));
#84935=CARTESIAN_POINT('Ctrl Pts',(48.8632334657013,3.60900411009789,48.5));
#84936=CARTESIAN_POINT('Ctrl Pts',(48.8632334657013,3.60900411009789,48.35));
#84937=CARTESIAN_POINT('Ctrl Pts',(49.211391646415,3.60900411009789,48.5));
#84938=CARTESIAN_POINT('Ctrl Pts',(49.211391646415,3.60900411009789,48.35));
#84939=CARTESIAN_POINT('',(48.6576399095356,3.35688957571983,48.5));
#84940=CARTESIAN_POINT('Ctrl Pts',(48.6576399095356,3.35688957571983,48.5));
#84941=CARTESIAN_POINT('Ctrl Pts',(48.8632334657013,3.60900411009789,48.5));
#84942=CARTESIAN_POINT('Ctrl Pts',(49.211391646415,3.60900411009789,48.5));
#84943=CARTESIAN_POINT('',(48.6576399095356,3.35688957571983,48.35));
#84944=CARTESIAN_POINT('',(48.6576399095356,3.35688957571983,48.5));
#84945=CARTESIAN_POINT('Ctrl Pts',(48.6576399095356,3.35688957571983,48.35));
#84946=CARTESIAN_POINT('Ctrl Pts',(48.8632334657013,3.60900411009789,48.35));
#84947=CARTESIAN_POINT('Ctrl Pts',(49.211391646415,3.60900411009789,48.35));
#84948=CARTESIAN_POINT('Ctrl Pts',(48.4220328815281,2.42946797609329,48.5));
#84949=CARTESIAN_POINT('Ctrl Pts',(48.4220328815281,2.42946797609329,48.35));
#84950=CARTESIAN_POINT('Ctrl Pts',(48.4220328815281,3.0672579407692,48.5));
#84951=CARTESIAN_POINT('Ctrl Pts',(48.4220328815281,3.0672579407692,48.35));
#84952=CARTESIAN_POINT('Ctrl Pts',(48.6576399095356,3.35688957571983,48.5));
#84953=CARTESIAN_POINT('Ctrl Pts',(48.6576399095356,3.35688957571983,48.35));
#84954=CARTESIAN_POINT('',(48.4220328815281,2.42946797609329,48.5));
#84955=CARTESIAN_POINT('Ctrl Pts',(48.4220328815281,2.42946797609329,48.5));
#84956=CARTESIAN_POINT('Ctrl Pts',(48.4220328815281,3.0672579407692,48.5));
#84957=CARTESIAN_POINT('Ctrl Pts',(48.6576399095356,3.35688957571983,48.5));
#84958=CARTESIAN_POINT('',(48.4220328815281,2.42946797609329,48.35));
#84959=CARTESIAN_POINT('',(48.4220328815281,2.42946797609329,48.5));
#84960=CARTESIAN_POINT('Ctrl Pts',(48.4220328815281,2.42946797609329,48.35));
#84961=CARTESIAN_POINT('Ctrl Pts',(48.4220328815281,3.0672579407692,48.35));
#84962=CARTESIAN_POINT('Ctrl Pts',(48.6576399095356,3.35688957571983,48.35));
#84963=CARTESIAN_POINT('Ctrl Pts',(48.6351297684014,1.61084586381912,48.5));
#84964=CARTESIAN_POINT('Ctrl Pts',(48.6351297684014,1.61084586381912,48.35));
#84965=CARTESIAN_POINT('Ctrl Pts',(48.4220328815281,1.85920888185501,48.5));
#84966=CARTESIAN_POINT('Ctrl Pts',(48.4220328815281,1.85920888185501,48.35));
#84967=CARTESIAN_POINT('Ctrl Pts',(48.4220328815281,2.42946797609329,48.5));
#84968=CARTESIAN_POINT('Ctrl Pts',(48.4220328815281,2.42946797609329,48.35));
#84969=CARTESIAN_POINT('',(48.6351297684014,1.61084586381912,48.5));
#84970=CARTESIAN_POINT('Ctrl Pts',(48.6351297684014,1.61084586381912,48.5));
#84971=CARTESIAN_POINT('Ctrl Pts',(48.4220328815281,1.85920888185501,48.5));
#84972=CARTESIAN_POINT('Ctrl Pts',(48.4220328815281,2.42946797609329,48.5));
#84973=CARTESIAN_POINT('',(48.6351297684014,1.61084586381912,48.35));
#84974=CARTESIAN_POINT('',(48.6351297684014,1.61084586381912,48.5));
#84975=CARTESIAN_POINT('Ctrl Pts',(48.6351297684014,1.61084586381912,48.35));
#84976=CARTESIAN_POINT('Ctrl Pts',(48.4220328815281,1.85920888185501,48.35));
#84977=CARTESIAN_POINT('Ctrl Pts',(48.4220328815281,2.42946797609329,48.35));
#84978=CARTESIAN_POINT('Ctrl Pts',(49.1858801133931,1.36248314380646,48.5));
#84979=CARTESIAN_POINT('Ctrl Pts',(49.1858801133931,1.36248314380646,48.35));
#84980=CARTESIAN_POINT('Ctrl Pts',(48.848226506263,1.36248314380646,48.5));
#84981=CARTESIAN_POINT('Ctrl Pts',(48.848226506263,1.36248314380646,48.35));
#84982=CARTESIAN_POINT('Ctrl Pts',(48.6351297684014,1.61084586381912,48.5));
#84983=CARTESIAN_POINT('Ctrl Pts',(48.6351297684014,1.61084586381912,48.35));
#84984=CARTESIAN_POINT('',(49.1858801133931,1.36248314380646,48.5));
#84985=CARTESIAN_POINT('Ctrl Pts',(49.1858801133931,1.36248314380646,48.5));
#84986=CARTESIAN_POINT('Ctrl Pts',(48.848226506263,1.36248314380646,48.5));
#84987=CARTESIAN_POINT('Ctrl Pts',(48.6351297684014,1.61084586381912,48.5));
#84988=CARTESIAN_POINT('',(49.1858801133931,1.36248314380646,48.35));
#84989=CARTESIAN_POINT('',(49.1858801133931,1.36248314380646,48.5));
#84990=CARTESIAN_POINT('Ctrl Pts',(49.1858801133931,1.36248314380646,48.35));
#84991=CARTESIAN_POINT('Ctrl Pts',(48.848226506263,1.36248314380646,48.35));
#84992=CARTESIAN_POINT('Ctrl Pts',(48.6351297684014,1.61084586381912,48.35));
#84993=CARTESIAN_POINT('Ctrl Pts',(49.5400412268937,1.45702594518662,48.5));
#84994=CARTESIAN_POINT('Ctrl Pts',(49.5400412268937,1.45702594518662,48.35));
#84995=CARTESIAN_POINT('Ctrl Pts',(49.383970040828,1.36248314380646,48.5));
#84996=CARTESIAN_POINT('Ctrl Pts',(49.383970040828,1.36248314380646,48.35));
#84997=CARTESIAN_POINT('Ctrl Pts',(49.1858801133931,1.36248314380646,48.5));
#84998=CARTESIAN_POINT('Ctrl Pts',(49.1858801133931,1.36248314380646,48.35));
#84999=CARTESIAN_POINT('',(49.5400412268937,1.45702594518662,48.5));
#85000=CARTESIAN_POINT('Ctrl Pts',(49.5400412268937,1.45702594518662,48.5));
#85001=CARTESIAN_POINT('Ctrl Pts',(49.383970040828,1.36248314380646,48.5));
#85002=CARTESIAN_POINT('Ctrl Pts',(49.1858801133931,1.36248314380646,48.5));
#85003=CARTESIAN_POINT('',(49.5400412268937,1.45702594518662,48.35));
#85004=CARTESIAN_POINT('',(49.5400412268937,1.45702594518662,48.5));
#85005=CARTESIAN_POINT('Ctrl Pts',(49.5400412268937,1.45702594518662,48.35));
#85006=CARTESIAN_POINT('Ctrl Pts',(49.383970040828,1.36248314380646,48.35));
#85007=CARTESIAN_POINT('Ctrl Pts',(49.1858801133931,1.36248314380646,48.35));
#85008=CARTESIAN_POINT('Ctrl Pts',(49.7854025550187,1.7293998003006,48.5));
#85009=CARTESIAN_POINT('Ctrl Pts',(49.7854025550187,1.7293998003006,48.35));
#85010=CARTESIAN_POINT('Ctrl Pts',(49.6961118169129,1.55156904459,48.5));
#85011=CARTESIAN_POINT('Ctrl Pts',(49.6961118169129,1.55156904459,48.35));
#85012=CARTESIAN_POINT('Ctrl Pts',(49.5400412268937,1.45702594518662,48.5));
#85013=CARTESIAN_POINT('Ctrl Pts',(49.5400412268937,1.45702594518662,48.35));
#85014=CARTESIAN_POINT('',(49.7854025550187,1.7293998003006,48.5));
#85015=CARTESIAN_POINT('Ctrl Pts',(49.7854025550187,1.7293998003006,48.5));
#85016=CARTESIAN_POINT('Ctrl Pts',(49.6961118169129,1.55156904459,48.5));
#85017=CARTESIAN_POINT('Ctrl Pts',(49.5400412268937,1.45702594518662,48.5));
#85018=CARTESIAN_POINT('',(49.7854025550187,1.7293998003006,48.35));
#85019=CARTESIAN_POINT('',(49.7854025550187,1.7293998003006,48.5));
#85020=CARTESIAN_POINT('Ctrl Pts',(49.7854025550187,1.7293998003006,48.35));
#85021=CARTESIAN_POINT('Ctrl Pts',(49.6961118169129,1.55156904459,48.35));
#85022=CARTESIAN_POINT('Ctrl Pts',(49.5400412268937,1.45702594518662,48.35));
#85023=CARTESIAN_POINT('Ctrl Pts',(49.8746932931244,2.11432480812073,48.5));
#85024=CARTESIAN_POINT('Ctrl Pts',(49.8746932931244,2.11432480812073,48.35));
#85025=CARTESIAN_POINT('Ctrl Pts',(49.8746932931244,1.9072305560112,48.5));
#85026=CARTESIAN_POINT('Ctrl Pts',(49.8746932931244,1.9072305560112,48.35));
#85027=CARTESIAN_POINT('Ctrl Pts',(49.7854025550187,1.7293998003006,48.5));
#85028=CARTESIAN_POINT('Ctrl Pts',(49.7854025550187,1.7293998003006,48.35));
#85029=CARTESIAN_POINT('',(49.8746932931244,2.11432480812073,48.5));
#85030=CARTESIAN_POINT('Ctrl Pts',(49.8746932931244,2.11432480812073,48.5));
#85031=CARTESIAN_POINT('Ctrl Pts',(49.8746932931244,1.9072305560112,48.5));
#85032=CARTESIAN_POINT('Ctrl Pts',(49.7854025550187,1.7293998003006,48.5));
#85033=CARTESIAN_POINT('',(49.8746932931244,2.11432480812073,48.35));
#85034=CARTESIAN_POINT('',(49.8746932931244,2.11432480812073,48.5));
#85035=CARTESIAN_POINT('Ctrl Pts',(49.8746932931244,2.11432480812073,48.35));
#85036=CARTESIAN_POINT('Ctrl Pts',(49.8746932931244,1.9072305560112,48.35));
#85037=CARTESIAN_POINT('Ctrl Pts',(49.7854025550187,1.7293998003006,48.35));
#85038=CARTESIAN_POINT('Ctrl Pts',(49.68485667184,2.62830847501755,48.5));
#85039=CARTESIAN_POINT('Ctrl Pts',(49.68485667184,2.62830847501755,48.35));
#85040=CARTESIAN_POINT('Ctrl Pts',(49.8746932931244,2.42946797609329,48.5));
#85041=CARTESIAN_POINT('Ctrl Pts',(49.8746932931244,2.42946797609329,48.35));
#85042=CARTESIAN_POINT('Ctrl Pts',(49.8746932931244,2.11432480812073,48.5));
#85043=CARTESIAN_POINT('Ctrl Pts',(49.8746932931244,2.11432480812073,48.35));
#85044=CARTESIAN_POINT('',(49.68485667184,2.62830847501755,48.5));
#85045=CARTESIAN_POINT('Ctrl Pts',(49.68485667184,2.62830847501755,48.5));
#85046=CARTESIAN_POINT('Ctrl Pts',(49.8746932931244,2.42946797609329,48.5));
#85047=CARTESIAN_POINT('Ctrl Pts',(49.8746932931244,2.11432480812073,48.5));
#85048=CARTESIAN_POINT('',(49.68485667184,2.62830847501755,48.35));
#85049=CARTESIAN_POINT('',(49.68485667184,2.62830847501755,48.5));
#85050=CARTESIAN_POINT('Ctrl Pts',(49.68485667184,2.62830847501755,48.35));
#85051=CARTESIAN_POINT('Ctrl Pts',(49.8746932931244,2.42946797609329,48.35));
#85052=CARTESIAN_POINT('Ctrl Pts',(49.8746932931244,2.11432480812073,48.35));
#85053=CARTESIAN_POINT('Ctrl Pts',(49.2248977608979,2.82714867591858,48.5));
#85054=CARTESIAN_POINT('Ctrl Pts',(49.2248977608979,2.82714867591858,48.35));
#85055=CARTESIAN_POINT('Ctrl Pts',(49.4950206466019,2.82714867591858,48.5));
#85056=CARTESIAN_POINT('Ctrl Pts',(49.4950206466019,2.82714867591858,48.35));
#85057=CARTESIAN_POINT('Ctrl Pts',(49.68485667184,2.62830847501755,48.5));
#85058=CARTESIAN_POINT('Ctrl Pts',(49.68485667184,2.62830847501755,48.35));
#85059=CARTESIAN_POINT('',(49.2248977608979,2.82714867591858,48.5));
#85060=CARTESIAN_POINT('Ctrl Pts',(49.2248977608979,2.82714867591858,48.5));
#85061=CARTESIAN_POINT('Ctrl Pts',(49.4950206466019,2.82714867591858,48.5));
#85062=CARTESIAN_POINT('Ctrl Pts',(49.68485667184,2.62830847501755,48.5));
#85063=CARTESIAN_POINT('',(49.2248977608979,2.82714867591858,48.35));
#85064=CARTESIAN_POINT('',(49.2248977608979,2.82714867591858,48.5));
#85065=CARTESIAN_POINT('Ctrl Pts',(49.2248977608979,2.82714867591858,48.35));
#85066=CARTESIAN_POINT('Ctrl Pts',(49.4950206466019,2.82714867591858,48.35));
#85067=CARTESIAN_POINT('Ctrl Pts',(49.68485667184,2.62830847501755,48.35));
#85068=CARTESIAN_POINT('Ctrl Pts',(48.9292634911835,2.75511601567268,48.5));
#85069=CARTESIAN_POINT('Ctrl Pts',(48.9292634911835,2.75511601567268,48.35));
#85070=CARTESIAN_POINT('Ctrl Pts',(49.0703275687993,2.82714867591858,48.5));
#85071=CARTESIAN_POINT('Ctrl Pts',(49.0703275687993,2.82714867591858,48.35));
#85072=CARTESIAN_POINT('Ctrl Pts',(49.2248977608979,2.82714867591858,48.5));
#85073=CARTESIAN_POINT('Ctrl Pts',(49.2248977608979,2.82714867591858,48.35));
#85074=CARTESIAN_POINT('',(48.9292634911835,2.75511601567268,48.5));
#85075=CARTESIAN_POINT('Ctrl Pts',(48.9292634911835,2.75511601567268,48.5));
#85076=CARTESIAN_POINT('Ctrl Pts',(49.0703275687993,2.82714867591858,48.5));
#85077=CARTESIAN_POINT('Ctrl Pts',(49.2248977608979,2.82714867591858,48.5));
#85078=CARTESIAN_POINT('',(48.9292634911835,2.75511601567268,48.35));
#85079=CARTESIAN_POINT('',(48.9292634911835,2.75511601567268,48.5));
#85080=CARTESIAN_POINT('Ctrl Pts',(48.9292634911835,2.75511601567268,48.35));
#85081=CARTESIAN_POINT('Ctrl Pts',(49.0703275687993,2.82714867591858,48.35));
#85082=CARTESIAN_POINT('Ctrl Pts',(49.2248977608979,2.82714867591858,48.35));
#85083=CARTESIAN_POINT('Ctrl Pts',(48.6906549222767,2.53451579809189,48.5));
#85084=CARTESIAN_POINT('Ctrl Pts',(48.6906549222767,2.53451579809189,48.35));
#85085=CARTESIAN_POINT('Ctrl Pts',(48.7881992645562,2.68308320641518,48.5));
#85086=CARTESIAN_POINT('Ctrl Pts',(48.7881992645562,2.68308320641518,48.35));
#85087=CARTESIAN_POINT('Ctrl Pts',(48.9292634911835,2.75511601567268,48.5));
#85088=CARTESIAN_POINT('Ctrl Pts',(48.9292634911835,2.75511601567268,48.35));
#85089=CARTESIAN_POINT('',(48.6906549222767,2.53451579809189,48.5));
#85090=CARTESIAN_POINT('Ctrl Pts',(48.6906549222767,2.53451579809189,48.5));
#85091=CARTESIAN_POINT('Ctrl Pts',(48.7881992645562,2.68308320641518,48.5));
#85092=CARTESIAN_POINT('Ctrl Pts',(48.9292634911835,2.75511601567268,48.5));
#85093=CARTESIAN_POINT('',(48.6906549222767,2.53451579809189,48.35));
#85094=CARTESIAN_POINT('',(48.6906549222767,2.53451579809189,48.5));
#85095=CARTESIAN_POINT('Ctrl Pts',(48.6906549222767,2.53451579809189,48.35));
#85096=CARTESIAN_POINT('Ctrl Pts',(48.7881992645562,2.68308320641518,48.35));
#85097=CARTESIAN_POINT('Ctrl Pts',(48.9292634911835,2.75511601567268,48.35));
#85098=CARTESIAN_POINT('Ctrl Pts',(48.7671898193657,3.04324695467949,48.5));
#85099=CARTESIAN_POINT('Ctrl Pts',(48.7671898193657,3.04324695467949,48.35));
#85100=CARTESIAN_POINT('Ctrl Pts',(48.6936563141644,2.86466577649117,48.5));
#85101=CARTESIAN_POINT('Ctrl Pts',(48.6936563141644,2.86466577649117,48.35));
#85102=CARTESIAN_POINT('Ctrl Pts',(48.6906549222767,2.53451579809189,48.5));
#85103=CARTESIAN_POINT('Ctrl Pts',(48.6906549222767,2.53451579809189,48.35));
#85104=CARTESIAN_POINT('',(48.7671898193657,3.04324695467949,48.5));
#85105=CARTESIAN_POINT('Ctrl Pts',(48.7671898193657,3.04324695467949,48.5));
#85106=CARTESIAN_POINT('Ctrl Pts',(48.6936563141644,2.86466577649117,48.5));
#85107=CARTESIAN_POINT('Ctrl Pts',(48.6906549222767,2.53451579809189,48.5));
#85108=CARTESIAN_POINT('',(48.7671898193657,3.04324695467949,48.35));
#85109=CARTESIAN_POINT('',(48.7671898193657,3.04324695467949,48.5));
#85110=CARTESIAN_POINT('Ctrl Pts',(48.7671898193657,3.04324695467949,48.35));
#85111=CARTESIAN_POINT('Ctrl Pts',(48.6936563141644,2.86466577649117,48.35));
#85112=CARTESIAN_POINT('Ctrl Pts',(48.6906549222767,2.53451579809189,48.35));
#85113=CARTESIAN_POINT('Ctrl Pts',(48.9682811386883,3.31487038731575,48.5));
#85114=CARTESIAN_POINT('Ctrl Pts',(48.9682811386883,3.31487038731575,48.35));
#85115=CARTESIAN_POINT('Ctrl Pts',(48.8407231755555,3.22182813286781,48.5));
#85116=CARTESIAN_POINT('Ctrl Pts',(48.8407231755555,3.22182813286781,48.35));
#85117=CARTESIAN_POINT('Ctrl Pts',(48.7671898193657,3.04324695467949,48.5));
#85118=CARTESIAN_POINT('Ctrl Pts',(48.7671898193657,3.04324695467949,48.35));
#85119=CARTESIAN_POINT('',(48.9682811386883,3.31487038731575,48.5));
#85120=CARTESIAN_POINT('Ctrl Pts',(48.9682811386883,3.31487038731575,48.5));
#85121=CARTESIAN_POINT('Ctrl Pts',(48.8407231755555,3.22182813286781,48.5));
#85122=CARTESIAN_POINT('Ctrl Pts',(48.7671898193657,3.04324695467949,48.5));
#85123=CARTESIAN_POINT('',(48.9682811386883,3.31487038731575,48.35));
#85124=CARTESIAN_POINT('',(48.9682811386883,3.31487038731575,48.5));
#85125=CARTESIAN_POINT('Ctrl Pts',(48.9682811386883,3.31487038731575,48.35));
#85126=CARTESIAN_POINT('Ctrl Pts',(48.8407231755555,3.22182813286781,48.35));
#85127=CARTESIAN_POINT('Ctrl Pts',(48.7671898193657,3.04324695467949,48.35));
#85128=CARTESIAN_POINT('Ctrl Pts',(49.1948841400445,3.38690319657326,48.5));
#85129=CARTESIAN_POINT('Ctrl Pts',(49.1948841400445,3.38690319657326,48.35));
#85130=CARTESIAN_POINT('Ctrl Pts',(49.0658254809678,3.38690319657326,48.5));
#85131=CARTESIAN_POINT('Ctrl Pts',(49.0658254809678,3.38690319657326,48.35));
#85132=CARTESIAN_POINT('Ctrl Pts',(48.9682811386883,3.31487038731575,48.5));
#85133=CARTESIAN_POINT('Ctrl Pts',(48.9682811386883,3.31487038731575,48.35));
#85134=CARTESIAN_POINT('',(49.1948841400445,3.38690319657326,48.5));
#85135=CARTESIAN_POINT('Ctrl Pts',(49.1948841400445,3.38690319657326,48.5));
#85136=CARTESIAN_POINT('Ctrl Pts',(49.0658254809678,3.38690319657326,48.5));
#85137=CARTESIAN_POINT('Ctrl Pts',(48.9682811386883,3.31487038731575,48.5));
#85138=CARTESIAN_POINT('',(49.1948841400445,3.38690319657326,48.35));
#85139=CARTESIAN_POINT('',(49.1948841400445,3.38690319657326,48.5));
#85140=CARTESIAN_POINT('Ctrl Pts',(49.1948841400445,3.38690319657326,48.35));
#85141=CARTESIAN_POINT('Ctrl Pts',(49.0658254809678,3.38690319657326,48.35));
#85142=CARTESIAN_POINT('Ctrl Pts',(48.9682811386883,3.31487038731575,48.35));
#85143=CARTESIAN_POINT('Ctrl Pts',(49.4650070257485,3.27135065197945,48.5));
#85144=CARTESIAN_POINT('Ctrl Pts',(49.4650070257485,3.27135065197945,48.35));
#85145=CARTESIAN_POINT('Ctrl Pts',(49.35545726493,3.38690319657326,48.5));
#85146=CARTESIAN_POINT('Ctrl Pts',(49.35545726493,3.38690319657326,48.35));
#85147=CARTESIAN_POINT('Ctrl Pts',(49.1948841400445,3.38690319657326,48.5));
#85148=CARTESIAN_POINT('Ctrl Pts',(49.1948841400445,3.38690319657326,48.35));
#85149=CARTESIAN_POINT('',(49.4650070257485,3.27135065197945,48.5));
#85150=CARTESIAN_POINT('Ctrl Pts',(49.4650070257485,3.27135065197945,48.5));
#85151=CARTESIAN_POINT('Ctrl Pts',(49.35545726493,3.38690319657326,48.5));
#85152=CARTESIAN_POINT('Ctrl Pts',(49.1948841400445,3.38690319657326,48.5));
#85153=CARTESIAN_POINT('',(49.4650070257485,3.27135065197945,48.35));
#85154=CARTESIAN_POINT('',(49.4650070257485,3.27135065197945,48.5));
#85155=CARTESIAN_POINT('Ctrl Pts',(49.4650070257485,3.27135065197945,48.35));
#85156=CARTESIAN_POINT('Ctrl Pts',(49.35545726493,3.38690319657326,48.35));
#85157=CARTESIAN_POINT('Ctrl Pts',(49.1948841400445,3.38690319657326,48.35));
#85158=CARTESIAN_POINT('Ctrl Pts',(49.5670534558594,3.04024556279182,48.5));
#85159=CARTESIAN_POINT('Ctrl Pts',(49.5670534558594,3.04024556279182,48.35));
#85160=CARTESIAN_POINT('Ctrl Pts',(49.5310370512307,3.19931784272194,48.5));
#85161=CARTESIAN_POINT('Ctrl Pts',(49.5310370512307,3.19931784272194,48.35));
#85162=CARTESIAN_POINT('Ctrl Pts',(49.4650070257485,3.27135065197945,48.5));
#85163=CARTESIAN_POINT('Ctrl Pts',(49.4650070257485,3.27135065197945,48.35));
#85164=CARTESIAN_POINT('',(49.5670534558594,3.04024556279182,48.5));
#85165=CARTESIAN_POINT('Ctrl Pts',(49.5670534558594,3.04024556279182,48.5));
#85166=CARTESIAN_POINT('Ctrl Pts',(49.5310370512307,3.19931784272194,48.5));
#85167=CARTESIAN_POINT('Ctrl Pts',(49.4650070257485,3.27135065197945,48.5));
#85168=CARTESIAN_POINT('',(49.5670534558594,3.04024556279182,48.35));
#85169=CARTESIAN_POINT('',(49.5670534558594,3.04024556279182,48.5));
#85170=CARTESIAN_POINT('Ctrl Pts',(49.5670534558594,3.04024556279182,48.35));
#85171=CARTESIAN_POINT('Ctrl Pts',(49.5310370512307,3.19931784272194,48.35));
#85172=CARTESIAN_POINT('Ctrl Pts',(49.4650070257485,3.27135065197945,48.35));
#85173=CARTESIAN_POINT('Origin',(49.835675496608,3.06125515699387,48.5));
#85174=CARTESIAN_POINT('',(49.835675496608,3.06125515699387,48.5));
#85175=CARTESIAN_POINT('',(25.2612996235975,1.13923243904573,48.5));
#85176=CARTESIAN_POINT('',(49.835675496608,3.06125515699387,48.35));
#85177=CARTESIAN_POINT('',(49.835675496608,3.06125515699387,48.5));
#85178=CARTESIAN_POINT('',(49.835675496608,3.06125515699387,48.35));
#85179=CARTESIAN_POINT('Ctrl Pts',(49.6368349976838,3.46343794465065,48.5));
#85180=CARTESIAN_POINT('Ctrl Pts',(49.6368349976838,3.46343794465065,48.35));
#85181=CARTESIAN_POINT('Ctrl Pts',(49.8026604838669,3.31787177920341,48.5));
#85182=CARTESIAN_POINT('Ctrl Pts',(49.8026604838669,3.31787177920341,48.35));
#85183=CARTESIAN_POINT('Ctrl Pts',(49.835675496608,3.06125515699387,48.5));
#85184=CARTESIAN_POINT('Ctrl Pts',(49.835675496608,3.06125515699387,48.35));
#85185=CARTESIAN_POINT('Ctrl Pts',(49.6368349976838,3.46343794465065,48.5));
#85186=CARTESIAN_POINT('Ctrl Pts',(49.8026604838669,3.31787177920341,48.5));
#85187=CARTESIAN_POINT('Ctrl Pts',(49.835675496608,3.06125515699387,48.5));
#85188=CARTESIAN_POINT('Ctrl Pts',(49.6368349976838,3.46343794465065,48.35));
#85189=CARTESIAN_POINT('Ctrl Pts',(49.8026604838669,3.31787177920341,48.35));
#85190=CARTESIAN_POINT('Ctrl Pts',(49.835675496608,3.06125515699387,48.35));
#85191=CARTESIAN_POINT('Origin',(49.9999999143183,2.48574362695217,48.35));
#85192=CARTESIAN_POINT('Origin',(0.,8.,48.5));
#85193=CARTESIAN_POINT('Origin',(0.,8.,48.5));
#85194=CARTESIAN_POINT('Ctrl Pts',(40.8426330685616,3.38540250062943,48.5));
#85195=CARTESIAN_POINT('Ctrl Pts',(40.8426330685616,3.38540250062943,48.35));
#85196=CARTESIAN_POINT('Ctrl Pts',(40.6565482616425,3.38540250062943,48.5));
#85197=CARTESIAN_POINT('Ctrl Pts',(40.6565482616425,3.38540250062943,48.35));
#85198=CARTESIAN_POINT('Ctrl Pts',(40.5454979538918,3.22783091664314,48.5));
#85199=CARTESIAN_POINT('Ctrl Pts',(40.5454979538918,3.22783091664314,48.35));
#85200=CARTESIAN_POINT('',(40.8426330685616,3.38540250062943,48.5));
#85201=CARTESIAN_POINT('',(40.5454979538918,3.22783091664314,48.5));
#85202=CARTESIAN_POINT('Ctrl Pts',(40.8426330685616,3.38540250062943,48.5));
#85203=CARTESIAN_POINT('Ctrl Pts',(40.6565482616425,3.38540250062943,48.5));
#85204=CARTESIAN_POINT('Ctrl Pts',(40.5454979538918,3.22783091664314,48.5));
#85205=CARTESIAN_POINT('',(40.8426330685616,3.38540250062943,48.35));
#85206=CARTESIAN_POINT('',(40.8426330685616,3.38540250062943,48.5));
#85207=CARTESIAN_POINT('',(40.5454979538918,3.22783091664314,48.35));
#85208=CARTESIAN_POINT('Ctrl Pts',(40.8426330685616,3.38540250062943,48.35));
#85209=CARTESIAN_POINT('Ctrl Pts',(40.6565482616425,3.38540250062943,48.35));
#85210=CARTESIAN_POINT('Ctrl Pts',(40.5454979538918,3.22783091664314,48.35));
#85211=CARTESIAN_POINT('',(40.5454979538918,3.22783091664314,48.5));
#85212=CARTESIAN_POINT('Ctrl Pts',(41.1585263609886,3.2068213224411,48.5));
#85213=CARTESIAN_POINT('Ctrl Pts',(41.1585263609886,3.2068213224411,48.35));
#85214=CARTESIAN_POINT('Ctrl Pts',(41.0317186713219,3.38540250062943,48.5));
#85215=CARTESIAN_POINT('Ctrl Pts',(41.0317186713219,3.38540250062943,48.35));
#85216=CARTESIAN_POINT('Ctrl Pts',(40.8426330685616,3.38540250062943,48.5));
#85217=CARTESIAN_POINT('Ctrl Pts',(40.8426330685616,3.38540250062943,48.35));
#85218=CARTESIAN_POINT('',(41.1585263609886,3.2068213224411,48.5));
#85219=CARTESIAN_POINT('Ctrl Pts',(41.1585263609886,3.2068213224411,48.5));
#85220=CARTESIAN_POINT('Ctrl Pts',(41.0317186713219,3.38540250062943,48.5));
#85221=CARTESIAN_POINT('Ctrl Pts',(40.8426330685616,3.38540250062943,48.5));
#85222=CARTESIAN_POINT('',(41.1585263609886,3.2068213224411,48.35));
#85223=CARTESIAN_POINT('',(41.1585263609886,3.2068213224411,48.5));
#85224=CARTESIAN_POINT('Ctrl Pts',(41.1585263609886,3.2068213224411,48.35));
#85225=CARTESIAN_POINT('Ctrl Pts',(41.0317186713219,3.38540250062943,48.35));
#85226=CARTESIAN_POINT('Ctrl Pts',(40.8426330685616,3.38540250062943,48.35));
#85227=CARTESIAN_POINT('Ctrl Pts',(41.2853340506554,2.48499327898026,48.5));
#85228=CARTESIAN_POINT('Ctrl Pts',(41.2853340506554,2.48499327898026,48.35));
#85229=CARTESIAN_POINT('Ctrl Pts',(41.2853340506554,3.02824014425278,48.5));
#85230=CARTESIAN_POINT('Ctrl Pts',(41.2853340506554,3.02824014425278,48.35));
#85231=CARTESIAN_POINT('Ctrl Pts',(41.1585263609886,3.2068213224411,48.5));
#85232=CARTESIAN_POINT('Ctrl Pts',(41.1585263609886,3.2068213224411,48.35));
#85233=CARTESIAN_POINT('',(41.2853340506554,2.48499327898026,48.5));
#85234=CARTESIAN_POINT('Ctrl Pts',(41.2853340506554,2.48499327898026,48.5));
#85235=CARTESIAN_POINT('Ctrl Pts',(41.2853340506554,3.02824014425278,48.5));
#85236=CARTESIAN_POINT('Ctrl Pts',(41.1585263609886,3.2068213224411,48.5));
#85237=CARTESIAN_POINT('',(41.2853340506554,2.48499327898026,48.35));
#85238=CARTESIAN_POINT('',(41.2853340506554,2.48499327898026,48.5));
#85239=CARTESIAN_POINT('Ctrl Pts',(41.2853340506554,2.48499327898026,48.35));
#85240=CARTESIAN_POINT('Ctrl Pts',(41.2853340506554,3.02824014425278,48.35));
#85241=CARTESIAN_POINT('Ctrl Pts',(41.1585263609886,3.2068213224411,48.35));
#85242=CARTESIAN_POINT('Ctrl Pts',(41.1585263609886,1.76466578245163,48.5));
#85243=CARTESIAN_POINT('Ctrl Pts',(41.1585263609886,1.76466578245163,48.35));
#85244=CARTESIAN_POINT('Ctrl Pts',(41.2853340506554,1.9447478055954,48.5));
#85245=CARTESIAN_POINT('Ctrl Pts',(41.2853340506554,1.9447478055954,48.35));
#85246=CARTESIAN_POINT('Ctrl Pts',(41.2853340506554,2.48499327898026,48.5));
#85247=CARTESIAN_POINT('Ctrl Pts',(41.2853340506554,2.48499327898026,48.35));
#85248=CARTESIAN_POINT('',(41.1585263609886,1.76466578245163,48.5));
#85249=CARTESIAN_POINT('Ctrl Pts',(41.1585263609886,1.76466578245163,48.5));
#85250=CARTESIAN_POINT('Ctrl Pts',(41.2853340506554,1.9447478055954,48.5));
#85251=CARTESIAN_POINT('Ctrl Pts',(41.2853340506554,2.48499327898026,48.5));
#85252=CARTESIAN_POINT('',(41.1585263609886,1.76466578245163,48.35));
#85253=CARTESIAN_POINT('',(41.1585263609886,1.76466578245163,48.5));
#85254=CARTESIAN_POINT('Ctrl Pts',(41.1585263609886,1.76466578245163,48.35));
#85255=CARTESIAN_POINT('Ctrl Pts',(41.2853340506554,1.9447478055954,48.35));
#85256=CARTESIAN_POINT('Ctrl Pts',(41.2853340506554,2.48499327898026,48.35));
#85257=CARTESIAN_POINT('Ctrl Pts',(40.845634162426,1.58458405733109,48.5));
#85258=CARTESIAN_POINT('Ctrl Pts',(40.845634162426,1.58458405733109,48.35));
#85259=CARTESIAN_POINT('Ctrl Pts',(41.0317186713219,1.58458405733109,48.5));
#85260=CARTESIAN_POINT('Ctrl Pts',(41.0317186713219,1.58458405733109,48.35));
#85261=CARTESIAN_POINT('Ctrl Pts',(41.1585263609886,1.76466578245163,48.5));
#85262=CARTESIAN_POINT('Ctrl Pts',(41.1585263609886,1.76466578245163,48.35));
#85263=CARTESIAN_POINT('',(40.845634162426,1.58458405733109,48.5));
#85264=CARTESIAN_POINT('Ctrl Pts',(40.845634162426,1.58458405733109,48.5));
#85265=CARTESIAN_POINT('Ctrl Pts',(41.0317186713219,1.58458405733109,48.5));
#85266=CARTESIAN_POINT('Ctrl Pts',(41.1585263609886,1.76466578245163,48.5));
#85267=CARTESIAN_POINT('',(40.845634162426,1.58458405733109,48.35));
#85268=CARTESIAN_POINT('',(40.845634162426,1.58458405733109,48.5));
#85269=CARTESIAN_POINT('Ctrl Pts',(40.845634162426,1.58458405733109,48.35));
#85270=CARTESIAN_POINT('Ctrl Pts',(41.0317186713219,1.58458405733109,48.35));
#85271=CARTESIAN_POINT('Ctrl Pts',(41.1585263609886,1.76466578245163,48.35));
#85272=CARTESIAN_POINT('Ctrl Pts',(40.5327419638634,1.76391565799713,48.5));
#85273=CARTESIAN_POINT('Ctrl Pts',(40.5327419638634,1.76391565799713,48.35));
#85274=CARTESIAN_POINT('Ctrl Pts',(40.6595496535301,1.58458405733109,48.5));
#85275=CARTESIAN_POINT('Ctrl Pts',(40.6595496535301,1.58458405733109,48.35));
#85276=CARTESIAN_POINT('Ctrl Pts',(40.845634162426,1.58458405733109,48.5));
#85277=CARTESIAN_POINT('Ctrl Pts',(40.845634162426,1.58458405733109,48.35));
#85278=CARTESIAN_POINT('',(40.5327419638634,1.76391565799713,48.5));
#85279=CARTESIAN_POINT('Ctrl Pts',(40.5327419638634,1.76391565799713,48.5));
#85280=CARTESIAN_POINT('Ctrl Pts',(40.6595496535301,1.58458405733109,48.5));
#85281=CARTESIAN_POINT('Ctrl Pts',(40.845634162426,1.58458405733109,48.5));
#85282=CARTESIAN_POINT('',(40.5327419638634,1.76391565799713,48.35));
#85283=CARTESIAN_POINT('',(40.5327419638634,1.76391565799713,48.5));
#85284=CARTESIAN_POINT('Ctrl Pts',(40.5327419638634,1.76391565799713,48.35));
#85285=CARTESIAN_POINT('Ctrl Pts',(40.6595496535301,1.58458405733109,48.35));
#85286=CARTESIAN_POINT('Ctrl Pts',(40.845634162426,1.58458405733109,48.35));
#85287=CARTESIAN_POINT('Ctrl Pts',(40.4059342741966,2.48499327898026,48.5));
#85288=CARTESIAN_POINT('Ctrl Pts',(40.4059342741966,2.48499327898026,48.35));
#85289=CARTESIAN_POINT('Ctrl Pts',(40.4059342741966,1.94324696063995,48.5));
#85290=CARTESIAN_POINT('Ctrl Pts',(40.4059342741966,1.94324696063995,48.35));
#85291=CARTESIAN_POINT('Ctrl Pts',(40.5327419638634,1.76391565799713,48.5));
#85292=CARTESIAN_POINT('Ctrl Pts',(40.5327419638634,1.76391565799713,48.35));
#85293=CARTESIAN_POINT('',(40.4059342741966,2.48499327898026,48.5));
#85294=CARTESIAN_POINT('Ctrl Pts',(40.4059342741966,2.48499327898026,48.5));
#85295=CARTESIAN_POINT('Ctrl Pts',(40.4059342741966,1.94324696063995,48.5));
#85296=CARTESIAN_POINT('Ctrl Pts',(40.5327419638634,1.76391565799713,48.5));
#85297=CARTESIAN_POINT('',(40.4059342741966,2.48499327898026,48.35));
#85298=CARTESIAN_POINT('',(40.4059342741966,2.48499327898026,48.5));
#85299=CARTESIAN_POINT('Ctrl Pts',(40.4059342741966,2.48499327898026,48.35));
#85300=CARTESIAN_POINT('Ctrl Pts',(40.4059342741966,1.94324696063995,48.35));
#85301=CARTESIAN_POINT('Ctrl Pts',(40.5327419638634,1.76391565799713,48.35));
#85302=CARTESIAN_POINT('Ctrl Pts',(40.5454979538918,3.22783091664314,48.5));
#85303=CARTESIAN_POINT('Ctrl Pts',(40.5454979538918,3.22783091664314,48.35));
#85304=CARTESIAN_POINT('Ctrl Pts',(40.4059342741966,3.02673944830894,48.5));
#85305=CARTESIAN_POINT('Ctrl Pts',(40.4059342741966,3.02673944830894,48.35));
#85306=CARTESIAN_POINT('Ctrl Pts',(40.4059342741966,2.48499327898026,48.5));
#85307=CARTESIAN_POINT('Ctrl Pts',(40.4059342741966,2.48499327898026,48.35));
#85308=CARTESIAN_POINT('Ctrl Pts',(40.5454979538918,3.22783091664314,48.5));
#85309=CARTESIAN_POINT('Ctrl Pts',(40.4059342741966,3.02673944830894,48.5));
#85310=CARTESIAN_POINT('Ctrl Pts',(40.4059342741966,2.48499327898026,48.5));
#85311=CARTESIAN_POINT('Ctrl Pts',(40.5454979538918,3.22783091664314,48.35));
#85312=CARTESIAN_POINT('Ctrl Pts',(40.4059342741966,3.02673944830894,48.35));
#85313=CARTESIAN_POINT('Ctrl Pts',(40.4059342741966,2.48499327898026,48.35));
#85314=CARTESIAN_POINT('Ctrl Pts',(40.845634162426,1.36248314380646,48.5));
#85315=CARTESIAN_POINT('Ctrl Pts',(40.845634162426,1.36248314380646,48.35));
#85316=CARTESIAN_POINT('Ctrl Pts',(40.5274896025658,1.36248314380646,48.5));
#85317=CARTESIAN_POINT('Ctrl Pts',(40.5274896025658,1.36248314380646,48.35));
#85318=CARTESIAN_POINT('Ctrl Pts',(40.3459070324898,1.59058684110642,48.5));
#85319=CARTESIAN_POINT('Ctrl Pts',(40.3459070324898,1.59058684110642,48.35));
#85320=CARTESIAN_POINT('',(40.845634162426,1.36248314380646,48.5));
#85321=CARTESIAN_POINT('',(40.3459070324898,1.59058684110642,48.5));
#85322=CARTESIAN_POINT('Ctrl Pts',(40.845634162426,1.36248314380646,48.5));
#85323=CARTESIAN_POINT('Ctrl Pts',(40.5274896025658,1.36248314380646,48.5));
#85324=CARTESIAN_POINT('Ctrl Pts',(40.3459070324898,1.59058684110642,48.5));
#85325=CARTESIAN_POINT('',(40.845634162426,1.36248314380646,48.35));
#85326=CARTESIAN_POINT('',(40.845634162426,1.36248314380646,48.5));
#85327=CARTESIAN_POINT('',(40.3459070324898,1.59058684110642,48.35));
#85328=CARTESIAN_POINT('Ctrl Pts',(40.845634162426,1.36248314380646,48.35));
#85329=CARTESIAN_POINT('Ctrl Pts',(40.5274896025658,1.36248314380646,48.35));
#85330=CARTESIAN_POINT('Ctrl Pts',(40.3459070324898,1.59058684110642,48.35));
#85331=CARTESIAN_POINT('',(40.3459070324898,1.59058684110642,48.5));
#85332=CARTESIAN_POINT('Ctrl Pts',(41.2455658316612,1.49229192733765,48.5));
#85333=CARTESIAN_POINT('Ctrl Pts',(41.2455658316612,1.49229192733765,48.35));
#85334=CARTESIAN_POINT('Ctrl Pts',(41.0872439742088,1.36248314380646,48.5));
#85335=CARTESIAN_POINT('Ctrl Pts',(41.0872439742088,1.36248314380646,48.35));
#85336=CARTESIAN_POINT('Ctrl Pts',(40.845634162426,1.36248314380646,48.5));
#85337=CARTESIAN_POINT('Ctrl Pts',(40.845634162426,1.36248314380646,48.35));
#85338=CARTESIAN_POINT('',(41.2455658316612,1.49229192733765,48.5));
#85339=CARTESIAN_POINT('Ctrl Pts',(41.2455658316612,1.49229192733765,48.5));
#85340=CARTESIAN_POINT('Ctrl Pts',(41.0872439742088,1.36248314380646,48.5));
#85341=CARTESIAN_POINT('Ctrl Pts',(40.845634162426,1.36248314380646,48.5));
#85342=CARTESIAN_POINT('',(41.2455658316612,1.49229192733765,48.35));
#85343=CARTESIAN_POINT('',(41.2455658316612,1.49229192733765,48.5));
#85344=CARTESIAN_POINT('Ctrl Pts',(41.2455658316612,1.49229192733765,48.35));
#85345=CARTESIAN_POINT('Ctrl Pts',(41.0872439742088,1.36248314380646,48.35));
#85346=CARTESIAN_POINT('Ctrl Pts',(40.845634162426,1.36248314380646,48.35));
#85347=CARTESIAN_POINT('Ctrl Pts',(41.4834241271019,1.85995900630951,48.5));
#85348=CARTESIAN_POINT('Ctrl Pts',(41.4834241271019,1.85995900630951,48.35));
#85349=CARTESIAN_POINT('Ctrl Pts',(41.4038876891136,1.62210100889206,48.5));
#85350=CARTESIAN_POINT('Ctrl Pts',(41.4038876891136,1.62210100889206,48.35));
#85351=CARTESIAN_POINT('Ctrl Pts',(41.2455658316612,1.49229192733765,48.5));
#85352=CARTESIAN_POINT('Ctrl Pts',(41.2455658316612,1.49229192733765,48.35));
#85353=CARTESIAN_POINT('',(41.4834241271019,1.85995900630951,48.5));
#85354=CARTESIAN_POINT('Ctrl Pts',(41.4834241271019,1.85995900630951,48.5));
#85355=CARTESIAN_POINT('Ctrl Pts',(41.4038876891136,1.62210100889206,48.5));
#85356=CARTESIAN_POINT('Ctrl Pts',(41.2455658316612,1.49229192733765,48.5));
#85357=CARTESIAN_POINT('',(41.4834241271019,1.85995900630951,48.35));
#85358=CARTESIAN_POINT('',(41.4834241271019,1.85995900630951,48.5));
#85359=CARTESIAN_POINT('Ctrl Pts',(41.4834241271019,1.85995900630951,48.35));
#85360=CARTESIAN_POINT('Ctrl Pts',(41.4038876891136,1.62210100889206,48.35));
#85361=CARTESIAN_POINT('Ctrl Pts',(41.2455658316612,1.49229192733765,48.35));
#85362=CARTESIAN_POINT('Ctrl Pts',(41.5629599690437,2.48499327898026,48.5));
#85363=CARTESIAN_POINT('Ctrl Pts',(41.5629599690437,2.48499327898026,48.35));
#85364=CARTESIAN_POINT('Ctrl Pts',(41.5629599690437,2.09781730175018,48.5));
#85365=CARTESIAN_POINT('Ctrl Pts',(41.5629599690437,2.09781730175018,48.35));
#85366=CARTESIAN_POINT('Ctrl Pts',(41.4834241271019,1.85995900630951,48.5));
#85367=CARTESIAN_POINT('Ctrl Pts',(41.4834241271019,1.85995900630951,48.35));
#85368=CARTESIAN_POINT('',(41.5629599690437,2.48499327898026,48.5));
#85369=CARTESIAN_POINT('Ctrl Pts',(41.5629599690437,2.48499327898026,48.5));
#85370=CARTESIAN_POINT('Ctrl Pts',(41.5629599690437,2.09781730175018,48.5));
#85371=CARTESIAN_POINT('Ctrl Pts',(41.4834241271019,1.85995900630951,48.5));
#85372=CARTESIAN_POINT('',(41.5629599690437,2.48499327898026,48.35));
#85373=CARTESIAN_POINT('',(41.5629599690437,2.48499327898026,48.5));
#85374=CARTESIAN_POINT('Ctrl Pts',(41.5629599690437,2.48499327898026,48.35));
#85375=CARTESIAN_POINT('Ctrl Pts',(41.5629599690437,2.09781730175018,48.35));
#85376=CARTESIAN_POINT('Ctrl Pts',(41.4834241271019,1.85995900630951,48.35));
#85377=CARTESIAN_POINT('Ctrl Pts',(41.5134374499321,3.00497958064079,48.5));
#85378=CARTESIAN_POINT('Ctrl Pts',(41.5134374499321,3.00497958064079,48.35));
#85379=CARTESIAN_POINT('Ctrl Pts',(41.5629599690437,2.81214186549187,48.5));
#85380=CARTESIAN_POINT('Ctrl Pts',(41.5629599690437,2.81214186549187,48.35));
#85381=CARTESIAN_POINT('Ctrl Pts',(41.5629599690437,2.48499327898026,48.5));
#85382=CARTESIAN_POINT('Ctrl Pts',(41.5629599690437,2.48499327898026,48.35));
#85383=CARTESIAN_POINT('',(41.5134374499321,3.00497958064079,48.5));
#85384=CARTESIAN_POINT('Ctrl Pts',(41.5134374499321,3.00497958064079,48.5));
#85385=CARTESIAN_POINT('Ctrl Pts',(41.5629599690437,2.81214186549187,48.5));
#85386=CARTESIAN_POINT('Ctrl Pts',(41.5629599690437,2.48499327898026,48.5));
#85387=CARTESIAN_POINT('',(41.5134374499321,3.00497958064079,48.35));
#85388=CARTESIAN_POINT('',(41.5134374499321,3.00497958064079,48.5));
#85389=CARTESIAN_POINT('Ctrl Pts',(41.5134374499321,3.00497958064079,48.35));
#85390=CARTESIAN_POINT('Ctrl Pts',(41.5629599690437,2.81214186549187,48.35));
#85391=CARTESIAN_POINT('Ctrl Pts',(41.5629599690437,2.48499327898026,48.35));
#85392=CARTESIAN_POINT('Ctrl Pts',(41.3768754601479,3.33212831616402,48.5));
#85393=CARTESIAN_POINT('Ctrl Pts',(41.3768754601479,3.33212831616402,48.35));
#85394=CARTESIAN_POINT('Ctrl Pts',(41.4639149308205,3.19781729578972,48.5));
#85395=CARTESIAN_POINT('Ctrl Pts',(41.4639149308205,3.19781729578972,48.35));
#85396=CARTESIAN_POINT('Ctrl Pts',(41.5134374499321,3.00497958064079,48.5));
#85397=CARTESIAN_POINT('Ctrl Pts',(41.5134374499321,3.00497958064079,48.35));
#85398=CARTESIAN_POINT('',(41.3768754601479,3.33212831616402,48.5));
#85399=CARTESIAN_POINT('Ctrl Pts',(41.3768754601479,3.33212831616402,48.5));
#85400=CARTESIAN_POINT('Ctrl Pts',(41.4639149308205,3.19781729578972,48.5));
#85401=CARTESIAN_POINT('Ctrl Pts',(41.5134374499321,3.00497958064079,48.5));
#85402=CARTESIAN_POINT('',(41.3768754601479,3.33212831616402,48.35));
#85403=CARTESIAN_POINT('',(41.3768754601479,3.33212831616402,48.5));
#85404=CARTESIAN_POINT('Ctrl Pts',(41.3768754601479,3.33212831616402,48.35));
#85405=CARTESIAN_POINT('Ctrl Pts',(41.4639149308205,3.19781729578972,48.35));
#85406=CARTESIAN_POINT('Ctrl Pts',(41.5134374499321,3.00497958064079,48.35));
#85407=CARTESIAN_POINT('Ctrl Pts',(41.1562756896019,3.5377217233181,48.5));
#85408=CARTESIAN_POINT('Ctrl Pts',(41.1562756896019,3.5377217233181,48.35));
#85409=CARTESIAN_POINT('Ctrl Pts',(41.2898359894753,3.46643933653831,48.5));
#85410=CARTESIAN_POINT('Ctrl Pts',(41.2898359894753,3.46643933653831,48.35));
#85411=CARTESIAN_POINT('Ctrl Pts',(41.3768754601479,3.33212831616402,48.5));
#85412=CARTESIAN_POINT('Ctrl Pts',(41.3768754601479,3.33212831616402,48.35));
#85413=CARTESIAN_POINT('',(41.1562756896019,3.5377217233181,48.5));
#85414=CARTESIAN_POINT('Ctrl Pts',(41.1562756896019,3.5377217233181,48.5));
#85415=CARTESIAN_POINT('Ctrl Pts',(41.2898359894753,3.46643933653831,48.5));
#85416=CARTESIAN_POINT('Ctrl Pts',(41.3768754601479,3.33212831616402,48.5));
#85417=CARTESIAN_POINT('',(41.1562756896019,3.5377217233181,48.35));
#85418=CARTESIAN_POINT('',(41.1562756896019,3.5377217233181,48.5));
#85419=CARTESIAN_POINT('Ctrl Pts',(41.1562756896019,3.5377217233181,48.35));
#85420=CARTESIAN_POINT('Ctrl Pts',(41.2898359894753,3.46643933653831,48.35));
#85421=CARTESIAN_POINT('Ctrl Pts',(41.3768754601479,3.33212831616402,48.35));
#85422=CARTESIAN_POINT('Ctrl Pts',(40.845634162426,3.60900411009789,48.5));
#85423=CARTESIAN_POINT('Ctrl Pts',(40.845634162426,3.60900411009789,48.35));
#85424=CARTESIAN_POINT('Ctrl Pts',(41.0227147936821,3.60900411009789,48.5));
#85425=CARTESIAN_POINT('Ctrl Pts',(41.0227147936821,3.60900411009789,48.35));
#85426=CARTESIAN_POINT('Ctrl Pts',(41.1562756896019,3.5377217233181,48.5));
#85427=CARTESIAN_POINT('Ctrl Pts',(41.1562756896019,3.5377217233181,48.35));
#85428=CARTESIAN_POINT('',(40.845634162426,3.60900411009789,48.5));
#85429=CARTESIAN_POINT('Ctrl Pts',(40.845634162426,3.60900411009789,48.5));
#85430=CARTESIAN_POINT('Ctrl Pts',(41.0227147936821,3.60900411009789,48.5));
#85431=CARTESIAN_POINT('Ctrl Pts',(41.1562756896019,3.5377217233181,48.5));
#85432=CARTESIAN_POINT('',(40.845634162426,3.60900411009789,48.35));
#85433=CARTESIAN_POINT('',(40.845634162426,3.60900411009789,48.5));
#85434=CARTESIAN_POINT('Ctrl Pts',(40.845634162426,3.60900411009789,48.35));
#85435=CARTESIAN_POINT('Ctrl Pts',(41.0227147936821,3.60900411009789,48.35));
#85436=CARTESIAN_POINT('Ctrl Pts',(41.1562756896019,3.5377217233181,48.35));
#85437=CARTESIAN_POINT('Ctrl Pts',(40.4472033381462,3.47994545102119,48.5));
#85438=CARTESIAN_POINT('Ctrl Pts',(40.4472033381462,3.47994545102119,48.35));
#85439=CARTESIAN_POINT('Ctrl Pts',(40.6055251955986,3.60900411009789,48.5));
#85440=CARTESIAN_POINT('Ctrl Pts',(40.6055251955986,3.60900411009789,48.35));
#85441=CARTESIAN_POINT('Ctrl Pts',(40.845634162426,3.60900411009789,48.5));
#85442=CARTESIAN_POINT('Ctrl Pts',(40.845634162426,3.60900411009789,48.35));
#85443=CARTESIAN_POINT('',(40.4472033381462,3.47994545102119,48.5));
#85444=CARTESIAN_POINT('Ctrl Pts',(40.4472033381462,3.47994545102119,48.5));
#85445=CARTESIAN_POINT('Ctrl Pts',(40.6055251955986,3.60900411009789,48.5));
#85446=CARTESIAN_POINT('Ctrl Pts',(40.845634162426,3.60900411009789,48.5));
#85447=CARTESIAN_POINT('',(40.4472033381462,3.47994545102119,48.35));
#85448=CARTESIAN_POINT('',(40.4472033381462,3.47994545102119,48.5));
#85449=CARTESIAN_POINT('Ctrl Pts',(40.4472033381462,3.47994545102119,48.35));
#85450=CARTESIAN_POINT('Ctrl Pts',(40.6055251955986,3.60900411009789,48.35));
#85451=CARTESIAN_POINT('Ctrl Pts',(40.845634162426,3.60900411009789,48.35));
#85452=CARTESIAN_POINT('Ctrl Pts',(40.2085946202278,3.11302864551544,48.5));
#85453=CARTESIAN_POINT('Ctrl Pts',(40.2085946202278,3.11302864551544,48.35));
#85454=CARTESIAN_POINT('Ctrl Pts',(40.2888811826706,3.3508867919445,48.5));
#85455=CARTESIAN_POINT('Ctrl Pts',(40.2888811826706,3.3508867919445,48.35));
#85456=CARTESIAN_POINT('Ctrl Pts',(40.4472033381462,3.47994545102119,48.5));
#85457=CARTESIAN_POINT('Ctrl Pts',(40.4472033381462,3.47994545102119,48.35));
#85458=CARTESIAN_POINT('',(40.2085946202278,3.11302864551544,48.5));
#85459=CARTESIAN_POINT('Ctrl Pts',(40.2085946202278,3.11302864551544,48.5));
#85460=CARTESIAN_POINT('Ctrl Pts',(40.2888811826706,3.3508867919445,48.5));
#85461=CARTESIAN_POINT('Ctrl Pts',(40.4472033381462,3.47994545102119,48.5));
#85462=CARTESIAN_POINT('',(40.2085946202278,3.11302864551544,48.35));
#85463=CARTESIAN_POINT('',(40.2085946202278,3.11302864551544,48.5));
#85464=CARTESIAN_POINT('Ctrl Pts',(40.2085946202278,3.11302864551544,48.35));
#85465=CARTESIAN_POINT('Ctrl Pts',(40.2888811826706,3.3508867919445,48.35));
#85466=CARTESIAN_POINT('Ctrl Pts',(40.4472033381462,3.47994545102119,48.35));
#85467=CARTESIAN_POINT('Ctrl Pts',(40.1283083558083,2.48499327898026,48.5));
#85468=CARTESIAN_POINT('Ctrl Pts',(40.1283083558083,2.48499327898026,48.35));
#85469=CARTESIAN_POINT('Ctrl Pts',(40.1283083558083,2.87517049908638,48.5));
#85470=CARTESIAN_POINT('Ctrl Pts',(40.1283083558083,2.87517049908638,48.35));
#85471=CARTESIAN_POINT('Ctrl Pts',(40.2085946202278,3.11302864551544,48.5));
#85472=CARTESIAN_POINT('Ctrl Pts',(40.2085946202278,3.11302864551544,48.35));
#85473=CARTESIAN_POINT('',(40.1283083558083,2.48499327898026,48.5));
#85474=CARTESIAN_POINT('Ctrl Pts',(40.1283083558083,2.48499327898026,48.5));
#85475=CARTESIAN_POINT('Ctrl Pts',(40.1283083558083,2.87517049908638,48.5));
#85476=CARTESIAN_POINT('Ctrl Pts',(40.2085946202278,3.11302864551544,48.5));
#85477=CARTESIAN_POINT('',(40.1283083558083,2.48499327898026,48.35));
#85478=CARTESIAN_POINT('',(40.1283083558083,2.48499327898026,48.5));
#85479=CARTESIAN_POINT('Ctrl Pts',(40.1283083558083,2.48499327898026,48.35));
#85480=CARTESIAN_POINT('Ctrl Pts',(40.1283083558083,2.87517049908638,48.35));
#85481=CARTESIAN_POINT('Ctrl Pts',(40.2085946202278,3.11302864551544,48.35));
#85482=CARTESIAN_POINT('Ctrl Pts',(40.3459070324898,1.59058684110642,48.5));
#85483=CARTESIAN_POINT('Ctrl Pts',(40.3459070324898,1.59058684110642,48.35));
#85484=CARTESIAN_POINT('Ctrl Pts',(40.1283083558083,1.86521166563034,48.5));
#85485=CARTESIAN_POINT('Ctrl Pts',(40.1283083558083,1.86521166563034,48.35));
#85486=CARTESIAN_POINT('Ctrl Pts',(40.1283083558083,2.48499327898026,48.5));
#85487=CARTESIAN_POINT('Ctrl Pts',(40.1283083558083,2.48499327898026,48.35));
#85488=CARTESIAN_POINT('Ctrl Pts',(40.3459070324898,1.59058684110642,48.5));
#85489=CARTESIAN_POINT('Ctrl Pts',(40.1283083558083,1.86521166563034,48.5));
#85490=CARTESIAN_POINT('Ctrl Pts',(40.1283083558083,2.48499327898026,48.5));
#85491=CARTESIAN_POINT('Ctrl Pts',(40.3459070324898,1.59058684110642,48.35));
#85492=CARTESIAN_POINT('Ctrl Pts',(40.1283083558083,1.86521166563034,48.35));
#85493=CARTESIAN_POINT('Ctrl Pts',(40.1283083558083,2.48499327898026,48.35));
#85494=CARTESIAN_POINT('Origin',(39.9999997466803,2.48574362695217,48.35));
#85495=CARTESIAN_POINT('Ctrl Pts',(39.1266029775143,2.7363575398922,48.5));
#85496=CARTESIAN_POINT('Ctrl Pts',(39.1266029775143,2.7363575398922,48.35));
#85497=CARTESIAN_POINT('Ctrl Pts',(39.3089358210564,3.07776266336441,48.5));
#85498=CARTESIAN_POINT('Ctrl Pts',(39.3089358210564,3.07776266336441,48.35));
#85499=CARTESIAN_POINT('Ctrl Pts',(39.5145292282104,3.3118691444397,48.5));
#85500=CARTESIAN_POINT('Ctrl Pts',(39.5145292282104,3.3118691444397,48.35));
#85501=CARTESIAN_POINT('',(39.1266029775143,2.7363575398922,48.5));
#85502=CARTESIAN_POINT('',(39.5145292282104,3.3118691444397,48.5));
#85503=CARTESIAN_POINT('Ctrl Pts',(39.1266029775143,2.7363575398922,48.5));
#85504=CARTESIAN_POINT('Ctrl Pts',(39.3089358210564,3.07776266336441,48.5));
#85505=CARTESIAN_POINT('Ctrl Pts',(39.5145292282104,3.3118691444397,48.5));
#85506=CARTESIAN_POINT('',(39.1266029775143,2.7363575398922,48.35));
#85507=CARTESIAN_POINT('',(39.1266029775143,2.7363575398922,48.5));
#85508=CARTESIAN_POINT('',(39.5145292282104,3.3118691444397,48.35));
#85509=CARTESIAN_POINT('Ctrl Pts',(39.1266029775143,2.7363575398922,48.35));
#85510=CARTESIAN_POINT('Ctrl Pts',(39.3089358210564,3.07776266336441,48.35));
#85511=CARTESIAN_POINT('Ctrl Pts',(39.5145292282104,3.3118691444397,48.35));
#85512=CARTESIAN_POINT('',(39.5145292282104,3.3118691444397,48.5));
#85513=CARTESIAN_POINT('Ctrl Pts',(38.8467257916927,2.02728533744812,48.5));
#85514=CARTESIAN_POINT('Ctrl Pts',(38.8467257916927,2.02728533744812,48.35));
#85515=CARTESIAN_POINT('Ctrl Pts',(38.9442701339722,2.39495241641998,48.5));
#85516=CARTESIAN_POINT('Ctrl Pts',(38.9442701339722,2.39495241641998,48.35));
#85517=CARTESIAN_POINT('Ctrl Pts',(39.1266029775143,2.7363575398922,48.5));
#85518=CARTESIAN_POINT('Ctrl Pts',(39.1266029775143,2.7363575398922,48.35));
#85519=CARTESIAN_POINT('',(38.8467257916927,2.02728533744812,48.5));
#85520=CARTESIAN_POINT('Ctrl Pts',(38.8467257916927,2.02728533744812,48.5));
#85521=CARTESIAN_POINT('Ctrl Pts',(38.9442701339722,2.39495241641998,48.5));
#85522=CARTESIAN_POINT('Ctrl Pts',(39.1266029775143,2.7363575398922,48.5));
#85523=CARTESIAN_POINT('',(38.8467257916927,2.02728533744812,48.35));
#85524=CARTESIAN_POINT('',(38.8467257916927,2.02728533744812,48.5));
#85525=CARTESIAN_POINT('Ctrl Pts',(38.8467257916927,2.02728533744812,48.35));
#85526=CARTESIAN_POINT('Ctrl Pts',(38.9442701339722,2.39495241641998,48.35));
#85527=CARTESIAN_POINT('Ctrl Pts',(39.1266029775143,2.7363575398922,48.35));
#85528=CARTESIAN_POINT('Ctrl Pts',(38.7446793615818,1.40000009536743,48.5));
#85529=CARTESIAN_POINT('Ctrl Pts',(38.7446793615818,1.40000009536743,48.35));
#85530=CARTESIAN_POINT('Ctrl Pts',(38.7491814494133,1.65961825847626,48.5));
#85531=CARTESIAN_POINT('Ctrl Pts',(38.7491814494133,1.65961825847626,48.35));
#85532=CARTESIAN_POINT('Ctrl Pts',(38.8467257916927,2.02728533744812,48.5));
#85533=CARTESIAN_POINT('Ctrl Pts',(38.8467257916927,2.02728533744812,48.35));
#85534=CARTESIAN_POINT('',(38.7446793615818,1.40000009536743,48.5));
#85535=CARTESIAN_POINT('Ctrl Pts',(38.7446793615818,1.40000009536743,48.5));
#85536=CARTESIAN_POINT('Ctrl Pts',(38.7491814494133,1.65961825847626,48.5));
#85537=CARTESIAN_POINT('Ctrl Pts',(38.8467257916927,2.02728533744812,48.5));
#85538=CARTESIAN_POINT('',(38.7446793615818,1.40000009536743,48.35));
#85539=CARTESIAN_POINT('',(38.7446793615818,1.40000009536743,48.5));
#85540=CARTESIAN_POINT('Ctrl Pts',(38.7446793615818,1.40000009536743,48.35));
#85541=CARTESIAN_POINT('Ctrl Pts',(38.7491814494133,1.65961825847626,48.35));
#85542=CARTESIAN_POINT('Ctrl Pts',(38.8467257916927,2.02728533744812,48.35));
#85543=CARTESIAN_POINT('Origin',(39.0223055779934,1.40000009536743,48.5));
#85544=CARTESIAN_POINT('',(39.0223055779934,1.40000009536743,48.5));
#85545=CARTESIAN_POINT('',(19.5111527889967,1.40000009536743,48.5));
#85546=CARTESIAN_POINT('',(39.0223055779934,1.40000009536743,48.35));
#85547=CARTESIAN_POINT('',(39.0223055779934,1.40000009536743,48.5));
#85548=CARTESIAN_POINT('',(39.0223055779934,1.40000009536743,48.35));
#85549=CARTESIAN_POINT('Ctrl Pts',(39.1258527040482,2.00477504730225,48.5));
#85550=CARTESIAN_POINT('Ctrl Pts',(39.1258527040482,2.00477504730225,48.35));
#85551=CARTESIAN_POINT('Ctrl Pts',(39.0448157191277,1.72864937782288,48.5));
#85552=CARTESIAN_POINT('Ctrl Pts',(39.0448157191277,1.72864937782288,48.35));
#85553=CARTESIAN_POINT('Ctrl Pts',(39.0223055779934,1.40000009536743,48.5));
#85554=CARTESIAN_POINT('Ctrl Pts',(39.0223055779934,1.40000009536743,48.35));
#85555=CARTESIAN_POINT('',(39.1258527040482,2.00477504730225,48.5));
#85556=CARTESIAN_POINT('Ctrl Pts',(39.1258527040482,2.00477504730225,48.5));
#85557=CARTESIAN_POINT('Ctrl Pts',(39.0448157191277,1.72864937782288,48.5));
#85558=CARTESIAN_POINT('Ctrl Pts',(39.0223055779934,1.40000009536743,48.5));
#85559=CARTESIAN_POINT('',(39.1258527040482,2.00477504730225,48.35));
#85560=CARTESIAN_POINT('',(39.1258527040482,2.00477504730225,48.5));
#85561=CARTESIAN_POINT('Ctrl Pts',(39.1258527040482,2.00477504730225,48.35));
#85562=CARTESIAN_POINT('Ctrl Pts',(39.0448157191277,1.72864937782288,48.35));
#85563=CARTESIAN_POINT('Ctrl Pts',(39.0223055779934,1.40000009536743,48.35));
#85564=CARTESIAN_POINT('Ctrl Pts',(39.4447473883629,2.76712143421173,48.5));
#85565=CARTESIAN_POINT('Ctrl Pts',(39.4447473883629,2.76712143421173,48.35));
#85566=CARTESIAN_POINT('Ctrl Pts',(39.2384038567543,2.3964529633522,48.5));
#85567=CARTESIAN_POINT('Ctrl Pts',(39.2384038567543,2.3964529633522,48.35));
#85568=CARTESIAN_POINT('Ctrl Pts',(39.1258527040482,2.00477504730225,48.5));
#85569=CARTESIAN_POINT('Ctrl Pts',(39.1258527040482,2.00477504730225,48.35));
#85570=CARTESIAN_POINT('',(39.4447473883629,2.76712143421173,48.5));
#85571=CARTESIAN_POINT('Ctrl Pts',(39.4447473883629,2.76712143421173,48.5));
#85572=CARTESIAN_POINT('Ctrl Pts',(39.2384038567543,2.3964529633522,48.5));
#85573=CARTESIAN_POINT('Ctrl Pts',(39.1258527040482,2.00477504730225,48.5));
#85574=CARTESIAN_POINT('',(39.4447473883629,2.76712143421173,48.35));
#85575=CARTESIAN_POINT('',(39.4447473883629,2.76712143421173,48.5));
#85576=CARTESIAN_POINT('Ctrl Pts',(39.4447473883629,2.76712143421173,48.35));
#85577=CARTESIAN_POINT('Ctrl Pts',(39.2384038567543,2.3964529633522,48.35));
#85578=CARTESIAN_POINT('Ctrl Pts',(39.1258527040482,2.00477504730225,48.35));
#85579=CARTESIAN_POINT('Ctrl Pts',(39.8611868619919,3.36139166355133,48.5));
#85580=CARTESIAN_POINT('Ctrl Pts',(39.8611868619919,3.36139166355133,48.35));
#85581=CARTESIAN_POINT('Ctrl Pts',(39.6510915160179,3.13779005408287,48.5));
#85582=CARTESIAN_POINT('Ctrl Pts',(39.6510915160179,3.13779005408287,48.35));
#85583=CARTESIAN_POINT('Ctrl Pts',(39.4447473883629,2.76712143421173,48.5));
#85584=CARTESIAN_POINT('Ctrl Pts',(39.4447473883629,2.76712143421173,48.35));
#85585=CARTESIAN_POINT('',(39.8611868619919,3.36139166355133,48.5));
#85586=CARTESIAN_POINT('Ctrl Pts',(39.8611868619919,3.36139166355133,48.5));
#85587=CARTESIAN_POINT('Ctrl Pts',(39.6510915160179,3.13779005408287,48.5));
#85588=CARTESIAN_POINT('Ctrl Pts',(39.4447473883629,2.76712143421173,48.5));
#85589=CARTESIAN_POINT('',(39.8611868619919,3.36139166355133,48.35));
#85590=CARTESIAN_POINT('',(39.8611868619919,3.36139166355133,48.5));
#85591=CARTESIAN_POINT('Ctrl Pts',(39.8611868619919,3.36139166355133,48.35));
#85592=CARTESIAN_POINT('Ctrl Pts',(39.6510915160179,3.13779005408287,48.35));
#85593=CARTESIAN_POINT('Ctrl Pts',(39.4447473883629,2.76712143421173,48.35));
#85594=CARTESIAN_POINT('Origin',(39.8611868619919,3.57148715853691,48.5));
#85595=CARTESIAN_POINT('',(39.8611868619919,3.57148715853691,48.5));
#85596=CARTESIAN_POINT('',(39.8611868619919,5.78574357926846,48.5));
#85597=CARTESIAN_POINT('',(39.8611868619919,3.57148715853691,48.35));
#85598=CARTESIAN_POINT('',(39.8611868619919,3.57148715853691,48.5));
#85599=CARTESIAN_POINT('',(39.8611868619919,3.57148715853691,48.35));
#85600=CARTESIAN_POINT('Origin',(38.4370395243168,3.57148715853691,48.5));
#85601=CARTESIAN_POINT('',(38.4370395243168,3.57148715853691,48.5));
#85602=CARTESIAN_POINT('',(19.2185197621584,3.57148715853691,48.5));
#85603=CARTESIAN_POINT('',(38.4370395243168,3.57148715853691,48.35));
#85604=CARTESIAN_POINT('',(38.4370395243168,3.57148715853691,48.5));
#85605=CARTESIAN_POINT('',(38.4370395243168,3.57148715853691,48.35));
#85606=CARTESIAN_POINT('Origin',(38.4370395243168,3.3118691444397,48.5));
#85607=CARTESIAN_POINT('',(38.4370395243168,3.3118691444397,48.5));
#85608=CARTESIAN_POINT('',(38.4370395243168,5.65593457221985,48.5));
#85609=CARTESIAN_POINT('',(38.4370395243168,3.3118691444397,48.35));
#85610=CARTESIAN_POINT('',(38.4370395243168,3.3118691444397,48.5));
#85611=CARTESIAN_POINT('',(38.4370395243168,3.3118691444397,48.35));
#85612=CARTESIAN_POINT('Origin',(39.5145292282104,3.3118691444397,48.5));
#85613=CARTESIAN_POINT('',(19.7572646141052,3.3118691444397,48.5));
#85614=CARTESIAN_POINT('',(39.5145292282104,3.3118691444397,48.35));
#85615=CARTESIAN_POINT('Origin',(39.9999997466803,2.48574362695217,48.35));
#85616=CARTESIAN_POINT('Origin',(0.,8.,48.5));
#85617=CARTESIAN_POINT('Ctrl Pts',(30.8531378936023,3.38540250062943,48.5));
#85618=CARTESIAN_POINT('Ctrl Pts',(30.8531378936023,3.38540250062943,48.35));
#85619=CARTESIAN_POINT('Ctrl Pts',(30.6670530866832,3.38540250062943,48.5));
#85620=CARTESIAN_POINT('Ctrl Pts',(30.6670530866832,3.38540250062943,48.35));
#85621=CARTESIAN_POINT('Ctrl Pts',(30.5560027789325,3.22783091664314,48.5));
#85622=CARTESIAN_POINT('Ctrl Pts',(30.5560027789325,3.22783091664314,48.35));
#85623=CARTESIAN_POINT('',(30.8531378936023,3.38540250062943,48.5));
#85624=CARTESIAN_POINT('',(30.5560027789325,3.22783091664314,48.5));
#85625=CARTESIAN_POINT('Ctrl Pts',(30.8531378936023,3.38540250062943,48.5));
#85626=CARTESIAN_POINT('Ctrl Pts',(30.6670530866832,3.38540250062943,48.5));
#85627=CARTESIAN_POINT('Ctrl Pts',(30.5560027789325,3.22783091664314,48.5));
#85628=CARTESIAN_POINT('',(30.8531378936023,3.38540250062943,48.35));
#85629=CARTESIAN_POINT('',(30.8531378936023,3.38540250062943,48.5));
#85630=CARTESIAN_POINT('',(30.5560027789325,3.22783091664314,48.35));
#85631=CARTESIAN_POINT('Ctrl Pts',(30.8531378936023,3.38540250062943,48.35));
#85632=CARTESIAN_POINT('Ctrl Pts',(30.6670530866832,3.38540250062943,48.35));
#85633=CARTESIAN_POINT('Ctrl Pts',(30.5560027789325,3.22783091664314,48.35));
#85634=CARTESIAN_POINT('',(30.5560027789325,3.22783091664314,48.5));
#85635=CARTESIAN_POINT('Ctrl Pts',(31.1690311860293,3.2068213224411,48.5));
#85636=CARTESIAN_POINT('Ctrl Pts',(31.1690311860293,3.2068213224411,48.35));
#85637=CARTESIAN_POINT('Ctrl Pts',(31.0422234963626,3.38540250062943,48.5));
#85638=CARTESIAN_POINT('Ctrl Pts',(31.0422234963626,3.38540250062943,48.35));
#85639=CARTESIAN_POINT('Ctrl Pts',(30.8531378936023,3.38540250062943,48.5));
#85640=CARTESIAN_POINT('Ctrl Pts',(30.8531378936023,3.38540250062943,48.35));
#85641=CARTESIAN_POINT('',(31.1690311860293,3.2068213224411,48.5));
#85642=CARTESIAN_POINT('Ctrl Pts',(31.1690311860293,3.2068213224411,48.5));
#85643=CARTESIAN_POINT('Ctrl Pts',(31.0422234963626,3.38540250062943,48.5));
#85644=CARTESIAN_POINT('Ctrl Pts',(30.8531378936023,3.38540250062943,48.5));
#85645=CARTESIAN_POINT('',(31.1690311860293,3.2068213224411,48.35));
#85646=CARTESIAN_POINT('',(31.1690311860293,3.2068213224411,48.5));
#85647=CARTESIAN_POINT('Ctrl Pts',(31.1690311860293,3.2068213224411,48.35));
#85648=CARTESIAN_POINT('Ctrl Pts',(31.0422234963626,3.38540250062943,48.35));
#85649=CARTESIAN_POINT('Ctrl Pts',(30.8531378936023,3.38540250062943,48.35));
#85650=CARTESIAN_POINT('Ctrl Pts',(31.2958388756961,2.48499327898026,48.5));
#85651=CARTESIAN_POINT('Ctrl Pts',(31.2958388756961,2.48499327898026,48.35));
#85652=CARTESIAN_POINT('Ctrl Pts',(31.2958388756961,3.02824014425278,48.5));
#85653=CARTESIAN_POINT('Ctrl Pts',(31.2958388756961,3.02824014425278,48.35));
#85654=CARTESIAN_POINT('Ctrl Pts',(31.1690311860293,3.2068213224411,48.5));
#85655=CARTESIAN_POINT('Ctrl Pts',(31.1690311860293,3.2068213224411,48.35));
#85656=CARTESIAN_POINT('',(31.2958388756961,2.48499327898026,48.5));
#85657=CARTESIAN_POINT('Ctrl Pts',(31.2958388756961,2.48499327898026,48.5));
#85658=CARTESIAN_POINT('Ctrl Pts',(31.2958388756961,3.02824014425278,48.5));
#85659=CARTESIAN_POINT('Ctrl Pts',(31.1690311860293,3.2068213224411,48.5));
#85660=CARTESIAN_POINT('',(31.2958388756961,2.48499327898026,48.35));
#85661=CARTESIAN_POINT('',(31.2958388756961,2.48499327898026,48.5));
#85662=CARTESIAN_POINT('Ctrl Pts',(31.2958388756961,2.48499327898026,48.35));
#85663=CARTESIAN_POINT('Ctrl Pts',(31.2958388756961,3.02824014425278,48.35));
#85664=CARTESIAN_POINT('Ctrl Pts',(31.1690311860293,3.2068213224411,48.35));
#85665=CARTESIAN_POINT('Ctrl Pts',(31.1690311860293,1.76466578245163,48.5));
#85666=CARTESIAN_POINT('Ctrl Pts',(31.1690311860293,1.76466578245163,48.35));
#85667=CARTESIAN_POINT('Ctrl Pts',(31.2958388756961,1.9447478055954,48.5));
#85668=CARTESIAN_POINT('Ctrl Pts',(31.2958388756961,1.9447478055954,48.35));
#85669=CARTESIAN_POINT('Ctrl Pts',(31.2958388756961,2.48499327898026,48.5));
#85670=CARTESIAN_POINT('Ctrl Pts',(31.2958388756961,2.48499327898026,48.35));
#85671=CARTESIAN_POINT('',(31.1690311860293,1.76466578245163,48.5));
#85672=CARTESIAN_POINT('Ctrl Pts',(31.1690311860293,1.76466578245163,48.5));
#85673=CARTESIAN_POINT('Ctrl Pts',(31.2958388756961,1.9447478055954,48.5));
#85674=CARTESIAN_POINT('Ctrl Pts',(31.2958388756961,2.48499327898026,48.5));
#85675=CARTESIAN_POINT('',(31.1690311860293,1.76466578245163,48.35));
#85676=CARTESIAN_POINT('',(31.1690311860293,1.76466578245163,48.5));
#85677=CARTESIAN_POINT('Ctrl Pts',(31.1690311860293,1.76466578245163,48.35));
#85678=CARTESIAN_POINT('Ctrl Pts',(31.2958388756961,1.9447478055954,48.35));
#85679=CARTESIAN_POINT('Ctrl Pts',(31.2958388756961,2.48499327898026,48.35));
#85680=CARTESIAN_POINT('Ctrl Pts',(30.8561389874667,1.58458405733109,48.5));
#85681=CARTESIAN_POINT('Ctrl Pts',(30.8561389874667,1.58458405733109,48.35));
#85682=CARTESIAN_POINT('Ctrl Pts',(31.0422234963626,1.58458405733109,48.5));
#85683=CARTESIAN_POINT('Ctrl Pts',(31.0422234963626,1.58458405733109,48.35));
#85684=CARTESIAN_POINT('Ctrl Pts',(31.1690311860293,1.76466578245163,48.5));
#85685=CARTESIAN_POINT('Ctrl Pts',(31.1690311860293,1.76466578245163,48.35));
#85686=CARTESIAN_POINT('',(30.8561389874667,1.58458405733109,48.5));
#85687=CARTESIAN_POINT('Ctrl Pts',(30.8561389874667,1.58458405733109,48.5));
#85688=CARTESIAN_POINT('Ctrl Pts',(31.0422234963626,1.58458405733109,48.5));
#85689=CARTESIAN_POINT('Ctrl Pts',(31.1690311860293,1.76466578245163,48.5));
#85690=CARTESIAN_POINT('',(30.8561389874667,1.58458405733109,48.35));
#85691=CARTESIAN_POINT('',(30.8561389874667,1.58458405733109,48.5));
#85692=CARTESIAN_POINT('Ctrl Pts',(30.8561389874667,1.58458405733109,48.35));
#85693=CARTESIAN_POINT('Ctrl Pts',(31.0422234963626,1.58458405733109,48.35));
#85694=CARTESIAN_POINT('Ctrl Pts',(31.1690311860293,1.76466578245163,48.35));
#85695=CARTESIAN_POINT('Ctrl Pts',(30.5432467889041,1.76391565799713,48.5));
#85696=CARTESIAN_POINT('Ctrl Pts',(30.5432467889041,1.76391565799713,48.35));
#85697=CARTESIAN_POINT('Ctrl Pts',(30.6700544785708,1.58458405733109,48.5));
#85698=CARTESIAN_POINT('Ctrl Pts',(30.6700544785708,1.58458405733109,48.35));
#85699=CARTESIAN_POINT('Ctrl Pts',(30.8561389874667,1.58458405733109,48.5));
#85700=CARTESIAN_POINT('Ctrl Pts',(30.8561389874667,1.58458405733109,48.35));
#85701=CARTESIAN_POINT('',(30.5432467889041,1.76391565799713,48.5));
#85702=CARTESIAN_POINT('Ctrl Pts',(30.5432467889041,1.76391565799713,48.5));
#85703=CARTESIAN_POINT('Ctrl Pts',(30.6700544785708,1.58458405733109,48.5));
#85704=CARTESIAN_POINT('Ctrl Pts',(30.8561389874667,1.58458405733109,48.5));
#85705=CARTESIAN_POINT('',(30.5432467889041,1.76391565799713,48.35));
#85706=CARTESIAN_POINT('',(30.5432467889041,1.76391565799713,48.5));
#85707=CARTESIAN_POINT('Ctrl Pts',(30.5432467889041,1.76391565799713,48.35));
#85708=CARTESIAN_POINT('Ctrl Pts',(30.6700544785708,1.58458405733109,48.35));
#85709=CARTESIAN_POINT('Ctrl Pts',(30.8561389874667,1.58458405733109,48.35));
#85710=CARTESIAN_POINT('Ctrl Pts',(30.4164390992373,2.48499327898026,48.5));
#85711=CARTESIAN_POINT('Ctrl Pts',(30.4164390992373,2.48499327898026,48.35));
#85712=CARTESIAN_POINT('Ctrl Pts',(30.4164390992373,1.94324696063995,48.5));
#85713=CARTESIAN_POINT('Ctrl Pts',(30.4164390992373,1.94324696063995,48.35));
#85714=CARTESIAN_POINT('Ctrl Pts',(30.5432467889041,1.76391565799713,48.5));
#85715=CARTESIAN_POINT('Ctrl Pts',(30.5432467889041,1.76391565799713,48.35));
#85716=CARTESIAN_POINT('',(30.4164390992373,2.48499327898026,48.5));
#85717=CARTESIAN_POINT('Ctrl Pts',(30.4164390992373,2.48499327898026,48.5));
#85718=CARTESIAN_POINT('Ctrl Pts',(30.4164390992373,1.94324696063995,48.5));
#85719=CARTESIAN_POINT('Ctrl Pts',(30.5432467889041,1.76391565799713,48.5));
#85720=CARTESIAN_POINT('',(30.4164390992373,2.48499327898026,48.35));
#85721=CARTESIAN_POINT('',(30.4164390992373,2.48499327898026,48.5));
#85722=CARTESIAN_POINT('Ctrl Pts',(30.4164390992373,2.48499327898026,48.35));
#85723=CARTESIAN_POINT('Ctrl Pts',(30.4164390992373,1.94324696063995,48.35));
#85724=CARTESIAN_POINT('Ctrl Pts',(30.5432467889041,1.76391565799713,48.35));
#85725=CARTESIAN_POINT('Ctrl Pts',(30.5560027789325,3.22783091664314,48.5));
#85726=CARTESIAN_POINT('Ctrl Pts',(30.5560027789325,3.22783091664314,48.35));
#85727=CARTESIAN_POINT('Ctrl Pts',(30.4164390992373,3.02673944830894,48.5));
#85728=CARTESIAN_POINT('Ctrl Pts',(30.4164390992373,3.02673944830894,48.35));
#85729=CARTESIAN_POINT('Ctrl Pts',(30.4164390992373,2.48499327898026,48.5));
#85730=CARTESIAN_POINT('Ctrl Pts',(30.4164390992373,2.48499327898026,48.35));
#85731=CARTESIAN_POINT('Ctrl Pts',(30.5560027789325,3.22783091664314,48.5));
#85732=CARTESIAN_POINT('Ctrl Pts',(30.4164390992373,3.02673944830894,48.5));
#85733=CARTESIAN_POINT('Ctrl Pts',(30.4164390992373,2.48499327898026,48.5));
#85734=CARTESIAN_POINT('Ctrl Pts',(30.5560027789325,3.22783091664314,48.35));
#85735=CARTESIAN_POINT('Ctrl Pts',(30.4164390992373,3.02673944830894,48.35));
#85736=CARTESIAN_POINT('Ctrl Pts',(30.4164390992373,2.48499327898026,48.35));
#85737=CARTESIAN_POINT('Ctrl Pts',(30.8561389874667,1.36248314380646,48.5));
#85738=CARTESIAN_POINT('Ctrl Pts',(30.8561389874667,1.36248314380646,48.35));
#85739=CARTESIAN_POINT('Ctrl Pts',(30.5379944276065,1.36248314380646,48.5));
#85740=CARTESIAN_POINT('Ctrl Pts',(30.5379944276065,1.36248314380646,48.35));
#85741=CARTESIAN_POINT('Ctrl Pts',(30.3564118575305,1.59058684110642,48.5));
#85742=CARTESIAN_POINT('Ctrl Pts',(30.3564118575305,1.59058684110642,48.35));
#85743=CARTESIAN_POINT('',(30.8561389874667,1.36248314380646,48.5));
#85744=CARTESIAN_POINT('',(30.3564118575305,1.59058684110642,48.5));
#85745=CARTESIAN_POINT('Ctrl Pts',(30.8561389874667,1.36248314380646,48.5));
#85746=CARTESIAN_POINT('Ctrl Pts',(30.5379944276065,1.36248314380646,48.5));
#85747=CARTESIAN_POINT('Ctrl Pts',(30.3564118575305,1.59058684110642,48.5));
#85748=CARTESIAN_POINT('',(30.8561389874667,1.36248314380646,48.35));
#85749=CARTESIAN_POINT('',(30.8561389874667,1.36248314380646,48.5));
#85750=CARTESIAN_POINT('',(30.3564118575305,1.59058684110642,48.35));
#85751=CARTESIAN_POINT('Ctrl Pts',(30.8561389874667,1.36248314380646,48.35));
#85752=CARTESIAN_POINT('Ctrl Pts',(30.5379944276065,1.36248314380646,48.35));
#85753=CARTESIAN_POINT('Ctrl Pts',(30.3564118575305,1.59058684110642,48.35));
#85754=CARTESIAN_POINT('',(30.3564118575305,1.59058684110642,48.5));
#85755=CARTESIAN_POINT('Ctrl Pts',(31.2560706567019,1.49229192733765,48.5));
#85756=CARTESIAN_POINT('Ctrl Pts',(31.2560706567019,1.49229192733765,48.35));
#85757=CARTESIAN_POINT('Ctrl Pts',(31.0977487992495,1.36248314380646,48.5));
#85758=CARTESIAN_POINT('Ctrl Pts',(31.0977487992495,1.36248314380646,48.35));
#85759=CARTESIAN_POINT('Ctrl Pts',(30.8561389874667,1.36248314380646,48.5));
#85760=CARTESIAN_POINT('Ctrl Pts',(30.8561389874667,1.36248314380646,48.35));
#85761=CARTESIAN_POINT('',(31.2560706567019,1.49229192733765,48.5));
#85762=CARTESIAN_POINT('Ctrl Pts',(31.2560706567019,1.49229192733765,48.5));
#85763=CARTESIAN_POINT('Ctrl Pts',(31.0977487992495,1.36248314380646,48.5));
#85764=CARTESIAN_POINT('Ctrl Pts',(30.8561389874667,1.36248314380646,48.5));
#85765=CARTESIAN_POINT('',(31.2560706567019,1.49229192733765,48.35));
#85766=CARTESIAN_POINT('',(31.2560706567019,1.49229192733765,48.5));
#85767=CARTESIAN_POINT('Ctrl Pts',(31.2560706567019,1.49229192733765,48.35));
#85768=CARTESIAN_POINT('Ctrl Pts',(31.0977487992495,1.36248314380646,48.35));
#85769=CARTESIAN_POINT('Ctrl Pts',(30.8561389874667,1.36248314380646,48.35));
#85770=CARTESIAN_POINT('Ctrl Pts',(31.4939289521426,1.85995900630951,48.5));
#85771=CARTESIAN_POINT('Ctrl Pts',(31.4939289521426,1.85995900630951,48.35));
#85772=CARTESIAN_POINT('Ctrl Pts',(31.4143925141543,1.62210100889206,48.5));
#85773=CARTESIAN_POINT('Ctrl Pts',(31.4143925141543,1.62210100889206,48.35));
#85774=CARTESIAN_POINT('Ctrl Pts',(31.2560706567019,1.49229192733765,48.5));
#85775=CARTESIAN_POINT('Ctrl Pts',(31.2560706567019,1.49229192733765,48.35));
#85776=CARTESIAN_POINT('',(31.4939289521426,1.85995900630951,48.5));
#85777=CARTESIAN_POINT('Ctrl Pts',(31.4939289521426,1.85995900630951,48.5));
#85778=CARTESIAN_POINT('Ctrl Pts',(31.4143925141543,1.62210100889206,48.5));
#85779=CARTESIAN_POINT('Ctrl Pts',(31.2560706567019,1.49229192733765,48.5));
#85780=CARTESIAN_POINT('',(31.4939289521426,1.85995900630951,48.35));
#85781=CARTESIAN_POINT('',(31.4939289521426,1.85995900630951,48.5));
#85782=CARTESIAN_POINT('Ctrl Pts',(31.4939289521426,1.85995900630951,48.35));
#85783=CARTESIAN_POINT('Ctrl Pts',(31.4143925141543,1.62210100889206,48.35));
#85784=CARTESIAN_POINT('Ctrl Pts',(31.2560706567019,1.49229192733765,48.35));
#85785=CARTESIAN_POINT('Ctrl Pts',(31.5734647940844,2.48499327898026,48.5));
#85786=CARTESIAN_POINT('Ctrl Pts',(31.5734647940844,2.48499327898026,48.35));
#85787=CARTESIAN_POINT('Ctrl Pts',(31.5734647940844,2.09781730175018,48.5));
#85788=CARTESIAN_POINT('Ctrl Pts',(31.5734647940844,2.09781730175018,48.35));
#85789=CARTESIAN_POINT('Ctrl Pts',(31.4939289521426,1.85995900630951,48.5));
#85790=CARTESIAN_POINT('Ctrl Pts',(31.4939289521426,1.85995900630951,48.35));
#85791=CARTESIAN_POINT('',(31.5734647940844,2.48499327898026,48.5));
#85792=CARTESIAN_POINT('Ctrl Pts',(31.5734647940844,2.48499327898026,48.5));
#85793=CARTESIAN_POINT('Ctrl Pts',(31.5734647940844,2.09781730175018,48.5));
#85794=CARTESIAN_POINT('Ctrl Pts',(31.4939289521426,1.85995900630951,48.5));
#85795=CARTESIAN_POINT('',(31.5734647940844,2.48499327898026,48.35));
#85796=CARTESIAN_POINT('',(31.5734647940844,2.48499327898026,48.5));
#85797=CARTESIAN_POINT('Ctrl Pts',(31.5734647940844,2.48499327898026,48.35));
#85798=CARTESIAN_POINT('Ctrl Pts',(31.5734647940844,2.09781730175018,48.35));
#85799=CARTESIAN_POINT('Ctrl Pts',(31.4939289521426,1.85995900630951,48.35));
#85800=CARTESIAN_POINT('Ctrl Pts',(31.5239422749728,3.00497958064079,48.5));
#85801=CARTESIAN_POINT('Ctrl Pts',(31.5239422749728,3.00497958064079,48.35));
#85802=CARTESIAN_POINT('Ctrl Pts',(31.5734647940844,2.81214186549187,48.5));
#85803=CARTESIAN_POINT('Ctrl Pts',(31.5734647940844,2.81214186549187,48.35));
#85804=CARTESIAN_POINT('Ctrl Pts',(31.5734647940844,2.48499327898026,48.5));
#85805=CARTESIAN_POINT('Ctrl Pts',(31.5734647940844,2.48499327898026,48.35));
#85806=CARTESIAN_POINT('',(31.5239422749728,3.00497958064079,48.5));
#85807=CARTESIAN_POINT('Ctrl Pts',(31.5239422749728,3.00497958064079,48.5));
#85808=CARTESIAN_POINT('Ctrl Pts',(31.5734647940844,2.81214186549187,48.5));
#85809=CARTESIAN_POINT('Ctrl Pts',(31.5734647940844,2.48499327898026,48.5));
#85810=CARTESIAN_POINT('',(31.5239422749728,3.00497958064079,48.35));
#85811=CARTESIAN_POINT('',(31.5239422749728,3.00497958064079,48.5));
#85812=CARTESIAN_POINT('Ctrl Pts',(31.5239422749728,3.00497958064079,48.35));
#85813=CARTESIAN_POINT('Ctrl Pts',(31.5734647940844,2.81214186549187,48.35));
#85814=CARTESIAN_POINT('Ctrl Pts',(31.5734647940844,2.48499327898026,48.35));
#85815=CARTESIAN_POINT('Ctrl Pts',(31.3873802851886,3.33212831616402,48.5));
#85816=CARTESIAN_POINT('Ctrl Pts',(31.3873802851886,3.33212831616402,48.35));
#85817=CARTESIAN_POINT('Ctrl Pts',(31.4744197558612,3.19781729578972,48.5));
#85818=CARTESIAN_POINT('Ctrl Pts',(31.4744197558612,3.19781729578972,48.35));
#85819=CARTESIAN_POINT('Ctrl Pts',(31.5239422749728,3.00497958064079,48.5));
#85820=CARTESIAN_POINT('Ctrl Pts',(31.5239422749728,3.00497958064079,48.35));
#85821=CARTESIAN_POINT('',(31.3873802851886,3.33212831616402,48.5));
#85822=CARTESIAN_POINT('Ctrl Pts',(31.3873802851886,3.33212831616402,48.5));
#85823=CARTESIAN_POINT('Ctrl Pts',(31.4744197558612,3.19781729578972,48.5));
#85824=CARTESIAN_POINT('Ctrl Pts',(31.5239422749728,3.00497958064079,48.5));
#85825=CARTESIAN_POINT('',(31.3873802851886,3.33212831616402,48.35));
#85826=CARTESIAN_POINT('',(31.3873802851886,3.33212831616402,48.5));
#85827=CARTESIAN_POINT('Ctrl Pts',(31.3873802851886,3.33212831616402,48.35));
#85828=CARTESIAN_POINT('Ctrl Pts',(31.4744197558612,3.19781729578972,48.35));
#85829=CARTESIAN_POINT('Ctrl Pts',(31.5239422749728,3.00497958064079,48.35));
#85830=CARTESIAN_POINT('Ctrl Pts',(31.1667805146426,3.5377217233181,48.5));
#85831=CARTESIAN_POINT('Ctrl Pts',(31.1667805146426,3.5377217233181,48.35));
#85832=CARTESIAN_POINT('Ctrl Pts',(31.3003408145159,3.46643933653831,48.5));
#85833=CARTESIAN_POINT('Ctrl Pts',(31.3003408145159,3.46643933653831,48.35));
#85834=CARTESIAN_POINT('Ctrl Pts',(31.3873802851886,3.33212831616402,48.5));
#85835=CARTESIAN_POINT('Ctrl Pts',(31.3873802851886,3.33212831616402,48.35));
#85836=CARTESIAN_POINT('',(31.1667805146426,3.5377217233181,48.5));
#85837=CARTESIAN_POINT('Ctrl Pts',(31.1667805146426,3.5377217233181,48.5));
#85838=CARTESIAN_POINT('Ctrl Pts',(31.3003408145159,3.46643933653831,48.5));
#85839=CARTESIAN_POINT('Ctrl Pts',(31.3873802851886,3.33212831616402,48.5));
#85840=CARTESIAN_POINT('',(31.1667805146426,3.5377217233181,48.35));
#85841=CARTESIAN_POINT('',(31.1667805146426,3.5377217233181,48.5));
#85842=CARTESIAN_POINT('Ctrl Pts',(31.1667805146426,3.5377217233181,48.35));
#85843=CARTESIAN_POINT('Ctrl Pts',(31.3003408145159,3.46643933653831,48.35));
#85844=CARTESIAN_POINT('Ctrl Pts',(31.3873802851886,3.33212831616402,48.35));
#85845=CARTESIAN_POINT('Ctrl Pts',(30.8561389874667,3.60900411009789,48.5));
#85846=CARTESIAN_POINT('Ctrl Pts',(30.8561389874667,3.60900411009789,48.35));
#85847=CARTESIAN_POINT('Ctrl Pts',(31.0332196187228,3.60900411009789,48.5));
#85848=CARTESIAN_POINT('Ctrl Pts',(31.0332196187228,3.60900411009789,48.35));
#85849=CARTESIAN_POINT('Ctrl Pts',(31.1667805146426,3.5377217233181,48.5));
#85850=CARTESIAN_POINT('Ctrl Pts',(31.1667805146426,3.5377217233181,48.35));
#85851=CARTESIAN_POINT('',(30.8561389874667,3.60900411009789,48.5));
#85852=CARTESIAN_POINT('Ctrl Pts',(30.8561389874667,3.60900411009789,48.5));
#85853=CARTESIAN_POINT('Ctrl Pts',(31.0332196187228,3.60900411009789,48.5));
#85854=CARTESIAN_POINT('Ctrl Pts',(31.1667805146426,3.5377217233181,48.5));
#85855=CARTESIAN_POINT('',(30.8561389874667,3.60900411009789,48.35));
#85856=CARTESIAN_POINT('',(30.8561389874667,3.60900411009789,48.5));
#85857=CARTESIAN_POINT('Ctrl Pts',(30.8561389874667,3.60900411009789,48.35));
#85858=CARTESIAN_POINT('Ctrl Pts',(31.0332196187228,3.60900411009789,48.35));
#85859=CARTESIAN_POINT('Ctrl Pts',(31.1667805146426,3.5377217233181,48.35));
#85860=CARTESIAN_POINT('Ctrl Pts',(30.4577081631869,3.47994545102119,48.5));
#85861=CARTESIAN_POINT('Ctrl Pts',(30.4577081631869,3.47994545102119,48.35));
#85862=CARTESIAN_POINT('Ctrl Pts',(30.6160300206393,3.60900411009789,48.5));
#85863=CARTESIAN_POINT('Ctrl Pts',(30.6160300206393,3.60900411009789,48.35));
#85864=CARTESIAN_POINT('Ctrl Pts',(30.8561389874667,3.60900411009789,48.5));
#85865=CARTESIAN_POINT('Ctrl Pts',(30.8561389874667,3.60900411009789,48.35));
#85866=CARTESIAN_POINT('',(30.4577081631869,3.47994545102119,48.5));
#85867=CARTESIAN_POINT('Ctrl Pts',(30.4577081631869,3.47994545102119,48.5));
#85868=CARTESIAN_POINT('Ctrl Pts',(30.6160300206393,3.60900411009789,48.5));
#85869=CARTESIAN_POINT('Ctrl Pts',(30.8561389874667,3.60900411009789,48.5));
#85870=CARTESIAN_POINT('',(30.4577081631869,3.47994545102119,48.35));
#85871=CARTESIAN_POINT('',(30.4577081631869,3.47994545102119,48.5));
#85872=CARTESIAN_POINT('Ctrl Pts',(30.4577081631869,3.47994545102119,48.35));
#85873=CARTESIAN_POINT('Ctrl Pts',(30.6160300206393,3.60900411009789,48.35));
#85874=CARTESIAN_POINT('Ctrl Pts',(30.8561389874667,3.60900411009789,48.35));
#85875=CARTESIAN_POINT('Ctrl Pts',(30.2190994452685,3.11302864551544,48.5));
#85876=CARTESIAN_POINT('Ctrl Pts',(30.2190994452685,3.11302864551544,48.35));
#85877=CARTESIAN_POINT('Ctrl Pts',(30.2993860077113,3.3508867919445,48.5));
#85878=CARTESIAN_POINT('Ctrl Pts',(30.2993860077113,3.3508867919445,48.35));
#85879=CARTESIAN_POINT('Ctrl Pts',(30.4577081631869,3.47994545102119,48.5));
#85880=CARTESIAN_POINT('Ctrl Pts',(30.4577081631869,3.47994545102119,48.35));
#85881=CARTESIAN_POINT('',(30.2190994452685,3.11302864551544,48.5));
#85882=CARTESIAN_POINT('Ctrl Pts',(30.2190994452685,3.11302864551544,48.5));
#85883=CARTESIAN_POINT('Ctrl Pts',(30.2993860077113,3.3508867919445,48.5));
#85884=CARTESIAN_POINT('Ctrl Pts',(30.4577081631869,3.47994545102119,48.5));
#85885=CARTESIAN_POINT('',(30.2190994452685,3.11302864551544,48.35));
#85886=CARTESIAN_POINT('',(30.2190994452685,3.11302864551544,48.5));
#85887=CARTESIAN_POINT('Ctrl Pts',(30.2190994452685,3.11302864551544,48.35));
#85888=CARTESIAN_POINT('Ctrl Pts',(30.2993860077113,3.3508867919445,48.35));
#85889=CARTESIAN_POINT('Ctrl Pts',(30.4577081631869,3.47994545102119,48.35));
#85890=CARTESIAN_POINT('Ctrl Pts',(30.138813180849,2.48499327898026,48.5));
#85891=CARTESIAN_POINT('Ctrl Pts',(30.138813180849,2.48499327898026,48.35));
#85892=CARTESIAN_POINT('Ctrl Pts',(30.138813180849,2.87517049908638,48.5));
#85893=CARTESIAN_POINT('Ctrl Pts',(30.138813180849,2.87517049908638,48.35));
#85894=CARTESIAN_POINT('Ctrl Pts',(30.2190994452685,3.11302864551544,48.5));
#85895=CARTESIAN_POINT('Ctrl Pts',(30.2190994452685,3.11302864551544,48.35));
#85896=CARTESIAN_POINT('',(30.138813180849,2.48499327898026,48.5));
#85897=CARTESIAN_POINT('Ctrl Pts',(30.138813180849,2.48499327898026,48.5));
#85898=CARTESIAN_POINT('Ctrl Pts',(30.138813180849,2.87517049908638,48.5));
#85899=CARTESIAN_POINT('Ctrl Pts',(30.2190994452685,3.11302864551544,48.5));
#85900=CARTESIAN_POINT('',(30.138813180849,2.48499327898026,48.35));
#85901=CARTESIAN_POINT('',(30.138813180849,2.48499327898026,48.5));
#85902=CARTESIAN_POINT('Ctrl Pts',(30.138813180849,2.48499327898026,48.35));
#85903=CARTESIAN_POINT('Ctrl Pts',(30.138813180849,2.87517049908638,48.35));
#85904=CARTESIAN_POINT('Ctrl Pts',(30.2190994452685,3.11302864551544,48.35));
#85905=CARTESIAN_POINT('Ctrl Pts',(30.3564118575305,1.59058684110642,48.5));
#85906=CARTESIAN_POINT('Ctrl Pts',(30.3564118575305,1.59058684110642,48.35));
#85907=CARTESIAN_POINT('Ctrl Pts',(30.138813180849,1.86521166563034,48.5));
#85908=CARTESIAN_POINT('Ctrl Pts',(30.138813180849,1.86521166563034,48.35));
#85909=CARTESIAN_POINT('Ctrl Pts',(30.138813180849,2.48499327898026,48.5));
#85910=CARTESIAN_POINT('Ctrl Pts',(30.138813180849,2.48499327898026,48.35));
#85911=CARTESIAN_POINT('Ctrl Pts',(30.3564118575305,1.59058684110642,48.5));
#85912=CARTESIAN_POINT('Ctrl Pts',(30.138813180849,1.86521166563034,48.5));
#85913=CARTESIAN_POINT('Ctrl Pts',(30.138813180849,2.48499327898026,48.5));
#85914=CARTESIAN_POINT('Ctrl Pts',(30.3564118575305,1.59058684110642,48.35));
#85915=CARTESIAN_POINT('Ctrl Pts',(30.138813180849,1.86521166563034,48.35));
#85916=CARTESIAN_POINT('Ctrl Pts',(30.138813180849,2.48499327898026,48.35));
#85917=CARTESIAN_POINT('Origin',(29.9999997746199,2.48574362695217,48.35));
#85918=CARTESIAN_POINT('Ctrl Pts',(29.1498636435717,3.38690319657326,48.5));
#85919=CARTESIAN_POINT('Ctrl Pts',(29.1498636435717,3.38690319657326,48.35));
#85920=CARTESIAN_POINT('Ctrl Pts',(28.9952933024615,3.38690319657326,48.5));
#85921=CARTESIAN_POINT('Ctrl Pts',(28.9952933024615,3.38690319657326,48.35));
#85922=CARTESIAN_POINT('Ctrl Pts',(28.8932468723506,3.28785815834999,48.5));
#85923=CARTESIAN_POINT('Ctrl Pts',(28.8932468723506,3.28785815834999,48.35));
#85924=CARTESIAN_POINT('',(29.1498636435717,3.38690319657326,48.5));
#85925=CARTESIAN_POINT('',(28.8932468723506,3.28785815834999,48.5));
#85926=CARTESIAN_POINT('Ctrl Pts',(29.1498636435717,3.38690319657326,48.5));
#85927=CARTESIAN_POINT('Ctrl Pts',(28.9952933024615,3.38690319657326,48.5));
#85928=CARTESIAN_POINT('Ctrl Pts',(28.8932468723506,3.28785815834999,48.5));
#85929=CARTESIAN_POINT('',(29.1498636435717,3.38690319657326,48.35));
#85930=CARTESIAN_POINT('',(29.1498636435717,3.38690319657326,48.5));
#85931=CARTESIAN_POINT('',(28.8932468723506,3.28785815834999,48.35));
#85932=CARTESIAN_POINT('Ctrl Pts',(29.1498636435717,3.38690319657326,48.35));
#85933=CARTESIAN_POINT('Ctrl Pts',(28.9952933024615,3.38690319657326,48.35));
#85934=CARTESIAN_POINT('Ctrl Pts',(28.8932468723506,3.28785815834999,48.35));
#85935=CARTESIAN_POINT('',(28.8932468723506,3.28785815834999,48.5));
#85936=CARTESIAN_POINT('Ctrl Pts',(29.4057299923152,3.28560718894005,48.5));
#85937=CARTESIAN_POINT('Ctrl Pts',(29.4057299923152,3.28560718894005,48.35));
#85938=CARTESIAN_POINT('Ctrl Pts',(29.3029331397265,3.38690319657326,48.5));
#85939=CARTESIAN_POINT('Ctrl Pts',(29.3029331397265,3.38690319657326,48.35));
#85940=CARTESIAN_POINT('Ctrl Pts',(29.1498636435717,3.38690319657326,48.5));
#85941=CARTESIAN_POINT('Ctrl Pts',(29.1498636435717,3.38690319657326,48.35));
#85942=CARTESIAN_POINT('',(29.4057299923152,3.28560718894005,48.5));
#85943=CARTESIAN_POINT('Ctrl Pts',(29.4057299923152,3.28560718894005,48.5));
#85944=CARTESIAN_POINT('Ctrl Pts',(29.3029331397265,3.38690319657326,48.5));
#85945=CARTESIAN_POINT('Ctrl Pts',(29.1498636435717,3.38690319657326,48.5));
#85946=CARTESIAN_POINT('',(29.4057299923152,3.28560718894005,48.35));
#85947=CARTESIAN_POINT('',(29.4057299923152,3.28560718894005,48.5));
#85948=CARTESIAN_POINT('Ctrl Pts',(29.4057299923152,3.28560718894005,48.35));
#85949=CARTESIAN_POINT('Ctrl Pts',(29.3029331397265,3.38690319657326,48.35));
#85950=CARTESIAN_POINT('Ctrl Pts',(29.1498636435717,3.38690319657326,48.35));
#85951=CARTESIAN_POINT('Ctrl Pts',(29.5085265468806,3.03574362397194,48.5));
#85952=CARTESIAN_POINT('Ctrl Pts',(29.5085265468806,3.03574362397194,48.35));
#85953=CARTESIAN_POINT('Ctrl Pts',(29.5085265468806,3.18431103229523,48.5));
#85954=CARTESIAN_POINT('Ctrl Pts',(29.5085265468806,3.18431103229523,48.35));
#85955=CARTESIAN_POINT('Ctrl Pts',(29.4057299923152,3.28560718894005,48.5));
#85956=CARTESIAN_POINT('Ctrl Pts',(29.4057299923152,3.28560718894005,48.35));
#85957=CARTESIAN_POINT('',(29.5085265468806,3.03574362397194,48.5));
#85958=CARTESIAN_POINT('Ctrl Pts',(29.5085265468806,3.03574362397194,48.5));
#85959=CARTESIAN_POINT('Ctrl Pts',(29.5085265468806,3.18431103229523,48.5));
#85960=CARTESIAN_POINT('Ctrl Pts',(29.4057299923152,3.28560718894005,48.5));
#85961=CARTESIAN_POINT('',(29.5085265468806,3.03574362397194,48.35));
#85962=CARTESIAN_POINT('',(29.5085265468806,3.03574362397194,48.5));
#85963=CARTESIAN_POINT('Ctrl Pts',(29.5085265468806,3.03574362397194,48.35));
#85964=CARTESIAN_POINT('Ctrl Pts',(29.5085265468806,3.18431103229523,48.35));
#85965=CARTESIAN_POINT('Ctrl Pts',(29.4057299923152,3.28560718894005,48.35));
#85966=CARTESIAN_POINT('Ctrl Pts',(29.4087313842028,2.79488408565521,48.5));
#85967=CARTESIAN_POINT('Ctrl Pts',(29.4087313842028,2.79488408565521,48.35));
#85968=CARTESIAN_POINT('Ctrl Pts',(29.5085265468806,2.89317870140076,48.5));
#85969=CARTESIAN_POINT('Ctrl Pts',(29.5085265468806,2.89317870140076,48.35));
#85970=CARTESIAN_POINT('Ctrl Pts',(29.5085265468806,3.03574362397194,48.5));
#85971=CARTESIAN_POINT('Ctrl Pts',(29.5085265468806,3.03574362397194,48.35));
#85972=CARTESIAN_POINT('',(29.4087313842028,2.79488408565521,48.5));
#85973=CARTESIAN_POINT('Ctrl Pts',(29.4087313842028,2.79488408565521,48.5));
#85974=CARTESIAN_POINT('Ctrl Pts',(29.5085265468806,2.89317870140076,48.5));
#85975=CARTESIAN_POINT('Ctrl Pts',(29.5085265468806,3.03574362397194,48.5));
#85976=CARTESIAN_POINT('',(29.4087313842028,2.79488408565521,48.35));
#85977=CARTESIAN_POINT('',(29.4087313842028,2.79488408565521,48.5));
#85978=CARTESIAN_POINT('Ctrl Pts',(29.4087313842028,2.79488408565521,48.35));
#85979=CARTESIAN_POINT('Ctrl Pts',(29.5085265468806,2.89317870140076,48.35));
#85980=CARTESIAN_POINT('Ctrl Pts',(29.5085265468806,3.03574362397194,48.35));
#85981=CARTESIAN_POINT('Ctrl Pts',(29.1528650354594,2.69658946990967,48.5));
#85982=CARTESIAN_POINT('Ctrl Pts',(29.1528650354594,2.69658946990967,48.35));
#85983=CARTESIAN_POINT('Ctrl Pts',(29.3089359235018,2.69658946990967,48.5));
#85984=CARTESIAN_POINT('Ctrl Pts',(29.3089359235018,2.69658946990967,48.35));
#85985=CARTESIAN_POINT('Ctrl Pts',(29.4087313842028,2.79488408565521,48.5));
#85986=CARTESIAN_POINT('Ctrl Pts',(29.4087313842028,2.79488408565521,48.35));
#85987=CARTESIAN_POINT('',(29.1528650354594,2.69658946990967,48.5));
#85988=CARTESIAN_POINT('Ctrl Pts',(29.1528650354594,2.69658946990967,48.5));
#85989=CARTESIAN_POINT('Ctrl Pts',(29.3089359235018,2.69658946990967,48.5));
#85990=CARTESIAN_POINT('Ctrl Pts',(29.4087313842028,2.79488408565521,48.5));
#85991=CARTESIAN_POINT('',(29.1528650354594,2.69658946990967,48.35));
#85992=CARTESIAN_POINT('',(29.1528650354594,2.69658946990967,48.5));
#85993=CARTESIAN_POINT('Ctrl Pts',(29.1528650354594,2.69658946990967,48.35));
#85994=CARTESIAN_POINT('Ctrl Pts',(29.3089359235018,2.69658946990967,48.35));
#85995=CARTESIAN_POINT('Ctrl Pts',(29.4087313842028,2.79488408565521,48.35));
#85996=CARTESIAN_POINT('Ctrl Pts',(28.8917463254184,2.79563435912132,48.5));
#85997=CARTESIAN_POINT('Ctrl Pts',(28.8917463254184,2.79563435912132,48.35));
#85998=CARTESIAN_POINT('Ctrl Pts',(28.9922919105738,2.69658946990967,48.5));
#85999=CARTESIAN_POINT('Ctrl Pts',(28.9922919105738,2.69658946990967,48.35));
#86000=CARTESIAN_POINT('Ctrl Pts',(29.1528650354594,2.69658946990967,48.5));
#86001=CARTESIAN_POINT('Ctrl Pts',(29.1528650354594,2.69658946990967,48.35));
#86002=CARTESIAN_POINT('',(28.8917463254184,2.79563435912132,48.5));
#86003=CARTESIAN_POINT('Ctrl Pts',(28.8917463254184,2.79563435912132,48.5));
#86004=CARTESIAN_POINT('Ctrl Pts',(28.9922919105738,2.69658946990967,48.5));
#86005=CARTESIAN_POINT('Ctrl Pts',(29.1528650354594,2.69658946990967,48.5));
#86006=CARTESIAN_POINT('',(28.8917463254184,2.79563435912132,48.35));
#86007=CARTESIAN_POINT('',(28.8917463254184,2.79563435912132,48.5));
#86008=CARTESIAN_POINT('Ctrl Pts',(28.8917463254184,2.79563435912132,48.35));
#86009=CARTESIAN_POINT('Ctrl Pts',(28.9922919105738,2.69658946990967,48.35));
#86010=CARTESIAN_POINT('Ctrl Pts',(29.1528650354594,2.69658946990967,48.35));
#86011=CARTESIAN_POINT('Ctrl Pts',(28.7912005912513,3.05075043439865,48.5));
#86012=CARTESIAN_POINT('Ctrl Pts',(28.7912005912513,3.05075043439865,48.35));
#86013=CARTESIAN_POINT('Ctrl Pts',(28.7912005912513,2.89467939734459,48.5));
#86014=CARTESIAN_POINT('Ctrl Pts',(28.7912005912513,2.89467939734459,48.35));
#86015=CARTESIAN_POINT('Ctrl Pts',(28.8917463254184,2.79563435912132,48.5));
#86016=CARTESIAN_POINT('Ctrl Pts',(28.8917463254184,2.79563435912132,48.35));
#86017=CARTESIAN_POINT('',(28.7912005912513,3.05075043439865,48.5));
#86018=CARTESIAN_POINT('Ctrl Pts',(28.7912005912513,3.05075043439865,48.5));
#86019=CARTESIAN_POINT('Ctrl Pts',(28.7912005912513,2.89467939734459,48.5));
#86020=CARTESIAN_POINT('Ctrl Pts',(28.8917463254184,2.79563435912132,48.5));
#86021=CARTESIAN_POINT('',(28.7912005912513,3.05075043439865,48.35));
#86022=CARTESIAN_POINT('',(28.7912005912513,3.05075043439865,48.5));
#86023=CARTESIAN_POINT('Ctrl Pts',(28.7912005912513,3.05075043439865,48.35));
#86024=CARTESIAN_POINT('Ctrl Pts',(28.7912005912513,2.89467939734459,48.35));
#86025=CARTESIAN_POINT('Ctrl Pts',(28.8917463254184,2.79563435912132,48.35));
#86026=CARTESIAN_POINT('Ctrl Pts',(28.8932468723506,3.28785815834999,48.5));
#86027=CARTESIAN_POINT('Ctrl Pts',(28.8932468723506,3.28785815834999,48.35));
#86028=CARTESIAN_POINT('Ctrl Pts',(28.7912005912513,3.18881312012672,48.5));
#86029=CARTESIAN_POINT('Ctrl Pts',(28.7912005912513,3.18881312012672,48.35));
#86030=CARTESIAN_POINT('Ctrl Pts',(28.7912005912513,3.05075043439865,48.5));
#86031=CARTESIAN_POINT('Ctrl Pts',(28.7912005912513,3.05075043439865,48.35));
#86032=CARTESIAN_POINT('Ctrl Pts',(28.8932468723506,3.28785815834999,48.5));
#86033=CARTESIAN_POINT('Ctrl Pts',(28.7912005912513,3.18881312012672,48.5));
#86034=CARTESIAN_POINT('Ctrl Pts',(28.7912005912513,3.05075043439865,48.5));
#86035=CARTESIAN_POINT('Ctrl Pts',(28.8932468723506,3.28785815834999,48.35));
#86036=CARTESIAN_POINT('Ctrl Pts',(28.7912005912513,3.18881312012672,48.35));
#86037=CARTESIAN_POINT('Ctrl Pts',(28.7912005912513,3.05075043439865,48.35));
#86038=CARTESIAN_POINT('Ctrl Pts',(29.1453615557402,2.47598910331726,48.5));
#86039=CARTESIAN_POINT('Ctrl Pts',(29.1453615557402,2.47598910331726,48.35));
#86040=CARTESIAN_POINT('Ctrl Pts',(28.9547749590129,2.47598910331726,48.5));
#86041=CARTESIAN_POINT('Ctrl Pts',(28.9547749590129,2.47598910331726,48.35));
#86042=CARTESIAN_POINT('Ctrl Pts',(28.82946796529,2.34993183612823,48.5));
#86043=CARTESIAN_POINT('Ctrl Pts',(28.82946796529,2.34993183612823,48.35));
#86044=CARTESIAN_POINT('',(29.1453615557402,2.47598910331726,48.5));
#86045=CARTESIAN_POINT('',(28.82946796529,2.34993183612823,48.5));
#86046=CARTESIAN_POINT('Ctrl Pts',(29.1453615557402,2.47598910331726,48.5));
#86047=CARTESIAN_POINT('Ctrl Pts',(28.9547749590129,2.47598910331726,48.5));
#86048=CARTESIAN_POINT('Ctrl Pts',(28.82946796529,2.34993183612823,48.5));
#86049=CARTESIAN_POINT('',(29.1453615557402,2.47598910331726,48.35));
#86050=CARTESIAN_POINT('',(29.1453615557402,2.47598910331726,48.5));
#86051=CARTESIAN_POINT('',(28.82946796529,2.34993183612823,48.35));
#86052=CARTESIAN_POINT('Ctrl Pts',(29.1453615557402,2.47598910331726,48.35));
#86053=CARTESIAN_POINT('Ctrl Pts',(28.9547749590129,2.47598910331726,48.35));
#86054=CARTESIAN_POINT('Ctrl Pts',(28.82946796529,2.34993183612823,48.35));
#86055=CARTESIAN_POINT('',(28.82946796529,2.34993183612823,48.5));
#86056=CARTESIAN_POINT('Ctrl Pts',(29.4702591728419,2.34843128919601,48.5));
#86057=CARTESIAN_POINT('Ctrl Pts',(29.4702591728419,2.34843128919601,48.35));
#86058=CARTESIAN_POINT('Ctrl Pts',(29.3404502402991,2.47598910331726,48.5));
#86059=CARTESIAN_POINT('Ctrl Pts',(29.3404502402991,2.47598910331726,48.35));
#86060=CARTESIAN_POINT('Ctrl Pts',(29.1453615557402,2.47598910331726,48.5));
#86061=CARTESIAN_POINT('Ctrl Pts',(29.1453615557402,2.47598910331726,48.35));
#86062=CARTESIAN_POINT('',(29.4702591728419,2.34843128919601,48.5));
#86063=CARTESIAN_POINT('Ctrl Pts',(29.4702591728419,2.34843128919601,48.5));
#86064=CARTESIAN_POINT('Ctrl Pts',(29.3404502402991,2.47598910331726,48.5));
#86065=CARTESIAN_POINT('Ctrl Pts',(29.1453615557402,2.47598910331726,48.5));
#86066=CARTESIAN_POINT('',(29.4702591728419,2.34843128919601,48.35));
#86067=CARTESIAN_POINT('',(29.4702591728419,2.34843128919601,48.5));
#86068=CARTESIAN_POINT('Ctrl Pts',(29.4702591728419,2.34843128919601,48.35));
#86069=CARTESIAN_POINT('Ctrl Pts',(29.3404502402991,2.47598910331726,48.35));
#86070=CARTESIAN_POINT('Ctrl Pts',(29.1453615557402,2.47598910331726,48.35));
#86071=CARTESIAN_POINT('Ctrl Pts',(29.6000682543963,2.02578449249268,48.5));
#86072=CARTESIAN_POINT('Ctrl Pts',(29.6000682543963,2.02578449249268,48.35));
#86073=CARTESIAN_POINT('Ctrl Pts',(29.6000682543963,2.22087317705154,48.5));
#86074=CARTESIAN_POINT('Ctrl Pts',(29.6000682543963,2.22087317705154,48.35));
#86075=CARTESIAN_POINT('Ctrl Pts',(29.4702591728419,2.34843128919601,48.5));
#86076=CARTESIAN_POINT('Ctrl Pts',(29.4702591728419,2.34843128919601,48.35));
#86077=CARTESIAN_POINT('',(29.6000682543963,2.02578449249268,48.5));
#86078=CARTESIAN_POINT('Ctrl Pts',(29.6000682543963,2.02578449249268,48.5));
#86079=CARTESIAN_POINT('Ctrl Pts',(29.6000682543963,2.22087317705154,48.5));
#86080=CARTESIAN_POINT('Ctrl Pts',(29.4702591728419,2.34843128919601,48.5));
#86081=CARTESIAN_POINT('',(29.6000682543963,2.02578449249268,48.35));
#86082=CARTESIAN_POINT('',(29.6000682543963,2.02578449249268,48.5));
#86083=CARTESIAN_POINT('Ctrl Pts',(29.6000682543963,2.02578449249268,48.35));
#86084=CARTESIAN_POINT('Ctrl Pts',(29.6000682543963,2.22087317705154,48.35));
#86085=CARTESIAN_POINT('Ctrl Pts',(29.4702591728419,2.34843128919601,48.35));
#86086=CARTESIAN_POINT('Ctrl Pts',(29.4740109872073,1.70914047956467,48.5));
#86087=CARTESIAN_POINT('Ctrl Pts',(29.4740109872073,1.70914047956467,48.35));
#86088=CARTESIAN_POINT('Ctrl Pts',(29.6000682543963,1.83369719982147,48.5));
#86089=CARTESIAN_POINT('Ctrl Pts',(29.6000682543963,1.83369719982147,48.35));
#86090=CARTESIAN_POINT('Ctrl Pts',(29.6000682543963,2.02578449249268,48.5));
#86091=CARTESIAN_POINT('Ctrl Pts',(29.6000682543963,2.02578449249268,48.35));
#86092=CARTESIAN_POINT('',(29.4740109872073,1.70914047956467,48.5));
#86093=CARTESIAN_POINT('Ctrl Pts',(29.4740109872073,1.70914047956467,48.5));
#86094=CARTESIAN_POINT('Ctrl Pts',(29.6000682543963,1.83369719982147,48.5));
#86095=CARTESIAN_POINT('Ctrl Pts',(29.6000682543963,2.02578449249268,48.5));
#86096=CARTESIAN_POINT('',(29.4740109872073,1.70914047956467,48.35));
#86097=CARTESIAN_POINT('',(29.4740109872073,1.70914047956467,48.5));
#86098=CARTESIAN_POINT('Ctrl Pts',(29.4740109872073,1.70914047956467,48.35));
#86099=CARTESIAN_POINT('Ctrl Pts',(29.6000682543963,1.83369719982147,48.35));
#86100=CARTESIAN_POINT('Ctrl Pts',(29.6000682543963,2.02578449249268,48.35));
#86101=CARTESIAN_POINT('Ctrl Pts',(29.1543655823916,1.58458405733109,48.5));
#86102=CARTESIAN_POINT('Ctrl Pts',(29.1543655823916,1.58458405733109,48.35));
#86103=CARTESIAN_POINT('Ctrl Pts',(29.3479537200183,1.58458405733109,48.5));
#86104=CARTESIAN_POINT('Ctrl Pts',(29.3479537200183,1.58458405733109,48.35));
#86105=CARTESIAN_POINT('Ctrl Pts',(29.4740109872073,1.70914047956467,48.5));
#86106=CARTESIAN_POINT('Ctrl Pts',(29.4740109872073,1.70914047956467,48.35));
#86107=CARTESIAN_POINT('',(29.1543655823916,1.58458405733109,48.5));
#86108=CARTESIAN_POINT('Ctrl Pts',(29.1543655823916,1.58458405733109,48.5));
#86109=CARTESIAN_POINT('Ctrl Pts',(29.3479537200183,1.58458405733109,48.5));
#86110=CARTESIAN_POINT('Ctrl Pts',(29.4740109872073,1.70914047956467,48.5));
#86111=CARTESIAN_POINT('',(29.1543655823916,1.58458405733109,48.35));
#86112=CARTESIAN_POINT('',(29.1543655823916,1.58458405733109,48.5));
#86113=CARTESIAN_POINT('Ctrl Pts',(29.1543655823916,1.58458405733109,48.35));
#86114=CARTESIAN_POINT('Ctrl Pts',(29.3479537200183,1.58458405733109,48.35));
#86115=CARTESIAN_POINT('Ctrl Pts',(29.4740109872073,1.70914047956467,48.35));
#86116=CARTESIAN_POINT('Ctrl Pts',(28.9217599462718,1.64386087656021,48.5));
#86117=CARTESIAN_POINT('Ctrl Pts',(28.9217599462718,1.64386087656021,48.35));
#86118=CARTESIAN_POINT('Ctrl Pts',(29.0298090111464,1.58458405733109,48.5));
#86119=CARTESIAN_POINT('Ctrl Pts',(29.0298090111464,1.58458405733109,48.35));
#86120=CARTESIAN_POINT('Ctrl Pts',(29.1543655823916,1.58458405733109,48.5));
#86121=CARTESIAN_POINT('Ctrl Pts',(29.1543655823916,1.58458405733109,48.35));
#86122=CARTESIAN_POINT('',(28.9217599462718,1.64386087656021,48.5));
#86123=CARTESIAN_POINT('Ctrl Pts',(28.9217599462718,1.64386087656021,48.5));
#86124=CARTESIAN_POINT('Ctrl Pts',(29.0298090111464,1.58458405733109,48.5));
#86125=CARTESIAN_POINT('Ctrl Pts',(29.1543655823916,1.58458405733109,48.5));
#86126=CARTESIAN_POINT('',(28.9217599462718,1.64386087656021,48.35));
#86127=CARTESIAN_POINT('',(28.9217599462718,1.64386087656021,48.5));
#86128=CARTESIAN_POINT('Ctrl Pts',(28.9217599462718,1.64386087656021,48.35));
#86129=CARTESIAN_POINT('Ctrl Pts',(29.0298090111464,1.58458405733109,48.35));
#86130=CARTESIAN_POINT('Ctrl Pts',(29.1543655823916,1.58458405733109,48.35));
#86131=CARTESIAN_POINT('Ctrl Pts',(28.7589358519763,1.8111869096756,48.5));
#86132=CARTESIAN_POINT('Ctrl Pts',(28.7589358519763,1.8111869096756,48.35));
#86133=CARTESIAN_POINT('Ctrl Pts',(28.8137107323855,1.70313799381256,48.5));
#86134=CARTESIAN_POINT('Ctrl Pts',(28.8137107323855,1.70313799381256,48.35));
#86135=CARTESIAN_POINT('Ctrl Pts',(28.9217599462718,1.64386087656021,48.5));
#86136=CARTESIAN_POINT('Ctrl Pts',(28.9217599462718,1.64386087656021,48.35));
#86137=CARTESIAN_POINT('',(28.7589358519763,1.8111869096756,48.5));
#86138=CARTESIAN_POINT('Ctrl Pts',(28.7589358519763,1.8111869096756,48.5));
#86139=CARTESIAN_POINT('Ctrl Pts',(28.8137107323855,1.70313799381256,48.5));
#86140=CARTESIAN_POINT('Ctrl Pts',(28.9217599462718,1.64386087656021,48.5));
#86141=CARTESIAN_POINT('',(28.7589358519763,1.8111869096756,48.35));
#86142=CARTESIAN_POINT('',(28.7589358519763,1.8111869096756,48.5));
#86143=CARTESIAN_POINT('Ctrl Pts',(28.7589358519763,1.8111869096756,48.35));
#86144=CARTESIAN_POINT('Ctrl Pts',(28.8137107323855,1.70313799381256,48.35));
#86145=CARTESIAN_POINT('Ctrl Pts',(28.9217599462718,1.64386087656021,48.35));
#86146=CARTESIAN_POINT('Ctrl Pts',(28.704160971567,2.03478866815567,48.5));
#86147=CARTESIAN_POINT('Ctrl Pts',(28.704160971567,2.03478866815567,48.35));
#86148=CARTESIAN_POINT('Ctrl Pts',(28.704160971567,1.91923612356186,48.5));
#86149=CARTESIAN_POINT('Ctrl Pts',(28.704160971567,1.91923612356186,48.35));
#86150=CARTESIAN_POINT('Ctrl Pts',(28.7589358519763,1.8111869096756,48.5));
#86151=CARTESIAN_POINT('Ctrl Pts',(28.7589358519763,1.8111869096756,48.35));
#86152=CARTESIAN_POINT('',(28.704160971567,2.03478866815567,48.5));
#86153=CARTESIAN_POINT('Ctrl Pts',(28.704160971567,2.03478866815567,48.5));
#86154=CARTESIAN_POINT('Ctrl Pts',(28.704160971567,1.91923612356186,48.5));
#86155=CARTESIAN_POINT('Ctrl Pts',(28.7589358519763,1.8111869096756,48.5));
#86156=CARTESIAN_POINT('',(28.704160971567,2.03478866815567,48.35));
#86157=CARTESIAN_POINT('',(28.704160971567,2.03478866815567,48.5));
#86158=CARTESIAN_POINT('Ctrl Pts',(28.704160971567,2.03478866815567,48.35));
#86159=CARTESIAN_POINT('Ctrl Pts',(28.704160971567,1.91923612356186,48.35));
#86160=CARTESIAN_POINT('Ctrl Pts',(28.7589358519763,1.8111869096756,48.35));
#86161=CARTESIAN_POINT('Ctrl Pts',(28.82946796529,2.34993183612823,48.5));
#86162=CARTESIAN_POINT('Ctrl Pts',(28.82946796529,2.34993183612823,48.35));
#86163=CARTESIAN_POINT('Ctrl Pts',(28.704160971567,2.22387456893921,48.5));
#86164=CARTESIAN_POINT('Ctrl Pts',(28.704160971567,2.22387456893921,48.35));
#86165=CARTESIAN_POINT('Ctrl Pts',(28.704160971567,2.03478866815567,48.5));
#86166=CARTESIAN_POINT('Ctrl Pts',(28.704160971567,2.03478866815567,48.35));
#86167=CARTESIAN_POINT('Ctrl Pts',(28.82946796529,2.34993183612823,48.5));
#86168=CARTESIAN_POINT('Ctrl Pts',(28.704160971567,2.22387456893921,48.5));
#86169=CARTESIAN_POINT('Ctrl Pts',(28.704160971567,2.03478866815567,48.5));
#86170=CARTESIAN_POINT('Ctrl Pts',(28.82946796529,2.34993183612823,48.35));
#86171=CARTESIAN_POINT('Ctrl Pts',(28.704160971567,2.22387456893921,48.35));
#86172=CARTESIAN_POINT('Ctrl Pts',(28.704160971567,2.03478866815567,48.35));
#86173=CARTESIAN_POINT('Ctrl Pts',(28.4265347551554,2.03628921508789,48.5));
#86174=CARTESIAN_POINT('Ctrl Pts',(28.4265347551554,2.03628921508789,48.35));
#86175=CARTESIAN_POINT('Ctrl Pts',(28.4265347551554,2.25088679790497,48.5));
#86176=CARTESIAN_POINT('Ctrl Pts',(28.4265347551554,2.25088679790497,48.35));
#86177=CARTESIAN_POINT('Ctrl Pts',(28.5353342425078,2.39570268988609,48.5));
#86178=CARTESIAN_POINT('Ctrl Pts',(28.5353342425078,2.39570268988609,48.35));
#86179=CARTESIAN_POINT('',(28.4265347551554,2.03628921508789,48.5));
#86180=CARTESIAN_POINT('',(28.5353342425078,2.39570268988609,48.5));
#86181=CARTESIAN_POINT('Ctrl Pts',(28.4265347551554,2.03628921508789,48.5));
#86182=CARTESIAN_POINT('Ctrl Pts',(28.4265347551554,2.25088679790497,48.5));
#86183=CARTESIAN_POINT('Ctrl Pts',(28.5353342425078,2.39570268988609,48.5));
#86184=CARTESIAN_POINT('',(28.4265347551554,2.03628921508789,48.35));
#86185=CARTESIAN_POINT('',(28.4265347551554,2.03628921508789,48.5));
#86186=CARTESIAN_POINT('',(28.5353342425078,2.39570268988609,48.35));
#86187=CARTESIAN_POINT('Ctrl Pts',(28.4265347551554,2.03628921508789,48.35));
#86188=CARTESIAN_POINT('Ctrl Pts',(28.4265347551554,2.25088679790497,48.35));
#86189=CARTESIAN_POINT('Ctrl Pts',(28.5353342425078,2.39570268988609,48.35));
#86190=CARTESIAN_POINT('',(28.5353342425078,2.39570268988609,48.5));
#86191=CARTESIAN_POINT('Ctrl Pts',(28.6261255275458,1.55532056093216,48.5));
#86192=CARTESIAN_POINT('Ctrl Pts',(28.6261255275458,1.55532056093216,48.35));
#86193=CARTESIAN_POINT('Ctrl Pts',(28.4265347551554,1.74815827608109,48.5));
#86194=CARTESIAN_POINT('Ctrl Pts',(28.4265347551554,1.74815827608109,48.35));
#86195=CARTESIAN_POINT('Ctrl Pts',(28.4265347551554,2.03628921508789,48.5));
#86196=CARTESIAN_POINT('Ctrl Pts',(28.4265347551554,2.03628921508789,48.35));
#86197=CARTESIAN_POINT('',(28.6261255275458,1.55532056093216,48.5));
#86198=CARTESIAN_POINT('Ctrl Pts',(28.6261255275458,1.55532056093216,48.5));
#86199=CARTESIAN_POINT('Ctrl Pts',(28.4265347551554,1.74815827608109,48.5));
#86200=CARTESIAN_POINT('Ctrl Pts',(28.4265347551554,2.03628921508789,48.5));
#86201=CARTESIAN_POINT('',(28.6261255275458,1.55532056093216,48.35));
#86202=CARTESIAN_POINT('',(28.6261255275458,1.55532056093216,48.5));
#86203=CARTESIAN_POINT('Ctrl Pts',(28.6261255275458,1.55532056093216,48.35));
#86204=CARTESIAN_POINT('Ctrl Pts',(28.4265347551554,1.74815827608109,48.35));
#86205=CARTESIAN_POINT('Ctrl Pts',(28.4265347551554,2.03628921508789,48.35));
#86206=CARTESIAN_POINT('Ctrl Pts',(29.151364190504,1.36248314380646,48.5));
#86207=CARTESIAN_POINT('Ctrl Pts',(29.151364190504,1.36248314380646,48.35));
#86208=CARTESIAN_POINT('Ctrl Pts',(28.8257162999362,1.36248314380646,48.5));
#86209=CARTESIAN_POINT('Ctrl Pts',(28.8257162999362,1.36248314380646,48.35));
#86210=CARTESIAN_POINT('Ctrl Pts',(28.6261255275458,1.55532056093216,48.5));
#86211=CARTESIAN_POINT('Ctrl Pts',(28.6261255275458,1.55532056093216,48.35));
#86212=CARTESIAN_POINT('',(29.151364190504,1.36248314380646,48.5));
#86213=CARTESIAN_POINT('Ctrl Pts',(29.151364190504,1.36248314380646,48.5));
#86214=CARTESIAN_POINT('Ctrl Pts',(28.8257162999362,1.36248314380646,48.5));
#86215=CARTESIAN_POINT('Ctrl Pts',(28.6261255275458,1.55532056093216,48.5));
#86216=CARTESIAN_POINT('',(29.151364190504,1.36248314380646,48.35));
#86217=CARTESIAN_POINT('',(29.151364190504,1.36248314380646,48.5));
#86218=CARTESIAN_POINT('Ctrl Pts',(29.151364190504,1.36248314380646,48.35));
#86219=CARTESIAN_POINT('Ctrl Pts',(28.8257162999362,1.36248314380646,48.35));
#86220=CARTESIAN_POINT('Ctrl Pts',(28.6261255275458,1.55532056093216,48.35));
#86221=CARTESIAN_POINT('Ctrl Pts',(29.6766030024737,1.55457043647766,48.5));
#86222=CARTESIAN_POINT('Ctrl Pts',(29.6766030024737,1.55457043647766,48.35));
#86223=CARTESIAN_POINT('Ctrl Pts',(29.477012379095,1.36248314380646,48.5));
#86224=CARTESIAN_POINT('Ctrl Pts',(29.477012379095,1.36248314380646,48.35));
#86225=CARTESIAN_POINT('Ctrl Pts',(29.151364190504,1.36248314380646,48.5));
#86226=CARTESIAN_POINT('Ctrl Pts',(29.151364190504,1.36248314380646,48.35));
#86227=CARTESIAN_POINT('',(29.6766030024737,1.55457043647766,48.5));
#86228=CARTESIAN_POINT('Ctrl Pts',(29.6766030024737,1.55457043647766,48.5));
#86229=CARTESIAN_POINT('Ctrl Pts',(29.477012379095,1.36248314380646,48.5));
#86230=CARTESIAN_POINT('Ctrl Pts',(29.151364190504,1.36248314380646,48.5));
#86231=CARTESIAN_POINT('',(29.6766030024737,1.55457043647766,48.35));
#86232=CARTESIAN_POINT('',(29.6766030024737,1.55457043647766,48.5));
#86233=CARTESIAN_POINT('Ctrl Pts',(29.6766030024737,1.55457043647766,48.35));
#86234=CARTESIAN_POINT('Ctrl Pts',(29.477012379095,1.36248314380646,48.35));
#86235=CARTESIAN_POINT('Ctrl Pts',(29.151364190504,1.36248314380646,48.35));
#86236=CARTESIAN_POINT('Ctrl Pts',(29.8761936258525,2.02878588438034,48.5));
#86237=CARTESIAN_POINT('Ctrl Pts',(29.8761936258525,2.02878588438034,48.35));
#86238=CARTESIAN_POINT('Ctrl Pts',(29.8761936258525,1.74665772914886,48.5));
#86239=CARTESIAN_POINT('Ctrl Pts',(29.8761936258525,1.74665772914886,48.35));
#86240=CARTESIAN_POINT('Ctrl Pts',(29.6766030024737,1.55457043647766,48.5));
#86241=CARTESIAN_POINT('Ctrl Pts',(29.6766030024737,1.55457043647766,48.35));
#86242=CARTESIAN_POINT('',(29.8761936258525,2.02878588438034,48.5));
#86243=CARTESIAN_POINT('Ctrl Pts',(29.8761936258525,2.02878588438034,48.5));
#86244=CARTESIAN_POINT('Ctrl Pts',(29.8761936258525,1.74665772914886,48.5));
#86245=CARTESIAN_POINT('Ctrl Pts',(29.6766030024737,1.55457043647766,48.5));
#86246=CARTESIAN_POINT('',(29.8761936258525,2.02878588438034,48.35));
#86247=CARTESIAN_POINT('',(29.8761936258525,2.02878588438034,48.5));
#86248=CARTESIAN_POINT('Ctrl Pts',(29.8761936258525,2.02878588438034,48.35));
#86249=CARTESIAN_POINT('Ctrl Pts',(29.8761936258525,1.74665772914886,48.35));
#86250=CARTESIAN_POINT('Ctrl Pts',(29.6766030024737,1.55457043647766,48.35));
#86251=CARTESIAN_POINT('Ctrl Pts',(29.7703956793994,2.37994545698166,48.5));
#86252=CARTESIAN_POINT('Ctrl Pts',(29.7703956793994,2.37994545698166,48.35));
#86253=CARTESIAN_POINT('Ctrl Pts',(29.8761936258525,2.2328787446022,48.5));
#86254=CARTESIAN_POINT('Ctrl Pts',(29.8761936258525,2.2328787446022,48.35));
#86255=CARTESIAN_POINT('Ctrl Pts',(29.8761936258525,2.02878588438034,48.5));
#86256=CARTESIAN_POINT('Ctrl Pts',(29.8761936258525,2.02878588438034,48.35));
#86257=CARTESIAN_POINT('',(29.7703956793994,2.37994545698166,48.5));
#86258=CARTESIAN_POINT('Ctrl Pts',(29.7703956793994,2.37994545698166,48.5));
#86259=CARTESIAN_POINT('Ctrl Pts',(29.8761936258525,2.2328787446022,48.5));
#86260=CARTESIAN_POINT('Ctrl Pts',(29.8761936258525,2.02878588438034,48.5));
#86261=CARTESIAN_POINT('',(29.7703956793994,2.37994545698166,48.35));
#86262=CARTESIAN_POINT('',(29.7703956793994,2.37994545698166,48.5));
#86263=CARTESIAN_POINT('Ctrl Pts',(29.7703956793994,2.37994545698166,48.35));
#86264=CARTESIAN_POINT('Ctrl Pts',(29.8761936258525,2.2328787446022,48.35));
#86265=CARTESIAN_POINT('Ctrl Pts',(29.8761936258525,2.02878588438034,48.35));
#86266=CARTESIAN_POINT('Ctrl Pts',(29.4620054196566,2.59304249286652,48.5));
#86267=CARTESIAN_POINT('Ctrl Pts',(29.4620054196566,2.59304249286652,48.35));
#86268=CARTESIAN_POINT('Ctrl Pts',(29.6645974349231,2.52701246738434,48.5));
#86269=CARTESIAN_POINT('Ctrl Pts',(29.6645974349231,2.52701246738434,48.35));
#86270=CARTESIAN_POINT('Ctrl Pts',(29.7703956793994,2.37994545698166,48.5));
#86271=CARTESIAN_POINT('Ctrl Pts',(29.7703956793994,2.37994545698166,48.35));
#86272=CARTESIAN_POINT('',(29.4620054196566,2.59304249286652,48.5));
#86273=CARTESIAN_POINT('Ctrl Pts',(29.4620054196566,2.59304249286652,48.5));
#86274=CARTESIAN_POINT('Ctrl Pts',(29.6645974349231,2.52701246738434,48.5));
#86275=CARTESIAN_POINT('Ctrl Pts',(29.7703956793994,2.37994545698166,48.5));
#86276=CARTESIAN_POINT('',(29.4620054196566,2.59304249286652,48.35));
#86277=CARTESIAN_POINT('',(29.4620054196566,2.59304249286652,48.5));
#86278=CARTESIAN_POINT('Ctrl Pts',(29.4620054196566,2.59304249286652,48.35));
#86279=CARTESIAN_POINT('Ctrl Pts',(29.6645974349231,2.52701246738434,48.35));
#86280=CARTESIAN_POINT('Ctrl Pts',(29.7703956793994,2.37994545698166,48.35));
#86281=CARTESIAN_POINT('Ctrl Pts',(29.7058662008494,2.76787185668945,48.5));
#86282=CARTESIAN_POINT('Ctrl Pts',(29.7058662008494,2.76787185668945,48.35));
#86283=CARTESIAN_POINT('Ctrl Pts',(29.6255796384066,2.65457028150558,48.5));
#86284=CARTESIAN_POINT('Ctrl Pts',(29.6255796384066,2.65457028150558,48.35));
#86285=CARTESIAN_POINT('Ctrl Pts',(29.4620054196566,2.59304249286652,48.5));
#86286=CARTESIAN_POINT('Ctrl Pts',(29.4620054196566,2.59304249286652,48.35));
#86287=CARTESIAN_POINT('',(29.7058662008494,2.76787185668945,48.5));
#86288=CARTESIAN_POINT('Ctrl Pts',(29.7058662008494,2.76787185668945,48.5));
#86289=CARTESIAN_POINT('Ctrl Pts',(29.6255796384066,2.65457028150558,48.5));
#86290=CARTESIAN_POINT('Ctrl Pts',(29.4620054196566,2.59304249286652,48.5));
#86291=CARTESIAN_POINT('',(29.7058662008494,2.76787185668945,48.35));
#86292=CARTESIAN_POINT('',(29.7058662008494,2.76787185668945,48.5));
#86293=CARTESIAN_POINT('Ctrl Pts',(29.7058662008494,2.76787185668945,48.35));
#86294=CARTESIAN_POINT('Ctrl Pts',(29.6255796384066,2.65457028150558,48.35));
#86295=CARTESIAN_POINT('Ctrl Pts',(29.4620054196566,2.59304249286652,48.35));
#86296=CARTESIAN_POINT('Ctrl Pts',(29.7861527632922,3.03424292802811,48.5));
#86297=CARTESIAN_POINT('Ctrl Pts',(29.7861527632922,3.03424292802811,48.35));
#86298=CARTESIAN_POINT('Ctrl Pts',(29.7861527632922,2.88117328286171,48.5));
#86299=CARTESIAN_POINT('Ctrl Pts',(29.7861527632922,2.88117328286171,48.35));
#86300=CARTESIAN_POINT('Ctrl Pts',(29.7058662008494,2.76787185668945,48.5));
#86301=CARTESIAN_POINT('Ctrl Pts',(29.7058662008494,2.76787185668945,48.35));
#86302=CARTESIAN_POINT('',(29.7861527632922,3.03424292802811,48.5));
#86303=CARTESIAN_POINT('Ctrl Pts',(29.7861527632922,3.03424292802811,48.5));
#86304=CARTESIAN_POINT('Ctrl Pts',(29.7861527632922,2.88117328286171,48.5));
#86305=CARTESIAN_POINT('Ctrl Pts',(29.7058662008494,2.76787185668945,48.5));
#86306=CARTESIAN_POINT('',(29.7861527632922,3.03424292802811,48.35));
#86307=CARTESIAN_POINT('',(29.7861527632922,3.03424292802811,48.5));
#86308=CARTESIAN_POINT('Ctrl Pts',(29.7861527632922,3.03424292802811,48.35));
#86309=CARTESIAN_POINT('Ctrl Pts',(29.7861527632922,2.88117328286171,48.35));
#86310=CARTESIAN_POINT('Ctrl Pts',(29.7058662008494,2.76787185668945,48.35));
#86311=CARTESIAN_POINT('Ctrl Pts',(29.6105729769915,3.4416780769825,48.5));
#86312=CARTESIAN_POINT('Ctrl Pts',(29.6105729769915,3.4416780769825,48.35));
#86313=CARTESIAN_POINT('Ctrl Pts',(29.7861527632922,3.27435204386711,48.5));
#86314=CARTESIAN_POINT('Ctrl Pts',(29.7861527632922,3.27435204386711,48.35));
#86315=CARTESIAN_POINT('Ctrl Pts',(29.7861527632922,3.03424292802811,48.5));
#86316=CARTESIAN_POINT('Ctrl Pts',(29.7861527632922,3.03424292802811,48.35));
#86317=CARTESIAN_POINT('',(29.6105729769915,3.4416780769825,48.5));
#86318=CARTESIAN_POINT('Ctrl Pts',(29.6105729769915,3.4416780769825,48.5));
#86319=CARTESIAN_POINT('Ctrl Pts',(29.7861527632922,3.27435204386711,48.5));
#86320=CARTESIAN_POINT('Ctrl Pts',(29.7861527632922,3.03424292802811,48.5));
#86321=CARTESIAN_POINT('',(29.6105729769915,3.4416780769825,48.35));
#86322=CARTESIAN_POINT('',(29.6105729769915,3.4416780769825,48.5));
#86323=CARTESIAN_POINT('Ctrl Pts',(29.6105729769915,3.4416780769825,48.35));
#86324=CARTESIAN_POINT('Ctrl Pts',(29.7861527632922,3.27435204386711,48.35));
#86325=CARTESIAN_POINT('Ctrl Pts',(29.7861527632922,3.03424292802811,48.35));
#86326=CARTESIAN_POINT('Ctrl Pts',(29.1468622516841,3.60900411009789,48.5));
#86327=CARTESIAN_POINT('Ctrl Pts',(29.1468622516841,3.60900411009789,48.35));
#86328=CARTESIAN_POINT('Ctrl Pts',(29.4349931906909,3.60900411009789,48.5));
#86329=CARTESIAN_POINT('Ctrl Pts',(29.4349931906909,3.60900411009789,48.35));
#86330=CARTESIAN_POINT('Ctrl Pts',(29.6105729769915,3.4416780769825,48.5));
#86331=CARTESIAN_POINT('Ctrl Pts',(29.6105729769915,3.4416780769825,48.35));
#86332=CARTESIAN_POINT('',(29.1468622516841,3.60900411009789,48.5));
#86333=CARTESIAN_POINT('Ctrl Pts',(29.1468622516841,3.60900411009789,48.5));
#86334=CARTESIAN_POINT('Ctrl Pts',(29.4349931906909,3.60900411009789,48.5));
#86335=CARTESIAN_POINT('Ctrl Pts',(29.6105729769915,3.4416780769825,48.5));
#86336=CARTESIAN_POINT('',(29.1468622516841,3.60900411009789,48.35));
#86337=CARTESIAN_POINT('',(29.1468622516841,3.60900411009789,48.5));
#86338=CARTESIAN_POINT('Ctrl Pts',(29.1468622516841,3.60900411009789,48.35));
#86339=CARTESIAN_POINT('Ctrl Pts',(29.4349931906909,3.60900411009789,48.35));
#86340=CARTESIAN_POINT('Ctrl Pts',(29.6105729769915,3.4416780769825,48.35));
#86341=CARTESIAN_POINT('Ctrl Pts',(28.6876534651965,3.44542974233627,48.5));
#86342=CARTESIAN_POINT('Ctrl Pts',(28.6876534651965,3.44542974233627,48.35));
#86343=CARTESIAN_POINT('Ctrl Pts',(28.8602318596095,3.60900411009789,48.5));
#86344=CARTESIAN_POINT('Ctrl Pts',(28.8602318596095,3.60900411009789,48.35));
#86345=CARTESIAN_POINT('Ctrl Pts',(29.1468622516841,3.60900411009789,48.5));
#86346=CARTESIAN_POINT('Ctrl Pts',(29.1468622516841,3.60900411009789,48.35));
#86347=CARTESIAN_POINT('',(28.6876534651965,3.44542974233627,48.5));
#86348=CARTESIAN_POINT('Ctrl Pts',(28.6876534651965,3.44542974233627,48.5));
#86349=CARTESIAN_POINT('Ctrl Pts',(28.8602318596095,3.60900411009789,48.5));
#86350=CARTESIAN_POINT('Ctrl Pts',(29.1468622516841,3.60900411009789,48.5));
#86351=CARTESIAN_POINT('',(28.6876534651965,3.44542974233627,48.35));
#86352=CARTESIAN_POINT('',(28.6876534651965,3.44542974233627,48.5));
#86353=CARTESIAN_POINT('Ctrl Pts',(28.6876534651965,3.44542974233627,48.35));
#86354=CARTESIAN_POINT('Ctrl Pts',(28.8602318596095,3.60900411009789,48.35));
#86355=CARTESIAN_POINT('Ctrl Pts',(29.1468622516841,3.60900411009789,48.35));
#86356=CARTESIAN_POINT('Ctrl Pts',(28.5150750707835,3.04174625873566,48.5));
#86357=CARTESIAN_POINT('Ctrl Pts',(28.5150750707835,3.04174625873566,48.35));
#86358=CARTESIAN_POINT('Ctrl Pts',(28.5150750707835,3.28185537457466,48.5));
#86359=CARTESIAN_POINT('Ctrl Pts',(28.5150750707835,3.28185537457466,48.35));
#86360=CARTESIAN_POINT('Ctrl Pts',(28.6876534651965,3.44542974233627,48.5));
#86361=CARTESIAN_POINT('Ctrl Pts',(28.6876534651965,3.44542974233627,48.35));
#86362=CARTESIAN_POINT('',(28.5150750707835,3.04174625873566,48.5));
#86363=CARTESIAN_POINT('Ctrl Pts',(28.5150750707835,3.04174625873566,48.5));
#86364=CARTESIAN_POINT('Ctrl Pts',(28.5150750707835,3.28185537457466,48.5));
#86365=CARTESIAN_POINT('Ctrl Pts',(28.6876534651965,3.44542974233627,48.5));
#86366=CARTESIAN_POINT('',(28.5150750707835,3.04174625873566,48.35));
#86367=CARTESIAN_POINT('',(28.5150750707835,3.04174625873566,48.5));
#86368=CARTESIAN_POINT('Ctrl Pts',(28.5150750707835,3.04174625873566,48.35));
#86369=CARTESIAN_POINT('Ctrl Pts',(28.5150750707835,3.28185537457466,48.35));
#86370=CARTESIAN_POINT('Ctrl Pts',(28.6876534651965,3.44542974233627,48.35));
#86371=CARTESIAN_POINT('Ctrl Pts',(28.5961119066924,2.76862213015556,48.5));
#86372=CARTESIAN_POINT('Ctrl Pts',(28.5961119066924,2.76862213015556,48.35));
#86373=CARTESIAN_POINT('Ctrl Pts',(28.5150750707835,2.88267397880554,48.5));
#86374=CARTESIAN_POINT('Ctrl Pts',(28.5150750707835,2.88267397880554,48.35));
#86375=CARTESIAN_POINT('Ctrl Pts',(28.5150750707835,3.04174625873566,48.5));
#86376=CARTESIAN_POINT('Ctrl Pts',(28.5150750707835,3.04174625873566,48.35));
#86377=CARTESIAN_POINT('',(28.5961119066924,2.76862213015556,48.5));
#86378=CARTESIAN_POINT('Ctrl Pts',(28.5961119066924,2.76862213015556,48.5));
#86379=CARTESIAN_POINT('Ctrl Pts',(28.5150750707835,2.88267397880554,48.5));
#86380=CARTESIAN_POINT('Ctrl Pts',(28.5150750707835,3.04174625873566,48.5));
#86381=CARTESIAN_POINT('',(28.5961119066924,2.76862213015556,48.35));
#86382=CARTESIAN_POINT('',(28.5961119066924,2.76862213015556,48.5));
#86383=CARTESIAN_POINT('Ctrl Pts',(28.5961119066924,2.76862213015556,48.35));
#86384=CARTESIAN_POINT('Ctrl Pts',(28.5150750707835,2.88267397880554,48.35));
#86385=CARTESIAN_POINT('Ctrl Pts',(28.5150750707835,3.04174625873566,48.35));
#86386=CARTESIAN_POINT('Ctrl Pts',(28.8452250491828,2.59304249286652,48.5));
#86387=CARTESIAN_POINT('Ctrl Pts',(28.8452250491828,2.59304249286652,48.35));
#86388=CARTESIAN_POINT('Ctrl Pts',(28.6771487426013,2.65457028150558,48.5));
#86389=CARTESIAN_POINT('Ctrl Pts',(28.6771487426013,2.65457028150558,48.35));
#86390=CARTESIAN_POINT('Ctrl Pts',(28.5961119066924,2.76862213015556,48.5));
#86391=CARTESIAN_POINT('Ctrl Pts',(28.5961119066924,2.76862213015556,48.35));
#86392=CARTESIAN_POINT('',(28.8452250491828,2.59304249286652,48.5));
#86393=CARTESIAN_POINT('Ctrl Pts',(28.8452250491828,2.59304249286652,48.5));
#86394=CARTESIAN_POINT('Ctrl Pts',(28.6771487426013,2.65457028150558,48.5));
#86395=CARTESIAN_POINT('Ctrl Pts',(28.5961119066924,2.76862213015556,48.5));
#86396=CARTESIAN_POINT('',(28.8452250491828,2.59304249286652,48.35));
#86397=CARTESIAN_POINT('',(28.8452250491828,2.59304249286652,48.5));
#86398=CARTESIAN_POINT('Ctrl Pts',(28.8452250491828,2.59304249286652,48.35));
#86399=CARTESIAN_POINT('Ctrl Pts',(28.6771487426013,2.65457028150558,48.35));
#86400=CARTESIAN_POINT('Ctrl Pts',(28.5961119066924,2.76862213015556,48.35));
#86401=CARTESIAN_POINT('Ctrl Pts',(28.5353342425078,2.39570268988609,48.5));
#86402=CARTESIAN_POINT('Ctrl Pts',(28.5353342425078,2.39570268988609,48.35));
#86403=CARTESIAN_POINT('Ctrl Pts',(28.6441337298602,2.54051858186722,48.5));
#86404=CARTESIAN_POINT('Ctrl Pts',(28.6441337298602,2.54051858186722,48.35));
#86405=CARTESIAN_POINT('Ctrl Pts',(28.8452250491828,2.59304249286652,48.5));
#86406=CARTESIAN_POINT('Ctrl Pts',(28.8452250491828,2.59304249286652,48.35));
#86407=CARTESIAN_POINT('Ctrl Pts',(28.5353342425078,2.39570268988609,48.5));
#86408=CARTESIAN_POINT('Ctrl Pts',(28.6441337298602,2.54051858186722,48.5));
#86409=CARTESIAN_POINT('Ctrl Pts',(28.8452250491828,2.59304249286652,48.5));
#86410=CARTESIAN_POINT('Ctrl Pts',(28.5353342425078,2.39570268988609,48.35));
#86411=CARTESIAN_POINT('Ctrl Pts',(28.6441337298602,2.54051858186722,48.35));
#86412=CARTESIAN_POINT('Ctrl Pts',(28.8452250491828,2.59304249286652,48.35));
#86413=CARTESIAN_POINT('Origin',(29.9999997746199,2.48574362695217,48.35));
#86414=CARTESIAN_POINT('Origin',(0.,8.,48.5));
#86415=CARTESIAN_POINT('Origin',(0.,8.,48.5));
#86416=CARTESIAN_POINT('Origin',(0.,8.,48.5));
#86417=CARTESIAN_POINT('Ctrl Pts',(20.8516373746097,3.38540250062943,48.5));
#86418=CARTESIAN_POINT('Ctrl Pts',(20.8516373746097,3.38540250062943,48.35));
#86419=CARTESIAN_POINT('Ctrl Pts',(20.6655525676906,3.38540250062943,48.5));
#86420=CARTESIAN_POINT('Ctrl Pts',(20.6655525676906,3.38540250062943,48.35));
#86421=CARTESIAN_POINT('Ctrl Pts',(20.5545022599399,3.22783091664314,48.5));
#86422=CARTESIAN_POINT('Ctrl Pts',(20.5545022599399,3.22783091664314,48.35));
#86423=CARTESIAN_POINT('',(20.8516373746097,3.38540250062943,48.5));
#86424=CARTESIAN_POINT('',(20.5545022599399,3.22783091664314,48.5));
#86425=CARTESIAN_POINT('Ctrl Pts',(20.8516373746097,3.38540250062943,48.5));
#86426=CARTESIAN_POINT('Ctrl Pts',(20.6655525676906,3.38540250062943,48.5));
#86427=CARTESIAN_POINT('Ctrl Pts',(20.5545022599399,3.22783091664314,48.5));
#86428=CARTESIAN_POINT('',(20.8516373746097,3.38540250062943,48.35));
#86429=CARTESIAN_POINT('',(20.8516373746097,3.38540250062943,48.5));
#86430=CARTESIAN_POINT('',(20.5545022599399,3.22783091664314,48.35));
#86431=CARTESIAN_POINT('Ctrl Pts',(20.8516373746097,3.38540250062943,48.35));
#86432=CARTESIAN_POINT('Ctrl Pts',(20.6655525676906,3.38540250062943,48.35));
#86433=CARTESIAN_POINT('Ctrl Pts',(20.5545022599399,3.22783091664314,48.35));
#86434=CARTESIAN_POINT('',(20.5545022599399,3.22783091664314,48.5));
#86435=CARTESIAN_POINT('Ctrl Pts',(21.1675306670368,3.2068213224411,48.5));
#86436=CARTESIAN_POINT('Ctrl Pts',(21.1675306670368,3.2068213224411,48.35));
#86437=CARTESIAN_POINT('Ctrl Pts',(21.04072297737,3.38540250062943,48.5));
#86438=CARTESIAN_POINT('Ctrl Pts',(21.04072297737,3.38540250062943,48.35));
#86439=CARTESIAN_POINT('Ctrl Pts',(20.8516373746097,3.38540250062943,48.5));
#86440=CARTESIAN_POINT('Ctrl Pts',(20.8516373746097,3.38540250062943,48.35));
#86441=CARTESIAN_POINT('',(21.1675306670368,3.2068213224411,48.5));
#86442=CARTESIAN_POINT('Ctrl Pts',(21.1675306670368,3.2068213224411,48.5));
#86443=CARTESIAN_POINT('Ctrl Pts',(21.04072297737,3.38540250062943,48.5));
#86444=CARTESIAN_POINT('Ctrl Pts',(20.8516373746097,3.38540250062943,48.5));
#86445=CARTESIAN_POINT('',(21.1675306670368,3.2068213224411,48.35));
#86446=CARTESIAN_POINT('',(21.1675306670368,3.2068213224411,48.5));
#86447=CARTESIAN_POINT('Ctrl Pts',(21.1675306670368,3.2068213224411,48.35));
#86448=CARTESIAN_POINT('Ctrl Pts',(21.04072297737,3.38540250062943,48.35));
#86449=CARTESIAN_POINT('Ctrl Pts',(20.8516373746097,3.38540250062943,48.35));
#86450=CARTESIAN_POINT('Ctrl Pts',(21.2943383567035,2.48499327898026,48.5));
#86451=CARTESIAN_POINT('Ctrl Pts',(21.2943383567035,2.48499327898026,48.35));
#86452=CARTESIAN_POINT('Ctrl Pts',(21.2943383567035,3.02824014425278,48.5));
#86453=CARTESIAN_POINT('Ctrl Pts',(21.2943383567035,3.02824014425278,48.35));
#86454=CARTESIAN_POINT('Ctrl Pts',(21.1675306670368,3.2068213224411,48.5));
#86455=CARTESIAN_POINT('Ctrl Pts',(21.1675306670368,3.2068213224411,48.35));
#86456=CARTESIAN_POINT('',(21.2943383567035,2.48499327898026,48.5));
#86457=CARTESIAN_POINT('Ctrl Pts',(21.2943383567035,2.48499327898026,48.5));
#86458=CARTESIAN_POINT('Ctrl Pts',(21.2943383567035,3.02824014425278,48.5));
#86459=CARTESIAN_POINT('Ctrl Pts',(21.1675306670368,3.2068213224411,48.5));
#86460=CARTESIAN_POINT('',(21.2943383567035,2.48499327898026,48.35));
#86461=CARTESIAN_POINT('',(21.2943383567035,2.48499327898026,48.5));
#86462=CARTESIAN_POINT('Ctrl Pts',(21.2943383567035,2.48499327898026,48.35));
#86463=CARTESIAN_POINT('Ctrl Pts',(21.2943383567035,3.02824014425278,48.35));
#86464=CARTESIAN_POINT('Ctrl Pts',(21.1675306670368,3.2068213224411,48.35));
#86465=CARTESIAN_POINT('Ctrl Pts',(21.1675306670368,1.76466578245163,48.5));
#86466=CARTESIAN_POINT('Ctrl Pts',(21.1675306670368,1.76466578245163,48.35));
#86467=CARTESIAN_POINT('Ctrl Pts',(21.2943383567035,1.9447478055954,48.5));
#86468=CARTESIAN_POINT('Ctrl Pts',(21.2943383567035,1.9447478055954,48.35));
#86469=CARTESIAN_POINT('Ctrl Pts',(21.2943383567035,2.48499327898026,48.5));
#86470=CARTESIAN_POINT('Ctrl Pts',(21.2943383567035,2.48499327898026,48.35));
#86471=CARTESIAN_POINT('',(21.1675306670368,1.76466578245163,48.5));
#86472=CARTESIAN_POINT('Ctrl Pts',(21.1675306670368,1.76466578245163,48.5));
#86473=CARTESIAN_POINT('Ctrl Pts',(21.2943383567035,1.9447478055954,48.5));
#86474=CARTESIAN_POINT('Ctrl Pts',(21.2943383567035,2.48499327898026,48.5));
#86475=CARTESIAN_POINT('',(21.1675306670368,1.76466578245163,48.35));
#86476=CARTESIAN_POINT('',(21.1675306670368,1.76466578245163,48.5));
#86477=CARTESIAN_POINT('Ctrl Pts',(21.1675306670368,1.76466578245163,48.35));
#86478=CARTESIAN_POINT('Ctrl Pts',(21.2943383567035,1.9447478055954,48.35));
#86479=CARTESIAN_POINT('Ctrl Pts',(21.2943383567035,2.48499327898026,48.35));
#86480=CARTESIAN_POINT('Ctrl Pts',(20.8546384684741,1.58458405733109,48.5));
#86481=CARTESIAN_POINT('Ctrl Pts',(20.8546384684741,1.58458405733109,48.35));
#86482=CARTESIAN_POINT('Ctrl Pts',(21.04072297737,1.58458405733109,48.5));
#86483=CARTESIAN_POINT('Ctrl Pts',(21.04072297737,1.58458405733109,48.35));
#86484=CARTESIAN_POINT('Ctrl Pts',(21.1675306670368,1.76466578245163,48.5));
#86485=CARTESIAN_POINT('Ctrl Pts',(21.1675306670368,1.76466578245163,48.35));
#86486=CARTESIAN_POINT('',(20.8546384684741,1.58458405733109,48.5));
#86487=CARTESIAN_POINT('Ctrl Pts',(20.8546384684741,1.58458405733109,48.5));
#86488=CARTESIAN_POINT('Ctrl Pts',(21.04072297737,1.58458405733109,48.5));
#86489=CARTESIAN_POINT('Ctrl Pts',(21.1675306670368,1.76466578245163,48.5));
#86490=CARTESIAN_POINT('',(20.8546384684741,1.58458405733109,48.35));
#86491=CARTESIAN_POINT('',(20.8546384684741,1.58458405733109,48.5));
#86492=CARTESIAN_POINT('Ctrl Pts',(20.8546384684741,1.58458405733109,48.35));
#86493=CARTESIAN_POINT('Ctrl Pts',(21.04072297737,1.58458405733109,48.35));
#86494=CARTESIAN_POINT('Ctrl Pts',(21.1675306670368,1.76466578245163,48.35));
#86495=CARTESIAN_POINT('Ctrl Pts',(20.5417462699115,1.76391565799713,48.5));
#86496=CARTESIAN_POINT('Ctrl Pts',(20.5417462699115,1.76391565799713,48.35));
#86497=CARTESIAN_POINT('Ctrl Pts',(20.6685539595783,1.58458405733109,48.5));
#86498=CARTESIAN_POINT('Ctrl Pts',(20.6685539595783,1.58458405733109,48.35));
#86499=CARTESIAN_POINT('Ctrl Pts',(20.8546384684741,1.58458405733109,48.5));
#86500=CARTESIAN_POINT('Ctrl Pts',(20.8546384684741,1.58458405733109,48.35));
#86501=CARTESIAN_POINT('',(20.5417462699115,1.76391565799713,48.5));
#86502=CARTESIAN_POINT('Ctrl Pts',(20.5417462699115,1.76391565799713,48.5));
#86503=CARTESIAN_POINT('Ctrl Pts',(20.6685539595783,1.58458405733109,48.5));
#86504=CARTESIAN_POINT('Ctrl Pts',(20.8546384684741,1.58458405733109,48.5));
#86505=CARTESIAN_POINT('',(20.5417462699115,1.76391565799713,48.35));
#86506=CARTESIAN_POINT('',(20.5417462699115,1.76391565799713,48.5));
#86507=CARTESIAN_POINT('Ctrl Pts',(20.5417462699115,1.76391565799713,48.35));
#86508=CARTESIAN_POINT('Ctrl Pts',(20.6685539595783,1.58458405733109,48.35));
#86509=CARTESIAN_POINT('Ctrl Pts',(20.8546384684741,1.58458405733109,48.35));
#86510=CARTESIAN_POINT('Ctrl Pts',(20.4149385802448,2.48499327898026,48.5));
#86511=CARTESIAN_POINT('Ctrl Pts',(20.4149385802448,2.48499327898026,48.35));
#86512=CARTESIAN_POINT('Ctrl Pts',(20.4149385802448,1.94324696063995,48.5));
#86513=CARTESIAN_POINT('Ctrl Pts',(20.4149385802448,1.94324696063995,48.35));
#86514=CARTESIAN_POINT('Ctrl Pts',(20.5417462699115,1.76391565799713,48.5));
#86515=CARTESIAN_POINT('Ctrl Pts',(20.5417462699115,1.76391565799713,48.35));
#86516=CARTESIAN_POINT('',(20.4149385802448,2.48499327898026,48.5));
#86517=CARTESIAN_POINT('Ctrl Pts',(20.4149385802448,2.48499327898026,48.5));
#86518=CARTESIAN_POINT('Ctrl Pts',(20.4149385802448,1.94324696063995,48.5));
#86519=CARTESIAN_POINT('Ctrl Pts',(20.5417462699115,1.76391565799713,48.5));
#86520=CARTESIAN_POINT('',(20.4149385802448,2.48499327898026,48.35));
#86521=CARTESIAN_POINT('',(20.4149385802448,2.48499327898026,48.5));
#86522=CARTESIAN_POINT('Ctrl Pts',(20.4149385802448,2.48499327898026,48.35));
#86523=CARTESIAN_POINT('Ctrl Pts',(20.4149385802448,1.94324696063995,48.35));
#86524=CARTESIAN_POINT('Ctrl Pts',(20.5417462699115,1.76391565799713,48.35));
#86525=CARTESIAN_POINT('Ctrl Pts',(20.5545022599399,3.22783091664314,48.5));
#86526=CARTESIAN_POINT('Ctrl Pts',(20.5545022599399,3.22783091664314,48.35));
#86527=CARTESIAN_POINT('Ctrl Pts',(20.4149385802448,3.02673944830894,48.5));
#86528=CARTESIAN_POINT('Ctrl Pts',(20.4149385802448,3.02673944830894,48.35));
#86529=CARTESIAN_POINT('Ctrl Pts',(20.4149385802448,2.48499327898026,48.5));
#86530=CARTESIAN_POINT('Ctrl Pts',(20.4149385802448,2.48499327898026,48.35));
#86531=CARTESIAN_POINT('Ctrl Pts',(20.5545022599399,3.22783091664314,48.5));
#86532=CARTESIAN_POINT('Ctrl Pts',(20.4149385802448,3.02673944830894,48.5));
#86533=CARTESIAN_POINT('Ctrl Pts',(20.4149385802448,2.48499327898026,48.5));
#86534=CARTESIAN_POINT('Ctrl Pts',(20.5545022599399,3.22783091664314,48.35));
#86535=CARTESIAN_POINT('Ctrl Pts',(20.4149385802448,3.02673944830894,48.35));
#86536=CARTESIAN_POINT('Ctrl Pts',(20.4149385802448,2.48499327898026,48.35));
#86537=CARTESIAN_POINT('Ctrl Pts',(20.8546384684741,1.36248314380646,48.5));
#86538=CARTESIAN_POINT('Ctrl Pts',(20.8546384684741,1.36248314380646,48.35));
#86539=CARTESIAN_POINT('Ctrl Pts',(20.5364939086139,1.36248314380646,48.5));
#86540=CARTESIAN_POINT('Ctrl Pts',(20.5364939086139,1.36248314380646,48.35));
#86541=CARTESIAN_POINT('Ctrl Pts',(20.3549113385379,1.59058684110642,48.5));
#86542=CARTESIAN_POINT('Ctrl Pts',(20.3549113385379,1.59058684110642,48.35));
#86543=CARTESIAN_POINT('',(20.8546384684741,1.36248314380646,48.5));
#86544=CARTESIAN_POINT('',(20.3549113385379,1.59058684110642,48.5));
#86545=CARTESIAN_POINT('Ctrl Pts',(20.8546384684741,1.36248314380646,48.5));
#86546=CARTESIAN_POINT('Ctrl Pts',(20.5364939086139,1.36248314380646,48.5));
#86547=CARTESIAN_POINT('Ctrl Pts',(20.3549113385379,1.59058684110642,48.5));
#86548=CARTESIAN_POINT('',(20.8546384684741,1.36248314380646,48.35));
#86549=CARTESIAN_POINT('',(20.8546384684741,1.36248314380646,48.5));
#86550=CARTESIAN_POINT('',(20.3549113385379,1.59058684110642,48.35));
#86551=CARTESIAN_POINT('Ctrl Pts',(20.8546384684741,1.36248314380646,48.35));
#86552=CARTESIAN_POINT('Ctrl Pts',(20.5364939086139,1.36248314380646,48.35));
#86553=CARTESIAN_POINT('Ctrl Pts',(20.3549113385379,1.59058684110642,48.35));
#86554=CARTESIAN_POINT('',(20.3549113385379,1.59058684110642,48.5));
#86555=CARTESIAN_POINT('Ctrl Pts',(21.2545701377094,1.49229192733765,48.5));
#86556=CARTESIAN_POINT('Ctrl Pts',(21.2545701377094,1.49229192733765,48.35));
#86557=CARTESIAN_POINT('Ctrl Pts',(21.096248280257,1.36248314380646,48.5));
#86558=CARTESIAN_POINT('Ctrl Pts',(21.096248280257,1.36248314380646,48.35));
#86559=CARTESIAN_POINT('Ctrl Pts',(20.8546384684741,1.36248314380646,48.5));
#86560=CARTESIAN_POINT('Ctrl Pts',(20.8546384684741,1.36248314380646,48.35));
#86561=CARTESIAN_POINT('',(21.2545701377094,1.49229192733765,48.5));
#86562=CARTESIAN_POINT('Ctrl Pts',(21.2545701377094,1.49229192733765,48.5));
#86563=CARTESIAN_POINT('Ctrl Pts',(21.096248280257,1.36248314380646,48.5));
#86564=CARTESIAN_POINT('Ctrl Pts',(20.8546384684741,1.36248314380646,48.5));
#86565=CARTESIAN_POINT('',(21.2545701377094,1.49229192733765,48.35));
#86566=CARTESIAN_POINT('',(21.2545701377094,1.49229192733765,48.5));
#86567=CARTESIAN_POINT('Ctrl Pts',(21.2545701377094,1.49229192733765,48.35));
#86568=CARTESIAN_POINT('Ctrl Pts',(21.096248280257,1.36248314380646,48.35));
#86569=CARTESIAN_POINT('Ctrl Pts',(20.8546384684741,1.36248314380646,48.35));
#86570=CARTESIAN_POINT('Ctrl Pts',(21.4924284331501,1.85995900630951,48.5));
#86571=CARTESIAN_POINT('Ctrl Pts',(21.4924284331501,1.85995900630951,48.35));
#86572=CARTESIAN_POINT('Ctrl Pts',(21.4128919951618,1.62210100889206,48.5));
#86573=CARTESIAN_POINT('Ctrl Pts',(21.4128919951618,1.62210100889206,48.35));
#86574=CARTESIAN_POINT('Ctrl Pts',(21.2545701377094,1.49229192733765,48.5));
#86575=CARTESIAN_POINT('Ctrl Pts',(21.2545701377094,1.49229192733765,48.35));
#86576=CARTESIAN_POINT('',(21.4924284331501,1.85995900630951,48.5));
#86577=CARTESIAN_POINT('Ctrl Pts',(21.4924284331501,1.85995900630951,48.5));
#86578=CARTESIAN_POINT('Ctrl Pts',(21.4128919951618,1.62210100889206,48.5));
#86579=CARTESIAN_POINT('Ctrl Pts',(21.2545701377094,1.49229192733765,48.5));
#86580=CARTESIAN_POINT('',(21.4924284331501,1.85995900630951,48.35));
#86581=CARTESIAN_POINT('',(21.4924284331501,1.85995900630951,48.5));
#86582=CARTESIAN_POINT('Ctrl Pts',(21.4924284331501,1.85995900630951,48.35));
#86583=CARTESIAN_POINT('Ctrl Pts',(21.4128919951618,1.62210100889206,48.35));
#86584=CARTESIAN_POINT('Ctrl Pts',(21.2545701377094,1.49229192733765,48.35));
#86585=CARTESIAN_POINT('Ctrl Pts',(21.5719642750919,2.48499327898026,48.5));
#86586=CARTESIAN_POINT('Ctrl Pts',(21.5719642750919,2.48499327898026,48.35));
#86587=CARTESIAN_POINT('Ctrl Pts',(21.5719642750919,2.09781730175018,48.5));
#86588=CARTESIAN_POINT('Ctrl Pts',(21.5719642750919,2.09781730175018,48.35));
#86589=CARTESIAN_POINT('Ctrl Pts',(21.4924284331501,1.85995900630951,48.5));
#86590=CARTESIAN_POINT('Ctrl Pts',(21.4924284331501,1.85995900630951,48.35));
#86591=CARTESIAN_POINT('',(21.5719642750919,2.48499327898026,48.5));
#86592=CARTESIAN_POINT('Ctrl Pts',(21.5719642750919,2.48499327898026,48.5));
#86593=CARTESIAN_POINT('Ctrl Pts',(21.5719642750919,2.09781730175018,48.5));
#86594=CARTESIAN_POINT('Ctrl Pts',(21.4924284331501,1.85995900630951,48.5));
#86595=CARTESIAN_POINT('',(21.5719642750919,2.48499327898026,48.35));
#86596=CARTESIAN_POINT('',(21.5719642750919,2.48499327898026,48.5));
#86597=CARTESIAN_POINT('Ctrl Pts',(21.5719642750919,2.48499327898026,48.35));
#86598=CARTESIAN_POINT('Ctrl Pts',(21.5719642750919,2.09781730175018,48.35));
#86599=CARTESIAN_POINT('Ctrl Pts',(21.4924284331501,1.85995900630951,48.35));
#86600=CARTESIAN_POINT('Ctrl Pts',(21.5224417559803,3.00497958064079,48.5));
#86601=CARTESIAN_POINT('Ctrl Pts',(21.5224417559803,3.00497958064079,48.35));
#86602=CARTESIAN_POINT('Ctrl Pts',(21.5719642750919,2.81214186549187,48.5));
#86603=CARTESIAN_POINT('Ctrl Pts',(21.5719642750919,2.81214186549187,48.35));
#86604=CARTESIAN_POINT('Ctrl Pts',(21.5719642750919,2.48499327898026,48.5));
#86605=CARTESIAN_POINT('Ctrl Pts',(21.5719642750919,2.48499327898026,48.35));
#86606=CARTESIAN_POINT('',(21.5224417559803,3.00497958064079,48.5));
#86607=CARTESIAN_POINT('Ctrl Pts',(21.5224417559803,3.00497958064079,48.5));
#86608=CARTESIAN_POINT('Ctrl Pts',(21.5719642750919,2.81214186549187,48.5));
#86609=CARTESIAN_POINT('Ctrl Pts',(21.5719642750919,2.48499327898026,48.5));
#86610=CARTESIAN_POINT('',(21.5224417559803,3.00497958064079,48.35));
#86611=CARTESIAN_POINT('',(21.5224417559803,3.00497958064079,48.5));
#86612=CARTESIAN_POINT('Ctrl Pts',(21.5224417559803,3.00497958064079,48.35));
#86613=CARTESIAN_POINT('Ctrl Pts',(21.5719642750919,2.81214186549187,48.35));
#86614=CARTESIAN_POINT('Ctrl Pts',(21.5719642750919,2.48499327898026,48.35));
#86615=CARTESIAN_POINT('Ctrl Pts',(21.385879766196,3.33212831616402,48.5));
#86616=CARTESIAN_POINT('Ctrl Pts',(21.385879766196,3.33212831616402,48.35));
#86617=CARTESIAN_POINT('Ctrl Pts',(21.4729192368686,3.19781729578972,48.5));
#86618=CARTESIAN_POINT('Ctrl Pts',(21.4729192368686,3.19781729578972,48.35));
#86619=CARTESIAN_POINT('Ctrl Pts',(21.5224417559803,3.00497958064079,48.5));
#86620=CARTESIAN_POINT('Ctrl Pts',(21.5224417559803,3.00497958064079,48.35));
#86621=CARTESIAN_POINT('',(21.385879766196,3.33212831616402,48.5));
#86622=CARTESIAN_POINT('Ctrl Pts',(21.385879766196,3.33212831616402,48.5));
#86623=CARTESIAN_POINT('Ctrl Pts',(21.4729192368686,3.19781729578972,48.5));
#86624=CARTESIAN_POINT('Ctrl Pts',(21.5224417559803,3.00497958064079,48.5));
#86625=CARTESIAN_POINT('',(21.385879766196,3.33212831616402,48.35));
#86626=CARTESIAN_POINT('',(21.385879766196,3.33212831616402,48.5));
#86627=CARTESIAN_POINT('Ctrl Pts',(21.385879766196,3.33212831616402,48.35));
#86628=CARTESIAN_POINT('Ctrl Pts',(21.4729192368686,3.19781729578972,48.35));
#86629=CARTESIAN_POINT('Ctrl Pts',(21.5224417559803,3.00497958064079,48.35));
#86630=CARTESIAN_POINT('Ctrl Pts',(21.1652799956501,3.5377217233181,48.5));
#86631=CARTESIAN_POINT('Ctrl Pts',(21.1652799956501,3.5377217233181,48.35));
#86632=CARTESIAN_POINT('Ctrl Pts',(21.2988402955234,3.46643933653831,48.5));
#86633=CARTESIAN_POINT('Ctrl Pts',(21.2988402955234,3.46643933653831,48.35));
#86634=CARTESIAN_POINT('Ctrl Pts',(21.385879766196,3.33212831616402,48.5));
#86635=CARTESIAN_POINT('Ctrl Pts',(21.385879766196,3.33212831616402,48.35));
#86636=CARTESIAN_POINT('',(21.1652799956501,3.5377217233181,48.5));
#86637=CARTESIAN_POINT('Ctrl Pts',(21.1652799956501,3.5377217233181,48.5));
#86638=CARTESIAN_POINT('Ctrl Pts',(21.2988402955234,3.46643933653831,48.5));
#86639=CARTESIAN_POINT('Ctrl Pts',(21.385879766196,3.33212831616402,48.5));
#86640=CARTESIAN_POINT('',(21.1652799956501,3.5377217233181,48.35));
#86641=CARTESIAN_POINT('',(21.1652799956501,3.5377217233181,48.5));
#86642=CARTESIAN_POINT('Ctrl Pts',(21.1652799956501,3.5377217233181,48.35));
#86643=CARTESIAN_POINT('Ctrl Pts',(21.2988402955234,3.46643933653831,48.35));
#86644=CARTESIAN_POINT('Ctrl Pts',(21.385879766196,3.33212831616402,48.35));
#86645=CARTESIAN_POINT('Ctrl Pts',(20.8546384684741,3.60900411009789,48.5));
#86646=CARTESIAN_POINT('Ctrl Pts',(20.8546384684741,3.60900411009789,48.35));
#86647=CARTESIAN_POINT('Ctrl Pts',(21.0317190997303,3.60900411009789,48.5));
#86648=CARTESIAN_POINT('Ctrl Pts',(21.0317190997303,3.60900411009789,48.35));
#86649=CARTESIAN_POINT('Ctrl Pts',(21.1652799956501,3.5377217233181,48.5));
#86650=CARTESIAN_POINT('Ctrl Pts',(21.1652799956501,3.5377217233181,48.35));
#86651=CARTESIAN_POINT('',(20.8546384684741,3.60900411009789,48.5));
#86652=CARTESIAN_POINT('Ctrl Pts',(20.8546384684741,3.60900411009789,48.5));
#86653=CARTESIAN_POINT('Ctrl Pts',(21.0317190997303,3.60900411009789,48.5));
#86654=CARTESIAN_POINT('Ctrl Pts',(21.1652799956501,3.5377217233181,48.5));
#86655=CARTESIAN_POINT('',(20.8546384684741,3.60900411009789,48.35));
#86656=CARTESIAN_POINT('',(20.8546384684741,3.60900411009789,48.5));
#86657=CARTESIAN_POINT('Ctrl Pts',(20.8546384684741,3.60900411009789,48.35));
#86658=CARTESIAN_POINT('Ctrl Pts',(21.0317190997303,3.60900411009789,48.35));
#86659=CARTESIAN_POINT('Ctrl Pts',(21.1652799956501,3.5377217233181,48.35));
#86660=CARTESIAN_POINT('Ctrl Pts',(20.4562076441944,3.47994545102119,48.5));
#86661=CARTESIAN_POINT('Ctrl Pts',(20.4562076441944,3.47994545102119,48.35));
#86662=CARTESIAN_POINT('Ctrl Pts',(20.6145295016468,3.60900411009789,48.5));
#86663=CARTESIAN_POINT('Ctrl Pts',(20.6145295016468,3.60900411009789,48.35));
#86664=CARTESIAN_POINT('Ctrl Pts',(20.8546384684741,3.60900411009789,48.5));
#86665=CARTESIAN_POINT('Ctrl Pts',(20.8546384684741,3.60900411009789,48.35));
#86666=CARTESIAN_POINT('',(20.4562076441944,3.47994545102119,48.5));
#86667=CARTESIAN_POINT('Ctrl Pts',(20.4562076441944,3.47994545102119,48.5));
#86668=CARTESIAN_POINT('Ctrl Pts',(20.6145295016468,3.60900411009789,48.5));
#86669=CARTESIAN_POINT('Ctrl Pts',(20.8546384684741,3.60900411009789,48.5));
#86670=CARTESIAN_POINT('',(20.4562076441944,3.47994545102119,48.35));
#86671=CARTESIAN_POINT('',(20.4562076441944,3.47994545102119,48.5));
#86672=CARTESIAN_POINT('Ctrl Pts',(20.4562076441944,3.47994545102119,48.35));
#86673=CARTESIAN_POINT('Ctrl Pts',(20.6145295016468,3.60900411009789,48.35));
#86674=CARTESIAN_POINT('Ctrl Pts',(20.8546384684741,3.60900411009789,48.35));
#86675=CARTESIAN_POINT('Ctrl Pts',(20.217598926276,3.11302864551544,48.5));
#86676=CARTESIAN_POINT('Ctrl Pts',(20.217598926276,3.11302864551544,48.35));
#86677=CARTESIAN_POINT('Ctrl Pts',(20.2978854887187,3.3508867919445,48.5));
#86678=CARTESIAN_POINT('Ctrl Pts',(20.2978854887187,3.3508867919445,48.35));
#86679=CARTESIAN_POINT('Ctrl Pts',(20.4562076441944,3.47994545102119,48.5));
#86680=CARTESIAN_POINT('Ctrl Pts',(20.4562076441944,3.47994545102119,48.35));
#86681=CARTESIAN_POINT('',(20.217598926276,3.11302864551544,48.5));
#86682=CARTESIAN_POINT('Ctrl Pts',(20.217598926276,3.11302864551544,48.5));
#86683=CARTESIAN_POINT('Ctrl Pts',(20.2978854887187,3.3508867919445,48.5));
#86684=CARTESIAN_POINT('Ctrl Pts',(20.4562076441944,3.47994545102119,48.5));
#86685=CARTESIAN_POINT('',(20.217598926276,3.11302864551544,48.35));
#86686=CARTESIAN_POINT('',(20.217598926276,3.11302864551544,48.5));
#86687=CARTESIAN_POINT('Ctrl Pts',(20.217598926276,3.11302864551544,48.35));
#86688=CARTESIAN_POINT('Ctrl Pts',(20.2978854887187,3.3508867919445,48.35));
#86689=CARTESIAN_POINT('Ctrl Pts',(20.4562076441944,3.47994545102119,48.35));
#86690=CARTESIAN_POINT('Ctrl Pts',(20.1373126618564,2.48499327898026,48.5));
#86691=CARTESIAN_POINT('Ctrl Pts',(20.1373126618564,2.48499327898026,48.35));
#86692=CARTESIAN_POINT('Ctrl Pts',(20.1373126618564,2.87517049908638,48.5));
#86693=CARTESIAN_POINT('Ctrl Pts',(20.1373126618564,2.87517049908638,48.35));
#86694=CARTESIAN_POINT('Ctrl Pts',(20.217598926276,3.11302864551544,48.5));
#86695=CARTESIAN_POINT('Ctrl Pts',(20.217598926276,3.11302864551544,48.35));
#86696=CARTESIAN_POINT('',(20.1373126618564,2.48499327898026,48.5));
#86697=CARTESIAN_POINT('Ctrl Pts',(20.1373126618564,2.48499327898026,48.5));
#86698=CARTESIAN_POINT('Ctrl Pts',(20.1373126618564,2.87517049908638,48.5));
#86699=CARTESIAN_POINT('Ctrl Pts',(20.217598926276,3.11302864551544,48.5));
#86700=CARTESIAN_POINT('',(20.1373126618564,2.48499327898026,48.35));
#86701=CARTESIAN_POINT('',(20.1373126618564,2.48499327898026,48.5));
#86702=CARTESIAN_POINT('Ctrl Pts',(20.1373126618564,2.48499327898026,48.35));
#86703=CARTESIAN_POINT('Ctrl Pts',(20.1373126618564,2.87517049908638,48.35));
#86704=CARTESIAN_POINT('Ctrl Pts',(20.217598926276,3.11302864551544,48.35));
#86705=CARTESIAN_POINT('Ctrl Pts',(20.3549113385379,1.59058684110642,48.5));
#86706=CARTESIAN_POINT('Ctrl Pts',(20.3549113385379,1.59058684110642,48.35));
#86707=CARTESIAN_POINT('Ctrl Pts',(20.1373126618564,1.86521166563034,48.5));
#86708=CARTESIAN_POINT('Ctrl Pts',(20.1373126618564,1.86521166563034,48.35));
#86709=CARTESIAN_POINT('Ctrl Pts',(20.1373126618564,2.48499327898026,48.5));
#86710=CARTESIAN_POINT('Ctrl Pts',(20.1373126618564,2.48499327898026,48.35));
#86711=CARTESIAN_POINT('Ctrl Pts',(20.3549113385379,1.59058684110642,48.5));
#86712=CARTESIAN_POINT('Ctrl Pts',(20.1373126618564,1.86521166563034,48.5));
#86713=CARTESIAN_POINT('Ctrl Pts',(20.1373126618564,2.48499327898026,48.5));
#86714=CARTESIAN_POINT('Ctrl Pts',(20.3549113385379,1.59058684110642,48.35));
#86715=CARTESIAN_POINT('Ctrl Pts',(20.1373126618564,1.86521166563034,48.35));
#86716=CARTESIAN_POINT('Ctrl Pts',(20.1373126618564,2.48499327898026,48.35));
#86717=CARTESIAN_POINT('Origin',(19.9999999515712,2.48574362695217,48.35));
#86718=CARTESIAN_POINT('Ctrl Pts',(19.1453617326915,2.38444769382477,48.5));
#86719=CARTESIAN_POINT('Ctrl Pts',(19.1453617326915,2.38444769382477,48.35));
#86720=CARTESIAN_POINT('Ctrl Pts',(19.3329469375312,2.38444769382477,48.5));
#86721=CARTESIAN_POINT('Ctrl Pts',(19.3329469375312,2.38444769382477,48.35));
#86722=CARTESIAN_POINT('Ctrl Pts',(19.453751694411,2.5157573223114,48.5));
#86723=CARTESIAN_POINT('Ctrl Pts',(19.453751694411,2.5157573223114,48.35));
#86724=CARTESIAN_POINT('',(19.1453617326915,2.38444769382477,48.5));
#86725=CARTESIAN_POINT('',(19.453751694411,2.5157573223114,48.5));
#86726=CARTESIAN_POINT('Ctrl Pts',(19.1453617326915,2.38444769382477,48.5));
#86727=CARTESIAN_POINT('Ctrl Pts',(19.3329469375312,2.38444769382477,48.5));
#86728=CARTESIAN_POINT('Ctrl Pts',(19.453751694411,2.5157573223114,48.5));
#86729=CARTESIAN_POINT('',(19.1453617326915,2.38444769382477,48.35));
#86730=CARTESIAN_POINT('',(19.1453617326915,2.38444769382477,48.5));
#86731=CARTESIAN_POINT('',(19.453751694411,2.5157573223114,48.35));
#86732=CARTESIAN_POINT('Ctrl Pts',(19.1453617326915,2.38444769382477,48.35));
#86733=CARTESIAN_POINT('Ctrl Pts',(19.3329469375312,2.38444769382477,48.35));
#86734=CARTESIAN_POINT('Ctrl Pts',(19.453751694411,2.5157573223114,48.35));
#86735=CARTESIAN_POINT('',(19.453751694411,2.5157573223114,48.5));
#86736=CARTESIAN_POINT('Ctrl Pts',(18.8324695341289,2.5157573223114,48.5));
#86737=CARTESIAN_POINT('Ctrl Pts',(18.8324695341289,2.5157573223114,48.35));
#86738=CARTESIAN_POINT('Ctrl Pts',(18.9592772237957,2.38444769382477,48.5));
#86739=CARTESIAN_POINT('Ctrl Pts',(18.9592772237957,2.38444769382477,48.35));
#86740=CARTESIAN_POINT('Ctrl Pts',(19.1453617326915,2.38444769382477,48.5));
#86741=CARTESIAN_POINT('Ctrl Pts',(19.1453617326915,2.38444769382477,48.35));
#86742=CARTESIAN_POINT('',(18.8324695341289,2.5157573223114,48.5));
#86743=CARTESIAN_POINT('Ctrl Pts',(18.8324695341289,2.5157573223114,48.5));
#86744=CARTESIAN_POINT('Ctrl Pts',(18.9592772237957,2.38444769382477,48.5));
#86745=CARTESIAN_POINT('Ctrl Pts',(19.1453617326915,2.38444769382477,48.5));
#86746=CARTESIAN_POINT('',(18.8324695341289,2.5157573223114,48.35));
#86747=CARTESIAN_POINT('',(18.8324695341289,2.5157573223114,48.5));
#86748=CARTESIAN_POINT('Ctrl Pts',(18.8324695341289,2.5157573223114,48.35));
#86749=CARTESIAN_POINT('Ctrl Pts',(18.9592772237957,2.38444769382477,48.35));
#86750=CARTESIAN_POINT('Ctrl Pts',(19.1453617326915,2.38444769382477,48.35));
#86751=CARTESIAN_POINT('Ctrl Pts',(18.7056618444622,2.85716244578362,48.5));
#86752=CARTESIAN_POINT('Ctrl Pts',(18.7056618444622,2.85716244578362,48.35));
#86753=CARTESIAN_POINT('Ctrl Pts',(18.7056618444622,2.64706695079803,48.5));
#86754=CARTESIAN_POINT('Ctrl Pts',(18.7056618444622,2.64706695079803,48.35));
#86755=CARTESIAN_POINT('Ctrl Pts',(18.8324695341289,2.5157573223114,48.5));
#86756=CARTESIAN_POINT('Ctrl Pts',(18.8324695341289,2.5157573223114,48.35));
#86757=CARTESIAN_POINT('',(18.7056618444622,2.85716244578362,48.5));
#86758=CARTESIAN_POINT('Ctrl Pts',(18.7056618444622,2.85716244578362,48.5));
#86759=CARTESIAN_POINT('Ctrl Pts',(18.7056618444622,2.64706695079803,48.5));
#86760=CARTESIAN_POINT('Ctrl Pts',(18.8324695341289,2.5157573223114,48.5));
#86761=CARTESIAN_POINT('',(18.7056618444622,2.85716244578362,48.35));
#86762=CARTESIAN_POINT('',(18.7056618444622,2.85716244578362,48.5));
#86763=CARTESIAN_POINT('Ctrl Pts',(18.7056618444622,2.85716244578362,48.35));
#86764=CARTESIAN_POINT('Ctrl Pts',(18.7056618444622,2.64706695079803,48.35));
#86765=CARTESIAN_POINT('Ctrl Pts',(18.8324695341289,2.5157573223114,48.35));
#86766=CARTESIAN_POINT('Ctrl Pts',(18.8392224423587,3.23833563923836,48.5));
#86767=CARTESIAN_POINT('Ctrl Pts',(18.8392224423587,3.23833563923836,48.35));
#86768=CARTESIAN_POINT('Ctrl Pts',(18.7056618444622,3.09126877784729,48.5));
#86769=CARTESIAN_POINT('Ctrl Pts',(18.7056618444622,3.09126877784729,48.35));
#86770=CARTESIAN_POINT('Ctrl Pts',(18.7056618444622,2.85716244578362,48.5));
#86771=CARTESIAN_POINT('Ctrl Pts',(18.7056618444622,2.85716244578362,48.35));
#86772=CARTESIAN_POINT('',(18.8392224423587,3.23833563923836,48.5));
#86773=CARTESIAN_POINT('Ctrl Pts',(18.8392224423587,3.23833563923836,48.5));
#86774=CARTESIAN_POINT('Ctrl Pts',(18.7056618444622,3.09126877784729,48.5));
#86775=CARTESIAN_POINT('Ctrl Pts',(18.7056618444622,2.85716244578362,48.5));
#86776=CARTESIAN_POINT('',(18.8392224423587,3.23833563923836,48.35));
#86777=CARTESIAN_POINT('',(18.8392224423587,3.23833563923836,48.5));
#86778=CARTESIAN_POINT('Ctrl Pts',(18.8392224423587,3.23833563923836,48.35));
#86779=CARTESIAN_POINT('Ctrl Pts',(18.7056618444622,3.09126877784729,48.35));
#86780=CARTESIAN_POINT('Ctrl Pts',(18.7056618444622,2.85716244578362,48.35));
#86781=CARTESIAN_POINT('Ctrl Pts',(19.1528650633991,3.38540250062943,48.5));
#86782=CARTESIAN_POINT('Ctrl Pts',(19.1528650633991,3.38540250062943,48.35));
#86783=CARTESIAN_POINT('Ctrl Pts',(18.9727833382785,3.38540250062943,48.5));
#86784=CARTESIAN_POINT('Ctrl Pts',(18.9727833382785,3.38540250062943,48.35));
#86785=CARTESIAN_POINT('Ctrl Pts',(18.8392224423587,3.23833563923836,48.5));
#86786=CARTESIAN_POINT('Ctrl Pts',(18.8392224423587,3.23833563923836,48.35));
#86787=CARTESIAN_POINT('',(19.1528650633991,3.38540250062943,48.5));
#86788=CARTESIAN_POINT('Ctrl Pts',(19.1528650633991,3.38540250062943,48.5));
#86789=CARTESIAN_POINT('Ctrl Pts',(18.9727833382785,3.38540250062943,48.5));
#86790=CARTESIAN_POINT('Ctrl Pts',(18.8392224423587,3.23833563923836,48.5));
#86791=CARTESIAN_POINT('',(19.1528650633991,3.38540250062943,48.35));
#86792=CARTESIAN_POINT('',(19.1528650633991,3.38540250062943,48.5));
#86793=CARTESIAN_POINT('Ctrl Pts',(19.1528650633991,3.38540250062943,48.35));
#86794=CARTESIAN_POINT('Ctrl Pts',(18.9727833382785,3.38540250062943,48.35));
#86795=CARTESIAN_POINT('Ctrl Pts',(18.8392224423587,3.23833563923836,48.35));
#86796=CARTESIAN_POINT('Ctrl Pts',(19.4507506005466,3.24884036183357,48.5));
#86797=CARTESIAN_POINT('Ctrl Pts',(19.4507506005466,3.24884036183357,48.35));
#86798=CARTESIAN_POINT('Ctrl Pts',(19.3269443027675,3.38540250062943,48.5));
#86799=CARTESIAN_POINT('Ctrl Pts',(19.3269443027675,3.38540250062943,48.35));
#86800=CARTESIAN_POINT('Ctrl Pts',(19.1528650633991,3.38540250062943,48.5));
#86801=CARTESIAN_POINT('Ctrl Pts',(19.1528650633991,3.38540250062943,48.35));
#86802=CARTESIAN_POINT('',(19.4507506005466,3.24884036183357,48.5));
#86803=CARTESIAN_POINT('Ctrl Pts',(19.4507506005466,3.24884036183357,48.5));
#86804=CARTESIAN_POINT('Ctrl Pts',(19.3269443027675,3.38540250062943,48.5));
#86805=CARTESIAN_POINT('Ctrl Pts',(19.1528650633991,3.38540250062943,48.5));
#86806=CARTESIAN_POINT('',(19.4507506005466,3.24884036183357,48.35));
#86807=CARTESIAN_POINT('',(19.4507506005466,3.24884036183357,48.5));
#86808=CARTESIAN_POINT('Ctrl Pts',(19.4507506005466,3.24884036183357,48.35));
#86809=CARTESIAN_POINT('Ctrl Pts',(19.3269443027675,3.38540250062943,48.35));
#86810=CARTESIAN_POINT('Ctrl Pts',(19.1528650633991,3.38540250062943,48.35));
#86811=CARTESIAN_POINT('Ctrl Pts',(19.5745566003025,2.87967258691788,48.5));
#86812=CARTESIAN_POINT('Ctrl Pts',(19.5745566003025,2.87967258691788,48.35));
#86813=CARTESIAN_POINT('Ctrl Pts',(19.5745566003025,3.11227837204933,48.5));
#86814=CARTESIAN_POINT('Ctrl Pts',(19.5745566003025,3.11227837204933,48.35));
#86815=CARTESIAN_POINT('Ctrl Pts',(19.4507506005466,3.24884036183357,48.5));
#86816=CARTESIAN_POINT('Ctrl Pts',(19.4507506005466,3.24884036183357,48.35));
#86817=CARTESIAN_POINT('',(19.5745566003025,2.87967258691788,48.5));
#86818=CARTESIAN_POINT('Ctrl Pts',(19.5745566003025,2.87967258691788,48.5));
#86819=CARTESIAN_POINT('Ctrl Pts',(19.5745566003025,3.11227837204933,48.5));
#86820=CARTESIAN_POINT('Ctrl Pts',(19.4507506005466,3.24884036183357,48.5));
#86821=CARTESIAN_POINT('',(19.5745566003025,2.87967258691788,48.35));
#86822=CARTESIAN_POINT('',(19.5745566003025,2.87967258691788,48.5));
#86823=CARTESIAN_POINT('Ctrl Pts',(19.5745566003025,2.87967258691788,48.35));
#86824=CARTESIAN_POINT('Ctrl Pts',(19.5745566003025,3.11227837204933,48.35));
#86825=CARTESIAN_POINT('Ctrl Pts',(19.4507506005466,3.24884036183357,48.35));
#86826=CARTESIAN_POINT('Ctrl Pts',(19.453751694411,2.5157573223114,48.5));
#86827=CARTESIAN_POINT('Ctrl Pts',(19.453751694411,2.5157573223114,48.35));
#86828=CARTESIAN_POINT('Ctrl Pts',(19.5745566003025,2.64706695079803,48.5));
#86829=CARTESIAN_POINT('Ctrl Pts',(19.5745566003025,2.64706695079803,48.35));
#86830=CARTESIAN_POINT('Ctrl Pts',(19.5745566003025,2.87967258691788,48.5));
#86831=CARTESIAN_POINT('Ctrl Pts',(19.5745566003025,2.87967258691788,48.35));
#86832=CARTESIAN_POINT('Ctrl Pts',(19.453751694411,2.5157573223114,48.5));
#86833=CARTESIAN_POINT('Ctrl Pts',(19.5745566003025,2.64706695079803,48.5));
#86834=CARTESIAN_POINT('Ctrl Pts',(19.5745566003025,2.87967258691788,48.5));
#86835=CARTESIAN_POINT('Ctrl Pts',(19.453751694411,2.5157573223114,48.35));
#86836=CARTESIAN_POINT('Ctrl Pts',(19.5745566003025,2.64706695079803,48.35));
#86837=CARTESIAN_POINT('Ctrl Pts',(19.5745566003025,2.87967258691788,48.35));
#86838=CARTESIAN_POINT('Ctrl Pts',(19.0868350379169,1.36248314380646,48.5));
#86839=CARTESIAN_POINT('Ctrl Pts',(19.0868350379169,1.36248314380646,48.35));
#86840=CARTESIAN_POINT('Ctrl Pts',(18.8287177197635,1.36248314380646,48.5));
#86841=CARTESIAN_POINT('Ctrl Pts',(18.8287177197635,1.36248314380646,48.35));
#86842=CARTESIAN_POINT('Ctrl Pts',(18.6651435010135,1.50579804182053,48.5));
#86843=CARTESIAN_POINT('Ctrl Pts',(18.6651435010135,1.50579804182053,48.35));
#86844=CARTESIAN_POINT('',(19.0868350379169,1.36248314380646,48.5));
#86845=CARTESIAN_POINT('',(18.6651435010135,1.50579804182053,48.5));
#86846=CARTESIAN_POINT('Ctrl Pts',(19.0868350379169,1.36248314380646,48.5));
#86847=CARTESIAN_POINT('Ctrl Pts',(18.8287177197635,1.36248314380646,48.5));
#86848=CARTESIAN_POINT('Ctrl Pts',(18.6651435010135,1.50579804182053,48.5));
#86849=CARTESIAN_POINT('',(19.0868350379169,1.36248314380646,48.35));
#86850=CARTESIAN_POINT('',(19.0868350379169,1.36248314380646,48.5));
#86851=CARTESIAN_POINT('',(18.6651435010135,1.50579804182053,48.35));
#86852=CARTESIAN_POINT('Ctrl Pts',(19.0868350379169,1.36248314380646,48.35));
#86853=CARTESIAN_POINT('Ctrl Pts',(18.8287177197635,1.36248314380646,48.35));
#86854=CARTESIAN_POINT('Ctrl Pts',(18.6651435010135,1.50579804182053,48.35));
#86855=CARTESIAN_POINT('',(18.6651435010135,1.50579804182053,48.5));
#86856=CARTESIAN_POINT('Ctrl Pts',(19.5107778422534,1.49304234981537,48.5));
#86857=CARTESIAN_POINT('Ctrl Pts',(19.5107778422534,1.49304234981537,48.35));
#86858=CARTESIAN_POINT('Ctrl Pts',(19.3299455456436,1.36248314380646,48.5));
#86859=CARTESIAN_POINT('Ctrl Pts',(19.3299455456436,1.36248314380646,48.35));
#86860=CARTESIAN_POINT('Ctrl Pts',(19.0868350379169,1.36248314380646,48.5));
#86861=CARTESIAN_POINT('Ctrl Pts',(19.0868350379169,1.36248314380646,48.35));
#86862=CARTESIAN_POINT('',(19.5107778422534,1.49304234981537,48.5));
#86863=CARTESIAN_POINT('Ctrl Pts',(19.5107778422534,1.49304234981537,48.5));
#86864=CARTESIAN_POINT('Ctrl Pts',(19.3299455456436,1.36248314380646,48.5));
#86865=CARTESIAN_POINT('Ctrl Pts',(19.0868350379169,1.36248314380646,48.5));
#86866=CARTESIAN_POINT('',(19.5107778422534,1.49304234981537,48.35));
#86867=CARTESIAN_POINT('',(19.5107778422534,1.49304234981537,48.5));
#86868=CARTESIAN_POINT('Ctrl Pts',(19.5107778422534,1.49304234981537,48.35));
#86869=CARTESIAN_POINT('Ctrl Pts',(19.3299455456436,1.36248314380646,48.35));
#86870=CARTESIAN_POINT('Ctrl Pts',(19.0868350379169,1.36248314380646,48.35));
#86871=CARTESIAN_POINT('Ctrl Pts',(19.7831513993442,1.87346541881561,48.5));
#86872=CARTESIAN_POINT('Ctrl Pts',(19.7831513993442,1.87346541881561,48.35));
#86873=CARTESIAN_POINT('Ctrl Pts',(19.6916099898517,1.6236018538475,48.5));
#86874=CARTESIAN_POINT('Ctrl Pts',(19.6916099898517,1.6236018538475,48.35));
#86875=CARTESIAN_POINT('Ctrl Pts',(19.5107778422534,1.49304234981537,48.5));
#86876=CARTESIAN_POINT('Ctrl Pts',(19.5107778422534,1.49304234981537,48.35));
#86877=CARTESIAN_POINT('',(19.7831513993442,1.87346541881561,48.5));
#86878=CARTESIAN_POINT('Ctrl Pts',(19.7831513993442,1.87346541881561,48.5));
#86879=CARTESIAN_POINT('Ctrl Pts',(19.6916099898517,1.6236018538475,48.5));
#86880=CARTESIAN_POINT('Ctrl Pts',(19.5107778422534,1.49304234981537,48.5));
#86881=CARTESIAN_POINT('',(19.7831513993442,1.87346541881561,48.35));
#86882=CARTESIAN_POINT('',(19.7831513993442,1.87346541881561,48.5));
#86883=CARTESIAN_POINT('Ctrl Pts',(19.7831513993442,1.87346541881561,48.35));
#86884=CARTESIAN_POINT('Ctrl Pts',(19.6916099898517,1.6236018538475,48.35));
#86885=CARTESIAN_POINT('Ctrl Pts',(19.5107778422534,1.49304234981537,48.35));
#86886=CARTESIAN_POINT('Ctrl Pts',(19.8746934048831,2.5450205206871,48.5));
#86887=CARTESIAN_POINT('Ctrl Pts',(19.8746934048831,2.5450205206871,48.35));
#86888=CARTESIAN_POINT('Ctrl Pts',(19.8746934048831,2.12332898378372,48.5));
#86889=CARTESIAN_POINT('Ctrl Pts',(19.8746934048831,2.12332898378372,48.35));
#86890=CARTESIAN_POINT('Ctrl Pts',(19.7831513993442,1.87346541881561,48.5));
#86891=CARTESIAN_POINT('Ctrl Pts',(19.7831513993442,1.87346541881561,48.35));
#86892=CARTESIAN_POINT('',(19.8746934048831,2.5450205206871,48.5));
#86893=CARTESIAN_POINT('Ctrl Pts',(19.8746934048831,2.5450205206871,48.5));
#86894=CARTESIAN_POINT('Ctrl Pts',(19.8746934048831,2.12332898378372,48.5));
#86895=CARTESIAN_POINT('Ctrl Pts',(19.7831513993442,1.87346541881561,48.5));
#86896=CARTESIAN_POINT('',(19.8746934048831,2.5450205206871,48.35));
#86897=CARTESIAN_POINT('',(19.8746934048831,2.5450205206871,48.5));
#86898=CARTESIAN_POINT('Ctrl Pts',(19.8746934048831,2.5450205206871,48.35));
#86899=CARTESIAN_POINT('Ctrl Pts',(19.8746934048831,2.12332898378372,48.35));
#86900=CARTESIAN_POINT('Ctrl Pts',(19.7831513993442,1.87346541881561,48.35));
#86901=CARTESIAN_POINT('Ctrl Pts',(19.7824012748897,3.16405186057091,48.5));
#86902=CARTESIAN_POINT('Ctrl Pts',(19.7824012748897,3.16405186057091,48.35));
#86903=CARTESIAN_POINT('Ctrl Pts',(19.8746934048831,2.95020470023155,48.5));
#86904=CARTESIAN_POINT('Ctrl Pts',(19.8746934048831,2.95020470023155,48.35));
#86905=CARTESIAN_POINT('Ctrl Pts',(19.8746934048831,2.5450205206871,48.5));
#86906=CARTESIAN_POINT('Ctrl Pts',(19.8746934048831,2.5450205206871,48.35));
#86907=CARTESIAN_POINT('',(19.7824012748897,3.16405186057091,48.5));
#86908=CARTESIAN_POINT('Ctrl Pts',(19.7824012748897,3.16405186057091,48.5));
#86909=CARTESIAN_POINT('Ctrl Pts',(19.8746934048831,2.95020470023155,48.5));
#86910=CARTESIAN_POINT('Ctrl Pts',(19.8746934048831,2.5450205206871,48.5));
#86911=CARTESIAN_POINT('',(19.7824012748897,3.16405186057091,48.35));
#86912=CARTESIAN_POINT('',(19.7824012748897,3.16405186057091,48.5));
#86913=CARTESIAN_POINT('Ctrl Pts',(19.7824012748897,3.16405186057091,48.35));
#86914=CARTESIAN_POINT('Ctrl Pts',(19.8746934048831,2.95020470023155,48.35));
#86915=CARTESIAN_POINT('Ctrl Pts',(19.8746934048831,2.5450205206871,48.35));
#86916=CARTESIAN_POINT('Ctrl Pts',(19.5122783891857,3.49345156550407,48.5));
#86917=CARTESIAN_POINT('Ctrl Pts',(19.5122783891857,3.49345156550407,48.35));
#86918=CARTESIAN_POINT('Ctrl Pts',(19.6901091448963,3.37789902091026,48.5));
#86919=CARTESIAN_POINT('Ctrl Pts',(19.6901091448963,3.37789902091026,48.35));
#86920=CARTESIAN_POINT('Ctrl Pts',(19.7824012748897,3.16405186057091,48.5));
#86921=CARTESIAN_POINT('Ctrl Pts',(19.7824012748897,3.16405186057091,48.35));
#86922=CARTESIAN_POINT('',(19.5122783891857,3.49345156550407,48.5));
#86923=CARTESIAN_POINT('Ctrl Pts',(19.5122783891857,3.49345156550407,48.5));
#86924=CARTESIAN_POINT('Ctrl Pts',(19.6901091448963,3.37789902091026,48.5));
#86925=CARTESIAN_POINT('Ctrl Pts',(19.7824012748897,3.16405186057091,48.5));
#86926=CARTESIAN_POINT('',(19.5122783891857,3.49345156550407,48.35));
#86927=CARTESIAN_POINT('',(19.5122783891857,3.49345156550407,48.5));
#86928=CARTESIAN_POINT('Ctrl Pts',(19.5122783891857,3.49345156550407,48.35));
#86929=CARTESIAN_POINT('Ctrl Pts',(19.6901091448963,3.37789902091026,48.35));
#86930=CARTESIAN_POINT('Ctrl Pts',(19.7824012748897,3.16405186057091,48.35));
#86931=CARTESIAN_POINT('Ctrl Pts',(19.119850050658,3.60900411009789,48.5));
#86932=CARTESIAN_POINT('Ctrl Pts',(19.119850050658,3.60900411009789,48.35));
#86933=CARTESIAN_POINT('Ctrl Pts',(19.3344476334751,3.60900411009789,48.5));
#86934=CARTESIAN_POINT('Ctrl Pts',(19.3344476334751,3.60900411009789,48.35));
#86935=CARTESIAN_POINT('Ctrl Pts',(19.5122783891857,3.49345156550407,48.5));
#86936=CARTESIAN_POINT('Ctrl Pts',(19.5122783891857,3.49345156550407,48.35));
#86937=CARTESIAN_POINT('',(19.119850050658,3.60900411009789,48.5));
#86938=CARTESIAN_POINT('Ctrl Pts',(19.119850050658,3.60900411009789,48.5));
#86939=CARTESIAN_POINT('Ctrl Pts',(19.3344476334751,3.60900411009789,48.5));
#86940=CARTESIAN_POINT('Ctrl Pts',(19.5122783891857,3.49345156550407,48.5));
#86941=CARTESIAN_POINT('',(19.119850050658,3.60900411009789,48.35));
#86942=CARTESIAN_POINT('',(19.119850050658,3.60900411009789,48.5));
#86943=CARTESIAN_POINT('Ctrl Pts',(19.119850050658,3.60900411009789,48.35));
#86944=CARTESIAN_POINT('Ctrl Pts',(19.3344476334751,3.60900411009789,48.35));
#86945=CARTESIAN_POINT('Ctrl Pts',(19.5122783891857,3.49345156550407,48.35));
#86946=CARTESIAN_POINT('Ctrl Pts',(18.6253752820194,3.40491139888763,48.5));
#86947=CARTESIAN_POINT('Ctrl Pts',(18.6253752820194,3.40491139888763,48.35));
#86948=CARTESIAN_POINT('Ctrl Pts',(18.8227149359882,3.60900411009789,48.5));
#86949=CARTESIAN_POINT('Ctrl Pts',(18.8227149359882,3.60900411009789,48.35));
#86950=CARTESIAN_POINT('Ctrl Pts',(19.119850050658,3.60900411009789,48.5));
#86951=CARTESIAN_POINT('Ctrl Pts',(19.119850050658,3.60900411009789,48.35));
#86952=CARTESIAN_POINT('',(18.6253752820194,3.40491139888763,48.5));
#86953=CARTESIAN_POINT('Ctrl Pts',(18.6253752820194,3.40491139888763,48.5));
#86954=CARTESIAN_POINT('Ctrl Pts',(18.8227149359882,3.60900411009789,48.5));
#86955=CARTESIAN_POINT('Ctrl Pts',(19.119850050658,3.60900411009789,48.5));
#86956=CARTESIAN_POINT('',(18.6253752820194,3.40491139888763,48.35));
#86957=CARTESIAN_POINT('',(18.6253752820194,3.40491139888763,48.5));
#86958=CARTESIAN_POINT('Ctrl Pts',(18.6253752820194,3.40491139888763,48.35));
#86959=CARTESIAN_POINT('Ctrl Pts',(18.8227149359882,3.60900411009789,48.35));
#86960=CARTESIAN_POINT('Ctrl Pts',(19.119850050658,3.60900411009789,48.35));
#86961=CARTESIAN_POINT('Ctrl Pts',(18.4280356280506,2.866166472435,48.5));
#86962=CARTESIAN_POINT('Ctrl Pts',(18.4280356280506,2.866166472435,48.35));
#86963=CARTESIAN_POINT('Ctrl Pts',(18.4280356280506,3.20081853866577,48.5));
#86964=CARTESIAN_POINT('Ctrl Pts',(18.4280356280506,3.20081853866577,48.35));
#86965=CARTESIAN_POINT('Ctrl Pts',(18.6253752820194,3.40491139888763,48.5));
#86966=CARTESIAN_POINT('Ctrl Pts',(18.6253752820194,3.40491139888763,48.35));
#86967=CARTESIAN_POINT('',(18.4280356280506,2.866166472435,48.5));
#86968=CARTESIAN_POINT('Ctrl Pts',(18.4280356280506,2.866166472435,48.5));
#86969=CARTESIAN_POINT('Ctrl Pts',(18.4280356280506,3.20081853866577,48.5));
#86970=CARTESIAN_POINT('Ctrl Pts',(18.6253752820194,3.40491139888763,48.5));
#86971=CARTESIAN_POINT('',(18.4280356280506,2.866166472435,48.35));
#86972=CARTESIAN_POINT('',(18.4280356280506,2.866166472435,48.5));
#86973=CARTESIAN_POINT('Ctrl Pts',(18.4280356280506,2.866166472435,48.35));
#86974=CARTESIAN_POINT('Ctrl Pts',(18.4280356280506,3.20081853866577,48.35));
#86975=CARTESIAN_POINT('Ctrl Pts',(18.6253752820194,3.40491139888763,48.35));
#86976=CARTESIAN_POINT('Ctrl Pts',(18.6171215288341,2.34392920136452,48.5));
#86977=CARTESIAN_POINT('Ctrl Pts',(18.6171215288341,2.34392920136452,48.35));
#86978=CARTESIAN_POINT('Ctrl Pts',(18.4280356280506,2.54201912879944,48.5));
#86979=CARTESIAN_POINT('Ctrl Pts',(18.4280356280506,2.54201912879944,48.35));
#86980=CARTESIAN_POINT('Ctrl Pts',(18.4280356280506,2.866166472435,48.5));
#86981=CARTESIAN_POINT('Ctrl Pts',(18.4280356280506,2.866166472435,48.35));
#86982=CARTESIAN_POINT('',(18.6171215288341,2.34392920136452,48.5));
#86983=CARTESIAN_POINT('Ctrl Pts',(18.6171215288341,2.34392920136452,48.5));
#86984=CARTESIAN_POINT('Ctrl Pts',(18.4280356280506,2.54201912879944,48.5));
#86985=CARTESIAN_POINT('Ctrl Pts',(18.4280356280506,2.866166472435,48.5));
#86986=CARTESIAN_POINT('',(18.6171215288341,2.34392920136452,48.35));
#86987=CARTESIAN_POINT('',(18.6171215288341,2.34392920136452,48.5));
#86988=CARTESIAN_POINT('Ctrl Pts',(18.6171215288341,2.34392920136452,48.35));
#86989=CARTESIAN_POINT('Ctrl Pts',(18.4280356280506,2.54201912879944,48.35));
#86990=CARTESIAN_POINT('Ctrl Pts',(18.4280356280506,2.866166472435,48.35));
#86991=CARTESIAN_POINT('Ctrl Pts',(19.0793317072093,2.14583912491798,48.5));
#86992=CARTESIAN_POINT('Ctrl Pts',(19.0793317072093,2.14583912491798,48.35));
#86993=CARTESIAN_POINT('Ctrl Pts',(18.8062074296176,2.14583912491798,48.5));
#86994=CARTESIAN_POINT('Ctrl Pts',(18.8062074296176,2.14583912491798,48.35));
#86995=CARTESIAN_POINT('Ctrl Pts',(18.6171215288341,2.34392920136452,48.5));
#86996=CARTESIAN_POINT('Ctrl Pts',(18.6171215288341,2.34392920136452,48.35));
#86997=CARTESIAN_POINT('',(19.0793317072093,2.14583912491798,48.5));
#86998=CARTESIAN_POINT('Ctrl Pts',(19.0793317072093,2.14583912491798,48.5));
#86999=CARTESIAN_POINT('Ctrl Pts',(18.8062074296176,2.14583912491798,48.5));
#87000=CARTESIAN_POINT('Ctrl Pts',(18.6171215288341,2.34392920136452,48.5));
#87001=CARTESIAN_POINT('',(19.0793317072093,2.14583912491798,48.35));
#87002=CARTESIAN_POINT('',(19.0793317072093,2.14583912491798,48.5));
#87003=CARTESIAN_POINT('Ctrl Pts',(19.0793317072093,2.14583912491798,48.35));
#87004=CARTESIAN_POINT('Ctrl Pts',(18.8062074296176,2.14583912491798,48.35));
#87005=CARTESIAN_POINT('Ctrl Pts',(18.6171215288341,2.34392920136452,48.35));
#87006=CARTESIAN_POINT('Ctrl Pts',(19.383219730109,2.22612553834915,48.5));
#87007=CARTESIAN_POINT('Ctrl Pts',(19.383219730109,2.22612553834915,48.35));
#87008=CARTESIAN_POINT('Ctrl Pts',(19.2429059259593,2.14583912491798,48.5));
#87009=CARTESIAN_POINT('Ctrl Pts',(19.2429059259593,2.14583912491798,48.35));
#87010=CARTESIAN_POINT('Ctrl Pts',(19.0793317072093,2.14583912491798,48.5));
#87011=CARTESIAN_POINT('Ctrl Pts',(19.0793317072093,2.14583912491798,48.35));
#87012=CARTESIAN_POINT('',(19.383219730109,2.22612553834915,48.5));
#87013=CARTESIAN_POINT('Ctrl Pts',(19.383219730109,2.22612553834915,48.5));
#87014=CARTESIAN_POINT('Ctrl Pts',(19.2429059259593,2.14583912491798,48.5));
#87015=CARTESIAN_POINT('Ctrl Pts',(19.0793317072093,2.14583912491798,48.5));
#87016=CARTESIAN_POINT('',(19.383219730109,2.22612553834915,48.35));
#87017=CARTESIAN_POINT('',(19.383219730109,2.22612553834915,48.5));
#87018=CARTESIAN_POINT('Ctrl Pts',(19.383219730109,2.22612553834915,48.35));
#87019=CARTESIAN_POINT('Ctrl Pts',(19.2429059259593,2.14583912491798,48.35));
#87020=CARTESIAN_POINT('Ctrl Pts',(19.0793317072093,2.14583912491798,48.35));
#87021=CARTESIAN_POINT('Ctrl Pts',(19.6045705191791,2.43547075986862,48.5));
#87022=CARTESIAN_POINT('Ctrl Pts',(19.6045705191791,2.43547075986862,48.35));
#87023=CARTESIAN_POINT('Ctrl Pts',(19.5235335342586,2.30641210079193,48.5));
#87024=CARTESIAN_POINT('Ctrl Pts',(19.5235335342586,2.30641210079193,48.35));
#87025=CARTESIAN_POINT('Ctrl Pts',(19.383219730109,2.22612553834915,48.5));
#87026=CARTESIAN_POINT('Ctrl Pts',(19.383219730109,2.22612553834915,48.35));
#87027=CARTESIAN_POINT('',(19.6045705191791,2.43547075986862,48.5));
#87028=CARTESIAN_POINT('Ctrl Pts',(19.6045705191791,2.43547075986862,48.5));
#87029=CARTESIAN_POINT('Ctrl Pts',(19.5235335342586,2.30641210079193,48.5));
#87030=CARTESIAN_POINT('Ctrl Pts',(19.383219730109,2.22612553834915,48.5));
#87031=CARTESIAN_POINT('',(19.6045705191791,2.43547075986862,48.35));
#87032=CARTESIAN_POINT('',(19.6045705191791,2.43547075986862,48.5));
#87033=CARTESIAN_POINT('Ctrl Pts',(19.6045705191791,2.43547075986862,48.35));
#87034=CARTESIAN_POINT('Ctrl Pts',(19.5235335342586,2.30641210079193,48.35));
#87035=CARTESIAN_POINT('Ctrl Pts',(19.383219730109,2.22612553834915,48.35));
#87036=CARTESIAN_POINT('Ctrl Pts',(19.6060710661113,2.3814463019371,48.5));
#87037=CARTESIAN_POINT('Ctrl Pts',(19.6060710661113,2.3814463019371,48.35));
#87038=CARTESIAN_POINT('Ctrl Pts',(19.6060710661113,2.39945435523987,48.5));
#87039=CARTESIAN_POINT('Ctrl Pts',(19.6060710661113,2.39945435523987,48.35));
#87040=CARTESIAN_POINT('Ctrl Pts',(19.6045705191791,2.43547075986862,48.5));
#87041=CARTESIAN_POINT('Ctrl Pts',(19.6045705191791,2.43547075986862,48.35));
#87042=CARTESIAN_POINT('',(19.6060710661113,2.3814463019371,48.5));
#87043=CARTESIAN_POINT('Ctrl Pts',(19.6060710661113,2.3814463019371,48.5));
#87044=CARTESIAN_POINT('Ctrl Pts',(19.6060710661113,2.39945435523987,48.5));
#87045=CARTESIAN_POINT('Ctrl Pts',(19.6045705191791,2.43547075986862,48.5));
#87046=CARTESIAN_POINT('',(19.6060710661113,2.3814463019371,48.35));
#87047=CARTESIAN_POINT('',(19.6060710661113,2.3814463019371,48.5));
#87048=CARTESIAN_POINT('Ctrl Pts',(19.6060710661113,2.3814463019371,48.35));
#87049=CARTESIAN_POINT('Ctrl Pts',(19.6060710661113,2.39945435523987,48.35));
#87050=CARTESIAN_POINT('Ctrl Pts',(19.6045705191791,2.43547075986862,48.35));
#87051=CARTESIAN_POINT('Ctrl Pts',(19.5655527226627,2.05129617452621,48.5));
#87052=CARTESIAN_POINT('Ctrl Pts',(19.5655527226627,2.05129617452621,48.35));
#87053=CARTESIAN_POINT('Ctrl Pts',(19.6060710661113,2.21336984634399,48.5));
#87054=CARTESIAN_POINT('Ctrl Pts',(19.6060710661113,2.21336984634399,48.35));
#87055=CARTESIAN_POINT('Ctrl Pts',(19.6060710661113,2.3814463019371,48.5));
#87056=CARTESIAN_POINT('Ctrl Pts',(19.6060710661113,2.3814463019371,48.35));
#87057=CARTESIAN_POINT('',(19.5655527226627,2.05129617452621,48.5));
#87058=CARTESIAN_POINT('Ctrl Pts',(19.5655527226627,2.05129617452621,48.5));
#87059=CARTESIAN_POINT('Ctrl Pts',(19.6060710661113,2.21336984634399,48.5));
#87060=CARTESIAN_POINT('Ctrl Pts',(19.6060710661113,2.3814463019371,48.5));
#87061=CARTESIAN_POINT('',(19.5655527226627,2.05129617452621,48.35));
#87062=CARTESIAN_POINT('',(19.5655527226627,2.05129617452621,48.5));
#87063=CARTESIAN_POINT('Ctrl Pts',(19.5655527226627,2.05129617452621,48.35));
#87064=CARTESIAN_POINT('Ctrl Pts',(19.6060710661113,2.21336984634399,48.35));
#87065=CARTESIAN_POINT('Ctrl Pts',(19.6060710661113,2.3814463019371,48.35));
#87066=CARTESIAN_POINT('Ctrl Pts',(19.465006839484,1.79392898082733,48.5));
#87067=CARTESIAN_POINT('Ctrl Pts',(19.465006839484,1.79392898082733,48.35));
#87068=CARTESIAN_POINT('Ctrl Pts',(19.5250340811908,1.88922250270844,48.5));
#87069=CARTESIAN_POINT('Ctrl Pts',(19.5250340811908,1.88922250270844,48.35));
#87070=CARTESIAN_POINT('Ctrl Pts',(19.5655527226627,2.05129617452621,48.5));
#87071=CARTESIAN_POINT('Ctrl Pts',(19.5655527226627,2.05129617452621,48.35));
#87072=CARTESIAN_POINT('',(19.465006839484,1.79392898082733,48.5));
#87073=CARTESIAN_POINT('Ctrl Pts',(19.465006839484,1.79392898082733,48.5));
#87074=CARTESIAN_POINT('Ctrl Pts',(19.5250340811908,1.88922250270844,48.5));
#87075=CARTESIAN_POINT('Ctrl Pts',(19.5655527226627,2.05129617452621,48.5));
#87076=CARTESIAN_POINT('',(19.465006839484,1.79392898082733,48.35));
#87077=CARTESIAN_POINT('',(19.465006839484,1.79392898082733,48.5));
#87078=CARTESIAN_POINT('Ctrl Pts',(19.465006839484,1.79392898082733,48.35));
#87079=CARTESIAN_POINT('Ctrl Pts',(19.5250340811908,1.88922250270844,48.35));
#87080=CARTESIAN_POINT('Ctrl Pts',(19.5655527226627,2.05129617452621,48.35));
#87081=CARTESIAN_POINT('Ctrl Pts',(19.3111870698631,1.64160990715027,48.5));
#87082=CARTESIAN_POINT('Ctrl Pts',(19.3111870698631,1.64160990715027,48.35));
#87083=CARTESIAN_POINT('Ctrl Pts',(19.4049795977771,1.69863575696945,48.5));
#87084=CARTESIAN_POINT('Ctrl Pts',(19.4049795977771,1.69863575696945,48.35));
#87085=CARTESIAN_POINT('Ctrl Pts',(19.465006839484,1.79392898082733,48.5));
#87086=CARTESIAN_POINT('Ctrl Pts',(19.465006839484,1.79392898082733,48.35));
#87087=CARTESIAN_POINT('',(19.3111870698631,1.64160990715027,48.5));
#87088=CARTESIAN_POINT('Ctrl Pts',(19.3111870698631,1.64160990715027,48.5));
#87089=CARTESIAN_POINT('Ctrl Pts',(19.4049795977771,1.69863575696945,48.5));
#87090=CARTESIAN_POINT('Ctrl Pts',(19.465006839484,1.79392898082733,48.5));
#87091=CARTESIAN_POINT('',(19.3111870698631,1.64160990715027,48.35));
#87092=CARTESIAN_POINT('',(19.3111870698631,1.64160990715027,48.5));
#87093=CARTESIAN_POINT('Ctrl Pts',(19.3111870698631,1.64160990715027,48.35));
#87094=CARTESIAN_POINT('Ctrl Pts',(19.4049795977771,1.69863575696945,48.35));
#87095=CARTESIAN_POINT('Ctrl Pts',(19.465006839484,1.79392898082733,48.35));
#87096=CARTESIAN_POINT('Ctrl Pts',(19.0928378216922,1.58458405733109,48.5));
#87097=CARTESIAN_POINT('Ctrl Pts',(19.0928378216922,1.58458405733109,48.35));
#87098=CARTESIAN_POINT('Ctrl Pts',(19.2173943929374,1.58458405733109,48.5));
#87099=CARTESIAN_POINT('Ctrl Pts',(19.2173943929374,1.58458405733109,48.35));
#87100=CARTESIAN_POINT('Ctrl Pts',(19.3111870698631,1.64160990715027,48.5));
#87101=CARTESIAN_POINT('Ctrl Pts',(19.3111870698631,1.64160990715027,48.35));
#87102=CARTESIAN_POINT('',(19.0928378216922,1.58458405733109,48.5));
#87103=CARTESIAN_POINT('Ctrl Pts',(19.0928378216922,1.58458405733109,48.5));
#87104=CARTESIAN_POINT('Ctrl Pts',(19.2173943929374,1.58458405733109,48.5));
#87105=CARTESIAN_POINT('Ctrl Pts',(19.3111870698631,1.64160990715027,48.5));
#87106=CARTESIAN_POINT('',(19.0928378216922,1.58458405733109,48.35));
#87107=CARTESIAN_POINT('',(19.0928378216922,1.58458405733109,48.5));
#87108=CARTESIAN_POINT('Ctrl Pts',(19.0928378216922,1.58458405733109,48.35));
#87109=CARTESIAN_POINT('Ctrl Pts',(19.2173943929374,1.58458405733109,48.35));
#87110=CARTESIAN_POINT('Ctrl Pts',(19.3111870698631,1.64160990715027,48.35));
#87111=CARTESIAN_POINT('Ctrl Pts',(18.8542294017971,1.66712158918381,48.5));
#87112=CARTESIAN_POINT('Ctrl Pts',(18.8542294017971,1.66712158918381,48.35));
#87113=CARTESIAN_POINT('Ctrl Pts',(18.947271656245,1.58458405733109,48.5));
#87114=CARTESIAN_POINT('Ctrl Pts',(18.947271656245,1.58458405733109,48.35));
#87115=CARTESIAN_POINT('Ctrl Pts',(19.0928378216922,1.58458405733109,48.5));
#87116=CARTESIAN_POINT('Ctrl Pts',(19.0928378216922,1.58458405733109,48.35));
#87117=CARTESIAN_POINT('',(18.8542294017971,1.66712158918381,48.5));
#87118=CARTESIAN_POINT('Ctrl Pts',(18.8542294017971,1.66712158918381,48.5));
#87119=CARTESIAN_POINT('Ctrl Pts',(18.947271656245,1.58458405733109,48.5));
#87120=CARTESIAN_POINT('Ctrl Pts',(19.0928378216922,1.58458405733109,48.5));
#87121=CARTESIAN_POINT('',(18.8542294017971,1.66712158918381,48.35));
#87122=CARTESIAN_POINT('',(18.8542294017971,1.66712158918381,48.5));
#87123=CARTESIAN_POINT('Ctrl Pts',(18.8542294017971,1.66712158918381,48.35));
#87124=CARTESIAN_POINT('Ctrl Pts',(18.947271656245,1.58458405733109,48.35));
#87125=CARTESIAN_POINT('Ctrl Pts',(19.0928378216922,1.58458405733109,48.35));
#87126=CARTESIAN_POINT('Ctrl Pts',(18.728172134608,1.93274223804474,48.5));
#87127=CARTESIAN_POINT('Ctrl Pts',(18.728172134608,1.93274223804474,48.35));
#87128=CARTESIAN_POINT('Ctrl Pts',(18.7611871473491,1.74965912103653,48.5));
#87129=CARTESIAN_POINT('Ctrl Pts',(18.7611871473491,1.74965912103653,48.35));
#87130=CARTESIAN_POINT('Ctrl Pts',(18.8542294017971,1.66712158918381,48.5));
#87131=CARTESIAN_POINT('Ctrl Pts',(18.8542294017971,1.66712158918381,48.35));
#87132=CARTESIAN_POINT('',(18.728172134608,1.93274223804474,48.5));
#87133=CARTESIAN_POINT('Ctrl Pts',(18.728172134608,1.93274223804474,48.5));
#87134=CARTESIAN_POINT('Ctrl Pts',(18.7611871473491,1.74965912103653,48.5));
#87135=CARTESIAN_POINT('Ctrl Pts',(18.8542294017971,1.66712158918381,48.5));
#87136=CARTESIAN_POINT('',(18.728172134608,1.93274223804474,48.35));
#87137=CARTESIAN_POINT('',(18.728172134608,1.93274223804474,48.5));
#87138=CARTESIAN_POINT('Ctrl Pts',(18.728172134608,1.93274223804474,48.35));
#87139=CARTESIAN_POINT('Ctrl Pts',(18.7611871473491,1.74965912103653,48.35));
#87140=CARTESIAN_POINT('Ctrl Pts',(18.8542294017971,1.66712158918381,48.35));
#87141=CARTESIAN_POINT('Origin',(18.4685541205108,1.90873140096664,48.5));
#87142=CARTESIAN_POINT('',(18.4685541205108,1.90873140096664,48.5));
#87143=CARTESIAN_POINT('',(9.5918801338843,1.08776998336471,48.5));
#87144=CARTESIAN_POINT('',(18.4685541205108,1.90873140096664,48.35));
#87145=CARTESIAN_POINT('',(18.4685541205108,1.90873140096664,48.5));
#87146=CARTESIAN_POINT('',(18.4685541205108,1.90873140096664,48.35));
#87147=CARTESIAN_POINT('Ctrl Pts',(18.6651435010135,1.50579804182053,48.5));
#87148=CARTESIAN_POINT('Ctrl Pts',(18.6651435010135,1.50579804182053,48.35));
#87149=CARTESIAN_POINT('Ctrl Pts',(18.5015691332519,1.64911323785782,48.5));
#87150=CARTESIAN_POINT('Ctrl Pts',(18.5015691332519,1.64911323785782,48.35));
#87151=CARTESIAN_POINT('Ctrl Pts',(18.4685541205108,1.90873140096664,48.5));
#87152=CARTESIAN_POINT('Ctrl Pts',(18.4685541205108,1.90873140096664,48.35));
#87153=CARTESIAN_POINT('Ctrl Pts',(18.6651435010135,1.50579804182053,48.5));
#87154=CARTESIAN_POINT('Ctrl Pts',(18.5015691332519,1.64911323785782,48.5));
#87155=CARTESIAN_POINT('Ctrl Pts',(18.4685541205108,1.90873140096664,48.5));
#87156=CARTESIAN_POINT('Ctrl Pts',(18.6651435010135,1.50579804182053,48.35));
#87157=CARTESIAN_POINT('Ctrl Pts',(18.5015691332519,1.64911323785782,48.35));
#87158=CARTESIAN_POINT('Ctrl Pts',(18.4685541205108,1.90873140096664,48.35));
#87159=CARTESIAN_POINT('Origin',(19.9999999515712,2.48574362695217,48.35));
#87160=CARTESIAN_POINT('Origin',(0.,8.,48.5));
#87161=CARTESIAN_POINT('Origin',(0.,8.,48.5));
#87162=CARTESIAN_POINT('Origin',(199.1,6.,48.5));
#87163=CARTESIAN_POINT('',(199.1,6.,48.5));
#87164=CARTESIAN_POINT('',(198.9,6.,48.5));
#87165=CARTESIAN_POINT('',(99.55,6.,48.5));
#87166=CARTESIAN_POINT('',(199.1,6.,48.35));
#87167=CARTESIAN_POINT('',(199.1,6.,48.5));
#87168=CARTESIAN_POINT('',(198.9,6.,48.35));
#87169=CARTESIAN_POINT('',(198.9,6.,48.35));
#87170=CARTESIAN_POINT('',(198.9,6.,48.5));
#87171=CARTESIAN_POINT('Origin',(199.1,7.4,48.5));
#87172=CARTESIAN_POINT('',(199.1,7.4,48.5));
#87173=CARTESIAN_POINT('',(199.1,7.7,48.5));
#87174=CARTESIAN_POINT('',(199.1,7.4,48.35));
#87175=CARTESIAN_POINT('',(199.1,7.4,48.5));
#87176=CARTESIAN_POINT('',(199.1,6.,48.35));
#87177=CARTESIAN_POINT('Origin',(198.9,7.4,48.5));
#87178=CARTESIAN_POINT('',(198.9,7.4,48.5));
#87179=CARTESIAN_POINT('',(99.45,7.4,48.5));
#87180=CARTESIAN_POINT('',(198.9,7.4,48.35));
#87181=CARTESIAN_POINT('',(198.9,7.4,48.5));
#87182=CARTESIAN_POINT('',(199.1,7.4,48.35));
#87183=CARTESIAN_POINT('Origin',(198.9,6.,48.5));
#87184=CARTESIAN_POINT('',(198.9,7.,48.5));
#87185=CARTESIAN_POINT('',(198.9,7.4,48.35));
#87186=CARTESIAN_POINT('Origin',(199.,6.7,48.35));
#87187=CARTESIAN_POINT('Origin',(197.1,6.,48.5));
#87188=CARTESIAN_POINT('',(197.1,6.,48.5));
#87189=CARTESIAN_POINT('',(196.9,6.,48.5));
#87190=CARTESIAN_POINT('',(98.55,6.,48.5));
#87191=CARTESIAN_POINT('',(197.1,6.,48.35));
#87192=CARTESIAN_POINT('',(197.1,6.,48.5));
#87193=CARTESIAN_POINT('',(196.9,6.,48.35));
#87194=CARTESIAN_POINT('',(196.9,6.,48.35));
#87195=CARTESIAN_POINT('',(196.9,6.,48.5));
#87196=CARTESIAN_POINT('Origin',(197.1,7.4,48.5));
#87197=CARTESIAN_POINT('',(197.1,7.4,48.5));
#87198=CARTESIAN_POINT('',(197.1,7.7,48.5));
#87199=CARTESIAN_POINT('',(197.1,7.4,48.35));
#87200=CARTESIAN_POINT('',(197.1,7.4,48.5));
#87201=CARTESIAN_POINT('',(197.1,6.,48.35));
#87202=CARTESIAN_POINT('Origin',(196.9,7.4,48.5));
#87203=CARTESIAN_POINT('',(196.9,7.4,48.5));
#87204=CARTESIAN_POINT('',(98.45,7.4,48.5));
#87205=CARTESIAN_POINT('',(196.9,7.4,48.35));
#87206=CARTESIAN_POINT('',(196.9,7.4,48.5));
#87207=CARTESIAN_POINT('',(197.1,7.4,48.35));
#87208=CARTESIAN_POINT('Origin',(196.9,6.,48.5));
#87209=CARTESIAN_POINT('',(196.9,7.,48.5));
#87210=CARTESIAN_POINT('',(196.9,7.4,48.35));
#87211=CARTESIAN_POINT('Origin',(197.,6.7,48.35));
#87212=CARTESIAN_POINT('Origin',(195.1,5.2,48.5));
#87213=CARTESIAN_POINT('',(195.1,5.2,48.5));
#87214=CARTESIAN_POINT('',(194.9,5.2,48.5));
#87215=CARTESIAN_POINT('',(97.55,5.2,48.5));
#87216=CARTESIAN_POINT('',(195.1,5.2,48.35));
#87217=CARTESIAN_POINT('',(195.1,5.2,48.5));
#87218=CARTESIAN_POINT('',(194.9,5.2,48.35));
#87219=CARTESIAN_POINT('',(194.9,5.2,48.35));
#87220=CARTESIAN_POINT('',(194.9,5.2,48.5));
#87221=CARTESIAN_POINT('Origin',(195.1,7.4,48.5));
#87222=CARTESIAN_POINT('',(195.1,7.4,48.5));
#87223=CARTESIAN_POINT('',(195.1,7.7,48.5));
#87224=CARTESIAN_POINT('',(195.1,7.4,48.35));
#87225=CARTESIAN_POINT('',(195.1,7.4,48.5));
#87226=CARTESIAN_POINT('',(195.1,5.2,48.35));
#87227=CARTESIAN_POINT('Origin',(194.9,7.4,48.5));
#87228=CARTESIAN_POINT('',(194.9,7.4,48.5));
#87229=CARTESIAN_POINT('',(97.45,7.4,48.5));
#87230=CARTESIAN_POINT('',(194.9,7.4,48.35));
#87231=CARTESIAN_POINT('',(194.9,7.4,48.5));
#87232=CARTESIAN_POINT('',(195.1,7.4,48.35));
#87233=CARTESIAN_POINT('Origin',(194.9,5.2,48.5));
#87234=CARTESIAN_POINT('',(194.9,6.6,48.5));
#87235=CARTESIAN_POINT('',(194.9,7.4,48.35));
#87236=CARTESIAN_POINT('Origin',(195.,6.3,48.35));
#87237=CARTESIAN_POINT('Origin',(193.1,6.,48.5));
#87238=CARTESIAN_POINT('',(193.1,6.,48.5));
#87239=CARTESIAN_POINT('',(192.9,6.,48.5));
#87240=CARTESIAN_POINT('',(96.55,6.,48.5));
#87241=CARTESIAN_POINT('',(193.1,6.,48.35));
#87242=CARTESIAN_POINT('',(193.1,6.,48.5));
#87243=CARTESIAN_POINT('',(192.9,6.,48.35));
#87244=CARTESIAN_POINT('',(192.9,6.,48.35));
#87245=CARTESIAN_POINT('',(192.9,6.,48.5));
#87246=CARTESIAN_POINT('Origin',(193.1,7.4,48.5));
#87247=CARTESIAN_POINT('',(193.1,7.4,48.5));
#87248=CARTESIAN_POINT('',(193.1,7.7,48.5));
#87249=CARTESIAN_POINT('',(193.1,7.4,48.35));
#87250=CARTESIAN_POINT('',(193.1,7.4,48.5));
#87251=CARTESIAN_POINT('',(193.1,6.,48.35));
#87252=CARTESIAN_POINT('Origin',(192.9,7.4,48.5));
#87253=CARTESIAN_POINT('',(192.9,7.4,48.5));
#87254=CARTESIAN_POINT('',(96.45,7.4,48.5));
#87255=CARTESIAN_POINT('',(192.9,7.4,48.35));
#87256=CARTESIAN_POINT('',(192.9,7.4,48.5));
#87257=CARTESIAN_POINT('',(193.1,7.4,48.35));
#87258=CARTESIAN_POINT('Origin',(192.9,6.,48.5));
#87259=CARTESIAN_POINT('',(192.9,7.,48.5));
#87260=CARTESIAN_POINT('',(192.9,7.4,48.35));
#87261=CARTESIAN_POINT('Origin',(193.,6.7,48.35));
#87262=CARTESIAN_POINT('Origin',(191.1,6.,48.5));
#87263=CARTESIAN_POINT('',(191.1,6.,48.5));
#87264=CARTESIAN_POINT('',(190.9,6.,48.5));
#87265=CARTESIAN_POINT('',(95.55,6.,48.5));
#87266=CARTESIAN_POINT('',(191.1,6.,48.35));
#87267=CARTESIAN_POINT('',(191.1,6.,48.5));
#87268=CARTESIAN_POINT('',(190.9,6.,48.35));
#87269=CARTESIAN_POINT('',(190.9,6.,48.35));
#87270=CARTESIAN_POINT('',(190.9,6.,48.5));
#87271=CARTESIAN_POINT('Origin',(191.1,7.4,48.5));
#87272=CARTESIAN_POINT('',(191.1,7.4,48.5));
#87273=CARTESIAN_POINT('',(191.1,7.7,48.5));
#87274=CARTESIAN_POINT('',(191.1,7.4,48.35));
#87275=CARTESIAN_POINT('',(191.1,7.4,48.5));
#87276=CARTESIAN_POINT('',(191.1,6.,48.35));
#87277=CARTESIAN_POINT('Origin',(190.9,7.4,48.5));
#87278=CARTESIAN_POINT('',(190.9,7.4,48.5));
#87279=CARTESIAN_POINT('',(95.45,7.4,48.5));
#87280=CARTESIAN_POINT('',(190.9,7.4,48.35));
#87281=CARTESIAN_POINT('',(190.9,7.4,48.5));
#87282=CARTESIAN_POINT('',(191.1,7.4,48.35));
#87283=CARTESIAN_POINT('Origin',(190.9,6.,48.5));
#87284=CARTESIAN_POINT('',(190.9,7.,48.5));
#87285=CARTESIAN_POINT('',(190.9,7.4,48.35));
#87286=CARTESIAN_POINT('Origin',(191.,6.7,48.35));
#87287=CARTESIAN_POINT('Origin',(189.1,6.,48.5));
#87288=CARTESIAN_POINT('',(189.1,6.,48.5));
#87289=CARTESIAN_POINT('',(188.9,6.,48.5));
#87290=CARTESIAN_POINT('',(94.55,6.,48.5));
#87291=CARTESIAN_POINT('',(189.1,6.,48.35));
#87292=CARTESIAN_POINT('',(189.1,6.,48.5));
#87293=CARTESIAN_POINT('',(188.9,6.,48.35));
#87294=CARTESIAN_POINT('',(188.9,6.,48.35));
#87295=CARTESIAN_POINT('',(188.9,6.,48.5));
#87296=CARTESIAN_POINT('Origin',(189.1,7.4,48.5));
#87297=CARTESIAN_POINT('',(189.1,7.4,48.5));
#87298=CARTESIAN_POINT('',(189.1,7.7,48.5));
#87299=CARTESIAN_POINT('',(189.1,7.4,48.35));
#87300=CARTESIAN_POINT('',(189.1,7.4,48.5));
#87301=CARTESIAN_POINT('',(189.1,6.,48.35));
#87302=CARTESIAN_POINT('Origin',(188.9,7.4,48.5));
#87303=CARTESIAN_POINT('',(188.9,7.4,48.5));
#87304=CARTESIAN_POINT('',(94.45,7.4,48.5));
#87305=CARTESIAN_POINT('',(188.9,7.4,48.35));
#87306=CARTESIAN_POINT('',(188.9,7.4,48.5));
#87307=CARTESIAN_POINT('',(189.1,7.4,48.35));
#87308=CARTESIAN_POINT('Origin',(188.9,6.,48.5));
#87309=CARTESIAN_POINT('',(188.9,7.,48.5));
#87310=CARTESIAN_POINT('',(188.9,7.4,48.35));
#87311=CARTESIAN_POINT('Origin',(189.,6.7,48.35));
#87312=CARTESIAN_POINT('Origin',(187.1,6.,48.5));
#87313=CARTESIAN_POINT('',(187.1,6.,48.5));
#87314=CARTESIAN_POINT('',(186.9,6.,48.5));
#87315=CARTESIAN_POINT('',(93.55,6.,48.5));
#87316=CARTESIAN_POINT('',(187.1,6.,48.35));
#87317=CARTESIAN_POINT('',(187.1,6.,48.5));
#87318=CARTESIAN_POINT('',(186.9,6.,48.35));
#87319=CARTESIAN_POINT('',(186.9,6.,48.35));
#87320=CARTESIAN_POINT('',(186.9,6.,48.5));
#87321=CARTESIAN_POINT('Origin',(187.1,7.4,48.5));
#87322=CARTESIAN_POINT('',(187.1,7.4,48.5));
#87323=CARTESIAN_POINT('',(187.1,7.7,48.5));
#87324=CARTESIAN_POINT('',(187.1,7.4,48.35));
#87325=CARTESIAN_POINT('',(187.1,7.4,48.5));
#87326=CARTESIAN_POINT('',(187.1,6.,48.35));
#87327=CARTESIAN_POINT('Origin',(186.9,7.4,48.5));
#87328=CARTESIAN_POINT('',(186.9,7.4,48.5));
#87329=CARTESIAN_POINT('',(93.45,7.4,48.5));
#87330=CARTESIAN_POINT('',(186.9,7.4,48.35));
#87331=CARTESIAN_POINT('',(186.9,7.4,48.5));
#87332=CARTESIAN_POINT('',(187.1,7.4,48.35));
#87333=CARTESIAN_POINT('Origin',(186.9,6.,48.5));
#87334=CARTESIAN_POINT('',(186.9,7.,48.5));
#87335=CARTESIAN_POINT('',(186.9,7.4,48.35));
#87336=CARTESIAN_POINT('Origin',(187.,6.7,48.35));
#87337=CARTESIAN_POINT('Origin',(185.1,5.2,48.5));
#87338=CARTESIAN_POINT('',(185.1,5.2,48.5));
#87339=CARTESIAN_POINT('',(184.9,5.2,48.5));
#87340=CARTESIAN_POINT('',(92.55,5.2,48.5));
#87341=CARTESIAN_POINT('',(185.1,5.2,48.35));
#87342=CARTESIAN_POINT('',(185.1,5.2,48.5));
#87343=CARTESIAN_POINT('',(184.9,5.2,48.35));
#87344=CARTESIAN_POINT('',(184.9,5.2,48.35));
#87345=CARTESIAN_POINT('',(184.9,5.2,48.5));
#87346=CARTESIAN_POINT('Origin',(185.1,7.4,48.5));
#87347=CARTESIAN_POINT('',(185.1,7.4,48.5));
#87348=CARTESIAN_POINT('',(185.1,7.7,48.5));
#87349=CARTESIAN_POINT('',(185.1,7.4,48.35));
#87350=CARTESIAN_POINT('',(185.1,7.4,48.5));
#87351=CARTESIAN_POINT('',(185.1,5.2,48.35));
#87352=CARTESIAN_POINT('Origin',(184.9,7.4,48.5));
#87353=CARTESIAN_POINT('',(184.9,7.4,48.5));
#87354=CARTESIAN_POINT('',(92.45,7.4,48.5));
#87355=CARTESIAN_POINT('',(184.9,7.4,48.35));
#87356=CARTESIAN_POINT('',(184.9,7.4,48.5));
#87357=CARTESIAN_POINT('',(185.1,7.4,48.35));
#87358=CARTESIAN_POINT('Origin',(184.9,5.2,48.5));
#87359=CARTESIAN_POINT('',(184.9,6.6,48.5));
#87360=CARTESIAN_POINT('',(184.9,7.4,48.35));
#87361=CARTESIAN_POINT('Origin',(185.,6.3,48.35));
#87362=CARTESIAN_POINT('Origin',(183.1,6.,48.5));
#87363=CARTESIAN_POINT('',(183.1,6.,48.5));
#87364=CARTESIAN_POINT('',(182.9,6.,48.5));
#87365=CARTESIAN_POINT('',(91.55,6.,48.5));
#87366=CARTESIAN_POINT('',(183.1,6.,48.35));
#87367=CARTESIAN_POINT('',(183.1,6.,48.5));
#87368=CARTESIAN_POINT('',(182.9,6.,48.35));
#87369=CARTESIAN_POINT('',(182.9,6.,48.35));
#87370=CARTESIAN_POINT('',(182.9,6.,48.5));
#87371=CARTESIAN_POINT('Origin',(183.1,7.4,48.5));
#87372=CARTESIAN_POINT('',(183.1,7.4,48.5));
#87373=CARTESIAN_POINT('',(183.1,7.7,48.5));
#87374=CARTESIAN_POINT('',(183.1,7.4,48.35));
#87375=CARTESIAN_POINT('',(183.1,7.4,48.5));
#87376=CARTESIAN_POINT('',(183.1,6.,48.35));
#87377=CARTESIAN_POINT('Origin',(182.9,7.4,48.5));
#87378=CARTESIAN_POINT('',(182.9,7.4,48.5));
#87379=CARTESIAN_POINT('',(91.45,7.4,48.5));
#87380=CARTESIAN_POINT('',(182.9,7.4,48.35));
#87381=CARTESIAN_POINT('',(182.9,7.4,48.5));
#87382=CARTESIAN_POINT('',(183.1,7.4,48.35));
#87383=CARTESIAN_POINT('Origin',(182.9,6.,48.5));
#87384=CARTESIAN_POINT('',(182.9,7.,48.5));
#87385=CARTESIAN_POINT('',(182.9,7.4,48.35));
#87386=CARTESIAN_POINT('Origin',(183.,6.7,48.35));
#87387=CARTESIAN_POINT('Origin',(181.1,6.,48.5));
#87388=CARTESIAN_POINT('',(181.1,6.,48.5));
#87389=CARTESIAN_POINT('',(180.9,6.,48.5));
#87390=CARTESIAN_POINT('',(90.55,6.,48.5));
#87391=CARTESIAN_POINT('',(181.1,6.,48.35));
#87392=CARTESIAN_POINT('',(181.1,6.,48.5));
#87393=CARTESIAN_POINT('',(180.9,6.,48.35));
#87394=CARTESIAN_POINT('',(180.9,6.,48.35));
#87395=CARTESIAN_POINT('',(180.9,6.,48.5));
#87396=CARTESIAN_POINT('Origin',(181.1,7.4,48.5));
#87397=CARTESIAN_POINT('',(181.1,7.4,48.5));
#87398=CARTESIAN_POINT('',(181.1,7.7,48.5));
#87399=CARTESIAN_POINT('',(181.1,7.4,48.35));
#87400=CARTESIAN_POINT('',(181.1,7.4,48.5));
#87401=CARTESIAN_POINT('',(181.1,6.,48.35));
#87402=CARTESIAN_POINT('Origin',(180.9,7.4,48.5));
#87403=CARTESIAN_POINT('',(180.9,7.4,48.5));
#87404=CARTESIAN_POINT('',(90.45,7.4,48.5));
#87405=CARTESIAN_POINT('',(180.9,7.4,48.35));
#87406=CARTESIAN_POINT('',(180.9,7.4,48.5));
#87407=CARTESIAN_POINT('',(181.1,7.4,48.35));
#87408=CARTESIAN_POINT('Origin',(180.9,6.,48.5));
#87409=CARTESIAN_POINT('',(180.9,7.,48.5));
#87410=CARTESIAN_POINT('',(180.9,7.4,48.35));
#87411=CARTESIAN_POINT('Origin',(181.,6.7,48.35));
#87412=CARTESIAN_POINT('Origin',(179.1,6.,48.5));
#87413=CARTESIAN_POINT('',(179.1,6.,48.5));
#87414=CARTESIAN_POINT('',(178.9,6.,48.5));
#87415=CARTESIAN_POINT('',(89.55,6.,48.5));
#87416=CARTESIAN_POINT('',(179.1,6.,48.35));
#87417=CARTESIAN_POINT('',(179.1,6.,48.5));
#87418=CARTESIAN_POINT('',(178.9,6.,48.35));
#87419=CARTESIAN_POINT('',(178.9,6.,48.35));
#87420=CARTESIAN_POINT('',(178.9,6.,48.5));
#87421=CARTESIAN_POINT('Origin',(179.1,7.4,48.5));
#87422=CARTESIAN_POINT('',(179.1,7.4,48.5));
#87423=CARTESIAN_POINT('',(179.1,7.7,48.5));
#87424=CARTESIAN_POINT('',(179.1,7.4,48.35));
#87425=CARTESIAN_POINT('',(179.1,7.4,48.5));
#87426=CARTESIAN_POINT('',(179.1,6.,48.35));
#87427=CARTESIAN_POINT('Origin',(178.9,7.4,48.5));
#87428=CARTESIAN_POINT('',(178.9,7.4,48.5));
#87429=CARTESIAN_POINT('',(89.45,7.4,48.5));
#87430=CARTESIAN_POINT('',(178.9,7.4,48.35));
#87431=CARTESIAN_POINT('',(178.9,7.4,48.5));
#87432=CARTESIAN_POINT('',(179.1,7.4,48.35));
#87433=CARTESIAN_POINT('Origin',(178.9,6.,48.5));
#87434=CARTESIAN_POINT('',(178.9,7.,48.5));
#87435=CARTESIAN_POINT('',(178.9,7.4,48.35));
#87436=CARTESIAN_POINT('Origin',(179.,6.7,48.35));
#87437=CARTESIAN_POINT('Origin',(177.1,6.,48.5));
#87438=CARTESIAN_POINT('',(177.1,6.,48.5));
#87439=CARTESIAN_POINT('',(176.9,6.,48.5));
#87440=CARTESIAN_POINT('',(88.55,6.,48.5));
#87441=CARTESIAN_POINT('',(177.1,6.,48.35));
#87442=CARTESIAN_POINT('',(177.1,6.,48.5));
#87443=CARTESIAN_POINT('',(176.9,6.,48.35));
#87444=CARTESIAN_POINT('',(176.9,6.,48.35));
#87445=CARTESIAN_POINT('',(176.9,6.,48.5));
#87446=CARTESIAN_POINT('Origin',(177.1,7.4,48.5));
#87447=CARTESIAN_POINT('',(177.1,7.4,48.5));
#87448=CARTESIAN_POINT('',(177.1,7.7,48.5));
#87449=CARTESIAN_POINT('',(177.1,7.4,48.35));
#87450=CARTESIAN_POINT('',(177.1,7.4,48.5));
#87451=CARTESIAN_POINT('',(177.1,6.,48.35));
#87452=CARTESIAN_POINT('Origin',(176.9,7.4,48.5));
#87453=CARTESIAN_POINT('',(176.9,7.4,48.5));
#87454=CARTESIAN_POINT('',(88.45,7.4,48.5));
#87455=CARTESIAN_POINT('',(176.9,7.4,48.35));
#87456=CARTESIAN_POINT('',(176.9,7.4,48.5));
#87457=CARTESIAN_POINT('',(177.1,7.4,48.35));
#87458=CARTESIAN_POINT('Origin',(176.9,6.,48.5));
#87459=CARTESIAN_POINT('',(176.9,7.,48.5));
#87460=CARTESIAN_POINT('',(176.9,7.4,48.35));
#87461=CARTESIAN_POINT('Origin',(177.,6.7,48.35));
#87462=CARTESIAN_POINT('Origin',(175.1,5.2,48.5));
#87463=CARTESIAN_POINT('',(175.1,5.2,48.5));
#87464=CARTESIAN_POINT('',(174.9,5.2,48.5));
#87465=CARTESIAN_POINT('',(87.55,5.2,48.5));
#87466=CARTESIAN_POINT('',(175.1,5.2,48.35));
#87467=CARTESIAN_POINT('',(175.1,5.2,48.5));
#87468=CARTESIAN_POINT('',(174.9,5.2,48.35));
#87469=CARTESIAN_POINT('',(174.9,5.2,48.35));
#87470=CARTESIAN_POINT('',(174.9,5.2,48.5));
#87471=CARTESIAN_POINT('Origin',(175.1,7.4,48.5));
#87472=CARTESIAN_POINT('',(175.1,7.4,48.5));
#87473=CARTESIAN_POINT('',(175.1,7.7,48.5));
#87474=CARTESIAN_POINT('',(175.1,7.4,48.35));
#87475=CARTESIAN_POINT('',(175.1,7.4,48.5));
#87476=CARTESIAN_POINT('',(175.1,5.2,48.35));
#87477=CARTESIAN_POINT('Origin',(174.9,7.4,48.5));
#87478=CARTESIAN_POINT('',(174.9,7.4,48.5));
#87479=CARTESIAN_POINT('',(87.45,7.4,48.5));
#87480=CARTESIAN_POINT('',(174.9,7.4,48.35));
#87481=CARTESIAN_POINT('',(174.9,7.4,48.5));
#87482=CARTESIAN_POINT('',(175.1,7.4,48.35));
#87483=CARTESIAN_POINT('Origin',(174.9,5.2,48.5));
#87484=CARTESIAN_POINT('',(174.9,6.6,48.5));
#87485=CARTESIAN_POINT('',(174.9,7.4,48.35));
#87486=CARTESIAN_POINT('Origin',(175.,6.3,48.35));
#87487=CARTESIAN_POINT('Origin',(173.1,6.,48.5));
#87488=CARTESIAN_POINT('',(173.1,6.,48.5));
#87489=CARTESIAN_POINT('',(172.9,6.,48.5));
#87490=CARTESIAN_POINT('',(86.55,6.,48.5));
#87491=CARTESIAN_POINT('',(173.1,6.,48.35));
#87492=CARTESIAN_POINT('',(173.1,6.,48.5));
#87493=CARTESIAN_POINT('',(172.9,6.,48.35));
#87494=CARTESIAN_POINT('',(172.9,6.,48.35));
#87495=CARTESIAN_POINT('',(172.9,6.,48.5));
#87496=CARTESIAN_POINT('Origin',(173.1,7.4,48.5));
#87497=CARTESIAN_POINT('',(173.1,7.4,48.5));
#87498=CARTESIAN_POINT('',(173.1,7.7,48.5));
#87499=CARTESIAN_POINT('',(173.1,7.4,48.35));
#87500=CARTESIAN_POINT('',(173.1,7.4,48.5));
#87501=CARTESIAN_POINT('',(173.1,6.,48.35));
#87502=CARTESIAN_POINT('Origin',(172.9,7.4,48.5));
#87503=CARTESIAN_POINT('',(172.9,7.4,48.5));
#87504=CARTESIAN_POINT('',(86.45,7.4,48.5));
#87505=CARTESIAN_POINT('',(172.9,7.4,48.35));
#87506=CARTESIAN_POINT('',(172.9,7.4,48.5));
#87507=CARTESIAN_POINT('',(173.1,7.4,48.35));
#87508=CARTESIAN_POINT('Origin',(172.9,6.,48.5));
#87509=CARTESIAN_POINT('',(172.9,7.,48.5));
#87510=CARTESIAN_POINT('',(172.9,7.4,48.35));
#87511=CARTESIAN_POINT('Origin',(173.,6.7,48.35));
#87512=CARTESIAN_POINT('Origin',(171.1,6.,48.5));
#87513=CARTESIAN_POINT('',(171.1,6.,48.5));
#87514=CARTESIAN_POINT('',(170.9,6.,48.5));
#87515=CARTESIAN_POINT('',(85.55,6.,48.5));
#87516=CARTESIAN_POINT('',(171.1,6.,48.35));
#87517=CARTESIAN_POINT('',(171.1,6.,48.5));
#87518=CARTESIAN_POINT('',(170.9,6.,48.35));
#87519=CARTESIAN_POINT('',(170.9,6.,48.35));
#87520=CARTESIAN_POINT('',(170.9,6.,48.5));
#87521=CARTESIAN_POINT('Origin',(171.1,7.4,48.5));
#87522=CARTESIAN_POINT('',(171.1,7.4,48.5));
#87523=CARTESIAN_POINT('',(171.1,7.7,48.5));
#87524=CARTESIAN_POINT('',(171.1,7.4,48.35));
#87525=CARTESIAN_POINT('',(171.1,7.4,48.5));
#87526=CARTESIAN_POINT('',(171.1,6.,48.35));
#87527=CARTESIAN_POINT('Origin',(170.9,7.4,48.5));
#87528=CARTESIAN_POINT('',(170.9,7.4,48.5));
#87529=CARTESIAN_POINT('',(85.45,7.4,48.5));
#87530=CARTESIAN_POINT('',(170.9,7.4,48.35));
#87531=CARTESIAN_POINT('',(170.9,7.4,48.5));
#87532=CARTESIAN_POINT('',(171.1,7.4,48.35));
#87533=CARTESIAN_POINT('Origin',(170.9,6.,48.5));
#87534=CARTESIAN_POINT('',(170.9,7.,48.5));
#87535=CARTESIAN_POINT('',(170.9,7.4,48.35));
#87536=CARTESIAN_POINT('Origin',(171.,6.7,48.35));
#87537=CARTESIAN_POINT('Origin',(169.1,6.,48.5));
#87538=CARTESIAN_POINT('',(169.1,6.,48.5));
#87539=CARTESIAN_POINT('',(168.9,6.,48.5));
#87540=CARTESIAN_POINT('',(84.55,6.,48.5));
#87541=CARTESIAN_POINT('',(169.1,6.,48.35));
#87542=CARTESIAN_POINT('',(169.1,6.,48.5));
#87543=CARTESIAN_POINT('',(168.9,6.,48.35));
#87544=CARTESIAN_POINT('',(168.9,6.,48.35));
#87545=CARTESIAN_POINT('',(168.9,6.,48.5));
#87546=CARTESIAN_POINT('Origin',(169.1,7.4,48.5));
#87547=CARTESIAN_POINT('',(169.1,7.4,48.5));
#87548=CARTESIAN_POINT('',(169.1,7.7,48.5));
#87549=CARTESIAN_POINT('',(169.1,7.4,48.35));
#87550=CARTESIAN_POINT('',(169.1,7.4,48.5));
#87551=CARTESIAN_POINT('',(169.1,6.,48.35));
#87552=CARTESIAN_POINT('Origin',(168.9,7.4,48.5));
#87553=CARTESIAN_POINT('',(168.9,7.4,48.5));
#87554=CARTESIAN_POINT('',(84.45,7.4,48.5));
#87555=CARTESIAN_POINT('',(168.9,7.4,48.35));
#87556=CARTESIAN_POINT('',(168.9,7.4,48.5));
#87557=CARTESIAN_POINT('',(169.1,7.4,48.35));
#87558=CARTESIAN_POINT('Origin',(168.9,6.,48.5));
#87559=CARTESIAN_POINT('',(168.9,7.,48.5));
#87560=CARTESIAN_POINT('',(168.9,7.4,48.35));
#87561=CARTESIAN_POINT('Origin',(169.,6.7,48.35));
#87562=CARTESIAN_POINT('Origin',(167.1,6.,48.5));
#87563=CARTESIAN_POINT('',(167.1,6.,48.5));
#87564=CARTESIAN_POINT('',(166.9,6.,48.5));
#87565=CARTESIAN_POINT('',(83.55,6.,48.5));
#87566=CARTESIAN_POINT('',(167.1,6.,48.35));
#87567=CARTESIAN_POINT('',(167.1,6.,48.5));
#87568=CARTESIAN_POINT('',(166.9,6.,48.35));
#87569=CARTESIAN_POINT('',(166.9,6.,48.35));
#87570=CARTESIAN_POINT('',(166.9,6.,48.5));
#87571=CARTESIAN_POINT('Origin',(167.1,7.4,48.5));
#87572=CARTESIAN_POINT('',(167.1,7.4,48.5));
#87573=CARTESIAN_POINT('',(167.1,7.7,48.5));
#87574=CARTESIAN_POINT('',(167.1,7.4,48.35));
#87575=CARTESIAN_POINT('',(167.1,7.4,48.5));
#87576=CARTESIAN_POINT('',(167.1,6.,48.35));
#87577=CARTESIAN_POINT('Origin',(166.9,7.4,48.5));
#87578=CARTESIAN_POINT('',(166.9,7.4,48.5));
#87579=CARTESIAN_POINT('',(83.45,7.4,48.5));
#87580=CARTESIAN_POINT('',(166.9,7.4,48.35));
#87581=CARTESIAN_POINT('',(166.9,7.4,48.5));
#87582=CARTESIAN_POINT('',(167.1,7.4,48.35));
#87583=CARTESIAN_POINT('Origin',(166.9,6.,48.5));
#87584=CARTESIAN_POINT('',(166.9,7.,48.5));
#87585=CARTESIAN_POINT('',(166.9,7.4,48.35));
#87586=CARTESIAN_POINT('Origin',(167.,6.7,48.35));
#87587=CARTESIAN_POINT('Origin',(165.1,5.2,48.5));
#87588=CARTESIAN_POINT('',(165.1,5.2,48.5));
#87589=CARTESIAN_POINT('',(164.9,5.2,48.5));
#87590=CARTESIAN_POINT('',(82.55,5.2,48.5));
#87591=CARTESIAN_POINT('',(165.1,5.2,48.35));
#87592=CARTESIAN_POINT('',(165.1,5.2,48.5));
#87593=CARTESIAN_POINT('',(164.9,5.2,48.35));
#87594=CARTESIAN_POINT('',(164.9,5.2,48.35));
#87595=CARTESIAN_POINT('',(164.9,5.2,48.5));
#87596=CARTESIAN_POINT('Origin',(165.1,7.4,48.5));
#87597=CARTESIAN_POINT('',(165.1,7.4,48.5));
#87598=CARTESIAN_POINT('',(165.1,7.7,48.5));
#87599=CARTESIAN_POINT('',(165.1,7.4,48.35));
#87600=CARTESIAN_POINT('',(165.1,7.4,48.5));
#87601=CARTESIAN_POINT('',(165.1,5.2,48.35));
#87602=CARTESIAN_POINT('Origin',(164.9,7.4,48.5));
#87603=CARTESIAN_POINT('',(164.9,7.4,48.5));
#87604=CARTESIAN_POINT('',(82.45,7.4,48.5));
#87605=CARTESIAN_POINT('',(164.9,7.4,48.35));
#87606=CARTESIAN_POINT('',(164.9,7.4,48.5));
#87607=CARTESIAN_POINT('',(165.1,7.4,48.35));
#87608=CARTESIAN_POINT('Origin',(164.9,5.2,48.5));
#87609=CARTESIAN_POINT('',(164.9,6.6,48.5));
#87610=CARTESIAN_POINT('',(164.9,7.4,48.35));
#87611=CARTESIAN_POINT('Origin',(165.,6.3,48.35));
#87612=CARTESIAN_POINT('Origin',(163.1,6.,48.5));
#87613=CARTESIAN_POINT('',(163.1,6.,48.5));
#87614=CARTESIAN_POINT('',(162.9,6.,48.5));
#87615=CARTESIAN_POINT('',(81.55,6.,48.5));
#87616=CARTESIAN_POINT('',(163.1,6.,48.35));
#87617=CARTESIAN_POINT('',(163.1,6.,48.5));
#87618=CARTESIAN_POINT('',(162.9,6.,48.35));
#87619=CARTESIAN_POINT('',(162.9,6.,48.35));
#87620=CARTESIAN_POINT('',(162.9,6.,48.5));
#87621=CARTESIAN_POINT('Origin',(163.1,7.4,48.5));
#87622=CARTESIAN_POINT('',(163.1,7.4,48.5));
#87623=CARTESIAN_POINT('',(163.1,7.7,48.5));
#87624=CARTESIAN_POINT('',(163.1,7.4,48.35));
#87625=CARTESIAN_POINT('',(163.1,7.4,48.5));
#87626=CARTESIAN_POINT('',(163.1,6.,48.35));
#87627=CARTESIAN_POINT('Origin',(162.9,7.4,48.5));
#87628=CARTESIAN_POINT('',(162.9,7.4,48.5));
#87629=CARTESIAN_POINT('',(81.45,7.4,48.5));
#87630=CARTESIAN_POINT('',(162.9,7.4,48.35));
#87631=CARTESIAN_POINT('',(162.9,7.4,48.5));
#87632=CARTESIAN_POINT('',(163.1,7.4,48.35));
#87633=CARTESIAN_POINT('Origin',(162.9,6.,48.5));
#87634=CARTESIAN_POINT('',(162.9,7.,48.5));
#87635=CARTESIAN_POINT('',(162.9,7.4,48.35));
#87636=CARTESIAN_POINT('Origin',(163.,6.7,48.35));
#87637=CARTESIAN_POINT('Origin',(161.1,6.,48.5));
#87638=CARTESIAN_POINT('',(161.1,6.,48.5));
#87639=CARTESIAN_POINT('',(160.9,6.,48.5));
#87640=CARTESIAN_POINT('',(80.55,6.,48.5));
#87641=CARTESIAN_POINT('',(161.1,6.,48.35));
#87642=CARTESIAN_POINT('',(161.1,6.,48.5));
#87643=CARTESIAN_POINT('',(160.9,6.,48.35));
#87644=CARTESIAN_POINT('',(160.9,6.,48.35));
#87645=CARTESIAN_POINT('',(160.9,6.,48.5));
#87646=CARTESIAN_POINT('Origin',(161.1,7.4,48.5));
#87647=CARTESIAN_POINT('',(161.1,7.4,48.5));
#87648=CARTESIAN_POINT('',(161.1,7.7,48.5));
#87649=CARTESIAN_POINT('',(161.1,7.4,48.35));
#87650=CARTESIAN_POINT('',(161.1,7.4,48.5));
#87651=CARTESIAN_POINT('',(161.1,6.,48.35));
#87652=CARTESIAN_POINT('Origin',(160.9,7.4,48.5));
#87653=CARTESIAN_POINT('',(160.9,7.4,48.5));
#87654=CARTESIAN_POINT('',(80.45,7.4,48.5));
#87655=CARTESIAN_POINT('',(160.9,7.4,48.35));
#87656=CARTESIAN_POINT('',(160.9,7.4,48.5));
#87657=CARTESIAN_POINT('',(161.1,7.4,48.35));
#87658=CARTESIAN_POINT('Origin',(160.9,6.,48.5));
#87659=CARTESIAN_POINT('',(160.9,7.,48.5));
#87660=CARTESIAN_POINT('',(160.9,7.4,48.35));
#87661=CARTESIAN_POINT('Origin',(161.,6.7,48.35));
#87662=CARTESIAN_POINT('Origin',(159.1,6.,48.5));
#87663=CARTESIAN_POINT('',(159.1,6.,48.5));
#87664=CARTESIAN_POINT('',(158.9,6.,48.5));
#87665=CARTESIAN_POINT('',(79.55,6.,48.5));
#87666=CARTESIAN_POINT('',(159.1,6.,48.35));
#87667=CARTESIAN_POINT('',(159.1,6.,48.5));
#87668=CARTESIAN_POINT('',(158.9,6.,48.35));
#87669=CARTESIAN_POINT('',(158.9,6.,48.35));
#87670=CARTESIAN_POINT('',(158.9,6.,48.5));
#87671=CARTESIAN_POINT('Origin',(159.1,7.4,48.5));
#87672=CARTESIAN_POINT('',(159.1,7.4,48.5));
#87673=CARTESIAN_POINT('',(159.1,7.7,48.5));
#87674=CARTESIAN_POINT('',(159.1,7.4,48.35));
#87675=CARTESIAN_POINT('',(159.1,7.4,48.5));
#87676=CARTESIAN_POINT('',(159.1,6.,48.35));
#87677=CARTESIAN_POINT('Origin',(158.9,7.4,48.5));
#87678=CARTESIAN_POINT('',(158.9,7.4,48.5));
#87679=CARTESIAN_POINT('',(79.45,7.4,48.5));
#87680=CARTESIAN_POINT('',(158.9,7.4,48.35));
#87681=CARTESIAN_POINT('',(158.9,7.4,48.5));
#87682=CARTESIAN_POINT('',(159.1,7.4,48.35));
#87683=CARTESIAN_POINT('Origin',(158.9,6.,48.5));
#87684=CARTESIAN_POINT('',(158.9,7.,48.5));
#87685=CARTESIAN_POINT('',(158.9,7.4,48.35));
#87686=CARTESIAN_POINT('Origin',(159.,6.7,48.35));
#87687=CARTESIAN_POINT('Origin',(157.1,6.,48.5));
#87688=CARTESIAN_POINT('',(157.1,6.,48.5));
#87689=CARTESIAN_POINT('',(156.9,6.,48.5));
#87690=CARTESIAN_POINT('',(78.55,6.,48.5));
#87691=CARTESIAN_POINT('',(157.1,6.,48.35));
#87692=CARTESIAN_POINT('',(157.1,6.,48.5));
#87693=CARTESIAN_POINT('',(156.9,6.,48.35));
#87694=CARTESIAN_POINT('',(156.9,6.,48.35));
#87695=CARTESIAN_POINT('',(156.9,6.,48.5));
#87696=CARTESIAN_POINT('Origin',(157.1,7.4,48.5));
#87697=CARTESIAN_POINT('',(157.1,7.4,48.5));
#87698=CARTESIAN_POINT('',(157.1,7.7,48.5));
#87699=CARTESIAN_POINT('',(157.1,7.4,48.35));
#87700=CARTESIAN_POINT('',(157.1,7.4,48.5));
#87701=CARTESIAN_POINT('',(157.1,6.,48.35));
#87702=CARTESIAN_POINT('Origin',(156.9,7.4,48.5));
#87703=CARTESIAN_POINT('',(156.9,7.4,48.5));
#87704=CARTESIAN_POINT('',(78.45,7.4,48.5));
#87705=CARTESIAN_POINT('',(156.9,7.4,48.35));
#87706=CARTESIAN_POINT('',(156.9,7.4,48.5));
#87707=CARTESIAN_POINT('',(157.1,7.4,48.35));
#87708=CARTESIAN_POINT('Origin',(156.9,6.,48.5));
#87709=CARTESIAN_POINT('',(156.9,7.,48.5));
#87710=CARTESIAN_POINT('',(156.9,7.4,48.35));
#87711=CARTESIAN_POINT('Origin',(157.,6.7,48.35));
#87712=CARTESIAN_POINT('Origin',(155.1,5.2,48.5));
#87713=CARTESIAN_POINT('',(155.1,5.2,48.5));
#87714=CARTESIAN_POINT('',(154.9,5.2,48.5));
#87715=CARTESIAN_POINT('',(77.55,5.2,48.5));
#87716=CARTESIAN_POINT('',(155.1,5.2,48.35));
#87717=CARTESIAN_POINT('',(155.1,5.2,48.5));
#87718=CARTESIAN_POINT('',(154.9,5.2,48.35));
#87719=CARTESIAN_POINT('',(154.9,5.2,48.35));
#87720=CARTESIAN_POINT('',(154.9,5.2,48.5));
#87721=CARTESIAN_POINT('Origin',(155.1,7.4,48.5));
#87722=CARTESIAN_POINT('',(155.1,7.4,48.5));
#87723=CARTESIAN_POINT('',(155.1,7.7,48.5));
#87724=CARTESIAN_POINT('',(155.1,7.4,48.35));
#87725=CARTESIAN_POINT('',(155.1,7.4,48.5));
#87726=CARTESIAN_POINT('',(155.1,5.2,48.35));
#87727=CARTESIAN_POINT('Origin',(154.9,7.4,48.5));
#87728=CARTESIAN_POINT('',(154.9,7.4,48.5));
#87729=CARTESIAN_POINT('',(77.45,7.4,48.5));
#87730=CARTESIAN_POINT('',(154.9,7.4,48.35));
#87731=CARTESIAN_POINT('',(154.9,7.4,48.5));
#87732=CARTESIAN_POINT('',(155.1,7.4,48.35));
#87733=CARTESIAN_POINT('Origin',(154.9,5.2,48.5));
#87734=CARTESIAN_POINT('',(154.9,6.6,48.5));
#87735=CARTESIAN_POINT('',(154.9,7.4,48.35));
#87736=CARTESIAN_POINT('Origin',(155.,6.3,48.35));
#87737=CARTESIAN_POINT('Origin',(153.1,6.,48.5));
#87738=CARTESIAN_POINT('',(153.1,6.,48.5));
#87739=CARTESIAN_POINT('',(152.9,6.,48.5));
#87740=CARTESIAN_POINT('',(76.55,6.,48.5));
#87741=CARTESIAN_POINT('',(153.1,6.,48.35));
#87742=CARTESIAN_POINT('',(153.1,6.,48.5));
#87743=CARTESIAN_POINT('',(152.9,6.,48.35));
#87744=CARTESIAN_POINT('',(152.9,6.,48.35));
#87745=CARTESIAN_POINT('',(152.9,6.,48.5));
#87746=CARTESIAN_POINT('Origin',(153.1,7.4,48.5));
#87747=CARTESIAN_POINT('',(153.1,7.4,48.5));
#87748=CARTESIAN_POINT('',(153.1,7.7,48.5));
#87749=CARTESIAN_POINT('',(153.1,7.4,48.35));
#87750=CARTESIAN_POINT('',(153.1,7.4,48.5));
#87751=CARTESIAN_POINT('',(153.1,6.,48.35));
#87752=CARTESIAN_POINT('Origin',(152.9,7.4,48.5));
#87753=CARTESIAN_POINT('',(152.9,7.4,48.5));
#87754=CARTESIAN_POINT('',(76.45,7.4,48.5));
#87755=CARTESIAN_POINT('',(152.9,7.4,48.35));
#87756=CARTESIAN_POINT('',(152.9,7.4,48.5));
#87757=CARTESIAN_POINT('',(153.1,7.4,48.35));
#87758=CARTESIAN_POINT('Origin',(152.9,6.,48.5));
#87759=CARTESIAN_POINT('',(152.9,7.,48.5));
#87760=CARTESIAN_POINT('',(152.9,7.4,48.35));
#87761=CARTESIAN_POINT('Origin',(153.,6.7,48.35));
#87762=CARTESIAN_POINT('Origin',(151.1,6.,48.5));
#87763=CARTESIAN_POINT('',(151.1,6.,48.5));
#87764=CARTESIAN_POINT('',(150.9,6.,48.5));
#87765=CARTESIAN_POINT('',(75.55,6.,48.5));
#87766=CARTESIAN_POINT('',(151.1,6.,48.35));
#87767=CARTESIAN_POINT('',(151.1,6.,48.5));
#87768=CARTESIAN_POINT('',(150.9,6.,48.35));
#87769=CARTESIAN_POINT('',(150.9,6.,48.35));
#87770=CARTESIAN_POINT('',(150.9,6.,48.5));
#87771=CARTESIAN_POINT('Origin',(151.1,7.4,48.5));
#87772=CARTESIAN_POINT('',(151.1,7.4,48.5));
#87773=CARTESIAN_POINT('',(151.1,7.7,48.5));
#87774=CARTESIAN_POINT('',(151.1,7.4,48.35));
#87775=CARTESIAN_POINT('',(151.1,7.4,48.5));
#87776=CARTESIAN_POINT('',(151.1,6.,48.35));
#87777=CARTESIAN_POINT('Origin',(150.9,7.4,48.5));
#87778=CARTESIAN_POINT('',(150.9,7.4,48.5));
#87779=CARTESIAN_POINT('',(75.45,7.4,48.5));
#87780=CARTESIAN_POINT('',(150.9,7.4,48.35));
#87781=CARTESIAN_POINT('',(150.9,7.4,48.5));
#87782=CARTESIAN_POINT('',(151.1,7.4,48.35));
#87783=CARTESIAN_POINT('Origin',(150.9,6.,48.5));
#87784=CARTESIAN_POINT('',(150.9,7.,48.5));
#87785=CARTESIAN_POINT('',(150.9,7.4,48.35));
#87786=CARTESIAN_POINT('Origin',(151.,6.7,48.35));
#87787=CARTESIAN_POINT('Origin',(149.1,6.,48.5));
#87788=CARTESIAN_POINT('',(149.1,6.,48.5));
#87789=CARTESIAN_POINT('',(148.9,6.,48.5));
#87790=CARTESIAN_POINT('',(74.55,6.,48.5));
#87791=CARTESIAN_POINT('',(149.1,6.,48.35));
#87792=CARTESIAN_POINT('',(149.1,6.,48.5));
#87793=CARTESIAN_POINT('',(148.9,6.,48.35));
#87794=CARTESIAN_POINT('',(148.9,6.,48.35));
#87795=CARTESIAN_POINT('',(148.9,6.,48.5));
#87796=CARTESIAN_POINT('Origin',(149.1,7.4,48.5));
#87797=CARTESIAN_POINT('',(149.1,7.4,48.5));
#87798=CARTESIAN_POINT('',(149.1,7.7,48.5));
#87799=CARTESIAN_POINT('',(149.1,7.4,48.35));
#87800=CARTESIAN_POINT('',(149.1,7.4,48.5));
#87801=CARTESIAN_POINT('',(149.1,6.,48.35));
#87802=CARTESIAN_POINT('Origin',(148.9,7.4,48.5));
#87803=CARTESIAN_POINT('',(148.9,7.4,48.5));
#87804=CARTESIAN_POINT('',(74.45,7.4,48.5));
#87805=CARTESIAN_POINT('',(148.9,7.4,48.35));
#87806=CARTESIAN_POINT('',(148.9,7.4,48.5));
#87807=CARTESIAN_POINT('',(149.1,7.4,48.35));
#87808=CARTESIAN_POINT('Origin',(148.9,6.,48.5));
#87809=CARTESIAN_POINT('',(148.9,7.,48.5));
#87810=CARTESIAN_POINT('',(148.9,7.4,48.35));
#87811=CARTESIAN_POINT('Origin',(149.,6.7,48.35));
#87812=CARTESIAN_POINT('Origin',(147.1,6.,48.5));
#87813=CARTESIAN_POINT('',(147.1,6.,48.5));
#87814=CARTESIAN_POINT('',(146.9,6.,48.5));
#87815=CARTESIAN_POINT('',(73.55,6.,48.5));
#87816=CARTESIAN_POINT('',(147.1,6.,48.35));
#87817=CARTESIAN_POINT('',(147.1,6.,48.5));
#87818=CARTESIAN_POINT('',(146.9,6.,48.35));
#87819=CARTESIAN_POINT('',(146.9,6.,48.35));
#87820=CARTESIAN_POINT('',(146.9,6.,48.5));
#87821=CARTESIAN_POINT('Origin',(147.1,7.4,48.5));
#87822=CARTESIAN_POINT('',(147.1,7.4,48.5));
#87823=CARTESIAN_POINT('',(147.1,7.7,48.5));
#87824=CARTESIAN_POINT('',(147.1,7.4,48.35));
#87825=CARTESIAN_POINT('',(147.1,7.4,48.5));
#87826=CARTESIAN_POINT('',(147.1,6.,48.35));
#87827=CARTESIAN_POINT('Origin',(146.9,7.4,48.5));
#87828=CARTESIAN_POINT('',(146.9,7.4,48.5));
#87829=CARTESIAN_POINT('',(73.45,7.4,48.5));
#87830=CARTESIAN_POINT('',(146.9,7.4,48.35));
#87831=CARTESIAN_POINT('',(146.9,7.4,48.5));
#87832=CARTESIAN_POINT('',(147.1,7.4,48.35));
#87833=CARTESIAN_POINT('Origin',(146.9,6.,48.5));
#87834=CARTESIAN_POINT('',(146.9,7.,48.5));
#87835=CARTESIAN_POINT('',(146.9,7.4,48.35));
#87836=CARTESIAN_POINT('Origin',(147.,6.7,48.35));
#87837=CARTESIAN_POINT('Origin',(145.1,5.2,48.5));
#87838=CARTESIAN_POINT('',(145.1,5.2,48.5));
#87839=CARTESIAN_POINT('',(144.9,5.2,48.5));
#87840=CARTESIAN_POINT('',(72.55,5.2,48.5));
#87841=CARTESIAN_POINT('',(145.1,5.2,48.35));
#87842=CARTESIAN_POINT('',(145.1,5.2,48.5));
#87843=CARTESIAN_POINT('',(144.9,5.2,48.35));
#87844=CARTESIAN_POINT('',(144.9,5.2,48.35));
#87845=CARTESIAN_POINT('',(144.9,5.2,48.5));
#87846=CARTESIAN_POINT('Origin',(145.1,7.4,48.5));
#87847=CARTESIAN_POINT('',(145.1,7.4,48.5));
#87848=CARTESIAN_POINT('',(145.1,7.7,48.5));
#87849=CARTESIAN_POINT('',(145.1,7.4,48.35));
#87850=CARTESIAN_POINT('',(145.1,7.4,48.5));
#87851=CARTESIAN_POINT('',(145.1,5.2,48.35));
#87852=CARTESIAN_POINT('Origin',(144.9,7.4,48.5));
#87853=CARTESIAN_POINT('',(144.9,7.4,48.5));
#87854=CARTESIAN_POINT('',(72.45,7.4,48.5));
#87855=CARTESIAN_POINT('',(144.9,7.4,48.35));
#87856=CARTESIAN_POINT('',(144.9,7.4,48.5));
#87857=CARTESIAN_POINT('',(145.1,7.4,48.35));
#87858=CARTESIAN_POINT('Origin',(144.9,5.2,48.5));
#87859=CARTESIAN_POINT('',(144.9,6.6,48.5));
#87860=CARTESIAN_POINT('',(144.9,7.4,48.35));
#87861=CARTESIAN_POINT('Origin',(145.,6.3,48.35));
#87862=CARTESIAN_POINT('Origin',(143.1,6.,48.5));
#87863=CARTESIAN_POINT('',(143.1,6.,48.5));
#87864=CARTESIAN_POINT('',(142.9,6.,48.5));
#87865=CARTESIAN_POINT('',(71.55,6.,48.5));
#87866=CARTESIAN_POINT('',(143.1,6.,48.35));
#87867=CARTESIAN_POINT('',(143.1,6.,48.5));
#87868=CARTESIAN_POINT('',(142.9,6.,48.35));
#87869=CARTESIAN_POINT('',(142.9,6.,48.35));
#87870=CARTESIAN_POINT('',(142.9,6.,48.5));
#87871=CARTESIAN_POINT('Origin',(143.1,7.4,48.5));
#87872=CARTESIAN_POINT('',(143.1,7.4,48.5));
#87873=CARTESIAN_POINT('',(143.1,7.7,48.5));
#87874=CARTESIAN_POINT('',(143.1,7.4,48.35));
#87875=CARTESIAN_POINT('',(143.1,7.4,48.5));
#87876=CARTESIAN_POINT('',(143.1,6.,48.35));
#87877=CARTESIAN_POINT('Origin',(142.9,7.4,48.5));
#87878=CARTESIAN_POINT('',(142.9,7.4,48.5));
#87879=CARTESIAN_POINT('',(71.45,7.4,48.5));
#87880=CARTESIAN_POINT('',(142.9,7.4,48.35));
#87881=CARTESIAN_POINT('',(142.9,7.4,48.5));
#87882=CARTESIAN_POINT('',(143.1,7.4,48.35));
#87883=CARTESIAN_POINT('Origin',(142.9,6.,48.5));
#87884=CARTESIAN_POINT('',(142.9,7.,48.5));
#87885=CARTESIAN_POINT('',(142.9,7.4,48.35));
#87886=CARTESIAN_POINT('Origin',(143.,6.7,48.35));
#87887=CARTESIAN_POINT('Origin',(141.1,6.,48.5));
#87888=CARTESIAN_POINT('',(141.1,6.,48.5));
#87889=CARTESIAN_POINT('',(140.9,6.,48.5));
#87890=CARTESIAN_POINT('',(70.55,6.,48.5));
#87891=CARTESIAN_POINT('',(141.1,6.,48.35));
#87892=CARTESIAN_POINT('',(141.1,6.,48.5));
#87893=CARTESIAN_POINT('',(140.9,6.,48.35));
#87894=CARTESIAN_POINT('',(140.9,6.,48.35));
#87895=CARTESIAN_POINT('',(140.9,6.,48.5));
#87896=CARTESIAN_POINT('Origin',(141.1,7.4,48.5));
#87897=CARTESIAN_POINT('',(141.1,7.4,48.5));
#87898=CARTESIAN_POINT('',(141.1,7.7,48.5));
#87899=CARTESIAN_POINT('',(141.1,7.4,48.35));
#87900=CARTESIAN_POINT('',(141.1,7.4,48.5));
#87901=CARTESIAN_POINT('',(141.1,6.,48.35));
#87902=CARTESIAN_POINT('Origin',(140.9,7.4,48.5));
#87903=CARTESIAN_POINT('',(140.9,7.4,48.5));
#87904=CARTESIAN_POINT('',(70.45,7.4,48.5));
#87905=CARTESIAN_POINT('',(140.9,7.4,48.35));
#87906=CARTESIAN_POINT('',(140.9,7.4,48.5));
#87907=CARTESIAN_POINT('',(141.1,7.4,48.35));
#87908=CARTESIAN_POINT('Origin',(140.9,6.,48.5));
#87909=CARTESIAN_POINT('',(140.9,7.,48.5));
#87910=CARTESIAN_POINT('',(140.9,7.4,48.35));
#87911=CARTESIAN_POINT('Origin',(141.,6.7,48.35));
#87912=CARTESIAN_POINT('Origin',(139.1,6.,48.5));
#87913=CARTESIAN_POINT('',(139.1,6.,48.5));
#87914=CARTESIAN_POINT('',(138.9,6.,48.5));
#87915=CARTESIAN_POINT('',(69.55,6.,48.5));
#87916=CARTESIAN_POINT('',(139.1,6.,48.35));
#87917=CARTESIAN_POINT('',(139.1,6.,48.5));
#87918=CARTESIAN_POINT('',(138.9,6.,48.35));
#87919=CARTESIAN_POINT('',(138.9,6.,48.35));
#87920=CARTESIAN_POINT('',(138.9,6.,48.5));
#87921=CARTESIAN_POINT('Origin',(139.1,7.4,48.5));
#87922=CARTESIAN_POINT('',(139.1,7.4,48.5));
#87923=CARTESIAN_POINT('',(139.1,7.7,48.5));
#87924=CARTESIAN_POINT('',(139.1,7.4,48.35));
#87925=CARTESIAN_POINT('',(139.1,7.4,48.5));
#87926=CARTESIAN_POINT('',(139.1,6.,48.35));
#87927=CARTESIAN_POINT('Origin',(138.9,7.4,48.5));
#87928=CARTESIAN_POINT('',(138.9,7.4,48.5));
#87929=CARTESIAN_POINT('',(69.45,7.4,48.5));
#87930=CARTESIAN_POINT('',(138.9,7.4,48.35));
#87931=CARTESIAN_POINT('',(138.9,7.4,48.5));
#87932=CARTESIAN_POINT('',(139.1,7.4,48.35));
#87933=CARTESIAN_POINT('Origin',(138.9,6.,48.5));
#87934=CARTESIAN_POINT('',(138.9,7.,48.5));
#87935=CARTESIAN_POINT('',(138.9,7.4,48.35));
#87936=CARTESIAN_POINT('Origin',(139.,6.7,48.35));
#87937=CARTESIAN_POINT('Origin',(137.1,6.,48.5));
#87938=CARTESIAN_POINT('',(137.1,6.,48.5));
#87939=CARTESIAN_POINT('',(136.9,6.,48.5));
#87940=CARTESIAN_POINT('',(68.55,6.,48.5));
#87941=CARTESIAN_POINT('',(137.1,6.,48.35));
#87942=CARTESIAN_POINT('',(137.1,6.,48.5));
#87943=CARTESIAN_POINT('',(136.9,6.,48.35));
#87944=CARTESIAN_POINT('',(136.9,6.,48.35));
#87945=CARTESIAN_POINT('',(136.9,6.,48.5));
#87946=CARTESIAN_POINT('Origin',(137.1,7.4,48.5));
#87947=CARTESIAN_POINT('',(137.1,7.4,48.5));
#87948=CARTESIAN_POINT('',(137.1,7.7,48.5));
#87949=CARTESIAN_POINT('',(137.1,7.4,48.35));
#87950=CARTESIAN_POINT('',(137.1,7.4,48.5));
#87951=CARTESIAN_POINT('',(137.1,6.,48.35));
#87952=CARTESIAN_POINT('Origin',(136.9,7.4,48.5));
#87953=CARTESIAN_POINT('',(136.9,7.4,48.5));
#87954=CARTESIAN_POINT('',(68.45,7.4,48.5));
#87955=CARTESIAN_POINT('',(136.9,7.4,48.35));
#87956=CARTESIAN_POINT('',(136.9,7.4,48.5));
#87957=CARTESIAN_POINT('',(137.1,7.4,48.35));
#87958=CARTESIAN_POINT('Origin',(136.9,6.,48.5));
#87959=CARTESIAN_POINT('',(136.9,7.,48.5));
#87960=CARTESIAN_POINT('',(136.9,7.4,48.35));
#87961=CARTESIAN_POINT('Origin',(137.,6.7,48.35));
#87962=CARTESIAN_POINT('Origin',(135.1,5.2,48.5));
#87963=CARTESIAN_POINT('',(135.1,5.2,48.5));
#87964=CARTESIAN_POINT('',(134.9,5.2,48.5));
#87965=CARTESIAN_POINT('',(67.55,5.2,48.5));
#87966=CARTESIAN_POINT('',(135.1,5.2,48.35));
#87967=CARTESIAN_POINT('',(135.1,5.2,48.5));
#87968=CARTESIAN_POINT('',(134.9,5.2,48.35));
#87969=CARTESIAN_POINT('',(134.9,5.2,48.35));
#87970=CARTESIAN_POINT('',(134.9,5.2,48.5));
#87971=CARTESIAN_POINT('Origin',(135.1,7.4,48.5));
#87972=CARTESIAN_POINT('',(135.1,7.4,48.5));
#87973=CARTESIAN_POINT('',(135.1,7.7,48.5));
#87974=CARTESIAN_POINT('',(135.1,7.4,48.35));
#87975=CARTESIAN_POINT('',(135.1,7.4,48.5));
#87976=CARTESIAN_POINT('',(135.1,5.2,48.35));
#87977=CARTESIAN_POINT('Origin',(134.9,7.4,48.5));
#87978=CARTESIAN_POINT('',(134.9,7.4,48.5));
#87979=CARTESIAN_POINT('',(67.45,7.4,48.5));
#87980=CARTESIAN_POINT('',(134.9,7.4,48.35));
#87981=CARTESIAN_POINT('',(134.9,7.4,48.5));
#87982=CARTESIAN_POINT('',(135.1,7.4,48.35));
#87983=CARTESIAN_POINT('Origin',(134.9,5.2,48.5));
#87984=CARTESIAN_POINT('',(134.9,6.6,48.5));
#87985=CARTESIAN_POINT('',(134.9,7.4,48.35));
#87986=CARTESIAN_POINT('Origin',(135.,6.3,48.35));
#87987=CARTESIAN_POINT('Origin',(133.1,6.,48.5));
#87988=CARTESIAN_POINT('',(133.1,6.,48.5));
#87989=CARTESIAN_POINT('',(132.9,6.,48.5));
#87990=CARTESIAN_POINT('',(66.55,6.,48.5));
#87991=CARTESIAN_POINT('',(133.1,6.,48.35));
#87992=CARTESIAN_POINT('',(133.1,6.,48.5));
#87993=CARTESIAN_POINT('',(132.9,6.,48.35));
#87994=CARTESIAN_POINT('',(132.9,6.,48.35));
#87995=CARTESIAN_POINT('',(132.9,6.,48.5));
#87996=CARTESIAN_POINT('Origin',(133.1,7.4,48.5));
#87997=CARTESIAN_POINT('',(133.1,7.4,48.5));
#87998=CARTESIAN_POINT('',(133.1,7.7,48.5));
#87999=CARTESIAN_POINT('',(133.1,7.4,48.35));
#88000=CARTESIAN_POINT('',(133.1,7.4,48.5));
#88001=CARTESIAN_POINT('',(133.1,6.,48.35));
#88002=CARTESIAN_POINT('Origin',(132.9,7.4,48.5));
#88003=CARTESIAN_POINT('',(132.9,7.4,48.5));
#88004=CARTESIAN_POINT('',(66.45,7.4,48.5));
#88005=CARTESIAN_POINT('',(132.9,7.4,48.35));
#88006=CARTESIAN_POINT('',(132.9,7.4,48.5));
#88007=CARTESIAN_POINT('',(133.1,7.4,48.35));
#88008=CARTESIAN_POINT('Origin',(132.9,6.,48.5));
#88009=CARTESIAN_POINT('',(132.9,7.,48.5));
#88010=CARTESIAN_POINT('',(132.9,7.4,48.35));
#88011=CARTESIAN_POINT('Origin',(133.,6.7,48.35));
#88012=CARTESIAN_POINT('Origin',(131.1,6.,48.5));
#88013=CARTESIAN_POINT('',(131.1,6.,48.5));
#88014=CARTESIAN_POINT('',(130.9,6.,48.5));
#88015=CARTESIAN_POINT('',(65.55,6.,48.5));
#88016=CARTESIAN_POINT('',(131.1,6.,48.35));
#88017=CARTESIAN_POINT('',(131.1,6.,48.5));
#88018=CARTESIAN_POINT('',(130.9,6.,48.35));
#88019=CARTESIAN_POINT('',(130.9,6.,48.35));
#88020=CARTESIAN_POINT('',(130.9,6.,48.5));
#88021=CARTESIAN_POINT('Origin',(131.1,7.4,48.5));
#88022=CARTESIAN_POINT('',(131.1,7.4,48.5));
#88023=CARTESIAN_POINT('',(131.1,7.7,48.5));
#88024=CARTESIAN_POINT('',(131.1,7.4,48.35));
#88025=CARTESIAN_POINT('',(131.1,7.4,48.5));
#88026=CARTESIAN_POINT('',(131.1,6.,48.35));
#88027=CARTESIAN_POINT('Origin',(130.9,7.4,48.5));
#88028=CARTESIAN_POINT('',(130.9,7.4,48.5));
#88029=CARTESIAN_POINT('',(65.45,7.4,48.5));
#88030=CARTESIAN_POINT('',(130.9,7.4,48.35));
#88031=CARTESIAN_POINT('',(130.9,7.4,48.5));
#88032=CARTESIAN_POINT('',(131.1,7.4,48.35));
#88033=CARTESIAN_POINT('Origin',(130.9,6.,48.5));
#88034=CARTESIAN_POINT('',(130.9,7.,48.5));
#88035=CARTESIAN_POINT('',(130.9,7.4,48.35));
#88036=CARTESIAN_POINT('Origin',(131.,6.7,48.35));
#88037=CARTESIAN_POINT('Origin',(129.1,6.,48.5));
#88038=CARTESIAN_POINT('',(129.1,6.,48.5));
#88039=CARTESIAN_POINT('',(128.9,6.,48.5));
#88040=CARTESIAN_POINT('',(64.55,6.,48.5));
#88041=CARTESIAN_POINT('',(129.1,6.,48.35));
#88042=CARTESIAN_POINT('',(129.1,6.,48.5));
#88043=CARTESIAN_POINT('',(128.9,6.,48.35));
#88044=CARTESIAN_POINT('',(128.9,6.,48.35));
#88045=CARTESIAN_POINT('',(128.9,6.,48.5));
#88046=CARTESIAN_POINT('Origin',(129.1,7.4,48.5));
#88047=CARTESIAN_POINT('',(129.1,7.4,48.5));
#88048=CARTESIAN_POINT('',(129.1,7.7,48.5));
#88049=CARTESIAN_POINT('',(129.1,7.4,48.35));
#88050=CARTESIAN_POINT('',(129.1,7.4,48.5));
#88051=CARTESIAN_POINT('',(129.1,6.,48.35));
#88052=CARTESIAN_POINT('Origin',(128.9,7.4,48.5));
#88053=CARTESIAN_POINT('',(128.9,7.4,48.5));
#88054=CARTESIAN_POINT('',(64.45,7.4,48.5));
#88055=CARTESIAN_POINT('',(128.9,7.4,48.35));
#88056=CARTESIAN_POINT('',(128.9,7.4,48.5));
#88057=CARTESIAN_POINT('',(129.1,7.4,48.35));
#88058=CARTESIAN_POINT('Origin',(128.9,6.,48.5));
#88059=CARTESIAN_POINT('',(128.9,7.,48.5));
#88060=CARTESIAN_POINT('',(128.9,7.4,48.35));
#88061=CARTESIAN_POINT('Origin',(129.,6.7,48.35));
#88062=CARTESIAN_POINT('Origin',(127.1,6.,48.5));
#88063=CARTESIAN_POINT('',(127.1,6.,48.5));
#88064=CARTESIAN_POINT('',(126.9,6.,48.5));
#88065=CARTESIAN_POINT('',(63.55,6.,48.5));
#88066=CARTESIAN_POINT('',(127.1,6.,48.35));
#88067=CARTESIAN_POINT('',(127.1,6.,48.5));
#88068=CARTESIAN_POINT('',(126.9,6.,48.35));
#88069=CARTESIAN_POINT('',(126.9,6.,48.35));
#88070=CARTESIAN_POINT('',(126.9,6.,48.5));
#88071=CARTESIAN_POINT('Origin',(127.1,7.4,48.5));
#88072=CARTESIAN_POINT('',(127.1,7.4,48.5));
#88073=CARTESIAN_POINT('',(127.1,7.7,48.5));
#88074=CARTESIAN_POINT('',(127.1,7.4,48.35));
#88075=CARTESIAN_POINT('',(127.1,7.4,48.5));
#88076=CARTESIAN_POINT('',(127.1,6.,48.35));
#88077=CARTESIAN_POINT('Origin',(126.9,7.4,48.5));
#88078=CARTESIAN_POINT('',(126.9,7.4,48.5));
#88079=CARTESIAN_POINT('',(63.45,7.4,48.5));
#88080=CARTESIAN_POINT('',(126.9,7.4,48.35));
#88081=CARTESIAN_POINT('',(126.9,7.4,48.5));
#88082=CARTESIAN_POINT('',(127.1,7.4,48.35));
#88083=CARTESIAN_POINT('Origin',(126.9,6.,48.5));
#88084=CARTESIAN_POINT('',(126.9,7.,48.5));
#88085=CARTESIAN_POINT('',(126.9,7.4,48.35));
#88086=CARTESIAN_POINT('Origin',(127.,6.7,48.35));
#88087=CARTESIAN_POINT('Origin',(125.1,5.2,48.5));
#88088=CARTESIAN_POINT('',(125.1,5.2,48.5));
#88089=CARTESIAN_POINT('',(124.9,5.2,48.5));
#88090=CARTESIAN_POINT('',(62.55,5.2,48.5));
#88091=CARTESIAN_POINT('',(125.1,5.2,48.35));
#88092=CARTESIAN_POINT('',(125.1,5.2,48.5));
#88093=CARTESIAN_POINT('',(124.9,5.2,48.35));
#88094=CARTESIAN_POINT('',(124.9,5.2,48.35));
#88095=CARTESIAN_POINT('',(124.9,5.2,48.5));
#88096=CARTESIAN_POINT('Origin',(125.1,7.4,48.5));
#88097=CARTESIAN_POINT('',(125.1,7.4,48.5));
#88098=CARTESIAN_POINT('',(125.1,7.7,48.5));
#88099=CARTESIAN_POINT('',(125.1,7.4,48.35));
#88100=CARTESIAN_POINT('',(125.1,7.4,48.5));
#88101=CARTESIAN_POINT('',(125.1,5.2,48.35));
#88102=CARTESIAN_POINT('Origin',(124.9,7.4,48.5));
#88103=CARTESIAN_POINT('',(124.9,7.4,48.5));
#88104=CARTESIAN_POINT('',(62.45,7.4,48.5));
#88105=CARTESIAN_POINT('',(124.9,7.4,48.35));
#88106=CARTESIAN_POINT('',(124.9,7.4,48.5));
#88107=CARTESIAN_POINT('',(125.1,7.4,48.35));
#88108=CARTESIAN_POINT('Origin',(124.9,5.2,48.5));
#88109=CARTESIAN_POINT('',(124.9,6.6,48.5));
#88110=CARTESIAN_POINT('',(124.9,7.4,48.35));
#88111=CARTESIAN_POINT('Origin',(125.,6.3,48.35));
#88112=CARTESIAN_POINT('Origin',(123.1,6.,48.5));
#88113=CARTESIAN_POINT('',(123.1,6.,48.5));
#88114=CARTESIAN_POINT('',(122.9,6.,48.5));
#88115=CARTESIAN_POINT('',(61.55,6.,48.5));
#88116=CARTESIAN_POINT('',(123.1,6.,48.35));
#88117=CARTESIAN_POINT('',(123.1,6.,48.5));
#88118=CARTESIAN_POINT('',(122.9,6.,48.35));
#88119=CARTESIAN_POINT('',(122.9,6.,48.35));
#88120=CARTESIAN_POINT('',(122.9,6.,48.5));
#88121=CARTESIAN_POINT('Origin',(123.1,7.4,48.5));
#88122=CARTESIAN_POINT('',(123.1,7.4,48.5));
#88123=CARTESIAN_POINT('',(123.1,7.7,48.5));
#88124=CARTESIAN_POINT('',(123.1,7.4,48.35));
#88125=CARTESIAN_POINT('',(123.1,7.4,48.5));
#88126=CARTESIAN_POINT('',(123.1,6.,48.35));
#88127=CARTESIAN_POINT('Origin',(122.9,7.4,48.5));
#88128=CARTESIAN_POINT('',(122.9,7.4,48.5));
#88129=CARTESIAN_POINT('',(61.45,7.4,48.5));
#88130=CARTESIAN_POINT('',(122.9,7.4,48.35));
#88131=CARTESIAN_POINT('',(122.9,7.4,48.5));
#88132=CARTESIAN_POINT('',(123.1,7.4,48.35));
#88133=CARTESIAN_POINT('Origin',(122.9,6.,48.5));
#88134=CARTESIAN_POINT('',(122.9,7.,48.5));
#88135=CARTESIAN_POINT('',(122.9,7.4,48.35));
#88136=CARTESIAN_POINT('Origin',(123.,6.7,48.35));
#88137=CARTESIAN_POINT('Origin',(121.1,6.,48.5));
#88138=CARTESIAN_POINT('',(121.1,6.,48.5));
#88139=CARTESIAN_POINT('',(120.9,6.,48.5));
#88140=CARTESIAN_POINT('',(60.55,6.,48.5));
#88141=CARTESIAN_POINT('',(121.1,6.,48.35));
#88142=CARTESIAN_POINT('',(121.1,6.,48.5));
#88143=CARTESIAN_POINT('',(120.9,6.,48.35));
#88144=CARTESIAN_POINT('',(120.9,6.,48.35));
#88145=CARTESIAN_POINT('',(120.9,6.,48.5));
#88146=CARTESIAN_POINT('Origin',(121.1,7.4,48.5));
#88147=CARTESIAN_POINT('',(121.1,7.4,48.5));
#88148=CARTESIAN_POINT('',(121.1,7.7,48.5));
#88149=CARTESIAN_POINT('',(121.1,7.4,48.35));
#88150=CARTESIAN_POINT('',(121.1,7.4,48.5));
#88151=CARTESIAN_POINT('',(121.1,6.,48.35));
#88152=CARTESIAN_POINT('Origin',(120.9,7.4,48.5));
#88153=CARTESIAN_POINT('',(120.9,7.4,48.5));
#88154=CARTESIAN_POINT('',(60.45,7.4,48.5));
#88155=CARTESIAN_POINT('',(120.9,7.4,48.35));
#88156=CARTESIAN_POINT('',(120.9,7.4,48.5));
#88157=CARTESIAN_POINT('',(121.1,7.4,48.35));
#88158=CARTESIAN_POINT('Origin',(120.9,6.,48.5));
#88159=CARTESIAN_POINT('',(120.9,7.,48.5));
#88160=CARTESIAN_POINT('',(120.9,7.4,48.35));
#88161=CARTESIAN_POINT('Origin',(121.,6.7,48.35));
#88162=CARTESIAN_POINT('Origin',(119.1,6.,48.5));
#88163=CARTESIAN_POINT('',(119.1,6.,48.5));
#88164=CARTESIAN_POINT('',(118.9,6.,48.5));
#88165=CARTESIAN_POINT('',(59.55,6.,48.5));
#88166=CARTESIAN_POINT('',(119.1,6.,48.35));
#88167=CARTESIAN_POINT('',(119.1,6.,48.5));
#88168=CARTESIAN_POINT('',(118.9,6.,48.35));
#88169=CARTESIAN_POINT('',(118.9,6.,48.35));
#88170=CARTESIAN_POINT('',(118.9,6.,48.5));
#88171=CARTESIAN_POINT('Origin',(119.1,7.4,48.5));
#88172=CARTESIAN_POINT('',(119.1,7.4,48.5));
#88173=CARTESIAN_POINT('',(119.1,7.7,48.5));
#88174=CARTESIAN_POINT('',(119.1,7.4,48.35));
#88175=CARTESIAN_POINT('',(119.1,7.4,48.5));
#88176=CARTESIAN_POINT('',(119.1,6.,48.35));
#88177=CARTESIAN_POINT('Origin',(118.9,7.4,48.5));
#88178=CARTESIAN_POINT('',(118.9,7.4,48.5));
#88179=CARTESIAN_POINT('',(59.45,7.4,48.5));
#88180=CARTESIAN_POINT('',(118.9,7.4,48.35));
#88181=CARTESIAN_POINT('',(118.9,7.4,48.5));
#88182=CARTESIAN_POINT('',(119.1,7.4,48.35));
#88183=CARTESIAN_POINT('Origin',(118.9,6.,48.5));
#88184=CARTESIAN_POINT('',(118.9,7.,48.5));
#88185=CARTESIAN_POINT('',(118.9,7.4,48.35));
#88186=CARTESIAN_POINT('Origin',(119.,6.7,48.35));
#88187=CARTESIAN_POINT('Origin',(117.1,6.,48.5));
#88188=CARTESIAN_POINT('',(117.1,6.,48.5));
#88189=CARTESIAN_POINT('',(116.9,6.,48.5));
#88190=CARTESIAN_POINT('',(58.55,6.,48.5));
#88191=CARTESIAN_POINT('',(117.1,6.,48.35));
#88192=CARTESIAN_POINT('',(117.1,6.,48.5));
#88193=CARTESIAN_POINT('',(116.9,6.,48.35));
#88194=CARTESIAN_POINT('',(116.9,6.,48.35));
#88195=CARTESIAN_POINT('',(116.9,6.,48.5));
#88196=CARTESIAN_POINT('Origin',(117.1,7.4,48.5));
#88197=CARTESIAN_POINT('',(117.1,7.4,48.5));
#88198=CARTESIAN_POINT('',(117.1,7.7,48.5));
#88199=CARTESIAN_POINT('',(117.1,7.4,48.35));
#88200=CARTESIAN_POINT('',(117.1,7.4,48.5));
#88201=CARTESIAN_POINT('',(117.1,6.,48.35));
#88202=CARTESIAN_POINT('Origin',(116.9,7.4,48.5));
#88203=CARTESIAN_POINT('',(116.9,7.4,48.5));
#88204=CARTESIAN_POINT('',(58.45,7.4,48.5));
#88205=CARTESIAN_POINT('',(116.9,7.4,48.35));
#88206=CARTESIAN_POINT('',(116.9,7.4,48.5));
#88207=CARTESIAN_POINT('',(117.1,7.4,48.35));
#88208=CARTESIAN_POINT('Origin',(116.9,6.,48.5));
#88209=CARTESIAN_POINT('',(116.9,7.,48.5));
#88210=CARTESIAN_POINT('',(116.9,7.4,48.35));
#88211=CARTESIAN_POINT('Origin',(117.,6.7,48.35));
#88212=CARTESIAN_POINT('Origin',(115.1,5.2,48.5));
#88213=CARTESIAN_POINT('',(115.1,5.2,48.5));
#88214=CARTESIAN_POINT('',(114.9,5.2,48.5));
#88215=CARTESIAN_POINT('',(57.55,5.2,48.5));
#88216=CARTESIAN_POINT('',(115.1,5.2,48.35));
#88217=CARTESIAN_POINT('',(115.1,5.2,48.5));
#88218=CARTESIAN_POINT('',(114.9,5.2,48.35));
#88219=CARTESIAN_POINT('',(114.9,5.2,48.35));
#88220=CARTESIAN_POINT('',(114.9,5.2,48.5));
#88221=CARTESIAN_POINT('Origin',(115.1,7.4,48.5));
#88222=CARTESIAN_POINT('',(115.1,7.4,48.5));
#88223=CARTESIAN_POINT('',(115.1,7.7,48.5));
#88224=CARTESIAN_POINT('',(115.1,7.4,48.35));
#88225=CARTESIAN_POINT('',(115.1,7.4,48.5));
#88226=CARTESIAN_POINT('',(115.1,5.2,48.35));
#88227=CARTESIAN_POINT('Origin',(114.9,7.4,48.5));
#88228=CARTESIAN_POINT('',(114.9,7.4,48.5));
#88229=CARTESIAN_POINT('',(57.45,7.4,48.5));
#88230=CARTESIAN_POINT('',(114.9,7.4,48.35));
#88231=CARTESIAN_POINT('',(114.9,7.4,48.5));
#88232=CARTESIAN_POINT('',(115.1,7.4,48.35));
#88233=CARTESIAN_POINT('Origin',(114.9,5.2,48.5));
#88234=CARTESIAN_POINT('',(114.9,6.6,48.5));
#88235=CARTESIAN_POINT('',(114.9,7.4,48.35));
#88236=CARTESIAN_POINT('Origin',(115.,6.3,48.35));
#88237=CARTESIAN_POINT('Origin',(113.1,6.,48.5));
#88238=CARTESIAN_POINT('',(113.1,6.,48.5));
#88239=CARTESIAN_POINT('',(112.9,6.,48.5));
#88240=CARTESIAN_POINT('',(56.55,6.,48.5));
#88241=CARTESIAN_POINT('',(113.1,6.,48.35));
#88242=CARTESIAN_POINT('',(113.1,6.,48.5));
#88243=CARTESIAN_POINT('',(112.9,6.,48.35));
#88244=CARTESIAN_POINT('',(112.9,6.,48.35));
#88245=CARTESIAN_POINT('',(112.9,6.,48.5));
#88246=CARTESIAN_POINT('Origin',(113.1,7.4,48.5));
#88247=CARTESIAN_POINT('',(113.1,7.4,48.5));
#88248=CARTESIAN_POINT('',(113.1,7.7,48.5));
#88249=CARTESIAN_POINT('',(113.1,7.4,48.35));
#88250=CARTESIAN_POINT('',(113.1,7.4,48.5));
#88251=CARTESIAN_POINT('',(113.1,6.,48.35));
#88252=CARTESIAN_POINT('Origin',(112.9,7.4,48.5));
#88253=CARTESIAN_POINT('',(112.9,7.4,48.5));
#88254=CARTESIAN_POINT('',(56.45,7.4,48.5));
#88255=CARTESIAN_POINT('',(112.9,7.4,48.35));
#88256=CARTESIAN_POINT('',(112.9,7.4,48.5));
#88257=CARTESIAN_POINT('',(113.1,7.4,48.35));
#88258=CARTESIAN_POINT('Origin',(112.9,6.,48.5));
#88259=CARTESIAN_POINT('',(112.9,7.,48.5));
#88260=CARTESIAN_POINT('',(112.9,7.4,48.35));
#88261=CARTESIAN_POINT('Origin',(113.,6.7,48.35));
#88262=CARTESIAN_POINT('Origin',(111.1,6.,48.5));
#88263=CARTESIAN_POINT('',(111.1,6.,48.5));
#88264=CARTESIAN_POINT('',(110.9,6.,48.5));
#88265=CARTESIAN_POINT('',(55.55,6.,48.5));
#88266=CARTESIAN_POINT('',(111.1,6.,48.35));
#88267=CARTESIAN_POINT('',(111.1,6.,48.5));
#88268=CARTESIAN_POINT('',(110.9,6.,48.35));
#88269=CARTESIAN_POINT('',(110.9,6.,48.35));
#88270=CARTESIAN_POINT('',(110.9,6.,48.5));
#88271=CARTESIAN_POINT('Origin',(111.1,7.4,48.5));
#88272=CARTESIAN_POINT('',(111.1,7.4,48.5));
#88273=CARTESIAN_POINT('',(111.1,7.7,48.5));
#88274=CARTESIAN_POINT('',(111.1,7.4,48.35));
#88275=CARTESIAN_POINT('',(111.1,7.4,48.5));
#88276=CARTESIAN_POINT('',(111.1,6.,48.35));
#88277=CARTESIAN_POINT('Origin',(110.9,7.4,48.5));
#88278=CARTESIAN_POINT('',(110.9,7.4,48.5));
#88279=CARTESIAN_POINT('',(55.45,7.4,48.5));
#88280=CARTESIAN_POINT('',(110.9,7.4,48.35));
#88281=CARTESIAN_POINT('',(110.9,7.4,48.5));
#88282=CARTESIAN_POINT('',(111.1,7.4,48.35));
#88283=CARTESIAN_POINT('Origin',(110.9,6.,48.5));
#88284=CARTESIAN_POINT('',(110.9,7.,48.5));
#88285=CARTESIAN_POINT('',(110.9,7.4,48.35));
#88286=CARTESIAN_POINT('Origin',(111.,6.7,48.35));
#88287=CARTESIAN_POINT('Origin',(110.1,4.4,48.5));
#88288=CARTESIAN_POINT('',(110.1,4.4,48.5));
#88289=CARTESIAN_POINT('',(109.9,4.4,48.5));
#88290=CARTESIAN_POINT('',(55.05,4.4,48.5));
#88291=CARTESIAN_POINT('',(110.1,4.4,48.35));
#88292=CARTESIAN_POINT('',(110.1,4.4,48.5));
#88293=CARTESIAN_POINT('',(109.9,4.4,48.35));
#88294=CARTESIAN_POINT('',(109.9,4.4,48.35));
#88295=CARTESIAN_POINT('',(109.9,4.4,48.5));
#88296=CARTESIAN_POINT('Origin',(110.1,7.4,48.5));
#88297=CARTESIAN_POINT('',(110.1,7.4,48.5));
#88298=CARTESIAN_POINT('',(110.1,7.7,48.5));
#88299=CARTESIAN_POINT('',(110.1,7.4,48.35));
#88300=CARTESIAN_POINT('',(110.1,7.4,48.5));
#88301=CARTESIAN_POINT('',(110.1,4.4,48.35));
#88302=CARTESIAN_POINT('Origin',(109.9,7.4,48.5));
#88303=CARTESIAN_POINT('',(109.9,7.4,48.5));
#88304=CARTESIAN_POINT('',(54.95,7.4,48.5));
#88305=CARTESIAN_POINT('',(109.9,7.4,48.35));
#88306=CARTESIAN_POINT('',(109.9,7.4,48.5));
#88307=CARTESIAN_POINT('',(110.1,7.4,48.35));
#88308=CARTESIAN_POINT('Origin',(109.9,4.4,48.5));
#88309=CARTESIAN_POINT('',(109.9,6.2,48.5));
#88310=CARTESIAN_POINT('',(109.9,7.4,48.35));
#88311=CARTESIAN_POINT('Origin',(110.,5.9,48.35));
#88312=CARTESIAN_POINT('Origin',(108.1,6.,48.5));
#88313=CARTESIAN_POINT('',(108.1,6.,48.5));
#88314=CARTESIAN_POINT('',(107.9,6.,48.5));
#88315=CARTESIAN_POINT('',(54.05,6.,48.5));
#88316=CARTESIAN_POINT('',(108.1,6.,48.35));
#88317=CARTESIAN_POINT('',(108.1,6.,48.5));
#88318=CARTESIAN_POINT('',(107.9,6.,48.35));
#88319=CARTESIAN_POINT('',(107.9,6.,48.35));
#88320=CARTESIAN_POINT('',(107.9,6.,48.5));
#88321=CARTESIAN_POINT('Origin',(108.1,7.4,48.5));
#88322=CARTESIAN_POINT('',(108.1,7.4,48.5));
#88323=CARTESIAN_POINT('',(108.1,7.7,48.5));
#88324=CARTESIAN_POINT('',(108.1,7.4,48.35));
#88325=CARTESIAN_POINT('',(108.1,7.4,48.5));
#88326=CARTESIAN_POINT('',(108.1,6.,48.35));
#88327=CARTESIAN_POINT('Origin',(107.9,7.4,48.5));
#88328=CARTESIAN_POINT('',(107.9,7.4,48.5));
#88329=CARTESIAN_POINT('',(53.95,7.4,48.5));
#88330=CARTESIAN_POINT('',(107.9,7.4,48.35));
#88331=CARTESIAN_POINT('',(107.9,7.4,48.5));
#88332=CARTESIAN_POINT('',(108.1,7.4,48.35));
#88333=CARTESIAN_POINT('Origin',(107.9,6.,48.5));
#88334=CARTESIAN_POINT('',(107.9,7.,48.5));
#88335=CARTESIAN_POINT('',(107.9,7.4,48.35));
#88336=CARTESIAN_POINT('Origin',(108.,6.7,48.35));
#88337=CARTESIAN_POINT('Origin',(106.1,6.,48.5));
#88338=CARTESIAN_POINT('',(106.1,6.,48.5));
#88339=CARTESIAN_POINT('',(105.9,6.,48.5));
#88340=CARTESIAN_POINT('',(53.05,6.,48.5));
#88341=CARTESIAN_POINT('',(106.1,6.,48.35));
#88342=CARTESIAN_POINT('',(106.1,6.,48.5));
#88343=CARTESIAN_POINT('',(105.9,6.,48.35));
#88344=CARTESIAN_POINT('',(105.9,6.,48.35));
#88345=CARTESIAN_POINT('',(105.9,6.,48.5));
#88346=CARTESIAN_POINT('Origin',(106.1,7.4,48.5));
#88347=CARTESIAN_POINT('',(106.1,7.4,48.5));
#88348=CARTESIAN_POINT('',(106.1,7.7,48.5));
#88349=CARTESIAN_POINT('',(106.1,7.4,48.35));
#88350=CARTESIAN_POINT('',(106.1,7.4,48.5));
#88351=CARTESIAN_POINT('',(106.1,6.,48.35));
#88352=CARTESIAN_POINT('Origin',(105.9,7.4,48.5));
#88353=CARTESIAN_POINT('',(105.9,7.4,48.5));
#88354=CARTESIAN_POINT('',(52.95,7.4,48.5));
#88355=CARTESIAN_POINT('',(105.9,7.4,48.35));
#88356=CARTESIAN_POINT('',(105.9,7.4,48.5));
#88357=CARTESIAN_POINT('',(106.1,7.4,48.35));
#88358=CARTESIAN_POINT('Origin',(105.9,6.,48.5));
#88359=CARTESIAN_POINT('',(105.9,7.,48.5));
#88360=CARTESIAN_POINT('',(105.9,7.4,48.35));
#88361=CARTESIAN_POINT('Origin',(106.,6.7,48.35));
#88362=CARTESIAN_POINT('Origin',(104.1,6.,48.5));
#88363=CARTESIAN_POINT('',(104.1,6.,48.5));
#88364=CARTESIAN_POINT('',(103.9,6.,48.5));
#88365=CARTESIAN_POINT('',(52.05,6.,48.5));
#88366=CARTESIAN_POINT('',(104.1,6.,48.35));
#88367=CARTESIAN_POINT('',(104.1,6.,48.5));
#88368=CARTESIAN_POINT('',(103.9,6.,48.35));
#88369=CARTESIAN_POINT('',(103.9,6.,48.35));
#88370=CARTESIAN_POINT('',(103.9,6.,48.5));
#88371=CARTESIAN_POINT('Origin',(104.1,7.4,48.5));
#88372=CARTESIAN_POINT('',(104.1,7.4,48.5));
#88373=CARTESIAN_POINT('',(104.1,7.7,48.5));
#88374=CARTESIAN_POINT('',(104.1,7.4,48.35));
#88375=CARTESIAN_POINT('',(104.1,7.4,48.5));
#88376=CARTESIAN_POINT('',(104.1,6.,48.35));
#88377=CARTESIAN_POINT('Origin',(103.9,7.4,48.5));
#88378=CARTESIAN_POINT('',(103.9,7.4,48.5));
#88379=CARTESIAN_POINT('',(51.95,7.4,48.5));
#88380=CARTESIAN_POINT('',(103.9,7.4,48.35));
#88381=CARTESIAN_POINT('',(103.9,7.4,48.5));
#88382=CARTESIAN_POINT('',(104.1,7.4,48.35));
#88383=CARTESIAN_POINT('Origin',(103.9,6.,48.5));
#88384=CARTESIAN_POINT('',(103.9,7.,48.5));
#88385=CARTESIAN_POINT('',(103.9,7.4,48.35));
#88386=CARTESIAN_POINT('Origin',(104.,6.7,48.35));
#88387=CARTESIAN_POINT('Origin',(102.1,6.,48.5));
#88388=CARTESIAN_POINT('',(102.1,6.,48.5));
#88389=CARTESIAN_POINT('',(101.9,6.,48.5));
#88390=CARTESIAN_POINT('',(51.05,6.,48.5));
#88391=CARTESIAN_POINT('',(102.1,6.,48.35));
#88392=CARTESIAN_POINT('',(102.1,6.,48.5));
#88393=CARTESIAN_POINT('',(101.9,6.,48.35));
#88394=CARTESIAN_POINT('',(101.9,6.,48.35));
#88395=CARTESIAN_POINT('',(101.9,6.,48.5));
#88396=CARTESIAN_POINT('Origin',(102.1,7.4,48.5));
#88397=CARTESIAN_POINT('',(102.1,7.4,48.5));
#88398=CARTESIAN_POINT('',(102.1,7.7,48.5));
#88399=CARTESIAN_POINT('',(102.1,7.4,48.35));
#88400=CARTESIAN_POINT('',(102.1,7.4,48.5));
#88401=CARTESIAN_POINT('',(102.1,6.,48.35));
#88402=CARTESIAN_POINT('Origin',(101.9,7.4,48.5));
#88403=CARTESIAN_POINT('',(101.9,7.4,48.5));
#88404=CARTESIAN_POINT('',(50.95,7.4,48.5));
#88405=CARTESIAN_POINT('',(101.9,7.4,48.35));
#88406=CARTESIAN_POINT('',(101.9,7.4,48.5));
#88407=CARTESIAN_POINT('',(102.1,7.4,48.35));
#88408=CARTESIAN_POINT('Origin',(101.9,6.,48.5));
#88409=CARTESIAN_POINT('',(101.9,7.,48.5));
#88410=CARTESIAN_POINT('',(101.9,7.4,48.35));
#88411=CARTESIAN_POINT('Origin',(102.,6.7,48.35));
#88412=CARTESIAN_POINT('Origin',(100.1,4.4,48.5));
#88413=CARTESIAN_POINT('',(100.1,4.4,48.5));
#88414=CARTESIAN_POINT('',(99.9,4.4,48.5));
#88415=CARTESIAN_POINT('',(50.05,4.4,48.5));
#88416=CARTESIAN_POINT('',(100.1,4.4,48.35));
#88417=CARTESIAN_POINT('',(100.1,4.4,48.5));
#88418=CARTESIAN_POINT('',(99.9,4.4,48.35));
#88419=CARTESIAN_POINT('',(99.9,4.4,48.35));
#88420=CARTESIAN_POINT('',(99.9,4.4,48.5));
#88421=CARTESIAN_POINT('Origin',(100.1,7.4,48.5));
#88422=CARTESIAN_POINT('',(100.1,7.4,48.5));
#88423=CARTESIAN_POINT('',(100.1,7.7,48.5));
#88424=CARTESIAN_POINT('',(100.1,7.4,48.35));
#88425=CARTESIAN_POINT('',(100.1,7.4,48.5));
#88426=CARTESIAN_POINT('',(100.1,4.4,48.35));
#88427=CARTESIAN_POINT('Origin',(99.9,7.4,48.5));
#88428=CARTESIAN_POINT('',(99.9,7.4,48.5));
#88429=CARTESIAN_POINT('',(49.95,7.4,48.5));
#88430=CARTESIAN_POINT('',(99.9,7.4,48.35));
#88431=CARTESIAN_POINT('',(99.9,7.4,48.5));
#88432=CARTESIAN_POINT('',(100.1,7.4,48.35));
#88433=CARTESIAN_POINT('Origin',(99.9,4.4,48.5));
#88434=CARTESIAN_POINT('',(99.9,6.2,48.5));
#88435=CARTESIAN_POINT('',(99.9,7.4,48.35));
#88436=CARTESIAN_POINT('Origin',(100.,5.9,48.35));
#88437=CARTESIAN_POINT('Origin',(98.1,6.,48.5));
#88438=CARTESIAN_POINT('',(98.1,6.,48.5));
#88439=CARTESIAN_POINT('',(97.9,6.,48.5));
#88440=CARTESIAN_POINT('',(49.05,6.,48.5));
#88441=CARTESIAN_POINT('',(98.1,6.,48.35));
#88442=CARTESIAN_POINT('',(98.1,6.,48.5));
#88443=CARTESIAN_POINT('',(97.9,6.,48.35));
#88444=CARTESIAN_POINT('',(97.9,6.,48.35));
#88445=CARTESIAN_POINT('',(97.9,6.,48.5));
#88446=CARTESIAN_POINT('Origin',(98.1,7.4,48.5));
#88447=CARTESIAN_POINT('',(98.1,7.4,48.5));
#88448=CARTESIAN_POINT('',(98.1,7.7,48.5));
#88449=CARTESIAN_POINT('',(98.1,7.4,48.35));
#88450=CARTESIAN_POINT('',(98.1,7.4,48.5));
#88451=CARTESIAN_POINT('',(98.1,6.,48.35));
#88452=CARTESIAN_POINT('Origin',(97.9,7.4,48.5));
#88453=CARTESIAN_POINT('',(97.9,7.4,48.5));
#88454=CARTESIAN_POINT('',(48.95,7.4,48.5));
#88455=CARTESIAN_POINT('',(97.9,7.4,48.35));
#88456=CARTESIAN_POINT('',(97.9,7.4,48.5));
#88457=CARTESIAN_POINT('',(98.1,7.4,48.35));
#88458=CARTESIAN_POINT('Origin',(97.9,6.,48.5));
#88459=CARTESIAN_POINT('',(97.9,7.,48.5));
#88460=CARTESIAN_POINT('',(97.9,7.4,48.35));
#88461=CARTESIAN_POINT('Origin',(98.,6.7,48.35));
#88462=CARTESIAN_POINT('Origin',(96.1,6.,48.5));
#88463=CARTESIAN_POINT('',(96.1,6.,48.5));
#88464=CARTESIAN_POINT('',(95.9,6.,48.5));
#88465=CARTESIAN_POINT('',(48.05,6.,48.5));
#88466=CARTESIAN_POINT('',(96.1,6.,48.35));
#88467=CARTESIAN_POINT('',(96.1,6.,48.5));
#88468=CARTESIAN_POINT('',(95.9,6.,48.35));
#88469=CARTESIAN_POINT('',(95.9,6.,48.35));
#88470=CARTESIAN_POINT('',(95.9,6.,48.5));
#88471=CARTESIAN_POINT('Origin',(96.1,7.4,48.5));
#88472=CARTESIAN_POINT('',(96.1,7.4,48.5));
#88473=CARTESIAN_POINT('',(96.1,7.7,48.5));
#88474=CARTESIAN_POINT('',(96.1,7.4,48.35));
#88475=CARTESIAN_POINT('',(96.1,7.4,48.5));
#88476=CARTESIAN_POINT('',(96.1,6.,48.35));
#88477=CARTESIAN_POINT('Origin',(95.9,7.4,48.5));
#88478=CARTESIAN_POINT('',(95.9,7.4,48.5));
#88479=CARTESIAN_POINT('',(47.95,7.4,48.5));
#88480=CARTESIAN_POINT('',(95.9,7.4,48.35));
#88481=CARTESIAN_POINT('',(95.9,7.4,48.5));
#88482=CARTESIAN_POINT('',(96.1,7.4,48.35));
#88483=CARTESIAN_POINT('Origin',(95.9,6.,48.5));
#88484=CARTESIAN_POINT('',(95.9,7.,48.5));
#88485=CARTESIAN_POINT('',(95.9,7.4,48.35));
#88486=CARTESIAN_POINT('Origin',(96.,6.7,48.35));
#88487=CARTESIAN_POINT('Origin',(94.1,6.,48.5));
#88488=CARTESIAN_POINT('',(94.1,6.,48.5));
#88489=CARTESIAN_POINT('',(93.9,6.,48.5));
#88490=CARTESIAN_POINT('',(47.05,6.,48.5));
#88491=CARTESIAN_POINT('',(94.1,6.,48.35));
#88492=CARTESIAN_POINT('',(94.1,6.,48.5));
#88493=CARTESIAN_POINT('',(93.9,6.,48.35));
#88494=CARTESIAN_POINT('',(93.9,6.,48.35));
#88495=CARTESIAN_POINT('',(93.9,6.,48.5));
#88496=CARTESIAN_POINT('Origin',(94.1,7.4,48.5));
#88497=CARTESIAN_POINT('',(94.1,7.4,48.5));
#88498=CARTESIAN_POINT('',(94.1,7.7,48.5));
#88499=CARTESIAN_POINT('',(94.1,7.4,48.35));
#88500=CARTESIAN_POINT('',(94.1,7.4,48.5));
#88501=CARTESIAN_POINT('',(94.1,6.,48.35));
#88502=CARTESIAN_POINT('Origin',(93.9,7.4,48.5));
#88503=CARTESIAN_POINT('',(93.9,7.4,48.5));
#88504=CARTESIAN_POINT('',(46.95,7.4,48.5));
#88505=CARTESIAN_POINT('',(93.9,7.4,48.35));
#88506=CARTESIAN_POINT('',(93.9,7.4,48.5));
#88507=CARTESIAN_POINT('',(94.1,7.4,48.35));
#88508=CARTESIAN_POINT('Origin',(93.9,6.,48.5));
#88509=CARTESIAN_POINT('',(93.9,7.,48.5));
#88510=CARTESIAN_POINT('',(93.9,7.4,48.35));
#88511=CARTESIAN_POINT('Origin',(94.,6.7,48.35));
#88512=CARTESIAN_POINT('Origin',(92.1,6.,48.5));
#88513=CARTESIAN_POINT('',(92.1,6.,48.5));
#88514=CARTESIAN_POINT('',(91.9,6.,48.5));
#88515=CARTESIAN_POINT('',(46.05,6.,48.5));
#88516=CARTESIAN_POINT('',(92.1,6.,48.35));
#88517=CARTESIAN_POINT('',(92.1,6.,48.5));
#88518=CARTESIAN_POINT('',(91.9,6.,48.35));
#88519=CARTESIAN_POINT('',(91.9,6.,48.35));
#88520=CARTESIAN_POINT('',(91.9,6.,48.5));
#88521=CARTESIAN_POINT('Origin',(92.1,7.4,48.5));
#88522=CARTESIAN_POINT('',(92.1,7.4,48.5));
#88523=CARTESIAN_POINT('',(92.1,7.7,48.5));
#88524=CARTESIAN_POINT('',(92.1,7.4,48.35));
#88525=CARTESIAN_POINT('',(92.1,7.4,48.5));
#88526=CARTESIAN_POINT('',(92.1,6.,48.35));
#88527=CARTESIAN_POINT('Origin',(91.9,7.4,48.5));
#88528=CARTESIAN_POINT('',(91.9,7.4,48.5));
#88529=CARTESIAN_POINT('',(45.95,7.4,48.5));
#88530=CARTESIAN_POINT('',(91.9,7.4,48.35));
#88531=CARTESIAN_POINT('',(91.9,7.4,48.5));
#88532=CARTESIAN_POINT('',(92.1,7.4,48.35));
#88533=CARTESIAN_POINT('Origin',(91.9,6.,48.5));
#88534=CARTESIAN_POINT('',(91.9,7.,48.5));
#88535=CARTESIAN_POINT('',(91.9,7.4,48.35));
#88536=CARTESIAN_POINT('Origin',(92.,6.7,48.35));
#88537=CARTESIAN_POINT('Origin',(90.1,4.4,48.5));
#88538=CARTESIAN_POINT('',(90.1,4.4,48.5));
#88539=CARTESIAN_POINT('',(89.9,4.4,48.5));
#88540=CARTESIAN_POINT('',(45.05,4.4,48.5));
#88541=CARTESIAN_POINT('',(90.1,4.4,48.35));
#88542=CARTESIAN_POINT('',(90.1,4.4,48.5));
#88543=CARTESIAN_POINT('',(89.9,4.4,48.35));
#88544=CARTESIAN_POINT('',(89.9,4.4,48.35));
#88545=CARTESIAN_POINT('',(89.9,4.4,48.5));
#88546=CARTESIAN_POINT('Origin',(90.1,7.4,48.5));
#88547=CARTESIAN_POINT('',(90.1,7.4,48.5));
#88548=CARTESIAN_POINT('',(90.1,7.7,48.5));
#88549=CARTESIAN_POINT('',(90.1,7.4,48.35));
#88550=CARTESIAN_POINT('',(90.1,7.4,48.5));
#88551=CARTESIAN_POINT('',(90.1,4.4,48.35));
#88552=CARTESIAN_POINT('Origin',(89.9,7.4,48.5));
#88553=CARTESIAN_POINT('',(89.9,7.4,48.5));
#88554=CARTESIAN_POINT('',(44.95,7.4,48.5));
#88555=CARTESIAN_POINT('',(89.9,7.4,48.35));
#88556=CARTESIAN_POINT('',(89.9,7.4,48.5));
#88557=CARTESIAN_POINT('',(90.1,7.4,48.35));
#88558=CARTESIAN_POINT('Origin',(89.9,4.4,48.5));
#88559=CARTESIAN_POINT('',(89.9,6.2,48.5));
#88560=CARTESIAN_POINT('',(89.9,7.4,48.35));
#88561=CARTESIAN_POINT('Origin',(90.,5.9,48.35));
#88562=CARTESIAN_POINT('Origin',(88.1,6.,48.5));
#88563=CARTESIAN_POINT('',(88.1,6.,48.5));
#88564=CARTESIAN_POINT('',(87.9,6.,48.5));
#88565=CARTESIAN_POINT('',(44.05,6.,48.5));
#88566=CARTESIAN_POINT('',(88.1,6.,48.35));
#88567=CARTESIAN_POINT('',(88.1,6.,48.5));
#88568=CARTESIAN_POINT('',(87.9,6.,48.35));
#88569=CARTESIAN_POINT('',(87.9,6.,48.35));
#88570=CARTESIAN_POINT('',(87.9,6.,48.5));
#88571=CARTESIAN_POINT('Origin',(88.1,7.4,48.5));
#88572=CARTESIAN_POINT('',(88.1,7.4,48.5));
#88573=CARTESIAN_POINT('',(88.1,7.7,48.5));
#88574=CARTESIAN_POINT('',(88.1,7.4,48.35));
#88575=CARTESIAN_POINT('',(88.1,7.4,48.5));
#88576=CARTESIAN_POINT('',(88.1,6.,48.35));
#88577=CARTESIAN_POINT('Origin',(87.9,7.4,48.5));
#88578=CARTESIAN_POINT('',(87.9,7.4,48.5));
#88579=CARTESIAN_POINT('',(43.95,7.4,48.5));
#88580=CARTESIAN_POINT('',(87.9,7.4,48.35));
#88581=CARTESIAN_POINT('',(87.9,7.4,48.5));
#88582=CARTESIAN_POINT('',(88.1,7.4,48.35));
#88583=CARTESIAN_POINT('Origin',(87.9,6.,48.5));
#88584=CARTESIAN_POINT('',(87.9,7.,48.5));
#88585=CARTESIAN_POINT('',(87.9,7.4,48.35));
#88586=CARTESIAN_POINT('Origin',(88.,6.7,48.35));
#88587=CARTESIAN_POINT('Origin',(86.1,6.,48.5));
#88588=CARTESIAN_POINT('',(86.1,6.,48.5));
#88589=CARTESIAN_POINT('',(85.9,6.,48.5));
#88590=CARTESIAN_POINT('',(43.05,6.,48.5));
#88591=CARTESIAN_POINT('',(86.1,6.,48.35));
#88592=CARTESIAN_POINT('',(86.1,6.,48.5));
#88593=CARTESIAN_POINT('',(85.9,6.,48.35));
#88594=CARTESIAN_POINT('',(85.9,6.,48.35));
#88595=CARTESIAN_POINT('',(85.9,6.,48.5));
#88596=CARTESIAN_POINT('Origin',(86.1,7.4,48.5));
#88597=CARTESIAN_POINT('',(86.1,7.4,48.5));
#88598=CARTESIAN_POINT('',(86.1,7.7,48.5));
#88599=CARTESIAN_POINT('',(86.1,7.4,48.35));
#88600=CARTESIAN_POINT('',(86.1,7.4,48.5));
#88601=CARTESIAN_POINT('',(86.1,6.,48.35));
#88602=CARTESIAN_POINT('Origin',(85.9,7.4,48.5));
#88603=CARTESIAN_POINT('',(85.9,7.4,48.5));
#88604=CARTESIAN_POINT('',(42.95,7.4,48.5));
#88605=CARTESIAN_POINT('',(85.9,7.4,48.35));
#88606=CARTESIAN_POINT('',(85.9,7.4,48.5));
#88607=CARTESIAN_POINT('',(86.1,7.4,48.35));
#88608=CARTESIAN_POINT('Origin',(85.9,6.,48.5));
#88609=CARTESIAN_POINT('',(85.9,7.,48.5));
#88610=CARTESIAN_POINT('',(85.9,7.4,48.35));
#88611=CARTESIAN_POINT('Origin',(86.,6.7,48.35));
#88612=CARTESIAN_POINT('Origin',(84.1,6.,48.5));
#88613=CARTESIAN_POINT('',(84.1,6.,48.5));
#88614=CARTESIAN_POINT('',(83.9,6.,48.5));
#88615=CARTESIAN_POINT('',(42.05,6.,48.5));
#88616=CARTESIAN_POINT('',(84.1,6.,48.35));
#88617=CARTESIAN_POINT('',(84.1,6.,48.5));
#88618=CARTESIAN_POINT('',(83.9,6.,48.35));
#88619=CARTESIAN_POINT('',(83.9,6.,48.35));
#88620=CARTESIAN_POINT('',(83.9,6.,48.5));
#88621=CARTESIAN_POINT('Origin',(84.1,7.4,48.5));
#88622=CARTESIAN_POINT('',(84.1,7.4,48.5));
#88623=CARTESIAN_POINT('',(84.1,7.7,48.5));
#88624=CARTESIAN_POINT('',(84.1,7.4,48.35));
#88625=CARTESIAN_POINT('',(84.1,7.4,48.5));
#88626=CARTESIAN_POINT('',(84.1,6.,48.35));
#88627=CARTESIAN_POINT('Origin',(83.9,7.4,48.5));
#88628=CARTESIAN_POINT('',(83.9,7.4,48.5));
#88629=CARTESIAN_POINT('',(41.95,7.4,48.5));
#88630=CARTESIAN_POINT('',(83.9,7.4,48.35));
#88631=CARTESIAN_POINT('',(83.9,7.4,48.5));
#88632=CARTESIAN_POINT('',(84.1,7.4,48.35));
#88633=CARTESIAN_POINT('Origin',(83.9,6.,48.5));
#88634=CARTESIAN_POINT('',(83.9,7.,48.5));
#88635=CARTESIAN_POINT('',(83.9,7.4,48.35));
#88636=CARTESIAN_POINT('Origin',(84.,6.7,48.35));
#88637=CARTESIAN_POINT('Origin',(82.1,6.,48.5));
#88638=CARTESIAN_POINT('',(82.1,6.,48.5));
#88639=CARTESIAN_POINT('',(81.9,6.,48.5));
#88640=CARTESIAN_POINT('',(41.05,6.,48.5));
#88641=CARTESIAN_POINT('',(82.1,6.,48.35));
#88642=CARTESIAN_POINT('',(82.1,6.,48.5));
#88643=CARTESIAN_POINT('',(81.9,6.,48.35));
#88644=CARTESIAN_POINT('',(81.9,6.,48.35));
#88645=CARTESIAN_POINT('',(81.9,6.,48.5));
#88646=CARTESIAN_POINT('Origin',(82.1,7.4,48.5));
#88647=CARTESIAN_POINT('',(82.1,7.4,48.5));
#88648=CARTESIAN_POINT('',(82.1,7.7,48.5));
#88649=CARTESIAN_POINT('',(82.1,7.4,48.35));
#88650=CARTESIAN_POINT('',(82.1,7.4,48.5));
#88651=CARTESIAN_POINT('',(82.1,6.,48.35));
#88652=CARTESIAN_POINT('Origin',(81.9,7.4,48.5));
#88653=CARTESIAN_POINT('',(81.9,7.4,48.5));
#88654=CARTESIAN_POINT('',(40.95,7.4,48.5));
#88655=CARTESIAN_POINT('',(81.9,7.4,48.35));
#88656=CARTESIAN_POINT('',(81.9,7.4,48.5));
#88657=CARTESIAN_POINT('',(82.1,7.4,48.35));
#88658=CARTESIAN_POINT('Origin',(81.9,6.,48.5));
#88659=CARTESIAN_POINT('',(81.9,7.,48.5));
#88660=CARTESIAN_POINT('',(81.9,7.4,48.35));
#88661=CARTESIAN_POINT('Origin',(82.,6.7,48.35));
#88662=CARTESIAN_POINT('Origin',(80.1,4.4,48.5));
#88663=CARTESIAN_POINT('',(80.1,4.4,48.5));
#88664=CARTESIAN_POINT('',(79.9,4.4,48.5));
#88665=CARTESIAN_POINT('',(40.05,4.4,48.5));
#88666=CARTESIAN_POINT('',(80.1,4.4,48.35));
#88667=CARTESIAN_POINT('',(80.1,4.4,48.5));
#88668=CARTESIAN_POINT('',(79.9,4.4,48.35));
#88669=CARTESIAN_POINT('',(79.9,4.4,48.35));
#88670=CARTESIAN_POINT('',(79.9,4.4,48.5));
#88671=CARTESIAN_POINT('Origin',(80.1,7.4,48.5));
#88672=CARTESIAN_POINT('',(80.1,7.4,48.5));
#88673=CARTESIAN_POINT('',(80.1,7.7,48.5));
#88674=CARTESIAN_POINT('',(80.1,7.4,48.35));
#88675=CARTESIAN_POINT('',(80.1,7.4,48.5));
#88676=CARTESIAN_POINT('',(80.1,4.4,48.35));
#88677=CARTESIAN_POINT('Origin',(79.9,7.4,48.5));
#88678=CARTESIAN_POINT('',(79.9,7.4,48.5));
#88679=CARTESIAN_POINT('',(39.95,7.4,48.5));
#88680=CARTESIAN_POINT('',(79.9,7.4,48.35));
#88681=CARTESIAN_POINT('',(79.9,7.4,48.5));
#88682=CARTESIAN_POINT('',(80.1,7.4,48.35));
#88683=CARTESIAN_POINT('Origin',(79.9,4.4,48.5));
#88684=CARTESIAN_POINT('',(79.9,6.2,48.5));
#88685=CARTESIAN_POINT('',(79.9,7.4,48.35));
#88686=CARTESIAN_POINT('Origin',(80.,5.9,48.35));
#88687=CARTESIAN_POINT('Origin',(78.1,6.,48.5));
#88688=CARTESIAN_POINT('',(78.1,6.,48.5));
#88689=CARTESIAN_POINT('',(77.9,6.,48.5));
#88690=CARTESIAN_POINT('',(39.05,6.,48.5));
#88691=CARTESIAN_POINT('',(78.1,6.,48.35));
#88692=CARTESIAN_POINT('',(78.1,6.,48.5));
#88693=CARTESIAN_POINT('',(77.9,6.,48.35));
#88694=CARTESIAN_POINT('',(77.9,6.,48.35));
#88695=CARTESIAN_POINT('',(77.9,6.,48.5));
#88696=CARTESIAN_POINT('Origin',(78.1,7.4,48.5));
#88697=CARTESIAN_POINT('',(78.1,7.4,48.5));
#88698=CARTESIAN_POINT('',(78.1,7.7,48.5));
#88699=CARTESIAN_POINT('',(78.1,7.4,48.35));
#88700=CARTESIAN_POINT('',(78.1,7.4,48.5));
#88701=CARTESIAN_POINT('',(78.1,6.,48.35));
#88702=CARTESIAN_POINT('Origin',(77.9,7.4,48.5));
#88703=CARTESIAN_POINT('',(77.9,7.4,48.5));
#88704=CARTESIAN_POINT('',(38.95,7.4,48.5));
#88705=CARTESIAN_POINT('',(77.9,7.4,48.35));
#88706=CARTESIAN_POINT('',(77.9,7.4,48.5));
#88707=CARTESIAN_POINT('',(78.1,7.4,48.35));
#88708=CARTESIAN_POINT('Origin',(77.9,6.,48.5));
#88709=CARTESIAN_POINT('',(77.9,7.,48.5));
#88710=CARTESIAN_POINT('',(77.9,7.4,48.35));
#88711=CARTESIAN_POINT('Origin',(78.,6.7,48.35));
#88712=CARTESIAN_POINT('Origin',(76.1,6.,48.5));
#88713=CARTESIAN_POINT('',(76.1,6.,48.5));
#88714=CARTESIAN_POINT('',(75.9,6.,48.5));
#88715=CARTESIAN_POINT('',(38.05,6.,48.5));
#88716=CARTESIAN_POINT('',(76.1,6.,48.35));
#88717=CARTESIAN_POINT('',(76.1,6.,48.5));
#88718=CARTESIAN_POINT('',(75.9,6.,48.35));
#88719=CARTESIAN_POINT('',(75.9,6.,48.35));
#88720=CARTESIAN_POINT('',(75.9,6.,48.5));
#88721=CARTESIAN_POINT('Origin',(76.1,7.4,48.5));
#88722=CARTESIAN_POINT('',(76.1,7.4,48.5));
#88723=CARTESIAN_POINT('',(76.1,7.7,48.5));
#88724=CARTESIAN_POINT('',(76.1,7.4,48.35));
#88725=CARTESIAN_POINT('',(76.1,7.4,48.5));
#88726=CARTESIAN_POINT('',(76.1,6.,48.35));
#88727=CARTESIAN_POINT('Origin',(75.9,7.4,48.5));
#88728=CARTESIAN_POINT('',(75.9,7.4,48.5));
#88729=CARTESIAN_POINT('',(37.95,7.4,48.5));
#88730=CARTESIAN_POINT('',(75.9,7.4,48.35));
#88731=CARTESIAN_POINT('',(75.9,7.4,48.5));
#88732=CARTESIAN_POINT('',(76.1,7.4,48.35));
#88733=CARTESIAN_POINT('Origin',(75.9,6.,48.5));
#88734=CARTESIAN_POINT('',(75.9,7.,48.5));
#88735=CARTESIAN_POINT('',(75.9,7.4,48.35));
#88736=CARTESIAN_POINT('Origin',(76.,6.7,48.35));
#88737=CARTESIAN_POINT('Origin',(74.1,6.,48.5));
#88738=CARTESIAN_POINT('',(74.1,6.,48.5));
#88739=CARTESIAN_POINT('',(73.9,6.,48.5));
#88740=CARTESIAN_POINT('',(37.05,6.,48.5));
#88741=CARTESIAN_POINT('',(74.1,6.,48.35));
#88742=CARTESIAN_POINT('',(74.1,6.,48.5));
#88743=CARTESIAN_POINT('',(73.9,6.,48.35));
#88744=CARTESIAN_POINT('',(73.9,6.,48.35));
#88745=CARTESIAN_POINT('',(73.9,6.,48.5));
#88746=CARTESIAN_POINT('Origin',(74.1,7.4,48.5));
#88747=CARTESIAN_POINT('',(74.1,7.4,48.5));
#88748=CARTESIAN_POINT('',(74.1,7.7,48.5));
#88749=CARTESIAN_POINT('',(74.1,7.4,48.35));
#88750=CARTESIAN_POINT('',(74.1,7.4,48.5));
#88751=CARTESIAN_POINT('',(74.1,6.,48.35));
#88752=CARTESIAN_POINT('Origin',(73.9,7.4,48.5));
#88753=CARTESIAN_POINT('',(73.9,7.4,48.5));
#88754=CARTESIAN_POINT('',(36.95,7.4,48.5));
#88755=CARTESIAN_POINT('',(73.9,7.4,48.35));
#88756=CARTESIAN_POINT('',(73.9,7.4,48.5));
#88757=CARTESIAN_POINT('',(74.1,7.4,48.35));
#88758=CARTESIAN_POINT('Origin',(73.9,6.,48.5));
#88759=CARTESIAN_POINT('',(73.9,7.,48.5));
#88760=CARTESIAN_POINT('',(73.9,7.4,48.35));
#88761=CARTESIAN_POINT('Origin',(74.,6.7,48.35));
#88762=CARTESIAN_POINT('Origin',(72.1,6.,48.5));
#88763=CARTESIAN_POINT('',(72.1,6.,48.5));
#88764=CARTESIAN_POINT('',(71.9,6.,48.5));
#88765=CARTESIAN_POINT('',(36.05,6.,48.5));
#88766=CARTESIAN_POINT('',(72.1,6.,48.35));
#88767=CARTESIAN_POINT('',(72.1,6.,48.5));
#88768=CARTESIAN_POINT('',(71.9,6.,48.35));
#88769=CARTESIAN_POINT('',(71.9,6.,48.35));
#88770=CARTESIAN_POINT('',(71.9,6.,48.5));
#88771=CARTESIAN_POINT('Origin',(72.1,7.4,48.5));
#88772=CARTESIAN_POINT('',(72.1,7.4,48.5));
#88773=CARTESIAN_POINT('',(72.1,7.7,48.5));
#88774=CARTESIAN_POINT('',(72.1,7.4,48.35));
#88775=CARTESIAN_POINT('',(72.1,7.4,48.5));
#88776=CARTESIAN_POINT('',(72.1,6.,48.35));
#88777=CARTESIAN_POINT('Origin',(71.9,7.4,48.5));
#88778=CARTESIAN_POINT('',(71.9,7.4,48.5));
#88779=CARTESIAN_POINT('',(35.95,7.4,48.5));
#88780=CARTESIAN_POINT('',(71.9,7.4,48.35));
#88781=CARTESIAN_POINT('',(71.9,7.4,48.5));
#88782=CARTESIAN_POINT('',(72.1,7.4,48.35));
#88783=CARTESIAN_POINT('Origin',(71.9,6.,48.5));
#88784=CARTESIAN_POINT('',(71.9,7.,48.5));
#88785=CARTESIAN_POINT('',(71.9,7.4,48.35));
#88786=CARTESIAN_POINT('Origin',(72.,6.7,48.35));
#88787=CARTESIAN_POINT('Origin',(70.1,4.4,48.5));
#88788=CARTESIAN_POINT('',(70.1,4.4,48.5));
#88789=CARTESIAN_POINT('',(69.9,4.4,48.5));
#88790=CARTESIAN_POINT('',(35.05,4.4,48.5));
#88791=CARTESIAN_POINT('',(70.1,4.4,48.35));
#88792=CARTESIAN_POINT('',(70.1,4.4,48.5));
#88793=CARTESIAN_POINT('',(69.9,4.4,48.35));
#88794=CARTESIAN_POINT('',(69.9,4.4,48.35));
#88795=CARTESIAN_POINT('',(69.9,4.4,48.5));
#88796=CARTESIAN_POINT('Origin',(70.1,7.4,48.5));
#88797=CARTESIAN_POINT('',(70.1,7.4,48.5));
#88798=CARTESIAN_POINT('',(70.1,7.7,48.5));
#88799=CARTESIAN_POINT('',(70.1,7.4,48.35));
#88800=CARTESIAN_POINT('',(70.1,7.4,48.5));
#88801=CARTESIAN_POINT('',(70.1,4.4,48.35));
#88802=CARTESIAN_POINT('Origin',(69.9,7.4,48.5));
#88803=CARTESIAN_POINT('',(69.9,7.4,48.5));
#88804=CARTESIAN_POINT('',(34.95,7.4,48.5));
#88805=CARTESIAN_POINT('',(69.9,7.4,48.35));
#88806=CARTESIAN_POINT('',(69.9,7.4,48.5));
#88807=CARTESIAN_POINT('',(70.1,7.4,48.35));
#88808=CARTESIAN_POINT('Origin',(69.9,4.4,48.5));
#88809=CARTESIAN_POINT('',(69.9,6.2,48.5));
#88810=CARTESIAN_POINT('',(69.9,7.4,48.35));
#88811=CARTESIAN_POINT('Origin',(70.,5.9,48.35));
#88812=CARTESIAN_POINT('Origin',(68.1,6.,48.5));
#88813=CARTESIAN_POINT('',(68.1,6.,48.5));
#88814=CARTESIAN_POINT('',(67.9,6.,48.5));
#88815=CARTESIAN_POINT('',(34.05,6.,48.5));
#88816=CARTESIAN_POINT('',(68.1,6.,48.35));
#88817=CARTESIAN_POINT('',(68.1,6.,48.5));
#88818=CARTESIAN_POINT('',(67.9,6.,48.35));
#88819=CARTESIAN_POINT('',(67.9,6.,48.35));
#88820=CARTESIAN_POINT('',(67.9,6.,48.5));
#88821=CARTESIAN_POINT('Origin',(68.1,7.4,48.5));
#88822=CARTESIAN_POINT('',(68.1,7.4,48.5));
#88823=CARTESIAN_POINT('',(68.1,7.7,48.5));
#88824=CARTESIAN_POINT('',(68.1,7.4,48.35));
#88825=CARTESIAN_POINT('',(68.1,7.4,48.5));
#88826=CARTESIAN_POINT('',(68.1,6.,48.35));
#88827=CARTESIAN_POINT('Origin',(67.9,7.4,48.5));
#88828=CARTESIAN_POINT('',(67.9,7.4,48.5));
#88829=CARTESIAN_POINT('',(33.95,7.4,48.5));
#88830=CARTESIAN_POINT('',(67.9,7.4,48.35));
#88831=CARTESIAN_POINT('',(67.9,7.4,48.5));
#88832=CARTESIAN_POINT('',(68.1,7.4,48.35));
#88833=CARTESIAN_POINT('Origin',(67.9,6.,48.5));
#88834=CARTESIAN_POINT('',(67.9,7.,48.5));
#88835=CARTESIAN_POINT('',(67.9,7.4,48.35));
#88836=CARTESIAN_POINT('Origin',(68.,6.7,48.35));
#88837=CARTESIAN_POINT('Origin',(66.1,6.,48.5));
#88838=CARTESIAN_POINT('',(66.1,6.,48.5));
#88839=CARTESIAN_POINT('',(65.9,6.,48.5));
#88840=CARTESIAN_POINT('',(33.05,6.,48.5));
#88841=CARTESIAN_POINT('',(66.1,6.,48.35));
#88842=CARTESIAN_POINT('',(66.1,6.,48.5));
#88843=CARTESIAN_POINT('',(65.9,6.,48.35));
#88844=CARTESIAN_POINT('',(65.9,6.,48.35));
#88845=CARTESIAN_POINT('',(65.9,6.,48.5));
#88846=CARTESIAN_POINT('Origin',(66.1,7.4,48.5));
#88847=CARTESIAN_POINT('',(66.1,7.4,48.5));
#88848=CARTESIAN_POINT('',(66.1,7.7,48.5));
#88849=CARTESIAN_POINT('',(66.1,7.4,48.35));
#88850=CARTESIAN_POINT('',(66.1,7.4,48.5));
#88851=CARTESIAN_POINT('',(66.1,6.,48.35));
#88852=CARTESIAN_POINT('Origin',(65.9,7.4,48.5));
#88853=CARTESIAN_POINT('',(65.9,7.4,48.5));
#88854=CARTESIAN_POINT('',(32.95,7.4,48.5));
#88855=CARTESIAN_POINT('',(65.9,7.4,48.35));
#88856=CARTESIAN_POINT('',(65.9,7.4,48.5));
#88857=CARTESIAN_POINT('',(66.1,7.4,48.35));
#88858=CARTESIAN_POINT('Origin',(65.9,6.,48.5));
#88859=CARTESIAN_POINT('',(65.9,7.,48.5));
#88860=CARTESIAN_POINT('',(65.9,7.4,48.35));
#88861=CARTESIAN_POINT('Origin',(66.,6.7,48.35));
#88862=CARTESIAN_POINT('Origin',(64.1,6.,48.5));
#88863=CARTESIAN_POINT('',(64.1,6.,48.5));
#88864=CARTESIAN_POINT('',(63.9,6.,48.5));
#88865=CARTESIAN_POINT('',(32.05,6.,48.5));
#88866=CARTESIAN_POINT('',(64.1,6.,48.35));
#88867=CARTESIAN_POINT('',(64.1,6.,48.5));
#88868=CARTESIAN_POINT('',(63.9,6.,48.35));
#88869=CARTESIAN_POINT('',(63.9,6.,48.35));
#88870=CARTESIAN_POINT('',(63.9,6.,48.5));
#88871=CARTESIAN_POINT('Origin',(64.1,7.4,48.5));
#88872=CARTESIAN_POINT('',(64.1,7.4,48.5));
#88873=CARTESIAN_POINT('',(64.1,7.7,48.5));
#88874=CARTESIAN_POINT('',(64.1,7.4,48.35));
#88875=CARTESIAN_POINT('',(64.1,7.4,48.5));
#88876=CARTESIAN_POINT('',(64.1,6.,48.35));
#88877=CARTESIAN_POINT('Origin',(63.9,7.4,48.5));
#88878=CARTESIAN_POINT('',(63.9,7.4,48.5));
#88879=CARTESIAN_POINT('',(31.95,7.4,48.5));
#88880=CARTESIAN_POINT('',(63.9,7.4,48.35));
#88881=CARTESIAN_POINT('',(63.9,7.4,48.5));
#88882=CARTESIAN_POINT('',(64.1,7.4,48.35));
#88883=CARTESIAN_POINT('Origin',(63.9,6.,48.5));
#88884=CARTESIAN_POINT('',(63.9,7.,48.5));
#88885=CARTESIAN_POINT('',(63.9,7.4,48.35));
#88886=CARTESIAN_POINT('Origin',(64.,6.7,48.35));
#88887=CARTESIAN_POINT('Origin',(62.1,6.,48.5));
#88888=CARTESIAN_POINT('',(62.1,6.,48.5));
#88889=CARTESIAN_POINT('',(61.9,6.,48.5));
#88890=CARTESIAN_POINT('',(31.05,6.,48.5));
#88891=CARTESIAN_POINT('',(62.1,6.,48.35));
#88892=CARTESIAN_POINT('',(62.1,6.,48.5));
#88893=CARTESIAN_POINT('',(61.9,6.,48.35));
#88894=CARTESIAN_POINT('',(61.9,6.,48.35));
#88895=CARTESIAN_POINT('',(61.9,6.,48.5));
#88896=CARTESIAN_POINT('Origin',(62.1,7.4,48.5));
#88897=CARTESIAN_POINT('',(62.1,7.4,48.5));
#88898=CARTESIAN_POINT('',(62.1,7.7,48.5));
#88899=CARTESIAN_POINT('',(62.1,7.4,48.35));
#88900=CARTESIAN_POINT('',(62.1,7.4,48.5));
#88901=CARTESIAN_POINT('',(62.1,6.,48.35));
#88902=CARTESIAN_POINT('Origin',(61.9,7.4,48.5));
#88903=CARTESIAN_POINT('',(61.9,7.4,48.5));
#88904=CARTESIAN_POINT('',(30.95,7.4,48.5));
#88905=CARTESIAN_POINT('',(61.9,7.4,48.35));
#88906=CARTESIAN_POINT('',(61.9,7.4,48.5));
#88907=CARTESIAN_POINT('',(62.1,7.4,48.35));
#88908=CARTESIAN_POINT('Origin',(61.9,6.,48.5));
#88909=CARTESIAN_POINT('',(61.9,7.,48.5));
#88910=CARTESIAN_POINT('',(61.9,7.4,48.35));
#88911=CARTESIAN_POINT('Origin',(62.,6.7,48.35));
#88912=CARTESIAN_POINT('Origin',(60.1,4.4,48.5));
#88913=CARTESIAN_POINT('',(60.1,4.4,48.5));
#88914=CARTESIAN_POINT('',(59.9,4.4,48.5));
#88915=CARTESIAN_POINT('',(30.05,4.4,48.5));
#88916=CARTESIAN_POINT('',(60.1,4.4,48.35));
#88917=CARTESIAN_POINT('',(60.1,4.4,48.5));
#88918=CARTESIAN_POINT('',(59.9,4.4,48.35));
#88919=CARTESIAN_POINT('',(59.9,4.4,48.35));
#88920=CARTESIAN_POINT('',(59.9,4.4,48.5));
#88921=CARTESIAN_POINT('Origin',(60.1,7.4,48.5));
#88922=CARTESIAN_POINT('',(60.1,7.4,48.5));
#88923=CARTESIAN_POINT('',(60.1,7.7,48.5));
#88924=CARTESIAN_POINT('',(60.1,7.4,48.35));
#88925=CARTESIAN_POINT('',(60.1,7.4,48.5));
#88926=CARTESIAN_POINT('',(60.1,4.4,48.35));
#88927=CARTESIAN_POINT('Origin',(59.9,7.4,48.5));
#88928=CARTESIAN_POINT('',(59.9,7.4,48.5));
#88929=CARTESIAN_POINT('',(29.95,7.4,48.5));
#88930=CARTESIAN_POINT('',(59.9,7.4,48.35));
#88931=CARTESIAN_POINT('',(59.9,7.4,48.5));
#88932=CARTESIAN_POINT('',(60.1,7.4,48.35));
#88933=CARTESIAN_POINT('Origin',(59.9,4.4,48.5));
#88934=CARTESIAN_POINT('',(59.9,6.2,48.5));
#88935=CARTESIAN_POINT('',(59.9,7.4,48.35));
#88936=CARTESIAN_POINT('Origin',(60.,5.9,48.35));
#88937=CARTESIAN_POINT('Origin',(58.1,6.,48.5));
#88938=CARTESIAN_POINT('',(58.1,6.,48.5));
#88939=CARTESIAN_POINT('',(57.9,6.,48.5));
#88940=CARTESIAN_POINT('',(29.05,6.,48.5));
#88941=CARTESIAN_POINT('',(58.1,6.,48.35));
#88942=CARTESIAN_POINT('',(58.1,6.,48.5));
#88943=CARTESIAN_POINT('',(57.9,6.,48.35));
#88944=CARTESIAN_POINT('',(57.9,6.,48.35));
#88945=CARTESIAN_POINT('',(57.9,6.,48.5));
#88946=CARTESIAN_POINT('Origin',(58.1,7.4,48.5));
#88947=CARTESIAN_POINT('',(58.1,7.4,48.5));
#88948=CARTESIAN_POINT('',(58.1,7.7,48.5));
#88949=CARTESIAN_POINT('',(58.1,7.4,48.35));
#88950=CARTESIAN_POINT('',(58.1,7.4,48.5));
#88951=CARTESIAN_POINT('',(58.1,6.,48.35));
#88952=CARTESIAN_POINT('Origin',(57.9,7.4,48.5));
#88953=CARTESIAN_POINT('',(57.9,7.4,48.5));
#88954=CARTESIAN_POINT('',(28.95,7.4,48.5));
#88955=CARTESIAN_POINT('',(57.9,7.4,48.35));
#88956=CARTESIAN_POINT('',(57.9,7.4,48.5));
#88957=CARTESIAN_POINT('',(58.1,7.4,48.35));
#88958=CARTESIAN_POINT('Origin',(57.9,6.,48.5));
#88959=CARTESIAN_POINT('',(57.9,7.,48.5));
#88960=CARTESIAN_POINT('',(57.9,7.4,48.35));
#88961=CARTESIAN_POINT('Origin',(58.,6.7,48.35));
#88962=CARTESIAN_POINT('Origin',(56.1,6.,48.5));
#88963=CARTESIAN_POINT('',(56.1,6.,48.5));
#88964=CARTESIAN_POINT('',(55.9,6.,48.5));
#88965=CARTESIAN_POINT('',(28.05,6.,48.5));
#88966=CARTESIAN_POINT('',(56.1,6.,48.35));
#88967=CARTESIAN_POINT('',(56.1,6.,48.5));
#88968=CARTESIAN_POINT('',(55.9,6.,48.35));
#88969=CARTESIAN_POINT('',(55.9,6.,48.35));
#88970=CARTESIAN_POINT('',(55.9,6.,48.5));
#88971=CARTESIAN_POINT('Origin',(56.1,7.4,48.5));
#88972=CARTESIAN_POINT('',(56.1,7.4,48.5));
#88973=CARTESIAN_POINT('',(56.1,7.7,48.5));
#88974=CARTESIAN_POINT('',(56.1,7.4,48.35));
#88975=CARTESIAN_POINT('',(56.1,7.4,48.5));
#88976=CARTESIAN_POINT('',(56.1,6.,48.35));
#88977=CARTESIAN_POINT('Origin',(55.9,7.4,48.5));
#88978=CARTESIAN_POINT('',(55.9,7.4,48.5));
#88979=CARTESIAN_POINT('',(27.95,7.4,48.5));
#88980=CARTESIAN_POINT('',(55.9,7.4,48.35));
#88981=CARTESIAN_POINT('',(55.9,7.4,48.5));
#88982=CARTESIAN_POINT('',(56.1,7.4,48.35));
#88983=CARTESIAN_POINT('Origin',(55.9,6.,48.5));
#88984=CARTESIAN_POINT('',(55.9,7.,48.5));
#88985=CARTESIAN_POINT('',(55.9,7.4,48.35));
#88986=CARTESIAN_POINT('Origin',(56.,6.7,48.35));
#88987=CARTESIAN_POINT('Origin',(54.1,6.,48.5));
#88988=CARTESIAN_POINT('',(54.1,6.,48.5));
#88989=CARTESIAN_POINT('',(53.9,6.,48.5));
#88990=CARTESIAN_POINT('',(27.05,6.,48.5));
#88991=CARTESIAN_POINT('',(54.1,6.,48.35));
#88992=CARTESIAN_POINT('',(54.1,6.,48.5));
#88993=CARTESIAN_POINT('',(53.9,6.,48.35));
#88994=CARTESIAN_POINT('',(53.9,6.,48.35));
#88995=CARTESIAN_POINT('',(53.9,6.,48.5));
#88996=CARTESIAN_POINT('Origin',(54.1,7.4,48.5));
#88997=CARTESIAN_POINT('',(54.1,7.4,48.5));
#88998=CARTESIAN_POINT('',(54.1,7.7,48.5));
#88999=CARTESIAN_POINT('',(54.1,7.4,48.35));
#89000=CARTESIAN_POINT('',(54.1,7.4,48.5));
#89001=CARTESIAN_POINT('',(54.1,6.,48.35));
#89002=CARTESIAN_POINT('Origin',(53.9,7.4,48.5));
#89003=CARTESIAN_POINT('',(53.9,7.4,48.5));
#89004=CARTESIAN_POINT('',(26.95,7.4,48.5));
#89005=CARTESIAN_POINT('',(53.9,7.4,48.35));
#89006=CARTESIAN_POINT('',(53.9,7.4,48.5));
#89007=CARTESIAN_POINT('',(54.1,7.4,48.35));
#89008=CARTESIAN_POINT('Origin',(53.9,6.,48.5));
#89009=CARTESIAN_POINT('',(53.9,7.,48.5));
#89010=CARTESIAN_POINT('',(53.9,7.4,48.35));
#89011=CARTESIAN_POINT('Origin',(54.,6.7,48.35));
#89012=CARTESIAN_POINT('Origin',(52.1,6.,48.5));
#89013=CARTESIAN_POINT('',(52.1,6.,48.5));
#89014=CARTESIAN_POINT('',(51.9,6.,48.5));
#89015=CARTESIAN_POINT('',(26.05,6.,48.5));
#89016=CARTESIAN_POINT('',(52.1,6.,48.35));
#89017=CARTESIAN_POINT('',(52.1,6.,48.5));
#89018=CARTESIAN_POINT('',(51.9,6.,48.35));
#89019=CARTESIAN_POINT('',(51.9,6.,48.35));
#89020=CARTESIAN_POINT('',(51.9,6.,48.5));
#89021=CARTESIAN_POINT('Origin',(52.1,7.4,48.5));
#89022=CARTESIAN_POINT('',(52.1,7.4,48.5));
#89023=CARTESIAN_POINT('',(52.1,7.7,48.5));
#89024=CARTESIAN_POINT('',(52.1,7.4,48.35));
#89025=CARTESIAN_POINT('',(52.1,7.4,48.5));
#89026=CARTESIAN_POINT('',(52.1,6.,48.35));
#89027=CARTESIAN_POINT('Origin',(51.9,7.4,48.5));
#89028=CARTESIAN_POINT('',(51.9,7.4,48.5));
#89029=CARTESIAN_POINT('',(25.95,7.4,48.5));
#89030=CARTESIAN_POINT('',(51.9,7.4,48.35));
#89031=CARTESIAN_POINT('',(51.9,7.4,48.5));
#89032=CARTESIAN_POINT('',(52.1,7.4,48.35));
#89033=CARTESIAN_POINT('Origin',(51.9,6.,48.5));
#89034=CARTESIAN_POINT('',(51.9,7.,48.5));
#89035=CARTESIAN_POINT('',(51.9,7.4,48.35));
#89036=CARTESIAN_POINT('Origin',(52.,6.7,48.35));
#89037=CARTESIAN_POINT('Origin',(50.1,4.4,48.5));
#89038=CARTESIAN_POINT('',(50.1,4.4,48.5));
#89039=CARTESIAN_POINT('',(49.9,4.4,48.5));
#89040=CARTESIAN_POINT('',(25.05,4.4,48.5));
#89041=CARTESIAN_POINT('',(50.1,4.4,48.35));
#89042=CARTESIAN_POINT('',(50.1,4.4,48.5));
#89043=CARTESIAN_POINT('',(49.9,4.4,48.35));
#89044=CARTESIAN_POINT('',(49.9,4.4,48.35));
#89045=CARTESIAN_POINT('',(49.9,4.4,48.5));
#89046=CARTESIAN_POINT('Origin',(50.1,7.4,48.5));
#89047=CARTESIAN_POINT('',(50.1,7.4,48.5));
#89048=CARTESIAN_POINT('',(50.1,7.7,48.5));
#89049=CARTESIAN_POINT('',(50.1,7.4,48.35));
#89050=CARTESIAN_POINT('',(50.1,7.4,48.5));
#89051=CARTESIAN_POINT('',(50.1,4.4,48.35));
#89052=CARTESIAN_POINT('Origin',(49.9,7.4,48.5));
#89053=CARTESIAN_POINT('',(49.9,7.4,48.5));
#89054=CARTESIAN_POINT('',(24.95,7.4,48.5));
#89055=CARTESIAN_POINT('',(49.9,7.4,48.35));
#89056=CARTESIAN_POINT('',(49.9,7.4,48.5));
#89057=CARTESIAN_POINT('',(50.1,7.4,48.35));
#89058=CARTESIAN_POINT('Origin',(49.9,4.4,48.5));
#89059=CARTESIAN_POINT('',(49.9,6.2,48.5));
#89060=CARTESIAN_POINT('',(49.9,7.4,48.35));
#89061=CARTESIAN_POINT('Origin',(50.,5.9,48.35));
#89062=CARTESIAN_POINT('Origin',(48.1,6.,48.5));
#89063=CARTESIAN_POINT('',(48.1,6.,48.5));
#89064=CARTESIAN_POINT('',(47.9,6.,48.5));
#89065=CARTESIAN_POINT('',(24.05,6.,48.5));
#89066=CARTESIAN_POINT('',(48.1,6.,48.35));
#89067=CARTESIAN_POINT('',(48.1,6.,48.5));
#89068=CARTESIAN_POINT('',(47.9,6.,48.35));
#89069=CARTESIAN_POINT('',(47.9,6.,48.35));
#89070=CARTESIAN_POINT('',(47.9,6.,48.5));
#89071=CARTESIAN_POINT('Origin',(48.1,7.4,48.5));
#89072=CARTESIAN_POINT('',(48.1,7.4,48.5));
#89073=CARTESIAN_POINT('',(48.1,7.7,48.5));
#89074=CARTESIAN_POINT('',(48.1,7.4,48.35));
#89075=CARTESIAN_POINT('',(48.1,7.4,48.5));
#89076=CARTESIAN_POINT('',(48.1,6.,48.35));
#89077=CARTESIAN_POINT('Origin',(47.9,7.4,48.5));
#89078=CARTESIAN_POINT('',(47.9,7.4,48.5));
#89079=CARTESIAN_POINT('',(23.95,7.4,48.5));
#89080=CARTESIAN_POINT('',(47.9,7.4,48.35));
#89081=CARTESIAN_POINT('',(47.9,7.4,48.5));
#89082=CARTESIAN_POINT('',(48.1,7.4,48.35));
#89083=CARTESIAN_POINT('Origin',(47.9,6.,48.5));
#89084=CARTESIAN_POINT('',(47.9,7.,48.5));
#89085=CARTESIAN_POINT('',(47.9,7.4,48.35));
#89086=CARTESIAN_POINT('Origin',(48.,6.7,48.35));
#89087=CARTESIAN_POINT('Origin',(46.1,6.,48.5));
#89088=CARTESIAN_POINT('',(46.1,6.,48.5));
#89089=CARTESIAN_POINT('',(45.9,6.,48.5));
#89090=CARTESIAN_POINT('',(23.05,6.,48.5));
#89091=CARTESIAN_POINT('',(46.1,6.,48.35));
#89092=CARTESIAN_POINT('',(46.1,6.,48.5));
#89093=CARTESIAN_POINT('',(45.9,6.,48.35));
#89094=CARTESIAN_POINT('',(45.9,6.,48.35));
#89095=CARTESIAN_POINT('',(45.9,6.,48.5));
#89096=CARTESIAN_POINT('Origin',(46.1,7.4,48.5));
#89097=CARTESIAN_POINT('',(46.1,7.4,48.5));
#89098=CARTESIAN_POINT('',(46.1,7.7,48.5));
#89099=CARTESIAN_POINT('',(46.1,7.4,48.35));
#89100=CARTESIAN_POINT('',(46.1,7.4,48.5));
#89101=CARTESIAN_POINT('',(46.1,6.,48.35));
#89102=CARTESIAN_POINT('Origin',(45.9,7.4,48.5));
#89103=CARTESIAN_POINT('',(45.9,7.4,48.5));
#89104=CARTESIAN_POINT('',(22.95,7.4,48.5));
#89105=CARTESIAN_POINT('',(45.9,7.4,48.35));
#89106=CARTESIAN_POINT('',(45.9,7.4,48.5));
#89107=CARTESIAN_POINT('',(46.1,7.4,48.35));
#89108=CARTESIAN_POINT('Origin',(45.9,6.,48.5));
#89109=CARTESIAN_POINT('',(45.9,7.,48.5));
#89110=CARTESIAN_POINT('',(45.9,7.4,48.35));
#89111=CARTESIAN_POINT('Origin',(46.,6.7,48.35));
#89112=CARTESIAN_POINT('Origin',(44.1,6.,48.5));
#89113=CARTESIAN_POINT('',(44.1,6.,48.5));
#89114=CARTESIAN_POINT('',(43.9,6.,48.5));
#89115=CARTESIAN_POINT('',(22.05,6.,48.5));
#89116=CARTESIAN_POINT('',(44.1,6.,48.35));
#89117=CARTESIAN_POINT('',(44.1,6.,48.5));
#89118=CARTESIAN_POINT('',(43.9,6.,48.35));
#89119=CARTESIAN_POINT('',(43.9,6.,48.35));
#89120=CARTESIAN_POINT('',(43.9,6.,48.5));
#89121=CARTESIAN_POINT('Origin',(44.1,7.4,48.5));
#89122=CARTESIAN_POINT('',(44.1,7.4,48.5));
#89123=CARTESIAN_POINT('',(44.1,7.7,48.5));
#89124=CARTESIAN_POINT('',(44.1,7.4,48.35));
#89125=CARTESIAN_POINT('',(44.1,7.4,48.5));
#89126=CARTESIAN_POINT('',(44.1,6.,48.35));
#89127=CARTESIAN_POINT('Origin',(43.9,7.4,48.5));
#89128=CARTESIAN_POINT('',(43.9,7.4,48.5));
#89129=CARTESIAN_POINT('',(21.95,7.4,48.5));
#89130=CARTESIAN_POINT('',(43.9,7.4,48.35));
#89131=CARTESIAN_POINT('',(43.9,7.4,48.5));
#89132=CARTESIAN_POINT('',(44.1,7.4,48.35));
#89133=CARTESIAN_POINT('Origin',(43.9,6.,48.5));
#89134=CARTESIAN_POINT('',(43.9,7.,48.5));
#89135=CARTESIAN_POINT('',(43.9,7.4,48.35));
#89136=CARTESIAN_POINT('Origin',(44.,6.7,48.35));
#89137=CARTESIAN_POINT('Origin',(42.1,6.,48.5));
#89138=CARTESIAN_POINT('',(42.1,6.,48.5));
#89139=CARTESIAN_POINT('',(41.9,6.,48.5));
#89140=CARTESIAN_POINT('',(21.05,6.,48.5));
#89141=CARTESIAN_POINT('',(42.1,6.,48.35));
#89142=CARTESIAN_POINT('',(42.1,6.,48.5));
#89143=CARTESIAN_POINT('',(41.9,6.,48.35));
#89144=CARTESIAN_POINT('',(41.9,6.,48.35));
#89145=CARTESIAN_POINT('',(41.9,6.,48.5));
#89146=CARTESIAN_POINT('Origin',(42.1,7.4,48.5));
#89147=CARTESIAN_POINT('',(42.1,7.4,48.5));
#89148=CARTESIAN_POINT('',(42.1,7.7,48.5));
#89149=CARTESIAN_POINT('',(42.1,7.4,48.35));
#89150=CARTESIAN_POINT('',(42.1,7.4,48.5));
#89151=CARTESIAN_POINT('',(42.1,6.,48.35));
#89152=CARTESIAN_POINT('Origin',(41.9,7.4,48.5));
#89153=CARTESIAN_POINT('',(41.9,7.4,48.5));
#89154=CARTESIAN_POINT('',(20.95,7.4,48.5));
#89155=CARTESIAN_POINT('',(41.9,7.4,48.35));
#89156=CARTESIAN_POINT('',(41.9,7.4,48.5));
#89157=CARTESIAN_POINT('',(42.1,7.4,48.35));
#89158=CARTESIAN_POINT('Origin',(41.9,6.,48.5));
#89159=CARTESIAN_POINT('',(41.9,7.,48.5));
#89160=CARTESIAN_POINT('',(41.9,7.4,48.35));
#89161=CARTESIAN_POINT('Origin',(42.,6.7,48.35));
#89162=CARTESIAN_POINT('Origin',(40.1,4.4,48.5));
#89163=CARTESIAN_POINT('',(40.1,4.4,48.5));
#89164=CARTESIAN_POINT('',(39.9,4.4,48.5));
#89165=CARTESIAN_POINT('',(20.05,4.4,48.5));
#89166=CARTESIAN_POINT('',(40.1,4.4,48.35));
#89167=CARTESIAN_POINT('',(40.1,4.4,48.5));
#89168=CARTESIAN_POINT('',(39.9,4.4,48.35));
#89169=CARTESIAN_POINT('',(39.9,4.4,48.35));
#89170=CARTESIAN_POINT('',(39.9,4.4,48.5));
#89171=CARTESIAN_POINT('Origin',(40.1,7.4,48.5));
#89172=CARTESIAN_POINT('',(40.1,7.4,48.5));
#89173=CARTESIAN_POINT('',(40.1,7.7,48.5));
#89174=CARTESIAN_POINT('',(40.1,7.4,48.35));
#89175=CARTESIAN_POINT('',(40.1,7.4,48.5));
#89176=CARTESIAN_POINT('',(40.1,4.4,48.35));
#89177=CARTESIAN_POINT('Origin',(39.9,7.4,48.5));
#89178=CARTESIAN_POINT('',(39.9,7.4,48.5));
#89179=CARTESIAN_POINT('',(19.95,7.4,48.5));
#89180=CARTESIAN_POINT('',(39.9,7.4,48.35));
#89181=CARTESIAN_POINT('',(39.9,7.4,48.5));
#89182=CARTESIAN_POINT('',(40.1,7.4,48.35));
#89183=CARTESIAN_POINT('Origin',(39.9,4.4,48.5));
#89184=CARTESIAN_POINT('',(39.9,6.2,48.5));
#89185=CARTESIAN_POINT('',(39.9,7.4,48.35));
#89186=CARTESIAN_POINT('Origin',(40.,5.9,48.35));
#89187=CARTESIAN_POINT('Origin',(38.1,6.,48.5));
#89188=CARTESIAN_POINT('',(38.1,6.,48.5));
#89189=CARTESIAN_POINT('',(37.9,6.,48.5));
#89190=CARTESIAN_POINT('',(19.05,6.,48.5));
#89191=CARTESIAN_POINT('',(38.1,6.,48.35));
#89192=CARTESIAN_POINT('',(38.1,6.,48.5));
#89193=CARTESIAN_POINT('',(37.9,6.,48.35));
#89194=CARTESIAN_POINT('',(37.9,6.,48.35));
#89195=CARTESIAN_POINT('',(37.9,6.,48.5));
#89196=CARTESIAN_POINT('Origin',(38.1,7.4,48.5));
#89197=CARTESIAN_POINT('',(38.1,7.4,48.5));
#89198=CARTESIAN_POINT('',(38.1,7.7,48.5));
#89199=CARTESIAN_POINT('',(38.1,7.4,48.35));
#89200=CARTESIAN_POINT('',(38.1,7.4,48.5));
#89201=CARTESIAN_POINT('',(38.1,6.,48.35));
#89202=CARTESIAN_POINT('Origin',(37.9,7.4,48.5));
#89203=CARTESIAN_POINT('',(37.9,7.4,48.5));
#89204=CARTESIAN_POINT('',(18.95,7.4,48.5));
#89205=CARTESIAN_POINT('',(37.9,7.4,48.35));
#89206=CARTESIAN_POINT('',(37.9,7.4,48.5));
#89207=CARTESIAN_POINT('',(38.1,7.4,48.35));
#89208=CARTESIAN_POINT('Origin',(37.9,6.,48.5));
#89209=CARTESIAN_POINT('',(37.9,7.,48.5));
#89210=CARTESIAN_POINT('',(37.9,7.4,48.35));
#89211=CARTESIAN_POINT('Origin',(38.,6.7,48.35));
#89212=CARTESIAN_POINT('Origin',(36.1,6.,48.5));
#89213=CARTESIAN_POINT('',(36.1,6.,48.5));
#89214=CARTESIAN_POINT('',(35.9,6.,48.5));
#89215=CARTESIAN_POINT('',(18.05,6.,48.5));
#89216=CARTESIAN_POINT('',(36.1,6.,48.35));
#89217=CARTESIAN_POINT('',(36.1,6.,48.5));
#89218=CARTESIAN_POINT('',(35.9,6.,48.35));
#89219=CARTESIAN_POINT('',(35.9,6.,48.35));
#89220=CARTESIAN_POINT('',(35.9,6.,48.5));
#89221=CARTESIAN_POINT('Origin',(36.1,7.4,48.5));
#89222=CARTESIAN_POINT('',(36.1,7.4,48.5));
#89223=CARTESIAN_POINT('',(36.1,7.7,48.5));
#89224=CARTESIAN_POINT('',(36.1,7.4,48.35));
#89225=CARTESIAN_POINT('',(36.1,7.4,48.5));
#89226=CARTESIAN_POINT('',(36.1,6.,48.35));
#89227=CARTESIAN_POINT('Origin',(35.9,7.4,48.5));
#89228=CARTESIAN_POINT('',(35.9,7.4,48.5));
#89229=CARTESIAN_POINT('',(17.95,7.4,48.5));
#89230=CARTESIAN_POINT('',(35.9,7.4,48.35));
#89231=CARTESIAN_POINT('',(35.9,7.4,48.5));
#89232=CARTESIAN_POINT('',(36.1,7.4,48.35));
#89233=CARTESIAN_POINT('Origin',(35.9,6.,48.5));
#89234=CARTESIAN_POINT('',(35.9,7.,48.5));
#89235=CARTESIAN_POINT('',(35.9,7.4,48.35));
#89236=CARTESIAN_POINT('Origin',(36.,6.7,48.35));
#89237=CARTESIAN_POINT('Origin',(34.1,6.,48.5));
#89238=CARTESIAN_POINT('',(34.1,6.,48.5));
#89239=CARTESIAN_POINT('',(33.9,6.,48.5));
#89240=CARTESIAN_POINT('',(17.05,6.,48.5));
#89241=CARTESIAN_POINT('',(34.1,6.,48.35));
#89242=CARTESIAN_POINT('',(34.1,6.,48.5));
#89243=CARTESIAN_POINT('',(33.9,6.,48.35));
#89244=CARTESIAN_POINT('',(33.9,6.,48.35));
#89245=CARTESIAN_POINT('',(33.9,6.,48.5));
#89246=CARTESIAN_POINT('Origin',(34.1,7.4,48.5));
#89247=CARTESIAN_POINT('',(34.1,7.4,48.5));
#89248=CARTESIAN_POINT('',(34.1,7.7,48.5));
#89249=CARTESIAN_POINT('',(34.1,7.4,48.35));
#89250=CARTESIAN_POINT('',(34.1,7.4,48.5));
#89251=CARTESIAN_POINT('',(34.1,6.,48.35));
#89252=CARTESIAN_POINT('Origin',(33.9,7.4,48.5));
#89253=CARTESIAN_POINT('',(33.9,7.4,48.5));
#89254=CARTESIAN_POINT('',(16.95,7.4,48.5));
#89255=CARTESIAN_POINT('',(33.9,7.4,48.35));
#89256=CARTESIAN_POINT('',(33.9,7.4,48.5));
#89257=CARTESIAN_POINT('',(34.1,7.4,48.35));
#89258=CARTESIAN_POINT('Origin',(33.9,6.,48.5));
#89259=CARTESIAN_POINT('',(33.9,7.,48.5));
#89260=CARTESIAN_POINT('',(33.9,7.4,48.35));
#89261=CARTESIAN_POINT('Origin',(34.,6.7,48.35));
#89262=CARTESIAN_POINT('Origin',(32.1,6.,48.5));
#89263=CARTESIAN_POINT('',(32.1,6.,48.5));
#89264=CARTESIAN_POINT('',(31.9,6.,48.5));
#89265=CARTESIAN_POINT('',(16.05,6.,48.5));
#89266=CARTESIAN_POINT('',(32.1,6.,48.35));
#89267=CARTESIAN_POINT('',(32.1,6.,48.5));
#89268=CARTESIAN_POINT('',(31.9,6.,48.35));
#89269=CARTESIAN_POINT('',(31.9,6.,48.35));
#89270=CARTESIAN_POINT('',(31.9,6.,48.5));
#89271=CARTESIAN_POINT('Origin',(32.1,7.4,48.5));
#89272=CARTESIAN_POINT('',(32.1,7.4,48.5));
#89273=CARTESIAN_POINT('',(32.1,7.7,48.5));
#89274=CARTESIAN_POINT('',(32.1,7.4,48.35));
#89275=CARTESIAN_POINT('',(32.1,7.4,48.5));
#89276=CARTESIAN_POINT('',(32.1,6.,48.35));
#89277=CARTESIAN_POINT('Origin',(31.9,7.4,48.5));
#89278=CARTESIAN_POINT('',(31.9,7.4,48.5));
#89279=CARTESIAN_POINT('',(15.95,7.4,48.5));
#89280=CARTESIAN_POINT('',(31.9,7.4,48.35));
#89281=CARTESIAN_POINT('',(31.9,7.4,48.5));
#89282=CARTESIAN_POINT('',(32.1,7.4,48.35));
#89283=CARTESIAN_POINT('Origin',(31.9,6.,48.5));
#89284=CARTESIAN_POINT('',(31.9,7.,48.5));
#89285=CARTESIAN_POINT('',(31.9,7.4,48.35));
#89286=CARTESIAN_POINT('Origin',(32.,6.7,48.35));
#89287=CARTESIAN_POINT('Origin',(30.1,4.4,48.5));
#89288=CARTESIAN_POINT('',(30.1,4.4,48.5));
#89289=CARTESIAN_POINT('',(29.9,4.4,48.5));
#89290=CARTESIAN_POINT('',(15.05,4.4,48.5));
#89291=CARTESIAN_POINT('',(30.1,4.4,48.35));
#89292=CARTESIAN_POINT('',(30.1,4.4,48.5));
#89293=CARTESIAN_POINT('',(29.9,4.4,48.35));
#89294=CARTESIAN_POINT('',(29.9,4.4,48.35));
#89295=CARTESIAN_POINT('',(29.9,4.4,48.5));
#89296=CARTESIAN_POINT('Origin',(30.1,7.4,48.5));
#89297=CARTESIAN_POINT('',(30.1,7.4,48.5));
#89298=CARTESIAN_POINT('',(30.1,7.7,48.5));
#89299=CARTESIAN_POINT('',(30.1,7.4,48.35));
#89300=CARTESIAN_POINT('',(30.1,7.4,48.5));
#89301=CARTESIAN_POINT('',(30.1,4.4,48.35));
#89302=CARTESIAN_POINT('Origin',(29.9,7.4,48.5));
#89303=CARTESIAN_POINT('',(29.9,7.4,48.5));
#89304=CARTESIAN_POINT('',(14.95,7.4,48.5));
#89305=CARTESIAN_POINT('',(29.9,7.4,48.35));
#89306=CARTESIAN_POINT('',(29.9,7.4,48.5));
#89307=CARTESIAN_POINT('',(30.1,7.4,48.35));
#89308=CARTESIAN_POINT('Origin',(29.9,4.4,48.5));
#89309=CARTESIAN_POINT('',(29.9,6.2,48.5));
#89310=CARTESIAN_POINT('',(29.9,7.4,48.35));
#89311=CARTESIAN_POINT('Origin',(30.,5.9,48.35));
#89312=CARTESIAN_POINT('Origin',(28.1,6.,48.5));
#89313=CARTESIAN_POINT('',(28.1,6.,48.5));
#89314=CARTESIAN_POINT('',(27.9,6.,48.5));
#89315=CARTESIAN_POINT('',(14.05,6.,48.5));
#89316=CARTESIAN_POINT('',(28.1,6.,48.35));
#89317=CARTESIAN_POINT('',(28.1,6.,48.5));
#89318=CARTESIAN_POINT('',(27.9,6.,48.35));
#89319=CARTESIAN_POINT('',(27.9,6.,48.35));
#89320=CARTESIAN_POINT('',(27.9,6.,48.5));
#89321=CARTESIAN_POINT('Origin',(28.1,7.4,48.5));
#89322=CARTESIAN_POINT('',(28.1,7.4,48.5));
#89323=CARTESIAN_POINT('',(28.1,7.7,48.5));
#89324=CARTESIAN_POINT('',(28.1,7.4,48.35));
#89325=CARTESIAN_POINT('',(28.1,7.4,48.5));
#89326=CARTESIAN_POINT('',(28.1,6.,48.35));
#89327=CARTESIAN_POINT('Origin',(27.9,7.4,48.5));
#89328=CARTESIAN_POINT('',(27.9,7.4,48.5));
#89329=CARTESIAN_POINT('',(13.95,7.4,48.5));
#89330=CARTESIAN_POINT('',(27.9,7.4,48.35));
#89331=CARTESIAN_POINT('',(27.9,7.4,48.5));
#89332=CARTESIAN_POINT('',(28.1,7.4,48.35));
#89333=CARTESIAN_POINT('Origin',(27.9,6.,48.5));
#89334=CARTESIAN_POINT('',(27.9,7.,48.5));
#89335=CARTESIAN_POINT('',(27.9,7.4,48.35));
#89336=CARTESIAN_POINT('Origin',(28.,6.7,48.35));
#89337=CARTESIAN_POINT('Origin',(26.1,6.,48.5));
#89338=CARTESIAN_POINT('',(26.1,6.,48.5));
#89339=CARTESIAN_POINT('',(25.9,6.,48.5));
#89340=CARTESIAN_POINT('',(13.05,6.,48.5));
#89341=CARTESIAN_POINT('',(26.1,6.,48.35));
#89342=CARTESIAN_POINT('',(26.1,6.,48.5));
#89343=CARTESIAN_POINT('',(25.9,6.,48.35));
#89344=CARTESIAN_POINT('',(25.9,6.,48.35));
#89345=CARTESIAN_POINT('',(25.9,6.,48.5));
#89346=CARTESIAN_POINT('Origin',(26.1,7.4,48.5));
#89347=CARTESIAN_POINT('',(26.1,7.4,48.5));
#89348=CARTESIAN_POINT('',(26.1,7.7,48.5));
#89349=CARTESIAN_POINT('',(26.1,7.4,48.35));
#89350=CARTESIAN_POINT('',(26.1,7.4,48.5));
#89351=CARTESIAN_POINT('',(26.1,6.,48.35));
#89352=CARTESIAN_POINT('Origin',(25.9,7.4,48.5));
#89353=CARTESIAN_POINT('',(25.9,7.4,48.5));
#89354=CARTESIAN_POINT('',(12.95,7.4,48.5));
#89355=CARTESIAN_POINT('',(25.9,7.4,48.35));
#89356=CARTESIAN_POINT('',(25.9,7.4,48.5));
#89357=CARTESIAN_POINT('',(26.1,7.4,48.35));
#89358=CARTESIAN_POINT('Origin',(25.9,6.,48.5));
#89359=CARTESIAN_POINT('',(25.9,7.,48.5));
#89360=CARTESIAN_POINT('',(25.9,7.4,48.35));
#89361=CARTESIAN_POINT('Origin',(26.,6.7,48.35));
#89362=CARTESIAN_POINT('Origin',(24.1,6.,48.5));
#89363=CARTESIAN_POINT('',(24.1,6.,48.5));
#89364=CARTESIAN_POINT('',(23.9,6.,48.5));
#89365=CARTESIAN_POINT('',(12.05,6.,48.5));
#89366=CARTESIAN_POINT('',(24.1,6.,48.35));
#89367=CARTESIAN_POINT('',(24.1,6.,48.5));
#89368=CARTESIAN_POINT('',(23.9,6.,48.35));
#89369=CARTESIAN_POINT('',(23.9,6.,48.35));
#89370=CARTESIAN_POINT('',(23.9,6.,48.5));
#89371=CARTESIAN_POINT('Origin',(24.1,7.4,48.5));
#89372=CARTESIAN_POINT('',(24.1,7.4,48.5));
#89373=CARTESIAN_POINT('',(24.1,7.7,48.5));
#89374=CARTESIAN_POINT('',(24.1,7.4,48.35));
#89375=CARTESIAN_POINT('',(24.1,7.4,48.5));
#89376=CARTESIAN_POINT('',(24.1,6.,48.35));
#89377=CARTESIAN_POINT('Origin',(23.9,7.4,48.5));
#89378=CARTESIAN_POINT('',(23.9,7.4,48.5));
#89379=CARTESIAN_POINT('',(11.95,7.4,48.5));
#89380=CARTESIAN_POINT('',(23.9,7.4,48.35));
#89381=CARTESIAN_POINT('',(23.9,7.4,48.5));
#89382=CARTESIAN_POINT('',(24.1,7.4,48.35));
#89383=CARTESIAN_POINT('Origin',(23.9,6.,48.5));
#89384=CARTESIAN_POINT('',(23.9,7.,48.5));
#89385=CARTESIAN_POINT('',(23.9,7.4,48.35));
#89386=CARTESIAN_POINT('Origin',(24.,6.7,48.35));
#89387=CARTESIAN_POINT('Origin',(22.1,6.,48.5));
#89388=CARTESIAN_POINT('',(22.1,6.,48.5));
#89389=CARTESIAN_POINT('',(21.9,6.,48.5));
#89390=CARTESIAN_POINT('',(11.05,6.,48.5));
#89391=CARTESIAN_POINT('',(22.1,6.,48.35));
#89392=CARTESIAN_POINT('',(22.1,6.,48.5));
#89393=CARTESIAN_POINT('',(21.9,6.,48.35));
#89394=CARTESIAN_POINT('',(21.9,6.,48.35));
#89395=CARTESIAN_POINT('',(21.9,6.,48.5));
#89396=CARTESIAN_POINT('Origin',(22.1,7.4,48.5));
#89397=CARTESIAN_POINT('',(22.1,7.4,48.5));
#89398=CARTESIAN_POINT('',(22.1,7.7,48.5));
#89399=CARTESIAN_POINT('',(22.1,7.4,48.35));
#89400=CARTESIAN_POINT('',(22.1,7.4,48.5));
#89401=CARTESIAN_POINT('',(22.1,6.,48.35));
#89402=CARTESIAN_POINT('Origin',(21.9,7.4,48.5));
#89403=CARTESIAN_POINT('',(21.9,7.4,48.5));
#89404=CARTESIAN_POINT('',(10.95,7.4,48.5));
#89405=CARTESIAN_POINT('',(21.9,7.4,48.35));
#89406=CARTESIAN_POINT('',(21.9,7.4,48.5));
#89407=CARTESIAN_POINT('',(22.1,7.4,48.35));
#89408=CARTESIAN_POINT('Origin',(21.9,6.,48.5));
#89409=CARTESIAN_POINT('',(21.9,7.,48.5));
#89410=CARTESIAN_POINT('',(21.9,7.4,48.35));
#89411=CARTESIAN_POINT('Origin',(22.,6.7,48.35));
#89412=CARTESIAN_POINT('Origin',(21.1,6.,48.5));
#89413=CARTESIAN_POINT('',(21.1,6.,48.5));
#89414=CARTESIAN_POINT('',(20.9,6.,48.5));
#89415=CARTESIAN_POINT('',(10.55,6.,48.5));
#89416=CARTESIAN_POINT('',(21.1,6.,48.35));
#89417=CARTESIAN_POINT('',(21.1,6.,48.5));
#89418=CARTESIAN_POINT('',(20.9,6.,48.35));
#89419=CARTESIAN_POINT('',(20.9,6.,48.35));
#89420=CARTESIAN_POINT('',(20.9,6.,48.5));
#89421=CARTESIAN_POINT('Origin',(21.1,7.4,48.5));
#89422=CARTESIAN_POINT('',(21.1,7.4,48.5));
#89423=CARTESIAN_POINT('',(21.1,7.7,48.5));
#89424=CARTESIAN_POINT('',(21.1,7.4,48.35));
#89425=CARTESIAN_POINT('',(21.1,7.4,48.5));
#89426=CARTESIAN_POINT('',(21.1,6.,48.35));
#89427=CARTESIAN_POINT('Origin',(20.9,7.4,48.5));
#89428=CARTESIAN_POINT('',(20.9,7.4,48.5));
#89429=CARTESIAN_POINT('',(10.45,7.4,48.5));
#89430=CARTESIAN_POINT('',(20.9,7.4,48.35));
#89431=CARTESIAN_POINT('',(20.9,7.4,48.5));
#89432=CARTESIAN_POINT('',(21.1,7.4,48.35));
#89433=CARTESIAN_POINT('Origin',(20.9,6.,48.5));
#89434=CARTESIAN_POINT('',(20.9,7.,48.5));
#89435=CARTESIAN_POINT('',(20.9,7.4,48.35));
#89436=CARTESIAN_POINT('Origin',(21.,6.7,48.35));
#89437=CARTESIAN_POINT('Origin',(23.1,6.,48.5));
#89438=CARTESIAN_POINT('',(23.1,6.,48.5));
#89439=CARTESIAN_POINT('',(22.9,6.,48.5));
#89440=CARTESIAN_POINT('',(11.55,6.,48.5));
#89441=CARTESIAN_POINT('',(23.1,6.,48.35));
#89442=CARTESIAN_POINT('',(23.1,6.,48.5));
#89443=CARTESIAN_POINT('',(22.9,6.,48.35));
#89444=CARTESIAN_POINT('',(22.9,6.,48.35));
#89445=CARTESIAN_POINT('',(22.9,6.,48.5));
#89446=CARTESIAN_POINT('Origin',(23.1,7.4,48.5));
#89447=CARTESIAN_POINT('',(23.1,7.4,48.5));
#89448=CARTESIAN_POINT('',(23.1,7.7,48.5));
#89449=CARTESIAN_POINT('',(23.1,7.4,48.35));
#89450=CARTESIAN_POINT('',(23.1,7.4,48.5));
#89451=CARTESIAN_POINT('',(23.1,6.,48.35));
#89452=CARTESIAN_POINT('Origin',(22.9,7.4,48.5));
#89453=CARTESIAN_POINT('',(22.9,7.4,48.5));
#89454=CARTESIAN_POINT('',(11.45,7.4,48.5));
#89455=CARTESIAN_POINT('',(22.9,7.4,48.35));
#89456=CARTESIAN_POINT('',(22.9,7.4,48.5));
#89457=CARTESIAN_POINT('',(23.1,7.4,48.35));
#89458=CARTESIAN_POINT('Origin',(22.9,6.,48.5));
#89459=CARTESIAN_POINT('',(22.9,7.,48.5));
#89460=CARTESIAN_POINT('',(22.9,7.4,48.35));
#89461=CARTESIAN_POINT('Origin',(23.,6.7,48.35));
#89462=CARTESIAN_POINT('Origin',(25.1,5.2,48.5));
#89463=CARTESIAN_POINT('',(25.1,5.2,48.5));
#89464=CARTESIAN_POINT('',(24.9,5.2,48.5));
#89465=CARTESIAN_POINT('',(12.55,5.2,48.5));
#89466=CARTESIAN_POINT('',(25.1,5.2,48.35));
#89467=CARTESIAN_POINT('',(25.1,5.2,48.5));
#89468=CARTESIAN_POINT('',(24.9,5.2,48.35));
#89469=CARTESIAN_POINT('',(24.9,5.2,48.35));
#89470=CARTESIAN_POINT('',(24.9,5.2,48.5));
#89471=CARTESIAN_POINT('Origin',(25.1,7.4,48.5));
#89472=CARTESIAN_POINT('',(25.1,7.4,48.5));
#89473=CARTESIAN_POINT('',(25.1,7.7,48.5));
#89474=CARTESIAN_POINT('',(25.1,7.4,48.35));
#89475=CARTESIAN_POINT('',(25.1,7.4,48.5));
#89476=CARTESIAN_POINT('',(25.1,5.2,48.35));
#89477=CARTESIAN_POINT('Origin',(24.9,7.4,48.5));
#89478=CARTESIAN_POINT('',(24.9,7.4,48.5));
#89479=CARTESIAN_POINT('',(12.45,7.4,48.5));
#89480=CARTESIAN_POINT('',(24.9,7.4,48.35));
#89481=CARTESIAN_POINT('',(24.9,7.4,48.5));
#89482=CARTESIAN_POINT('',(25.1,7.4,48.35));
#89483=CARTESIAN_POINT('Origin',(24.9,5.2,48.5));
#89484=CARTESIAN_POINT('',(24.9,6.6,48.5));
#89485=CARTESIAN_POINT('',(24.9,7.4,48.35));
#89486=CARTESIAN_POINT('Origin',(25.,6.3,48.35));
#89487=CARTESIAN_POINT('Origin',(27.1,6.,48.5));
#89488=CARTESIAN_POINT('',(27.1,6.,48.5));
#89489=CARTESIAN_POINT('',(26.9,6.,48.5));
#89490=CARTESIAN_POINT('',(13.55,6.,48.5));
#89491=CARTESIAN_POINT('',(27.1,6.,48.35));
#89492=CARTESIAN_POINT('',(27.1,6.,48.5));
#89493=CARTESIAN_POINT('',(26.9,6.,48.35));
#89494=CARTESIAN_POINT('',(26.9,6.,48.35));
#89495=CARTESIAN_POINT('',(26.9,6.,48.5));
#89496=CARTESIAN_POINT('Origin',(27.1,7.4,48.5));
#89497=CARTESIAN_POINT('',(27.1,7.4,48.5));
#89498=CARTESIAN_POINT('',(27.1,7.7,48.5));
#89499=CARTESIAN_POINT('',(27.1,7.4,48.35));
#89500=CARTESIAN_POINT('',(27.1,7.4,48.5));
#89501=CARTESIAN_POINT('',(27.1,6.,48.35));
#89502=CARTESIAN_POINT('Origin',(26.9,7.4,48.5));
#89503=CARTESIAN_POINT('',(26.9,7.4,48.5));
#89504=CARTESIAN_POINT('',(13.45,7.4,48.5));
#89505=CARTESIAN_POINT('',(26.9,7.4,48.35));
#89506=CARTESIAN_POINT('',(26.9,7.4,48.5));
#89507=CARTESIAN_POINT('',(27.1,7.4,48.35));
#89508=CARTESIAN_POINT('Origin',(26.9,6.,48.5));
#89509=CARTESIAN_POINT('',(26.9,7.,48.5));
#89510=CARTESIAN_POINT('',(26.9,7.4,48.35));
#89511=CARTESIAN_POINT('Origin',(27.,6.7,48.35));
#89512=CARTESIAN_POINT('Origin',(29.1,6.,48.5));
#89513=CARTESIAN_POINT('',(29.1,6.,48.5));
#89514=CARTESIAN_POINT('',(28.9,6.,48.5));
#89515=CARTESIAN_POINT('',(14.55,6.,48.5));
#89516=CARTESIAN_POINT('',(29.1,6.,48.35));
#89517=CARTESIAN_POINT('',(29.1,6.,48.5));
#89518=CARTESIAN_POINT('',(28.9,6.,48.35));
#89519=CARTESIAN_POINT('',(28.9,6.,48.35));
#89520=CARTESIAN_POINT('',(28.9,6.,48.5));
#89521=CARTESIAN_POINT('Origin',(29.1,7.4,48.5));
#89522=CARTESIAN_POINT('',(29.1,7.4,48.5));
#89523=CARTESIAN_POINT('',(29.1,7.7,48.5));
#89524=CARTESIAN_POINT('',(29.1,7.4,48.35));
#89525=CARTESIAN_POINT('',(29.1,7.4,48.5));
#89526=CARTESIAN_POINT('',(29.1,6.,48.35));
#89527=CARTESIAN_POINT('Origin',(28.9,7.4,48.5));
#89528=CARTESIAN_POINT('',(28.9,7.4,48.5));
#89529=CARTESIAN_POINT('',(14.45,7.4,48.5));
#89530=CARTESIAN_POINT('',(28.9,7.4,48.35));
#89531=CARTESIAN_POINT('',(28.9,7.4,48.5));
#89532=CARTESIAN_POINT('',(29.1,7.4,48.35));
#89533=CARTESIAN_POINT('Origin',(28.9,6.,48.5));
#89534=CARTESIAN_POINT('',(28.9,7.,48.5));
#89535=CARTESIAN_POINT('',(28.9,7.4,48.35));
#89536=CARTESIAN_POINT('Origin',(29.,6.7,48.35));
#89537=CARTESIAN_POINT('Origin',(31.1,6.,48.5));
#89538=CARTESIAN_POINT('',(31.1,6.,48.5));
#89539=CARTESIAN_POINT('',(30.9,6.,48.5));
#89540=CARTESIAN_POINT('',(15.55,6.,48.5));
#89541=CARTESIAN_POINT('',(31.1,6.,48.35));
#89542=CARTESIAN_POINT('',(31.1,6.,48.5));
#89543=CARTESIAN_POINT('',(30.9,6.,48.35));
#89544=CARTESIAN_POINT('',(30.9,6.,48.35));
#89545=CARTESIAN_POINT('',(30.9,6.,48.5));
#89546=CARTESIAN_POINT('Origin',(31.1,7.4,48.5));
#89547=CARTESIAN_POINT('',(31.1,7.4,48.5));
#89548=CARTESIAN_POINT('',(31.1,7.7,48.5));
#89549=CARTESIAN_POINT('',(31.1,7.4,48.35));
#89550=CARTESIAN_POINT('',(31.1,7.4,48.5));
#89551=CARTESIAN_POINT('',(31.1,6.,48.35));
#89552=CARTESIAN_POINT('Origin',(30.9,7.4,48.5));
#89553=CARTESIAN_POINT('',(30.9,7.4,48.5));
#89554=CARTESIAN_POINT('',(15.45,7.4,48.5));
#89555=CARTESIAN_POINT('',(30.9,7.4,48.35));
#89556=CARTESIAN_POINT('',(30.9,7.4,48.5));
#89557=CARTESIAN_POINT('',(31.1,7.4,48.35));
#89558=CARTESIAN_POINT('Origin',(30.9,6.,48.5));
#89559=CARTESIAN_POINT('',(30.9,7.,48.5));
#89560=CARTESIAN_POINT('',(30.9,7.4,48.35));
#89561=CARTESIAN_POINT('Origin',(31.,6.7,48.35));
#89562=CARTESIAN_POINT('Origin',(33.1,6.,48.5));
#89563=CARTESIAN_POINT('',(33.1,6.,48.5));
#89564=CARTESIAN_POINT('',(32.9,6.,48.5));
#89565=CARTESIAN_POINT('',(16.55,6.,48.5));
#89566=CARTESIAN_POINT('',(33.1,6.,48.35));
#89567=CARTESIAN_POINT('',(33.1,6.,48.5));
#89568=CARTESIAN_POINT('',(32.9,6.,48.35));
#89569=CARTESIAN_POINT('',(32.9,6.,48.35));
#89570=CARTESIAN_POINT('',(32.9,6.,48.5));
#89571=CARTESIAN_POINT('Origin',(33.1,7.4,48.5));
#89572=CARTESIAN_POINT('',(33.1,7.4,48.5));
#89573=CARTESIAN_POINT('',(33.1,7.7,48.5));
#89574=CARTESIAN_POINT('',(33.1,7.4,48.35));
#89575=CARTESIAN_POINT('',(33.1,7.4,48.5));
#89576=CARTESIAN_POINT('',(33.1,6.,48.35));
#89577=CARTESIAN_POINT('Origin',(32.9,7.4,48.5));
#89578=CARTESIAN_POINT('',(32.9,7.4,48.5));
#89579=CARTESIAN_POINT('',(16.45,7.4,48.5));
#89580=CARTESIAN_POINT('',(32.9,7.4,48.35));
#89581=CARTESIAN_POINT('',(32.9,7.4,48.5));
#89582=CARTESIAN_POINT('',(33.1,7.4,48.35));
#89583=CARTESIAN_POINT('Origin',(32.9,6.,48.5));
#89584=CARTESIAN_POINT('',(32.9,7.,48.5));
#89585=CARTESIAN_POINT('',(32.9,7.4,48.35));
#89586=CARTESIAN_POINT('Origin',(33.,6.7,48.35));
#89587=CARTESIAN_POINT('Origin',(35.1,5.2,48.5));
#89588=CARTESIAN_POINT('',(35.1,5.2,48.5));
#89589=CARTESIAN_POINT('',(34.9,5.2,48.5));
#89590=CARTESIAN_POINT('',(17.55,5.2,48.5));
#89591=CARTESIAN_POINT('',(35.1,5.2,48.35));
#89592=CARTESIAN_POINT('',(35.1,5.2,48.5));
#89593=CARTESIAN_POINT('',(34.9,5.2,48.35));
#89594=CARTESIAN_POINT('',(34.9,5.2,48.35));
#89595=CARTESIAN_POINT('',(34.9,5.2,48.5));
#89596=CARTESIAN_POINT('Origin',(35.1,7.4,48.5));
#89597=CARTESIAN_POINT('',(35.1,7.4,48.5));
#89598=CARTESIAN_POINT('',(35.1,7.7,48.5));
#89599=CARTESIAN_POINT('',(35.1,7.4,48.35));
#89600=CARTESIAN_POINT('',(35.1,7.4,48.5));
#89601=CARTESIAN_POINT('',(35.1,5.2,48.35));
#89602=CARTESIAN_POINT('Origin',(34.9,7.4,48.5));
#89603=CARTESIAN_POINT('',(34.9,7.4,48.5));
#89604=CARTESIAN_POINT('',(17.45,7.4,48.5));
#89605=CARTESIAN_POINT('',(34.9,7.4,48.35));
#89606=CARTESIAN_POINT('',(34.9,7.4,48.5));
#89607=CARTESIAN_POINT('',(35.1,7.4,48.35));
#89608=CARTESIAN_POINT('Origin',(34.9,5.2,48.5));
#89609=CARTESIAN_POINT('',(34.9,6.6,48.5));
#89610=CARTESIAN_POINT('',(34.9,7.4,48.35));
#89611=CARTESIAN_POINT('Origin',(35.,6.3,48.35));
#89612=CARTESIAN_POINT('Origin',(37.1,6.,48.5));
#89613=CARTESIAN_POINT('',(37.1,6.,48.5));
#89614=CARTESIAN_POINT('',(36.9,6.,48.5));
#89615=CARTESIAN_POINT('',(18.55,6.,48.5));
#89616=CARTESIAN_POINT('',(37.1,6.,48.35));
#89617=CARTESIAN_POINT('',(37.1,6.,48.5));
#89618=CARTESIAN_POINT('',(36.9,6.,48.35));
#89619=CARTESIAN_POINT('',(36.9,6.,48.35));
#89620=CARTESIAN_POINT('',(36.9,6.,48.5));
#89621=CARTESIAN_POINT('Origin',(37.1,7.4,48.5));
#89622=CARTESIAN_POINT('',(37.1,7.4,48.5));
#89623=CARTESIAN_POINT('',(37.1,7.7,48.5));
#89624=CARTESIAN_POINT('',(37.1,7.4,48.35));
#89625=CARTESIAN_POINT('',(37.1,7.4,48.5));
#89626=CARTESIAN_POINT('',(37.1,6.,48.35));
#89627=CARTESIAN_POINT('Origin',(36.9,7.4,48.5));
#89628=CARTESIAN_POINT('',(36.9,7.4,48.5));
#89629=CARTESIAN_POINT('',(18.45,7.4,48.5));
#89630=CARTESIAN_POINT('',(36.9,7.4,48.35));
#89631=CARTESIAN_POINT('',(36.9,7.4,48.5));
#89632=CARTESIAN_POINT('',(37.1,7.4,48.35));
#89633=CARTESIAN_POINT('Origin',(36.9,6.,48.5));
#89634=CARTESIAN_POINT('',(36.9,7.,48.5));
#89635=CARTESIAN_POINT('',(36.9,7.4,48.35));
#89636=CARTESIAN_POINT('Origin',(37.,6.7,48.35));
#89637=CARTESIAN_POINT('Origin',(39.1,6.,48.5));
#89638=CARTESIAN_POINT('',(39.1,6.,48.5));
#89639=CARTESIAN_POINT('',(38.9,6.,48.5));
#89640=CARTESIAN_POINT('',(19.55,6.,48.5));
#89641=CARTESIAN_POINT('',(39.1,6.,48.35));
#89642=CARTESIAN_POINT('',(39.1,6.,48.5));
#89643=CARTESIAN_POINT('',(38.9,6.,48.35));
#89644=CARTESIAN_POINT('',(38.9,6.,48.35));
#89645=CARTESIAN_POINT('',(38.9,6.,48.5));
#89646=CARTESIAN_POINT('Origin',(39.1,7.4,48.5));
#89647=CARTESIAN_POINT('',(39.1,7.4,48.5));
#89648=CARTESIAN_POINT('',(39.1,7.7,48.5));
#89649=CARTESIAN_POINT('',(39.1,7.4,48.35));
#89650=CARTESIAN_POINT('',(39.1,7.4,48.5));
#89651=CARTESIAN_POINT('',(39.1,6.,48.35));
#89652=CARTESIAN_POINT('Origin',(38.9,7.4,48.5));
#89653=CARTESIAN_POINT('',(38.9,7.4,48.5));
#89654=CARTESIAN_POINT('',(19.45,7.4,48.5));
#89655=CARTESIAN_POINT('',(38.9,7.4,48.35));
#89656=CARTESIAN_POINT('',(38.9,7.4,48.5));
#89657=CARTESIAN_POINT('',(39.1,7.4,48.35));
#89658=CARTESIAN_POINT('Origin',(38.9,6.,48.5));
#89659=CARTESIAN_POINT('',(38.9,7.,48.5));
#89660=CARTESIAN_POINT('',(38.9,7.4,48.35));
#89661=CARTESIAN_POINT('Origin',(39.,6.7,48.35));
#89662=CARTESIAN_POINT('Origin',(41.1,6.,48.5));
#89663=CARTESIAN_POINT('',(41.1,6.,48.5));
#89664=CARTESIAN_POINT('',(40.9,6.,48.5));
#89665=CARTESIAN_POINT('',(20.55,6.,48.5));
#89666=CARTESIAN_POINT('',(41.1,6.,48.35));
#89667=CARTESIAN_POINT('',(41.1,6.,48.5));
#89668=CARTESIAN_POINT('',(40.9,6.,48.35));
#89669=CARTESIAN_POINT('',(40.9,6.,48.35));
#89670=CARTESIAN_POINT('',(40.9,6.,48.5));
#89671=CARTESIAN_POINT('Origin',(41.1,7.4,48.5));
#89672=CARTESIAN_POINT('',(41.1,7.4,48.5));
#89673=CARTESIAN_POINT('',(41.1,7.7,48.5));
#89674=CARTESIAN_POINT('',(41.1,7.4,48.35));
#89675=CARTESIAN_POINT('',(41.1,7.4,48.5));
#89676=CARTESIAN_POINT('',(41.1,6.,48.35));
#89677=CARTESIAN_POINT('Origin',(40.9,7.4,48.5));
#89678=CARTESIAN_POINT('',(40.9,7.4,48.5));
#89679=CARTESIAN_POINT('',(20.45,7.4,48.5));
#89680=CARTESIAN_POINT('',(40.9,7.4,48.35));
#89681=CARTESIAN_POINT('',(40.9,7.4,48.5));
#89682=CARTESIAN_POINT('',(41.1,7.4,48.35));
#89683=CARTESIAN_POINT('Origin',(40.9,6.,48.5));
#89684=CARTESIAN_POINT('',(40.9,7.,48.5));
#89685=CARTESIAN_POINT('',(40.9,7.4,48.35));
#89686=CARTESIAN_POINT('Origin',(41.,6.7,48.35));
#89687=CARTESIAN_POINT('Origin',(43.1,6.,48.5));
#89688=CARTESIAN_POINT('',(43.1,6.,48.5));
#89689=CARTESIAN_POINT('',(42.9,6.,48.5));
#89690=CARTESIAN_POINT('',(21.55,6.,48.5));
#89691=CARTESIAN_POINT('',(43.1,6.,48.35));
#89692=CARTESIAN_POINT('',(43.1,6.,48.5));
#89693=CARTESIAN_POINT('',(42.9,6.,48.35));
#89694=CARTESIAN_POINT('',(42.9,6.,48.35));
#89695=CARTESIAN_POINT('',(42.9,6.,48.5));
#89696=CARTESIAN_POINT('Origin',(43.1,7.4,48.5));
#89697=CARTESIAN_POINT('',(43.1,7.4,48.5));
#89698=CARTESIAN_POINT('',(43.1,7.7,48.5));
#89699=CARTESIAN_POINT('',(43.1,7.4,48.35));
#89700=CARTESIAN_POINT('',(43.1,7.4,48.5));
#89701=CARTESIAN_POINT('',(43.1,6.,48.35));
#89702=CARTESIAN_POINT('Origin',(42.9,7.4,48.5));
#89703=CARTESIAN_POINT('',(42.9,7.4,48.5));
#89704=CARTESIAN_POINT('',(21.45,7.4,48.5));
#89705=CARTESIAN_POINT('',(42.9,7.4,48.35));
#89706=CARTESIAN_POINT('',(42.9,7.4,48.5));
#89707=CARTESIAN_POINT('',(43.1,7.4,48.35));
#89708=CARTESIAN_POINT('Origin',(42.9,6.,48.5));
#89709=CARTESIAN_POINT('',(42.9,7.,48.5));
#89710=CARTESIAN_POINT('',(42.9,7.4,48.35));
#89711=CARTESIAN_POINT('Origin',(43.,6.7,48.35));
#89712=CARTESIAN_POINT('Origin',(45.1,5.2,48.5));
#89713=CARTESIAN_POINT('',(45.1,5.2,48.5));
#89714=CARTESIAN_POINT('',(44.9,5.2,48.5));
#89715=CARTESIAN_POINT('',(22.55,5.2,48.5));
#89716=CARTESIAN_POINT('',(45.1,5.2,48.35));
#89717=CARTESIAN_POINT('',(45.1,5.2,48.5));
#89718=CARTESIAN_POINT('',(44.9,5.2,48.35));
#89719=CARTESIAN_POINT('',(44.9,5.2,48.35));
#89720=CARTESIAN_POINT('',(44.9,5.2,48.5));
#89721=CARTESIAN_POINT('Origin',(45.1,7.4,48.5));
#89722=CARTESIAN_POINT('',(45.1,7.4,48.5));
#89723=CARTESIAN_POINT('',(45.1,7.7,48.5));
#89724=CARTESIAN_POINT('',(45.1,7.4,48.35));
#89725=CARTESIAN_POINT('',(45.1,7.4,48.5));
#89726=CARTESIAN_POINT('',(45.1,5.2,48.35));
#89727=CARTESIAN_POINT('Origin',(44.9,7.4,48.5));
#89728=CARTESIAN_POINT('',(44.9,7.4,48.5));
#89729=CARTESIAN_POINT('',(22.45,7.4,48.5));
#89730=CARTESIAN_POINT('',(44.9,7.4,48.35));
#89731=CARTESIAN_POINT('',(44.9,7.4,48.5));
#89732=CARTESIAN_POINT('',(45.1,7.4,48.35));
#89733=CARTESIAN_POINT('Origin',(44.9,5.2,48.5));
#89734=CARTESIAN_POINT('',(44.9,6.6,48.5));
#89735=CARTESIAN_POINT('',(44.9,7.4,48.35));
#89736=CARTESIAN_POINT('Origin',(45.,6.3,48.35));
#89737=CARTESIAN_POINT('Origin',(47.1,6.,48.5));
#89738=CARTESIAN_POINT('',(47.1,6.,48.5));
#89739=CARTESIAN_POINT('',(46.9,6.,48.5));
#89740=CARTESIAN_POINT('',(23.55,6.,48.5));
#89741=CARTESIAN_POINT('',(47.1,6.,48.35));
#89742=CARTESIAN_POINT('',(47.1,6.,48.5));
#89743=CARTESIAN_POINT('',(46.9,6.,48.35));
#89744=CARTESIAN_POINT('',(46.9,6.,48.35));
#89745=CARTESIAN_POINT('',(46.9,6.,48.5));
#89746=CARTESIAN_POINT('Origin',(47.1,7.4,48.5));
#89747=CARTESIAN_POINT('',(47.1,7.4,48.5));
#89748=CARTESIAN_POINT('',(47.1,7.7,48.5));
#89749=CARTESIAN_POINT('',(47.1,7.4,48.35));
#89750=CARTESIAN_POINT('',(47.1,7.4,48.5));
#89751=CARTESIAN_POINT('',(47.1,6.,48.35));
#89752=CARTESIAN_POINT('Origin',(46.9,7.4,48.5));
#89753=CARTESIAN_POINT('',(46.9,7.4,48.5));
#89754=CARTESIAN_POINT('',(23.45,7.4,48.5));
#89755=CARTESIAN_POINT('',(46.9,7.4,48.35));
#89756=CARTESIAN_POINT('',(46.9,7.4,48.5));
#89757=CARTESIAN_POINT('',(47.1,7.4,48.35));
#89758=CARTESIAN_POINT('Origin',(46.9,6.,48.5));
#89759=CARTESIAN_POINT('',(46.9,7.,48.5));
#89760=CARTESIAN_POINT('',(46.9,7.4,48.35));
#89761=CARTESIAN_POINT('Origin',(47.,6.7,48.35));
#89762=CARTESIAN_POINT('Origin',(49.1,6.,48.5));
#89763=CARTESIAN_POINT('',(49.1,6.,48.5));
#89764=CARTESIAN_POINT('',(48.9,6.,48.5));
#89765=CARTESIAN_POINT('',(24.55,6.,48.5));
#89766=CARTESIAN_POINT('',(49.1,6.,48.35));
#89767=CARTESIAN_POINT('',(49.1,6.,48.5));
#89768=CARTESIAN_POINT('',(48.9,6.,48.35));
#89769=CARTESIAN_POINT('',(48.9,6.,48.35));
#89770=CARTESIAN_POINT('',(48.9,6.,48.5));
#89771=CARTESIAN_POINT('Origin',(49.1,7.4,48.5));
#89772=CARTESIAN_POINT('',(49.1,7.4,48.5));
#89773=CARTESIAN_POINT('',(49.1,7.7,48.5));
#89774=CARTESIAN_POINT('',(49.1,7.4,48.35));
#89775=CARTESIAN_POINT('',(49.1,7.4,48.5));
#89776=CARTESIAN_POINT('',(49.1,6.,48.35));
#89777=CARTESIAN_POINT('Origin',(48.9,7.4,48.5));
#89778=CARTESIAN_POINT('',(48.9,7.4,48.5));
#89779=CARTESIAN_POINT('',(24.45,7.4,48.5));
#89780=CARTESIAN_POINT('',(48.9,7.4,48.35));
#89781=CARTESIAN_POINT('',(48.9,7.4,48.5));
#89782=CARTESIAN_POINT('',(49.1,7.4,48.35));
#89783=CARTESIAN_POINT('Origin',(48.9,6.,48.5));
#89784=CARTESIAN_POINT('',(48.9,7.,48.5));
#89785=CARTESIAN_POINT('',(48.9,7.4,48.35));
#89786=CARTESIAN_POINT('Origin',(49.,6.7,48.35));
#89787=CARTESIAN_POINT('Origin',(51.1,6.,48.5));
#89788=CARTESIAN_POINT('',(51.1,6.,48.5));
#89789=CARTESIAN_POINT('',(50.9,6.,48.5));
#89790=CARTESIAN_POINT('',(25.55,6.,48.5));
#89791=CARTESIAN_POINT('',(51.1,6.,48.35));
#89792=CARTESIAN_POINT('',(51.1,6.,48.5));
#89793=CARTESIAN_POINT('',(50.9,6.,48.35));
#89794=CARTESIAN_POINT('',(50.9,6.,48.35));
#89795=CARTESIAN_POINT('',(50.9,6.,48.5));
#89796=CARTESIAN_POINT('Origin',(51.1,7.4,48.5));
#89797=CARTESIAN_POINT('',(51.1,7.4,48.5));
#89798=CARTESIAN_POINT('',(51.1,7.7,48.5));
#89799=CARTESIAN_POINT('',(51.1,7.4,48.35));
#89800=CARTESIAN_POINT('',(51.1,7.4,48.5));
#89801=CARTESIAN_POINT('',(51.1,6.,48.35));
#89802=CARTESIAN_POINT('Origin',(50.9,7.4,48.5));
#89803=CARTESIAN_POINT('',(50.9,7.4,48.5));
#89804=CARTESIAN_POINT('',(25.45,7.4,48.5));
#89805=CARTESIAN_POINT('',(50.9,7.4,48.35));
#89806=CARTESIAN_POINT('',(50.9,7.4,48.5));
#89807=CARTESIAN_POINT('',(51.1,7.4,48.35));
#89808=CARTESIAN_POINT('Origin',(50.9,6.,48.5));
#89809=CARTESIAN_POINT('',(50.9,7.,48.5));
#89810=CARTESIAN_POINT('',(50.9,7.4,48.35));
#89811=CARTESIAN_POINT('Origin',(51.,6.7,48.35));
#89812=CARTESIAN_POINT('Origin',(53.1,6.,48.5));
#89813=CARTESIAN_POINT('',(53.1,6.,48.5));
#89814=CARTESIAN_POINT('',(52.9,6.,48.5));
#89815=CARTESIAN_POINT('',(26.55,6.,48.5));
#89816=CARTESIAN_POINT('',(53.1,6.,48.35));
#89817=CARTESIAN_POINT('',(53.1,6.,48.5));
#89818=CARTESIAN_POINT('',(52.9,6.,48.35));
#89819=CARTESIAN_POINT('',(52.9,6.,48.35));
#89820=CARTESIAN_POINT('',(52.9,6.,48.5));
#89821=CARTESIAN_POINT('Origin',(53.1,7.4,48.5));
#89822=CARTESIAN_POINT('',(53.1,7.4,48.5));
#89823=CARTESIAN_POINT('',(53.1,7.7,48.5));
#89824=CARTESIAN_POINT('',(53.1,7.4,48.35));
#89825=CARTESIAN_POINT('',(53.1,7.4,48.5));
#89826=CARTESIAN_POINT('',(53.1,6.,48.35));
#89827=CARTESIAN_POINT('Origin',(52.9,7.4,48.5));
#89828=CARTESIAN_POINT('',(52.9,7.4,48.5));
#89829=CARTESIAN_POINT('',(26.45,7.4,48.5));
#89830=CARTESIAN_POINT('',(52.9,7.4,48.35));
#89831=CARTESIAN_POINT('',(52.9,7.4,48.5));
#89832=CARTESIAN_POINT('',(53.1,7.4,48.35));
#89833=CARTESIAN_POINT('Origin',(52.9,6.,48.5));
#89834=CARTESIAN_POINT('',(52.9,7.,48.5));
#89835=CARTESIAN_POINT('',(52.9,7.4,48.35));
#89836=CARTESIAN_POINT('Origin',(53.,6.7,48.35));
#89837=CARTESIAN_POINT('Origin',(55.1,5.2,48.5));
#89838=CARTESIAN_POINT('',(55.1,5.2,48.5));
#89839=CARTESIAN_POINT('',(54.9,5.2,48.5));
#89840=CARTESIAN_POINT('',(27.55,5.2,48.5));
#89841=CARTESIAN_POINT('',(55.1,5.2,48.35));
#89842=CARTESIAN_POINT('',(55.1,5.2,48.5));
#89843=CARTESIAN_POINT('',(54.9,5.2,48.35));
#89844=CARTESIAN_POINT('',(54.9,5.2,48.35));
#89845=CARTESIAN_POINT('',(54.9,5.2,48.5));
#89846=CARTESIAN_POINT('Origin',(55.1,7.4,48.5));
#89847=CARTESIAN_POINT('',(55.1,7.4,48.5));
#89848=CARTESIAN_POINT('',(55.1,7.7,48.5));
#89849=CARTESIAN_POINT('',(55.1,7.4,48.35));
#89850=CARTESIAN_POINT('',(55.1,7.4,48.5));
#89851=CARTESIAN_POINT('',(55.1,5.2,48.35));
#89852=CARTESIAN_POINT('Origin',(54.9,7.4,48.5));
#89853=CARTESIAN_POINT('',(54.9,7.4,48.5));
#89854=CARTESIAN_POINT('',(27.45,7.4,48.5));
#89855=CARTESIAN_POINT('',(54.9,7.4,48.35));
#89856=CARTESIAN_POINT('',(54.9,7.4,48.5));
#89857=CARTESIAN_POINT('',(55.1,7.4,48.35));
#89858=CARTESIAN_POINT('Origin',(54.9,5.2,48.5));
#89859=CARTESIAN_POINT('',(54.9,6.6,48.5));
#89860=CARTESIAN_POINT('',(54.9,7.4,48.35));
#89861=CARTESIAN_POINT('Origin',(55.,6.3,48.35));
#89862=CARTESIAN_POINT('Origin',(57.1,6.,48.5));
#89863=CARTESIAN_POINT('',(57.1,6.,48.5));
#89864=CARTESIAN_POINT('',(56.9,6.,48.5));
#89865=CARTESIAN_POINT('',(28.55,6.,48.5));
#89866=CARTESIAN_POINT('',(57.1,6.,48.35));
#89867=CARTESIAN_POINT('',(57.1,6.,48.5));
#89868=CARTESIAN_POINT('',(56.9,6.,48.35));
#89869=CARTESIAN_POINT('',(56.9,6.,48.35));
#89870=CARTESIAN_POINT('',(56.9,6.,48.5));
#89871=CARTESIAN_POINT('Origin',(57.1,7.4,48.5));
#89872=CARTESIAN_POINT('',(57.1,7.4,48.5));
#89873=CARTESIAN_POINT('',(57.1,7.7,48.5));
#89874=CARTESIAN_POINT('',(57.1,7.4,48.35));
#89875=CARTESIAN_POINT('',(57.1,7.4,48.5));
#89876=CARTESIAN_POINT('',(57.1,6.,48.35));
#89877=CARTESIAN_POINT('Origin',(56.9,7.4,48.5));
#89878=CARTESIAN_POINT('',(56.9,7.4,48.5));
#89879=CARTESIAN_POINT('',(28.45,7.4,48.5));
#89880=CARTESIAN_POINT('',(56.9,7.4,48.35));
#89881=CARTESIAN_POINT('',(56.9,7.4,48.5));
#89882=CARTESIAN_POINT('',(57.1,7.4,48.35));
#89883=CARTESIAN_POINT('Origin',(56.9,6.,48.5));
#89884=CARTESIAN_POINT('',(56.9,7.,48.5));
#89885=CARTESIAN_POINT('',(56.9,7.4,48.35));
#89886=CARTESIAN_POINT('Origin',(57.,6.7,48.35));
#89887=CARTESIAN_POINT('Origin',(59.1,6.,48.5));
#89888=CARTESIAN_POINT('',(59.1,6.,48.5));
#89889=CARTESIAN_POINT('',(58.9,6.,48.5));
#89890=CARTESIAN_POINT('',(29.55,6.,48.5));
#89891=CARTESIAN_POINT('',(59.1,6.,48.35));
#89892=CARTESIAN_POINT('',(59.1,6.,48.5));
#89893=CARTESIAN_POINT('',(58.9,6.,48.35));
#89894=CARTESIAN_POINT('',(58.9,6.,48.35));
#89895=CARTESIAN_POINT('',(58.9,6.,48.5));
#89896=CARTESIAN_POINT('Origin',(59.1,7.4,48.5));
#89897=CARTESIAN_POINT('',(59.1,7.4,48.5));
#89898=CARTESIAN_POINT('',(59.1,7.7,48.5));
#89899=CARTESIAN_POINT('',(59.1,7.4,48.35));
#89900=CARTESIAN_POINT('',(59.1,7.4,48.5));
#89901=CARTESIAN_POINT('',(59.1,6.,48.35));
#89902=CARTESIAN_POINT('Origin',(58.9,7.4,48.5));
#89903=CARTESIAN_POINT('',(58.9,7.4,48.5));
#89904=CARTESIAN_POINT('',(29.45,7.4,48.5));
#89905=CARTESIAN_POINT('',(58.9,7.4,48.35));
#89906=CARTESIAN_POINT('',(58.9,7.4,48.5));
#89907=CARTESIAN_POINT('',(59.1,7.4,48.35));
#89908=CARTESIAN_POINT('Origin',(58.9,6.,48.5));
#89909=CARTESIAN_POINT('',(58.9,7.,48.5));
#89910=CARTESIAN_POINT('',(58.9,7.4,48.35));
#89911=CARTESIAN_POINT('Origin',(59.,6.7,48.35));
#89912=CARTESIAN_POINT('Origin',(61.1,6.,48.5));
#89913=CARTESIAN_POINT('',(61.1,6.,48.5));
#89914=CARTESIAN_POINT('',(60.9,6.,48.5));
#89915=CARTESIAN_POINT('',(30.55,6.,48.5));
#89916=CARTESIAN_POINT('',(61.1,6.,48.35));
#89917=CARTESIAN_POINT('',(61.1,6.,48.5));
#89918=CARTESIAN_POINT('',(60.9,6.,48.35));
#89919=CARTESIAN_POINT('',(60.9,6.,48.35));
#89920=CARTESIAN_POINT('',(60.9,6.,48.5));
#89921=CARTESIAN_POINT('Origin',(61.1,7.4,48.5));
#89922=CARTESIAN_POINT('',(61.1,7.4,48.5));
#89923=CARTESIAN_POINT('',(61.1,7.7,48.5));
#89924=CARTESIAN_POINT('',(61.1,7.4,48.35));
#89925=CARTESIAN_POINT('',(61.1,7.4,48.5));
#89926=CARTESIAN_POINT('',(61.1,6.,48.35));
#89927=CARTESIAN_POINT('Origin',(60.9,7.4,48.5));
#89928=CARTESIAN_POINT('',(60.9,7.4,48.5));
#89929=CARTESIAN_POINT('',(30.45,7.4,48.5));
#89930=CARTESIAN_POINT('',(60.9,7.4,48.35));
#89931=CARTESIAN_POINT('',(60.9,7.4,48.5));
#89932=CARTESIAN_POINT('',(61.1,7.4,48.35));
#89933=CARTESIAN_POINT('Origin',(60.9,6.,48.5));
#89934=CARTESIAN_POINT('',(60.9,7.,48.5));
#89935=CARTESIAN_POINT('',(60.9,7.4,48.35));
#89936=CARTESIAN_POINT('Origin',(61.,6.7,48.35));
#89937=CARTESIAN_POINT('Origin',(63.1,6.,48.5));
#89938=CARTESIAN_POINT('',(63.1,6.,48.5));
#89939=CARTESIAN_POINT('',(62.9,6.,48.5));
#89940=CARTESIAN_POINT('',(31.55,6.,48.5));
#89941=CARTESIAN_POINT('',(63.1,6.,48.35));
#89942=CARTESIAN_POINT('',(63.1,6.,48.5));
#89943=CARTESIAN_POINT('',(62.9,6.,48.35));
#89944=CARTESIAN_POINT('',(62.9,6.,48.35));
#89945=CARTESIAN_POINT('',(62.9,6.,48.5));
#89946=CARTESIAN_POINT('Origin',(63.1,7.4,48.5));
#89947=CARTESIAN_POINT('',(63.1,7.4,48.5));
#89948=CARTESIAN_POINT('',(63.1,7.7,48.5));
#89949=CARTESIAN_POINT('',(63.1,7.4,48.35));
#89950=CARTESIAN_POINT('',(63.1,7.4,48.5));
#89951=CARTESIAN_POINT('',(63.1,6.,48.35));
#89952=CARTESIAN_POINT('Origin',(62.9,7.4,48.5));
#89953=CARTESIAN_POINT('',(62.9,7.4,48.5));
#89954=CARTESIAN_POINT('',(31.45,7.4,48.5));
#89955=CARTESIAN_POINT('',(62.9,7.4,48.35));
#89956=CARTESIAN_POINT('',(62.9,7.4,48.5));
#89957=CARTESIAN_POINT('',(63.1,7.4,48.35));
#89958=CARTESIAN_POINT('Origin',(62.9,6.,48.5));
#89959=CARTESIAN_POINT('',(62.9,7.,48.5));
#89960=CARTESIAN_POINT('',(62.9,7.4,48.35));
#89961=CARTESIAN_POINT('Origin',(63.,6.7,48.35));
#89962=CARTESIAN_POINT('Origin',(65.1,5.2,48.5));
#89963=CARTESIAN_POINT('',(65.1,5.2,48.5));
#89964=CARTESIAN_POINT('',(64.9,5.2,48.5));
#89965=CARTESIAN_POINT('',(32.55,5.2,48.5));
#89966=CARTESIAN_POINT('',(65.1,5.2,48.35));
#89967=CARTESIAN_POINT('',(65.1,5.2,48.5));
#89968=CARTESIAN_POINT('',(64.9,5.2,48.35));
#89969=CARTESIAN_POINT('',(64.9,5.2,48.35));
#89970=CARTESIAN_POINT('',(64.9,5.2,48.5));
#89971=CARTESIAN_POINT('Origin',(65.1,7.4,48.5));
#89972=CARTESIAN_POINT('',(65.1,7.4,48.5));
#89973=CARTESIAN_POINT('',(65.1,7.7,48.5));
#89974=CARTESIAN_POINT('',(65.1,7.4,48.35));
#89975=CARTESIAN_POINT('',(65.1,7.4,48.5));
#89976=CARTESIAN_POINT('',(65.1,5.2,48.35));
#89977=CARTESIAN_POINT('Origin',(64.9,7.4,48.5));
#89978=CARTESIAN_POINT('',(64.9,7.4,48.5));
#89979=CARTESIAN_POINT('',(32.45,7.4,48.5));
#89980=CARTESIAN_POINT('',(64.9,7.4,48.35));
#89981=CARTESIAN_POINT('',(64.9,7.4,48.5));
#89982=CARTESIAN_POINT('',(65.1,7.4,48.35));
#89983=CARTESIAN_POINT('Origin',(64.9,5.2,48.5));
#89984=CARTESIAN_POINT('',(64.9,6.6,48.5));
#89985=CARTESIAN_POINT('',(64.9,7.4,48.35));
#89986=CARTESIAN_POINT('Origin',(65.,6.3,48.35));
#89987=CARTESIAN_POINT('Origin',(67.1,6.,48.5));
#89988=CARTESIAN_POINT('',(67.1,6.,48.5));
#89989=CARTESIAN_POINT('',(66.9,6.,48.5));
#89990=CARTESIAN_POINT('',(33.55,6.,48.5));
#89991=CARTESIAN_POINT('',(67.1,6.,48.35));
#89992=CARTESIAN_POINT('',(67.1,6.,48.5));
#89993=CARTESIAN_POINT('',(66.9,6.,48.35));
#89994=CARTESIAN_POINT('',(66.9,6.,48.35));
#89995=CARTESIAN_POINT('',(66.9,6.,48.5));
#89996=CARTESIAN_POINT('Origin',(67.1,7.4,48.5));
#89997=CARTESIAN_POINT('',(67.1,7.4,48.5));
#89998=CARTESIAN_POINT('',(67.1,7.7,48.5));
#89999=CARTESIAN_POINT('',(67.1,7.4,48.35));
#90000=CARTESIAN_POINT('',(67.1,7.4,48.5));
#90001=CARTESIAN_POINT('',(67.1,6.,48.35));
#90002=CARTESIAN_POINT('Origin',(66.9,7.4,48.5));
#90003=CARTESIAN_POINT('',(66.9,7.4,48.5));
#90004=CARTESIAN_POINT('',(33.45,7.4,48.5));
#90005=CARTESIAN_POINT('',(66.9,7.4,48.35));
#90006=CARTESIAN_POINT('',(66.9,7.4,48.5));
#90007=CARTESIAN_POINT('',(67.1,7.4,48.35));
#90008=CARTESIAN_POINT('Origin',(66.9,6.,48.5));
#90009=CARTESIAN_POINT('',(66.9,7.,48.5));
#90010=CARTESIAN_POINT('',(66.9,7.4,48.35));
#90011=CARTESIAN_POINT('Origin',(67.,6.7,48.35));
#90012=CARTESIAN_POINT('Origin',(69.1,6.,48.5));
#90013=CARTESIAN_POINT('',(69.1,6.,48.5));
#90014=CARTESIAN_POINT('',(68.9,6.,48.5));
#90015=CARTESIAN_POINT('',(34.55,6.,48.5));
#90016=CARTESIAN_POINT('',(69.1,6.,48.35));
#90017=CARTESIAN_POINT('',(69.1,6.,48.5));
#90018=CARTESIAN_POINT('',(68.9,6.,48.35));
#90019=CARTESIAN_POINT('',(68.9,6.,48.35));
#90020=CARTESIAN_POINT('',(68.9,6.,48.5));
#90021=CARTESIAN_POINT('Origin',(69.1,7.4,48.5));
#90022=CARTESIAN_POINT('',(69.1,7.4,48.5));
#90023=CARTESIAN_POINT('',(69.1,7.7,48.5));
#90024=CARTESIAN_POINT('',(69.1,7.4,48.35));
#90025=CARTESIAN_POINT('',(69.1,7.4,48.5));
#90026=CARTESIAN_POINT('',(69.1,6.,48.35));
#90027=CARTESIAN_POINT('Origin',(68.9,7.4,48.5));
#90028=CARTESIAN_POINT('',(68.9,7.4,48.5));
#90029=CARTESIAN_POINT('',(34.45,7.4,48.5));
#90030=CARTESIAN_POINT('',(68.9,7.4,48.35));
#90031=CARTESIAN_POINT('',(68.9,7.4,48.5));
#90032=CARTESIAN_POINT('',(69.1,7.4,48.35));
#90033=CARTESIAN_POINT('Origin',(68.9,6.,48.5));
#90034=CARTESIAN_POINT('',(68.9,7.,48.5));
#90035=CARTESIAN_POINT('',(68.9,7.4,48.35));
#90036=CARTESIAN_POINT('Origin',(69.,6.7,48.35));
#90037=CARTESIAN_POINT('Origin',(71.1,6.,48.5));
#90038=CARTESIAN_POINT('',(71.1,6.,48.5));
#90039=CARTESIAN_POINT('',(70.9,6.,48.5));
#90040=CARTESIAN_POINT('',(35.55,6.,48.5));
#90041=CARTESIAN_POINT('',(71.1,6.,48.35));
#90042=CARTESIAN_POINT('',(71.1,6.,48.5));
#90043=CARTESIAN_POINT('',(70.9,6.,48.35));
#90044=CARTESIAN_POINT('',(70.9,6.,48.35));
#90045=CARTESIAN_POINT('',(70.9,6.,48.5));
#90046=CARTESIAN_POINT('Origin',(71.1,7.4,48.5));
#90047=CARTESIAN_POINT('',(71.1,7.4,48.5));
#90048=CARTESIAN_POINT('',(71.1,7.7,48.5));
#90049=CARTESIAN_POINT('',(71.1,7.4,48.35));
#90050=CARTESIAN_POINT('',(71.1,7.4,48.5));
#90051=CARTESIAN_POINT('',(71.1,6.,48.35));
#90052=CARTESIAN_POINT('Origin',(70.9,7.4,48.5));
#90053=CARTESIAN_POINT('',(70.9,7.4,48.5));
#90054=CARTESIAN_POINT('',(35.45,7.4,48.5));
#90055=CARTESIAN_POINT('',(70.9,7.4,48.35));
#90056=CARTESIAN_POINT('',(70.9,7.4,48.5));
#90057=CARTESIAN_POINT('',(71.1,7.4,48.35));
#90058=CARTESIAN_POINT('Origin',(70.9,6.,48.5));
#90059=CARTESIAN_POINT('',(70.9,7.,48.5));
#90060=CARTESIAN_POINT('',(70.9,7.4,48.35));
#90061=CARTESIAN_POINT('Origin',(71.,6.7,48.35));
#90062=CARTESIAN_POINT('Origin',(73.1,6.,48.5));
#90063=CARTESIAN_POINT('',(73.1,6.,48.5));
#90064=CARTESIAN_POINT('',(72.9,6.,48.5));
#90065=CARTESIAN_POINT('',(36.55,6.,48.5));
#90066=CARTESIAN_POINT('',(73.1,6.,48.35));
#90067=CARTESIAN_POINT('',(73.1,6.,48.5));
#90068=CARTESIAN_POINT('',(72.9,6.,48.35));
#90069=CARTESIAN_POINT('',(72.9,6.,48.35));
#90070=CARTESIAN_POINT('',(72.9,6.,48.5));
#90071=CARTESIAN_POINT('Origin',(73.1,7.4,48.5));
#90072=CARTESIAN_POINT('',(73.1,7.4,48.5));
#90073=CARTESIAN_POINT('',(73.1,7.7,48.5));
#90074=CARTESIAN_POINT('',(73.1,7.4,48.35));
#90075=CARTESIAN_POINT('',(73.1,7.4,48.5));
#90076=CARTESIAN_POINT('',(73.1,6.,48.35));
#90077=CARTESIAN_POINT('Origin',(72.9,7.4,48.5));
#90078=CARTESIAN_POINT('',(72.9,7.4,48.5));
#90079=CARTESIAN_POINT('',(36.45,7.4,48.5));
#90080=CARTESIAN_POINT('',(72.9,7.4,48.35));
#90081=CARTESIAN_POINT('',(72.9,7.4,48.5));
#90082=CARTESIAN_POINT('',(73.1,7.4,48.35));
#90083=CARTESIAN_POINT('Origin',(72.9,6.,48.5));
#90084=CARTESIAN_POINT('',(72.9,7.,48.5));
#90085=CARTESIAN_POINT('',(72.9,7.4,48.35));
#90086=CARTESIAN_POINT('Origin',(73.,6.7,48.35));
#90087=CARTESIAN_POINT('Origin',(75.1,5.2,48.5));
#90088=CARTESIAN_POINT('',(75.1,5.2,48.5));
#90089=CARTESIAN_POINT('',(74.9,5.2,48.5));
#90090=CARTESIAN_POINT('',(37.55,5.2,48.5));
#90091=CARTESIAN_POINT('',(75.1,5.2,48.35));
#90092=CARTESIAN_POINT('',(75.1,5.2,48.5));
#90093=CARTESIAN_POINT('',(74.9,5.2,48.35));
#90094=CARTESIAN_POINT('',(74.9,5.2,48.35));
#90095=CARTESIAN_POINT('',(74.9,5.2,48.5));
#90096=CARTESIAN_POINT('Origin',(75.1,7.4,48.5));
#90097=CARTESIAN_POINT('',(75.1,7.4,48.5));
#90098=CARTESIAN_POINT('',(75.1,7.7,48.5));
#90099=CARTESIAN_POINT('',(75.1,7.4,48.35));
#90100=CARTESIAN_POINT('',(75.1,7.4,48.5));
#90101=CARTESIAN_POINT('',(75.1,5.2,48.35));
#90102=CARTESIAN_POINT('Origin',(74.9,7.4,48.5));
#90103=CARTESIAN_POINT('',(74.9,7.4,48.5));
#90104=CARTESIAN_POINT('',(37.45,7.4,48.5));
#90105=CARTESIAN_POINT('',(74.9,7.4,48.35));
#90106=CARTESIAN_POINT('',(74.9,7.4,48.5));
#90107=CARTESIAN_POINT('',(75.1,7.4,48.35));
#90108=CARTESIAN_POINT('Origin',(74.9,5.2,48.5));
#90109=CARTESIAN_POINT('',(74.9,6.6,48.5));
#90110=CARTESIAN_POINT('',(74.9,7.4,48.35));
#90111=CARTESIAN_POINT('Origin',(75.,6.3,48.35));
#90112=CARTESIAN_POINT('Origin',(77.1,6.,48.5));
#90113=CARTESIAN_POINT('',(77.1,6.,48.5));
#90114=CARTESIAN_POINT('',(76.9,6.,48.5));
#90115=CARTESIAN_POINT('',(38.55,6.,48.5));
#90116=CARTESIAN_POINT('',(77.1,6.,48.35));
#90117=CARTESIAN_POINT('',(77.1,6.,48.5));
#90118=CARTESIAN_POINT('',(76.9,6.,48.35));
#90119=CARTESIAN_POINT('',(76.9,6.,48.35));
#90120=CARTESIAN_POINT('',(76.9,6.,48.5));
#90121=CARTESIAN_POINT('Origin',(77.1,7.4,48.5));
#90122=CARTESIAN_POINT('',(77.1,7.4,48.5));
#90123=CARTESIAN_POINT('',(77.1,7.7,48.5));
#90124=CARTESIAN_POINT('',(77.1,7.4,48.35));
#90125=CARTESIAN_POINT('',(77.1,7.4,48.5));
#90126=CARTESIAN_POINT('',(77.1,6.,48.35));
#90127=CARTESIAN_POINT('Origin',(76.9,7.4,48.5));
#90128=CARTESIAN_POINT('',(76.9,7.4,48.5));
#90129=CARTESIAN_POINT('',(38.45,7.4,48.5));
#90130=CARTESIAN_POINT('',(76.9,7.4,48.35));
#90131=CARTESIAN_POINT('',(76.9,7.4,48.5));
#90132=CARTESIAN_POINT('',(77.1,7.4,48.35));
#90133=CARTESIAN_POINT('Origin',(76.9,6.,48.5));
#90134=CARTESIAN_POINT('',(76.9,7.,48.5));
#90135=CARTESIAN_POINT('',(76.9,7.4,48.35));
#90136=CARTESIAN_POINT('Origin',(77.,6.7,48.35));
#90137=CARTESIAN_POINT('Origin',(79.1,6.,48.5));
#90138=CARTESIAN_POINT('',(79.1,6.,48.5));
#90139=CARTESIAN_POINT('',(78.9,6.,48.5));
#90140=CARTESIAN_POINT('',(39.55,6.,48.5));
#90141=CARTESIAN_POINT('',(79.1,6.,48.35));
#90142=CARTESIAN_POINT('',(79.1,6.,48.5));
#90143=CARTESIAN_POINT('',(78.9,6.,48.35));
#90144=CARTESIAN_POINT('',(78.9,6.,48.35));
#90145=CARTESIAN_POINT('',(78.9,6.,48.5));
#90146=CARTESIAN_POINT('Origin',(79.1,7.4,48.5));
#90147=CARTESIAN_POINT('',(79.1,7.4,48.5));
#90148=CARTESIAN_POINT('',(79.1,7.7,48.5));
#90149=CARTESIAN_POINT('',(79.1,7.4,48.35));
#90150=CARTESIAN_POINT('',(79.1,7.4,48.5));
#90151=CARTESIAN_POINT('',(79.1,6.,48.35));
#90152=CARTESIAN_POINT('Origin',(78.9,7.4,48.5));
#90153=CARTESIAN_POINT('',(78.9,7.4,48.5));
#90154=CARTESIAN_POINT('',(39.45,7.4,48.5));
#90155=CARTESIAN_POINT('',(78.9,7.4,48.35));
#90156=CARTESIAN_POINT('',(78.9,7.4,48.5));
#90157=CARTESIAN_POINT('',(79.1,7.4,48.35));
#90158=CARTESIAN_POINT('Origin',(78.9,6.,48.5));
#90159=CARTESIAN_POINT('',(78.9,7.,48.5));
#90160=CARTESIAN_POINT('',(78.9,7.4,48.35));
#90161=CARTESIAN_POINT('Origin',(79.,6.7,48.35));
#90162=CARTESIAN_POINT('Origin',(81.1,6.,48.5));
#90163=CARTESIAN_POINT('',(81.1,6.,48.5));
#90164=CARTESIAN_POINT('',(80.9,6.,48.5));
#90165=CARTESIAN_POINT('',(40.55,6.,48.5));
#90166=CARTESIAN_POINT('',(81.1,6.,48.35));
#90167=CARTESIAN_POINT('',(81.1,6.,48.5));
#90168=CARTESIAN_POINT('',(80.9,6.,48.35));
#90169=CARTESIAN_POINT('',(80.9,6.,48.35));
#90170=CARTESIAN_POINT('',(80.9,6.,48.5));
#90171=CARTESIAN_POINT('Origin',(81.1,7.4,48.5));
#90172=CARTESIAN_POINT('',(81.1,7.4,48.5));
#90173=CARTESIAN_POINT('',(81.1,7.7,48.5));
#90174=CARTESIAN_POINT('',(81.1,7.4,48.35));
#90175=CARTESIAN_POINT('',(81.1,7.4,48.5));
#90176=CARTESIAN_POINT('',(81.1,6.,48.35));
#90177=CARTESIAN_POINT('Origin',(80.9,7.4,48.5));
#90178=CARTESIAN_POINT('',(80.9,7.4,48.5));
#90179=CARTESIAN_POINT('',(40.45,7.4,48.5));
#90180=CARTESIAN_POINT('',(80.9,7.4,48.35));
#90181=CARTESIAN_POINT('',(80.9,7.4,48.5));
#90182=CARTESIAN_POINT('',(81.1,7.4,48.35));
#90183=CARTESIAN_POINT('Origin',(80.9,6.,48.5));
#90184=CARTESIAN_POINT('',(80.9,7.,48.5));
#90185=CARTESIAN_POINT('',(80.9,7.4,48.35));
#90186=CARTESIAN_POINT('Origin',(81.,6.7,48.35));
#90187=CARTESIAN_POINT('Origin',(83.1,6.,48.5));
#90188=CARTESIAN_POINT('',(83.1,6.,48.5));
#90189=CARTESIAN_POINT('',(82.9,6.,48.5));
#90190=CARTESIAN_POINT('',(41.55,6.,48.5));
#90191=CARTESIAN_POINT('',(83.1,6.,48.35));
#90192=CARTESIAN_POINT('',(83.1,6.,48.5));
#90193=CARTESIAN_POINT('',(82.9,6.,48.35));
#90194=CARTESIAN_POINT('',(82.9,6.,48.35));
#90195=CARTESIAN_POINT('',(82.9,6.,48.5));
#90196=CARTESIAN_POINT('Origin',(83.1,7.4,48.5));
#90197=CARTESIAN_POINT('',(83.1,7.4,48.5));
#90198=CARTESIAN_POINT('',(83.1,7.7,48.5));
#90199=CARTESIAN_POINT('',(83.1,7.4,48.35));
#90200=CARTESIAN_POINT('',(83.1,7.4,48.5));
#90201=CARTESIAN_POINT('',(83.1,6.,48.35));
#90202=CARTESIAN_POINT('Origin',(82.9,7.4,48.5));
#90203=CARTESIAN_POINT('',(82.9,7.4,48.5));
#90204=CARTESIAN_POINT('',(41.45,7.4,48.5));
#90205=CARTESIAN_POINT('',(82.9,7.4,48.35));
#90206=CARTESIAN_POINT('',(82.9,7.4,48.5));
#90207=CARTESIAN_POINT('',(83.1,7.4,48.35));
#90208=CARTESIAN_POINT('Origin',(82.9,6.,48.5));
#90209=CARTESIAN_POINT('',(82.9,7.,48.5));
#90210=CARTESIAN_POINT('',(82.9,7.4,48.35));
#90211=CARTESIAN_POINT('Origin',(83.,6.7,48.35));
#90212=CARTESIAN_POINT('Origin',(85.1,5.2,48.5));
#90213=CARTESIAN_POINT('',(85.1,5.2,48.5));
#90214=CARTESIAN_POINT('',(84.9,5.2,48.5));
#90215=CARTESIAN_POINT('',(42.55,5.2,48.5));
#90216=CARTESIAN_POINT('',(85.1,5.2,48.35));
#90217=CARTESIAN_POINT('',(85.1,5.2,48.5));
#90218=CARTESIAN_POINT('',(84.9,5.2,48.35));
#90219=CARTESIAN_POINT('',(84.9,5.2,48.35));
#90220=CARTESIAN_POINT('',(84.9,5.2,48.5));
#90221=CARTESIAN_POINT('Origin',(85.1,7.4,48.5));
#90222=CARTESIAN_POINT('',(85.1,7.4,48.5));
#90223=CARTESIAN_POINT('',(85.1,7.7,48.5));
#90224=CARTESIAN_POINT('',(85.1,7.4,48.35));
#90225=CARTESIAN_POINT('',(85.1,7.4,48.5));
#90226=CARTESIAN_POINT('',(85.1,5.2,48.35));
#90227=CARTESIAN_POINT('Origin',(84.9,7.4,48.5));
#90228=CARTESIAN_POINT('',(84.9,7.4,48.5));
#90229=CARTESIAN_POINT('',(42.45,7.4,48.5));
#90230=CARTESIAN_POINT('',(84.9,7.4,48.35));
#90231=CARTESIAN_POINT('',(84.9,7.4,48.5));
#90232=CARTESIAN_POINT('',(85.1,7.4,48.35));
#90233=CARTESIAN_POINT('Origin',(84.9,5.2,48.5));
#90234=CARTESIAN_POINT('',(84.9,6.6,48.5));
#90235=CARTESIAN_POINT('',(84.9,7.4,48.35));
#90236=CARTESIAN_POINT('Origin',(85.,6.3,48.35));
#90237=CARTESIAN_POINT('Origin',(87.1,6.,48.5));
#90238=CARTESIAN_POINT('',(87.1,6.,48.5));
#90239=CARTESIAN_POINT('',(86.9,6.,48.5));
#90240=CARTESIAN_POINT('',(43.55,6.,48.5));
#90241=CARTESIAN_POINT('',(87.1,6.,48.35));
#90242=CARTESIAN_POINT('',(87.1,6.,48.5));
#90243=CARTESIAN_POINT('',(86.9,6.,48.35));
#90244=CARTESIAN_POINT('',(86.9,6.,48.35));
#90245=CARTESIAN_POINT('',(86.9,6.,48.5));
#90246=CARTESIAN_POINT('Origin',(87.1,7.4,48.5));
#90247=CARTESIAN_POINT('',(87.1,7.4,48.5));
#90248=CARTESIAN_POINT('',(87.1,7.7,48.5));
#90249=CARTESIAN_POINT('',(87.1,7.4,48.35));
#90250=CARTESIAN_POINT('',(87.1,7.4,48.5));
#90251=CARTESIAN_POINT('',(87.1,6.,48.35));
#90252=CARTESIAN_POINT('Origin',(86.9,7.4,48.5));
#90253=CARTESIAN_POINT('',(86.9,7.4,48.5));
#90254=CARTESIAN_POINT('',(43.45,7.4,48.5));
#90255=CARTESIAN_POINT('',(86.9,7.4,48.35));
#90256=CARTESIAN_POINT('',(86.9,7.4,48.5));
#90257=CARTESIAN_POINT('',(87.1,7.4,48.35));
#90258=CARTESIAN_POINT('Origin',(86.9,6.,48.5));
#90259=CARTESIAN_POINT('',(86.9,7.,48.5));
#90260=CARTESIAN_POINT('',(86.9,7.4,48.35));
#90261=CARTESIAN_POINT('Origin',(87.,6.7,48.35));
#90262=CARTESIAN_POINT('Origin',(89.1,6.,48.5));
#90263=CARTESIAN_POINT('',(89.1,6.,48.5));
#90264=CARTESIAN_POINT('',(88.9,6.,48.5));
#90265=CARTESIAN_POINT('',(44.55,6.,48.5));
#90266=CARTESIAN_POINT('',(89.1,6.,48.35));
#90267=CARTESIAN_POINT('',(89.1,6.,48.5));
#90268=CARTESIAN_POINT('',(88.9,6.,48.35));
#90269=CARTESIAN_POINT('',(88.9,6.,48.35));
#90270=CARTESIAN_POINT('',(88.9,6.,48.5));
#90271=CARTESIAN_POINT('Origin',(89.1,7.4,48.5));
#90272=CARTESIAN_POINT('',(89.1,7.4,48.5));
#90273=CARTESIAN_POINT('',(89.1,7.7,48.5));
#90274=CARTESIAN_POINT('',(89.1,7.4,48.35));
#90275=CARTESIAN_POINT('',(89.1,7.4,48.5));
#90276=CARTESIAN_POINT('',(89.1,6.,48.35));
#90277=CARTESIAN_POINT('Origin',(88.9,7.4,48.5));
#90278=CARTESIAN_POINT('',(88.9,7.4,48.5));
#90279=CARTESIAN_POINT('',(44.45,7.4,48.5));
#90280=CARTESIAN_POINT('',(88.9,7.4,48.35));
#90281=CARTESIAN_POINT('',(88.9,7.4,48.5));
#90282=CARTESIAN_POINT('',(89.1,7.4,48.35));
#90283=CARTESIAN_POINT('Origin',(88.9,6.,48.5));
#90284=CARTESIAN_POINT('',(88.9,7.,48.5));
#90285=CARTESIAN_POINT('',(88.9,7.4,48.35));
#90286=CARTESIAN_POINT('Origin',(89.,6.7,48.35));
#90287=CARTESIAN_POINT('Origin',(91.1,6.,48.5));
#90288=CARTESIAN_POINT('',(91.1,6.,48.5));
#90289=CARTESIAN_POINT('',(90.9,6.,48.5));
#90290=CARTESIAN_POINT('',(45.55,6.,48.5));
#90291=CARTESIAN_POINT('',(91.1,6.,48.35));
#90292=CARTESIAN_POINT('',(91.1,6.,48.5));
#90293=CARTESIAN_POINT('',(90.9,6.,48.35));
#90294=CARTESIAN_POINT('',(90.9,6.,48.35));
#90295=CARTESIAN_POINT('',(90.9,6.,48.5));
#90296=CARTESIAN_POINT('Origin',(91.1,7.4,48.5));
#90297=CARTESIAN_POINT('',(91.1,7.4,48.5));
#90298=CARTESIAN_POINT('',(91.1,7.7,48.5));
#90299=CARTESIAN_POINT('',(91.1,7.4,48.35));
#90300=CARTESIAN_POINT('',(91.1,7.4,48.5));
#90301=CARTESIAN_POINT('',(91.1,6.,48.35));
#90302=CARTESIAN_POINT('Origin',(90.9,7.4,48.5));
#90303=CARTESIAN_POINT('',(90.9,7.4,48.5));
#90304=CARTESIAN_POINT('',(45.45,7.4,48.5));
#90305=CARTESIAN_POINT('',(90.9,7.4,48.35));
#90306=CARTESIAN_POINT('',(90.9,7.4,48.5));
#90307=CARTESIAN_POINT('',(91.1,7.4,48.35));
#90308=CARTESIAN_POINT('Origin',(90.9,6.,48.5));
#90309=CARTESIAN_POINT('',(90.9,7.,48.5));
#90310=CARTESIAN_POINT('',(90.9,7.4,48.35));
#90311=CARTESIAN_POINT('Origin',(91.,6.7,48.35));
#90312=CARTESIAN_POINT('Origin',(93.1,6.,48.5));
#90313=CARTESIAN_POINT('',(93.1,6.,48.5));
#90314=CARTESIAN_POINT('',(92.9,6.,48.5));
#90315=CARTESIAN_POINT('',(46.55,6.,48.5));
#90316=CARTESIAN_POINT('',(93.1,6.,48.35));
#90317=CARTESIAN_POINT('',(93.1,6.,48.5));
#90318=CARTESIAN_POINT('',(92.9,6.,48.35));
#90319=CARTESIAN_POINT('',(92.9,6.,48.35));
#90320=CARTESIAN_POINT('',(92.9,6.,48.5));
#90321=CARTESIAN_POINT('Origin',(93.1,7.4,48.5));
#90322=CARTESIAN_POINT('',(93.1,7.4,48.5));
#90323=CARTESIAN_POINT('',(93.1,7.7,48.5));
#90324=CARTESIAN_POINT('',(93.1,7.4,48.35));
#90325=CARTESIAN_POINT('',(93.1,7.4,48.5));
#90326=CARTESIAN_POINT('',(93.1,6.,48.35));
#90327=CARTESIAN_POINT('Origin',(92.9,7.4,48.5));
#90328=CARTESIAN_POINT('',(92.9,7.4,48.5));
#90329=CARTESIAN_POINT('',(46.45,7.4,48.5));
#90330=CARTESIAN_POINT('',(92.9,7.4,48.35));
#90331=CARTESIAN_POINT('',(92.9,7.4,48.5));
#90332=CARTESIAN_POINT('',(93.1,7.4,48.35));
#90333=CARTESIAN_POINT('Origin',(92.9,6.,48.5));
#90334=CARTESIAN_POINT('',(92.9,7.,48.5));
#90335=CARTESIAN_POINT('',(92.9,7.4,48.35));
#90336=CARTESIAN_POINT('Origin',(93.,6.7,48.35));
#90337=CARTESIAN_POINT('Origin',(95.1,5.2,48.5));
#90338=CARTESIAN_POINT('',(95.1,5.2,48.5));
#90339=CARTESIAN_POINT('',(94.9,5.2,48.5));
#90340=CARTESIAN_POINT('',(47.55,5.2,48.5));
#90341=CARTESIAN_POINT('',(95.1,5.2,48.35));
#90342=CARTESIAN_POINT('',(95.1,5.2,48.5));
#90343=CARTESIAN_POINT('',(94.9,5.2,48.35));
#90344=CARTESIAN_POINT('',(94.9,5.2,48.35));
#90345=CARTESIAN_POINT('',(94.9,5.2,48.5));
#90346=CARTESIAN_POINT('Origin',(95.1,7.4,48.5));
#90347=CARTESIAN_POINT('',(95.1,7.4,48.5));
#90348=CARTESIAN_POINT('',(95.1,7.7,48.5));
#90349=CARTESIAN_POINT('',(95.1,7.4,48.35));
#90350=CARTESIAN_POINT('',(95.1,7.4,48.5));
#90351=CARTESIAN_POINT('',(95.1,5.2,48.35));
#90352=CARTESIAN_POINT('Origin',(94.9,7.4,48.5));
#90353=CARTESIAN_POINT('',(94.9,7.4,48.5));
#90354=CARTESIAN_POINT('',(47.45,7.4,48.5));
#90355=CARTESIAN_POINT('',(94.9,7.4,48.35));
#90356=CARTESIAN_POINT('',(94.9,7.4,48.5));
#90357=CARTESIAN_POINT('',(95.1,7.4,48.35));
#90358=CARTESIAN_POINT('Origin',(94.9,5.2,48.5));
#90359=CARTESIAN_POINT('',(94.9,6.6,48.5));
#90360=CARTESIAN_POINT('',(94.9,7.4,48.35));
#90361=CARTESIAN_POINT('Origin',(95.,6.3,48.35));
#90362=CARTESIAN_POINT('Origin',(97.1,6.,48.5));
#90363=CARTESIAN_POINT('',(97.1,6.,48.5));
#90364=CARTESIAN_POINT('',(96.9,6.,48.5));
#90365=CARTESIAN_POINT('',(48.55,6.,48.5));
#90366=CARTESIAN_POINT('',(97.1,6.,48.35));
#90367=CARTESIAN_POINT('',(97.1,6.,48.5));
#90368=CARTESIAN_POINT('',(96.9,6.,48.35));
#90369=CARTESIAN_POINT('',(96.9,6.,48.35));
#90370=CARTESIAN_POINT('',(96.9,6.,48.5));
#90371=CARTESIAN_POINT('Origin',(97.1,7.4,48.5));
#90372=CARTESIAN_POINT('',(97.1,7.4,48.5));
#90373=CARTESIAN_POINT('',(97.1,7.7,48.5));
#90374=CARTESIAN_POINT('',(97.1,7.4,48.35));
#90375=CARTESIAN_POINT('',(97.1,7.4,48.5));
#90376=CARTESIAN_POINT('',(97.1,6.,48.35));
#90377=CARTESIAN_POINT('Origin',(96.9,7.4,48.5));
#90378=CARTESIAN_POINT('',(96.9,7.4,48.5));
#90379=CARTESIAN_POINT('',(48.45,7.4,48.5));
#90380=CARTESIAN_POINT('',(96.9,7.4,48.35));
#90381=CARTESIAN_POINT('',(96.9,7.4,48.5));
#90382=CARTESIAN_POINT('',(97.1,7.4,48.35));
#90383=CARTESIAN_POINT('Origin',(96.9,6.,48.5));
#90384=CARTESIAN_POINT('',(96.9,7.,48.5));
#90385=CARTESIAN_POINT('',(96.9,7.4,48.35));
#90386=CARTESIAN_POINT('Origin',(97.,6.7,48.35));
#90387=CARTESIAN_POINT('Origin',(99.1,6.,48.5));
#90388=CARTESIAN_POINT('',(99.1,6.,48.5));
#90389=CARTESIAN_POINT('',(98.9,6.,48.5));
#90390=CARTESIAN_POINT('',(49.55,6.,48.5));
#90391=CARTESIAN_POINT('',(99.1,6.,48.35));
#90392=CARTESIAN_POINT('',(99.1,6.,48.5));
#90393=CARTESIAN_POINT('',(98.9,6.,48.35));
#90394=CARTESIAN_POINT('',(98.9,6.,48.35));
#90395=CARTESIAN_POINT('',(98.9,6.,48.5));
#90396=CARTESIAN_POINT('Origin',(99.1,7.4,48.5));
#90397=CARTESIAN_POINT('',(99.1,7.4,48.5));
#90398=CARTESIAN_POINT('',(99.1,7.7,48.5));
#90399=CARTESIAN_POINT('',(99.1,7.4,48.35));
#90400=CARTESIAN_POINT('',(99.1,7.4,48.5));
#90401=CARTESIAN_POINT('',(99.1,6.,48.35));
#90402=CARTESIAN_POINT('Origin',(98.9,7.4,48.5));
#90403=CARTESIAN_POINT('',(98.9,7.4,48.5));
#90404=CARTESIAN_POINT('',(49.45,7.4,48.5));
#90405=CARTESIAN_POINT('',(98.9,7.4,48.35));
#90406=CARTESIAN_POINT('',(98.9,7.4,48.5));
#90407=CARTESIAN_POINT('',(99.1,7.4,48.35));
#90408=CARTESIAN_POINT('Origin',(98.9,6.,48.5));
#90409=CARTESIAN_POINT('',(98.9,7.,48.5));
#90410=CARTESIAN_POINT('',(98.9,7.4,48.35));
#90411=CARTESIAN_POINT('Origin',(99.,6.7,48.35));
#90412=CARTESIAN_POINT('Origin',(101.1,6.,48.5));
#90413=CARTESIAN_POINT('',(101.1,6.,48.5));
#90414=CARTESIAN_POINT('',(100.9,6.,48.5));
#90415=CARTESIAN_POINT('',(50.55,6.,48.5));
#90416=CARTESIAN_POINT('',(101.1,6.,48.35));
#90417=CARTESIAN_POINT('',(101.1,6.,48.5));
#90418=CARTESIAN_POINT('',(100.9,6.,48.35));
#90419=CARTESIAN_POINT('',(100.9,6.,48.35));
#90420=CARTESIAN_POINT('',(100.9,6.,48.5));
#90421=CARTESIAN_POINT('Origin',(101.1,7.4,48.5));
#90422=CARTESIAN_POINT('',(101.1,7.4,48.5));
#90423=CARTESIAN_POINT('',(101.1,7.7,48.5));
#90424=CARTESIAN_POINT('',(101.1,7.4,48.35));
#90425=CARTESIAN_POINT('',(101.1,7.4,48.5));
#90426=CARTESIAN_POINT('',(101.1,6.,48.35));
#90427=CARTESIAN_POINT('Origin',(100.9,7.4,48.5));
#90428=CARTESIAN_POINT('',(100.9,7.4,48.5));
#90429=CARTESIAN_POINT('',(50.45,7.4,48.5));
#90430=CARTESIAN_POINT('',(100.9,7.4,48.35));
#90431=CARTESIAN_POINT('',(100.9,7.4,48.5));
#90432=CARTESIAN_POINT('',(101.1,7.4,48.35));
#90433=CARTESIAN_POINT('Origin',(100.9,6.,48.5));
#90434=CARTESIAN_POINT('',(100.9,7.,48.5));
#90435=CARTESIAN_POINT('',(100.9,7.4,48.35));
#90436=CARTESIAN_POINT('Origin',(101.,6.7,48.35));
#90437=CARTESIAN_POINT('Origin',(103.1,6.,48.5));
#90438=CARTESIAN_POINT('',(103.1,6.,48.5));
#90439=CARTESIAN_POINT('',(102.9,6.,48.5));
#90440=CARTESIAN_POINT('',(51.55,6.,48.5));
#90441=CARTESIAN_POINT('',(103.1,6.,48.35));
#90442=CARTESIAN_POINT('',(103.1,6.,48.5));
#90443=CARTESIAN_POINT('',(102.9,6.,48.35));
#90444=CARTESIAN_POINT('',(102.9,6.,48.35));
#90445=CARTESIAN_POINT('',(102.9,6.,48.5));
#90446=CARTESIAN_POINT('Origin',(103.1,7.4,48.5));
#90447=CARTESIAN_POINT('',(103.1,7.4,48.5));
#90448=CARTESIAN_POINT('',(103.1,7.7,48.5));
#90449=CARTESIAN_POINT('',(103.1,7.4,48.35));
#90450=CARTESIAN_POINT('',(103.1,7.4,48.5));
#90451=CARTESIAN_POINT('',(103.1,6.,48.35));
#90452=CARTESIAN_POINT('Origin',(102.9,7.4,48.5));
#90453=CARTESIAN_POINT('',(102.9,7.4,48.5));
#90454=CARTESIAN_POINT('',(51.45,7.4,48.5));
#90455=CARTESIAN_POINT('',(102.9,7.4,48.35));
#90456=CARTESIAN_POINT('',(102.9,7.4,48.5));
#90457=CARTESIAN_POINT('',(103.1,7.4,48.35));
#90458=CARTESIAN_POINT('Origin',(102.9,6.,48.5));
#90459=CARTESIAN_POINT('',(102.9,7.,48.5));
#90460=CARTESIAN_POINT('',(102.9,7.4,48.35));
#90461=CARTESIAN_POINT('Origin',(103.,6.7,48.35));
#90462=CARTESIAN_POINT('Origin',(105.1,5.2,48.5));
#90463=CARTESIAN_POINT('',(105.1,5.2,48.5));
#90464=CARTESIAN_POINT('',(104.9,5.2,48.5));
#90465=CARTESIAN_POINT('',(52.55,5.2,48.5));
#90466=CARTESIAN_POINT('',(105.1,5.2,48.35));
#90467=CARTESIAN_POINT('',(105.1,5.2,48.5));
#90468=CARTESIAN_POINT('',(104.9,5.2,48.35));
#90469=CARTESIAN_POINT('',(104.9,5.2,48.35));
#90470=CARTESIAN_POINT('',(104.9,5.2,48.5));
#90471=CARTESIAN_POINT('Origin',(105.1,7.4,48.5));
#90472=CARTESIAN_POINT('',(105.1,7.4,48.5));
#90473=CARTESIAN_POINT('',(105.1,7.7,48.5));
#90474=CARTESIAN_POINT('',(105.1,7.4,48.35));
#90475=CARTESIAN_POINT('',(105.1,7.4,48.5));
#90476=CARTESIAN_POINT('',(105.1,5.2,48.35));
#90477=CARTESIAN_POINT('Origin',(104.9,7.4,48.5));
#90478=CARTESIAN_POINT('',(104.9,7.4,48.5));
#90479=CARTESIAN_POINT('',(52.45,7.4,48.5));
#90480=CARTESIAN_POINT('',(104.9,7.4,48.35));
#90481=CARTESIAN_POINT('',(104.9,7.4,48.5));
#90482=CARTESIAN_POINT('',(105.1,7.4,48.35));
#90483=CARTESIAN_POINT('Origin',(104.9,5.2,48.5));
#90484=CARTESIAN_POINT('',(104.9,6.6,48.5));
#90485=CARTESIAN_POINT('',(104.9,7.4,48.35));
#90486=CARTESIAN_POINT('Origin',(105.,6.3,48.35));
#90487=CARTESIAN_POINT('Origin',(107.1,6.,48.5));
#90488=CARTESIAN_POINT('',(107.1,6.,48.5));
#90489=CARTESIAN_POINT('',(106.9,6.,48.5));
#90490=CARTESIAN_POINT('',(53.55,6.,48.5));
#90491=CARTESIAN_POINT('',(107.1,6.,48.35));
#90492=CARTESIAN_POINT('',(107.1,6.,48.5));
#90493=CARTESIAN_POINT('',(106.9,6.,48.35));
#90494=CARTESIAN_POINT('',(106.9,6.,48.35));
#90495=CARTESIAN_POINT('',(106.9,6.,48.5));
#90496=CARTESIAN_POINT('Origin',(107.1,7.4,48.5));
#90497=CARTESIAN_POINT('',(107.1,7.4,48.5));
#90498=CARTESIAN_POINT('',(107.1,7.7,48.5));
#90499=CARTESIAN_POINT('',(107.1,7.4,48.35));
#90500=CARTESIAN_POINT('',(107.1,7.4,48.5));
#90501=CARTESIAN_POINT('',(107.1,6.,48.35));
#90502=CARTESIAN_POINT('Origin',(106.9,7.4,48.5));
#90503=CARTESIAN_POINT('',(106.9,7.4,48.5));
#90504=CARTESIAN_POINT('',(53.45,7.4,48.5));
#90505=CARTESIAN_POINT('',(106.9,7.4,48.35));
#90506=CARTESIAN_POINT('',(106.9,7.4,48.5));
#90507=CARTESIAN_POINT('',(107.1,7.4,48.35));
#90508=CARTESIAN_POINT('Origin',(106.9,6.,48.5));
#90509=CARTESIAN_POINT('',(106.9,7.,48.5));
#90510=CARTESIAN_POINT('',(106.9,7.4,48.35));
#90511=CARTESIAN_POINT('Origin',(107.,6.7,48.35));
#90512=CARTESIAN_POINT('Origin',(109.1,6.,48.5));
#90513=CARTESIAN_POINT('',(109.1,6.,48.5));
#90514=CARTESIAN_POINT('',(108.9,6.,48.5));
#90515=CARTESIAN_POINT('',(54.55,6.,48.5));
#90516=CARTESIAN_POINT('',(109.1,6.,48.35));
#90517=CARTESIAN_POINT('',(109.1,6.,48.5));
#90518=CARTESIAN_POINT('',(108.9,6.,48.35));
#90519=CARTESIAN_POINT('',(108.9,6.,48.35));
#90520=CARTESIAN_POINT('',(108.9,6.,48.5));
#90521=CARTESIAN_POINT('Origin',(109.1,7.4,48.5));
#90522=CARTESIAN_POINT('',(109.1,7.4,48.5));
#90523=CARTESIAN_POINT('',(109.1,7.7,48.5));
#90524=CARTESIAN_POINT('',(109.1,7.4,48.35));
#90525=CARTESIAN_POINT('',(109.1,7.4,48.5));
#90526=CARTESIAN_POINT('',(109.1,6.,48.35));
#90527=CARTESIAN_POINT('Origin',(108.9,7.4,48.5));
#90528=CARTESIAN_POINT('',(108.9,7.4,48.5));
#90529=CARTESIAN_POINT('',(54.45,7.4,48.5));
#90530=CARTESIAN_POINT('',(108.9,7.4,48.35));
#90531=CARTESIAN_POINT('',(108.9,7.4,48.5));
#90532=CARTESIAN_POINT('',(109.1,7.4,48.35));
#90533=CARTESIAN_POINT('Origin',(108.9,6.,48.5));
#90534=CARTESIAN_POINT('',(108.9,7.,48.5));
#90535=CARTESIAN_POINT('',(108.9,7.4,48.35));
#90536=CARTESIAN_POINT('Origin',(109.,6.7,48.35));
#90537=CARTESIAN_POINT('Origin',(20.1,4.4,48.5));
#90538=CARTESIAN_POINT('',(20.1,4.4,48.5));
#90539=CARTESIAN_POINT('',(19.9,4.4,48.5));
#90540=CARTESIAN_POINT('',(10.05,4.4,48.5));
#90541=CARTESIAN_POINT('',(20.1,4.4,48.35));
#90542=CARTESIAN_POINT('',(20.1,4.4,48.5));
#90543=CARTESIAN_POINT('',(19.9,4.4,48.35));
#90544=CARTESIAN_POINT('',(19.9,4.4,48.35));
#90545=CARTESIAN_POINT('',(19.9,4.4,48.5));
#90546=CARTESIAN_POINT('Origin',(20.1,7.4,48.5));
#90547=CARTESIAN_POINT('',(20.1,7.4,48.5));
#90548=CARTESIAN_POINT('',(20.1,7.7,48.5));
#90549=CARTESIAN_POINT('',(20.1,7.4,48.35));
#90550=CARTESIAN_POINT('',(20.1,7.4,48.5));
#90551=CARTESIAN_POINT('',(20.1,4.4,48.35));
#90552=CARTESIAN_POINT('Origin',(19.9,7.4,48.5));
#90553=CARTESIAN_POINT('',(19.9,7.4,48.5));
#90554=CARTESIAN_POINT('',(9.95,7.4,48.5));
#90555=CARTESIAN_POINT('',(19.9,7.4,48.35));
#90556=CARTESIAN_POINT('',(19.9,7.4,48.5));
#90557=CARTESIAN_POINT('',(20.1,7.4,48.35));
#90558=CARTESIAN_POINT('Origin',(19.9,4.4,48.5));
#90559=CARTESIAN_POINT('',(19.9,6.2,48.5));
#90560=CARTESIAN_POINT('',(19.9,7.4,48.35));
#90561=CARTESIAN_POINT('Origin',(20.,5.9,48.35));
#90562=CARTESIAN_POINT('Origin',(112.1,6.,48.5));
#90563=CARTESIAN_POINT('',(112.1,6.,48.5));
#90564=CARTESIAN_POINT('',(111.9,6.,48.5));
#90565=CARTESIAN_POINT('',(56.05,6.,48.5));
#90566=CARTESIAN_POINT('',(112.1,6.,48.35));
#90567=CARTESIAN_POINT('',(112.1,6.,48.5));
#90568=CARTESIAN_POINT('',(111.9,6.,48.35));
#90569=CARTESIAN_POINT('',(111.9,6.,48.35));
#90570=CARTESIAN_POINT('',(111.9,6.,48.5));
#90571=CARTESIAN_POINT('Origin',(112.1,7.4,48.5));
#90572=CARTESIAN_POINT('',(112.1,7.4,48.5));
#90573=CARTESIAN_POINT('',(112.1,7.7,48.5));
#90574=CARTESIAN_POINT('',(112.1,7.4,48.35));
#90575=CARTESIAN_POINT('',(112.1,7.4,48.5));
#90576=CARTESIAN_POINT('',(112.1,6.,48.35));
#90577=CARTESIAN_POINT('Origin',(111.9,7.4,48.5));
#90578=CARTESIAN_POINT('',(111.9,7.4,48.5));
#90579=CARTESIAN_POINT('',(55.95,7.4,48.5));
#90580=CARTESIAN_POINT('',(111.9,7.4,48.35));
#90581=CARTESIAN_POINT('',(111.9,7.4,48.5));
#90582=CARTESIAN_POINT('',(112.1,7.4,48.35));
#90583=CARTESIAN_POINT('Origin',(111.9,6.,48.5));
#90584=CARTESIAN_POINT('',(111.9,7.,48.5));
#90585=CARTESIAN_POINT('',(111.9,7.4,48.35));
#90586=CARTESIAN_POINT('Origin',(112.,6.7,48.35));
#90587=CARTESIAN_POINT('Origin',(114.1,6.,48.5));
#90588=CARTESIAN_POINT('',(114.1,6.,48.5));
#90589=CARTESIAN_POINT('',(113.9,6.,48.5));
#90590=CARTESIAN_POINT('',(57.05,6.,48.5));
#90591=CARTESIAN_POINT('',(114.1,6.,48.35));
#90592=CARTESIAN_POINT('',(114.1,6.,48.5));
#90593=CARTESIAN_POINT('',(113.9,6.,48.35));
#90594=CARTESIAN_POINT('',(113.9,6.,48.35));
#90595=CARTESIAN_POINT('',(113.9,6.,48.5));
#90596=CARTESIAN_POINT('Origin',(114.1,7.4,48.5));
#90597=CARTESIAN_POINT('',(114.1,7.4,48.5));
#90598=CARTESIAN_POINT('',(114.1,7.7,48.5));
#90599=CARTESIAN_POINT('',(114.1,7.4,48.35));
#90600=CARTESIAN_POINT('',(114.1,7.4,48.5));
#90601=CARTESIAN_POINT('',(114.1,6.,48.35));
#90602=CARTESIAN_POINT('Origin',(113.9,7.4,48.5));
#90603=CARTESIAN_POINT('',(113.9,7.4,48.5));
#90604=CARTESIAN_POINT('',(56.95,7.4,48.5));
#90605=CARTESIAN_POINT('',(113.9,7.4,48.35));
#90606=CARTESIAN_POINT('',(113.9,7.4,48.5));
#90607=CARTESIAN_POINT('',(114.1,7.4,48.35));
#90608=CARTESIAN_POINT('Origin',(113.9,6.,48.5));
#90609=CARTESIAN_POINT('',(113.9,7.,48.5));
#90610=CARTESIAN_POINT('',(113.9,7.4,48.35));
#90611=CARTESIAN_POINT('Origin',(114.,6.7,48.35));
#90612=CARTESIAN_POINT('Origin',(116.1,6.,48.5));
#90613=CARTESIAN_POINT('',(116.1,6.,48.5));
#90614=CARTESIAN_POINT('',(115.9,6.,48.5));
#90615=CARTESIAN_POINT('',(58.05,6.,48.5));
#90616=CARTESIAN_POINT('',(116.1,6.,48.35));
#90617=CARTESIAN_POINT('',(116.1,6.,48.5));
#90618=CARTESIAN_POINT('',(115.9,6.,48.35));
#90619=CARTESIAN_POINT('',(115.9,6.,48.35));
#90620=CARTESIAN_POINT('',(115.9,6.,48.5));
#90621=CARTESIAN_POINT('Origin',(116.1,7.4,48.5));
#90622=CARTESIAN_POINT('',(116.1,7.4,48.5));
#90623=CARTESIAN_POINT('',(116.1,7.7,48.5));
#90624=CARTESIAN_POINT('',(116.1,7.4,48.35));
#90625=CARTESIAN_POINT('',(116.1,7.4,48.5));
#90626=CARTESIAN_POINT('',(116.1,6.,48.35));
#90627=CARTESIAN_POINT('Origin',(115.9,7.4,48.5));
#90628=CARTESIAN_POINT('',(115.9,7.4,48.5));
#90629=CARTESIAN_POINT('',(57.95,7.4,48.5));
#90630=CARTESIAN_POINT('',(115.9,7.4,48.35));
#90631=CARTESIAN_POINT('',(115.9,7.4,48.5));
#90632=CARTESIAN_POINT('',(116.1,7.4,48.35));
#90633=CARTESIAN_POINT('Origin',(115.9,6.,48.5));
#90634=CARTESIAN_POINT('',(115.9,7.,48.5));
#90635=CARTESIAN_POINT('',(115.9,7.4,48.35));
#90636=CARTESIAN_POINT('Origin',(116.,6.7,48.35));
#90637=CARTESIAN_POINT('Origin',(118.1,6.,48.5));
#90638=CARTESIAN_POINT('',(118.1,6.,48.5));
#90639=CARTESIAN_POINT('',(117.9,6.,48.5));
#90640=CARTESIAN_POINT('',(59.05,6.,48.5));
#90641=CARTESIAN_POINT('',(118.1,6.,48.35));
#90642=CARTESIAN_POINT('',(118.1,6.,48.5));
#90643=CARTESIAN_POINT('',(117.9,6.,48.35));
#90644=CARTESIAN_POINT('',(117.9,6.,48.35));
#90645=CARTESIAN_POINT('',(117.9,6.,48.5));
#90646=CARTESIAN_POINT('Origin',(118.1,7.4,48.5));
#90647=CARTESIAN_POINT('',(118.1,7.4,48.5));
#90648=CARTESIAN_POINT('',(118.1,7.7,48.5));
#90649=CARTESIAN_POINT('',(118.1,7.4,48.35));
#90650=CARTESIAN_POINT('',(118.1,7.4,48.5));
#90651=CARTESIAN_POINT('',(118.1,6.,48.35));
#90652=CARTESIAN_POINT('Origin',(117.9,7.4,48.5));
#90653=CARTESIAN_POINT('',(117.9,7.4,48.5));
#90654=CARTESIAN_POINT('',(58.95,7.4,48.5));
#90655=CARTESIAN_POINT('',(117.9,7.4,48.35));
#90656=CARTESIAN_POINT('',(117.9,7.4,48.5));
#90657=CARTESIAN_POINT('',(118.1,7.4,48.35));
#90658=CARTESIAN_POINT('Origin',(117.9,6.,48.5));
#90659=CARTESIAN_POINT('',(117.9,7.,48.5));
#90660=CARTESIAN_POINT('',(117.9,7.4,48.35));
#90661=CARTESIAN_POINT('Origin',(118.,6.7,48.35));
#90662=CARTESIAN_POINT('Origin',(120.1,4.4,48.5));
#90663=CARTESIAN_POINT('',(120.1,4.4,48.5));
#90664=CARTESIAN_POINT('',(119.9,4.4,48.5));
#90665=CARTESIAN_POINT('',(60.05,4.4,48.5));
#90666=CARTESIAN_POINT('',(120.1,4.4,48.35));
#90667=CARTESIAN_POINT('',(120.1,4.4,48.5));
#90668=CARTESIAN_POINT('',(119.9,4.4,48.35));
#90669=CARTESIAN_POINT('',(119.9,4.4,48.35));
#90670=CARTESIAN_POINT('',(119.9,4.4,48.5));
#90671=CARTESIAN_POINT('Origin',(120.1,7.4,48.5));
#90672=CARTESIAN_POINT('',(120.1,7.4,48.5));
#90673=CARTESIAN_POINT('',(120.1,7.7,48.5));
#90674=CARTESIAN_POINT('',(120.1,7.4,48.35));
#90675=CARTESIAN_POINT('',(120.1,7.4,48.5));
#90676=CARTESIAN_POINT('',(120.1,4.4,48.35));
#90677=CARTESIAN_POINT('Origin',(119.9,7.4,48.5));
#90678=CARTESIAN_POINT('',(119.9,7.4,48.5));
#90679=CARTESIAN_POINT('',(59.95,7.4,48.5));
#90680=CARTESIAN_POINT('',(119.9,7.4,48.35));
#90681=CARTESIAN_POINT('',(119.9,7.4,48.5));
#90682=CARTESIAN_POINT('',(120.1,7.4,48.35));
#90683=CARTESIAN_POINT('Origin',(119.9,4.4,48.5));
#90684=CARTESIAN_POINT('',(119.9,6.2,48.5));
#90685=CARTESIAN_POINT('',(119.9,7.4,48.35));
#90686=CARTESIAN_POINT('Origin',(120.,5.9,48.35));
#90687=CARTESIAN_POINT('Origin',(122.1,6.,48.5));
#90688=CARTESIAN_POINT('',(122.1,6.,48.5));
#90689=CARTESIAN_POINT('',(121.9,6.,48.5));
#90690=CARTESIAN_POINT('',(61.05,6.,48.5));
#90691=CARTESIAN_POINT('',(122.1,6.,48.35));
#90692=CARTESIAN_POINT('',(122.1,6.,48.5));
#90693=CARTESIAN_POINT('',(121.9,6.,48.35));
#90694=CARTESIAN_POINT('',(121.9,6.,48.35));
#90695=CARTESIAN_POINT('',(121.9,6.,48.5));
#90696=CARTESIAN_POINT('Origin',(122.1,7.4,48.5));
#90697=CARTESIAN_POINT('',(122.1,7.4,48.5));
#90698=CARTESIAN_POINT('',(122.1,7.7,48.5));
#90699=CARTESIAN_POINT('',(122.1,7.4,48.35));
#90700=CARTESIAN_POINT('',(122.1,7.4,48.5));
#90701=CARTESIAN_POINT('',(122.1,6.,48.35));
#90702=CARTESIAN_POINT('Origin',(121.9,7.4,48.5));
#90703=CARTESIAN_POINT('',(121.9,7.4,48.5));
#90704=CARTESIAN_POINT('',(60.95,7.4,48.5));
#90705=CARTESIAN_POINT('',(121.9,7.4,48.35));
#90706=CARTESIAN_POINT('',(121.9,7.4,48.5));
#90707=CARTESIAN_POINT('',(122.1,7.4,48.35));
#90708=CARTESIAN_POINT('Origin',(121.9,6.,48.5));
#90709=CARTESIAN_POINT('',(121.9,7.,48.5));
#90710=CARTESIAN_POINT('',(121.9,7.4,48.35));
#90711=CARTESIAN_POINT('Origin',(122.,6.7,48.35));
#90712=CARTESIAN_POINT('Origin',(124.1,6.,48.5));
#90713=CARTESIAN_POINT('',(124.1,6.,48.5));
#90714=CARTESIAN_POINT('',(123.9,6.,48.5));
#90715=CARTESIAN_POINT('',(62.05,6.,48.5));
#90716=CARTESIAN_POINT('',(124.1,6.,48.35));
#90717=CARTESIAN_POINT('',(124.1,6.,48.5));
#90718=CARTESIAN_POINT('',(123.9,6.,48.35));
#90719=CARTESIAN_POINT('',(123.9,6.,48.35));
#90720=CARTESIAN_POINT('',(123.9,6.,48.5));
#90721=CARTESIAN_POINT('Origin',(124.1,7.4,48.5));
#90722=CARTESIAN_POINT('',(124.1,7.4,48.5));
#90723=CARTESIAN_POINT('',(124.1,7.7,48.5));
#90724=CARTESIAN_POINT('',(124.1,7.4,48.35));
#90725=CARTESIAN_POINT('',(124.1,7.4,48.5));
#90726=CARTESIAN_POINT('',(124.1,6.,48.35));
#90727=CARTESIAN_POINT('Origin',(123.9,7.4,48.5));
#90728=CARTESIAN_POINT('',(123.9,7.4,48.5));
#90729=CARTESIAN_POINT('',(61.95,7.4,48.5));
#90730=CARTESIAN_POINT('',(123.9,7.4,48.35));
#90731=CARTESIAN_POINT('',(123.9,7.4,48.5));
#90732=CARTESIAN_POINT('',(124.1,7.4,48.35));
#90733=CARTESIAN_POINT('Origin',(123.9,6.,48.5));
#90734=CARTESIAN_POINT('',(123.9,7.,48.5));
#90735=CARTESIAN_POINT('',(123.9,7.4,48.35));
#90736=CARTESIAN_POINT('Origin',(124.,6.7,48.35));
#90737=CARTESIAN_POINT('Origin',(126.1,6.,48.5));
#90738=CARTESIAN_POINT('',(126.1,6.,48.5));
#90739=CARTESIAN_POINT('',(125.9,6.,48.5));
#90740=CARTESIAN_POINT('',(63.05,6.,48.5));
#90741=CARTESIAN_POINT('',(126.1,6.,48.35));
#90742=CARTESIAN_POINT('',(126.1,6.,48.5));
#90743=CARTESIAN_POINT('',(125.9,6.,48.35));
#90744=CARTESIAN_POINT('',(125.9,6.,48.35));
#90745=CARTESIAN_POINT('',(125.9,6.,48.5));
#90746=CARTESIAN_POINT('Origin',(126.1,7.4,48.5));
#90747=CARTESIAN_POINT('',(126.1,7.4,48.5));
#90748=CARTESIAN_POINT('',(126.1,7.7,48.5));
#90749=CARTESIAN_POINT('',(126.1,7.4,48.35));
#90750=CARTESIAN_POINT('',(126.1,7.4,48.5));
#90751=CARTESIAN_POINT('',(126.1,6.,48.35));
#90752=CARTESIAN_POINT('Origin',(125.9,7.4,48.5));
#90753=CARTESIAN_POINT('',(125.9,7.4,48.5));
#90754=CARTESIAN_POINT('',(62.95,7.4,48.5));
#90755=CARTESIAN_POINT('',(125.9,7.4,48.35));
#90756=CARTESIAN_POINT('',(125.9,7.4,48.5));
#90757=CARTESIAN_POINT('',(126.1,7.4,48.35));
#90758=CARTESIAN_POINT('Origin',(125.9,6.,48.5));
#90759=CARTESIAN_POINT('',(125.9,7.,48.5));
#90760=CARTESIAN_POINT('',(125.9,7.4,48.35));
#90761=CARTESIAN_POINT('Origin',(126.,6.7,48.35));
#90762=CARTESIAN_POINT('Origin',(128.1,6.,48.5));
#90763=CARTESIAN_POINT('',(128.1,6.,48.5));
#90764=CARTESIAN_POINT('',(127.9,6.,48.5));
#90765=CARTESIAN_POINT('',(64.05,6.,48.5));
#90766=CARTESIAN_POINT('',(128.1,6.,48.35));
#90767=CARTESIAN_POINT('',(128.1,6.,48.5));
#90768=CARTESIAN_POINT('',(127.9,6.,48.35));
#90769=CARTESIAN_POINT('',(127.9,6.,48.35));
#90770=CARTESIAN_POINT('',(127.9,6.,48.5));
#90771=CARTESIAN_POINT('Origin',(128.1,7.4,48.5));
#90772=CARTESIAN_POINT('',(128.1,7.4,48.5));
#90773=CARTESIAN_POINT('',(128.1,7.7,48.5));
#90774=CARTESIAN_POINT('',(128.1,7.4,48.35));
#90775=CARTESIAN_POINT('',(128.1,7.4,48.5));
#90776=CARTESIAN_POINT('',(128.1,6.,48.35));
#90777=CARTESIAN_POINT('Origin',(127.9,7.4,48.5));
#90778=CARTESIAN_POINT('',(127.9,7.4,48.5));
#90779=CARTESIAN_POINT('',(63.95,7.4,48.5));
#90780=CARTESIAN_POINT('',(127.9,7.4,48.35));
#90781=CARTESIAN_POINT('',(127.9,7.4,48.5));
#90782=CARTESIAN_POINT('',(128.1,7.4,48.35));
#90783=CARTESIAN_POINT('Origin',(127.9,6.,48.5));
#90784=CARTESIAN_POINT('',(127.9,7.,48.5));
#90785=CARTESIAN_POINT('',(127.9,7.4,48.35));
#90786=CARTESIAN_POINT('Origin',(128.,6.7,48.35));
#90787=CARTESIAN_POINT('Origin',(130.1,4.4,48.5));
#90788=CARTESIAN_POINT('',(130.1,4.4,48.5));
#90789=CARTESIAN_POINT('',(129.9,4.4,48.5));
#90790=CARTESIAN_POINT('',(65.05,4.4,48.5));
#90791=CARTESIAN_POINT('',(130.1,4.4,48.35));
#90792=CARTESIAN_POINT('',(130.1,4.4,48.5));
#90793=CARTESIAN_POINT('',(129.9,4.4,48.35));
#90794=CARTESIAN_POINT('',(129.9,4.4,48.35));
#90795=CARTESIAN_POINT('',(129.9,4.4,48.5));
#90796=CARTESIAN_POINT('Origin',(130.1,7.4,48.5));
#90797=CARTESIAN_POINT('',(130.1,7.4,48.5));
#90798=CARTESIAN_POINT('',(130.1,7.7,48.5));
#90799=CARTESIAN_POINT('',(130.1,7.4,48.35));
#90800=CARTESIAN_POINT('',(130.1,7.4,48.5));
#90801=CARTESIAN_POINT('',(130.1,4.4,48.35));
#90802=CARTESIAN_POINT('Origin',(129.9,7.4,48.5));
#90803=CARTESIAN_POINT('',(129.9,7.4,48.5));
#90804=CARTESIAN_POINT('',(64.95,7.4,48.5));
#90805=CARTESIAN_POINT('',(129.9,7.4,48.35));
#90806=CARTESIAN_POINT('',(129.9,7.4,48.5));
#90807=CARTESIAN_POINT('',(130.1,7.4,48.35));
#90808=CARTESIAN_POINT('Origin',(129.9,4.4,48.5));
#90809=CARTESIAN_POINT('',(129.9,6.2,48.5));
#90810=CARTESIAN_POINT('',(129.9,7.4,48.35));
#90811=CARTESIAN_POINT('Origin',(130.,5.9,48.35));
#90812=CARTESIAN_POINT('Origin',(132.1,6.,48.5));
#90813=CARTESIAN_POINT('',(132.1,6.,48.5));
#90814=CARTESIAN_POINT('',(131.9,6.,48.5));
#90815=CARTESIAN_POINT('',(66.05,6.,48.5));
#90816=CARTESIAN_POINT('',(132.1,6.,48.35));
#90817=CARTESIAN_POINT('',(132.1,6.,48.5));
#90818=CARTESIAN_POINT('',(131.9,6.,48.35));
#90819=CARTESIAN_POINT('',(131.9,6.,48.35));
#90820=CARTESIAN_POINT('',(131.9,6.,48.5));
#90821=CARTESIAN_POINT('Origin',(132.1,7.4,48.5));
#90822=CARTESIAN_POINT('',(132.1,7.4,48.5));
#90823=CARTESIAN_POINT('',(132.1,7.7,48.5));
#90824=CARTESIAN_POINT('',(132.1,7.4,48.35));
#90825=CARTESIAN_POINT('',(132.1,7.4,48.5));
#90826=CARTESIAN_POINT('',(132.1,6.,48.35));
#90827=CARTESIAN_POINT('Origin',(131.9,7.4,48.5));
#90828=CARTESIAN_POINT('',(131.9,7.4,48.5));
#90829=CARTESIAN_POINT('',(65.95,7.4,48.5));
#90830=CARTESIAN_POINT('',(131.9,7.4,48.35));
#90831=CARTESIAN_POINT('',(131.9,7.4,48.5));
#90832=CARTESIAN_POINT('',(132.1,7.4,48.35));
#90833=CARTESIAN_POINT('Origin',(131.9,6.,48.5));
#90834=CARTESIAN_POINT('',(131.9,7.,48.5));
#90835=CARTESIAN_POINT('',(131.9,7.4,48.35));
#90836=CARTESIAN_POINT('Origin',(132.,6.7,48.35));
#90837=CARTESIAN_POINT('Origin',(134.1,6.,48.5));
#90838=CARTESIAN_POINT('',(134.1,6.,48.5));
#90839=CARTESIAN_POINT('',(133.9,6.,48.5));
#90840=CARTESIAN_POINT('',(67.05,6.,48.5));
#90841=CARTESIAN_POINT('',(134.1,6.,48.35));
#90842=CARTESIAN_POINT('',(134.1,6.,48.5));
#90843=CARTESIAN_POINT('',(133.9,6.,48.35));
#90844=CARTESIAN_POINT('',(133.9,6.,48.35));
#90845=CARTESIAN_POINT('',(133.9,6.,48.5));
#90846=CARTESIAN_POINT('Origin',(134.1,7.4,48.5));
#90847=CARTESIAN_POINT('',(134.1,7.4,48.5));
#90848=CARTESIAN_POINT('',(134.1,7.7,48.5));
#90849=CARTESIAN_POINT('',(134.1,7.4,48.35));
#90850=CARTESIAN_POINT('',(134.1,7.4,48.5));
#90851=CARTESIAN_POINT('',(134.1,6.,48.35));
#90852=CARTESIAN_POINT('Origin',(133.9,7.4,48.5));
#90853=CARTESIAN_POINT('',(133.9,7.4,48.5));
#90854=CARTESIAN_POINT('',(66.95,7.4,48.5));
#90855=CARTESIAN_POINT('',(133.9,7.4,48.35));
#90856=CARTESIAN_POINT('',(133.9,7.4,48.5));
#90857=CARTESIAN_POINT('',(134.1,7.4,48.35));
#90858=CARTESIAN_POINT('Origin',(133.9,6.,48.5));
#90859=CARTESIAN_POINT('',(133.9,7.,48.5));
#90860=CARTESIAN_POINT('',(133.9,7.4,48.35));
#90861=CARTESIAN_POINT('Origin',(134.,6.7,48.35));
#90862=CARTESIAN_POINT('Origin',(136.1,6.,48.5));
#90863=CARTESIAN_POINT('',(136.1,6.,48.5));
#90864=CARTESIAN_POINT('',(135.9,6.,48.5));
#90865=CARTESIAN_POINT('',(68.05,6.,48.5));
#90866=CARTESIAN_POINT('',(136.1,6.,48.35));
#90867=CARTESIAN_POINT('',(136.1,6.,48.5));
#90868=CARTESIAN_POINT('',(135.9,6.,48.35));
#90869=CARTESIAN_POINT('',(135.9,6.,48.35));
#90870=CARTESIAN_POINT('',(135.9,6.,48.5));
#90871=CARTESIAN_POINT('Origin',(136.1,7.4,48.5));
#90872=CARTESIAN_POINT('',(136.1,7.4,48.5));
#90873=CARTESIAN_POINT('',(136.1,7.7,48.5));
#90874=CARTESIAN_POINT('',(136.1,7.4,48.35));
#90875=CARTESIAN_POINT('',(136.1,7.4,48.5));
#90876=CARTESIAN_POINT('',(136.1,6.,48.35));
#90877=CARTESIAN_POINT('Origin',(135.9,7.4,48.5));
#90878=CARTESIAN_POINT('',(135.9,7.4,48.5));
#90879=CARTESIAN_POINT('',(67.95,7.4,48.5));
#90880=CARTESIAN_POINT('',(135.9,7.4,48.35));
#90881=CARTESIAN_POINT('',(135.9,7.4,48.5));
#90882=CARTESIAN_POINT('',(136.1,7.4,48.35));
#90883=CARTESIAN_POINT('Origin',(135.9,6.,48.5));
#90884=CARTESIAN_POINT('',(135.9,7.,48.5));
#90885=CARTESIAN_POINT('',(135.9,7.4,48.35));
#90886=CARTESIAN_POINT('Origin',(136.,6.7,48.35));
#90887=CARTESIAN_POINT('Origin',(138.1,6.,48.5));
#90888=CARTESIAN_POINT('',(138.1,6.,48.5));
#90889=CARTESIAN_POINT('',(137.9,6.,48.5));
#90890=CARTESIAN_POINT('',(69.05,6.,48.5));
#90891=CARTESIAN_POINT('',(138.1,6.,48.35));
#90892=CARTESIAN_POINT('',(138.1,6.,48.5));
#90893=CARTESIAN_POINT('',(137.9,6.,48.35));
#90894=CARTESIAN_POINT('',(137.9,6.,48.35));
#90895=CARTESIAN_POINT('',(137.9,6.,48.5));
#90896=CARTESIAN_POINT('Origin',(138.1,7.4,48.5));
#90897=CARTESIAN_POINT('',(138.1,7.4,48.5));
#90898=CARTESIAN_POINT('',(138.1,7.7,48.5));
#90899=CARTESIAN_POINT('',(138.1,7.4,48.35));
#90900=CARTESIAN_POINT('',(138.1,7.4,48.5));
#90901=CARTESIAN_POINT('',(138.1,6.,48.35));
#90902=CARTESIAN_POINT('Origin',(137.9,7.4,48.5));
#90903=CARTESIAN_POINT('',(137.9,7.4,48.5));
#90904=CARTESIAN_POINT('',(68.95,7.4,48.5));
#90905=CARTESIAN_POINT('',(137.9,7.4,48.35));
#90906=CARTESIAN_POINT('',(137.9,7.4,48.5));
#90907=CARTESIAN_POINT('',(138.1,7.4,48.35));
#90908=CARTESIAN_POINT('Origin',(137.9,6.,48.5));
#90909=CARTESIAN_POINT('',(137.9,7.,48.5));
#90910=CARTESIAN_POINT('',(137.9,7.4,48.35));
#90911=CARTESIAN_POINT('Origin',(138.,6.7,48.35));
#90912=CARTESIAN_POINT('Origin',(140.1,4.4,48.5));
#90913=CARTESIAN_POINT('',(140.1,4.4,48.5));
#90914=CARTESIAN_POINT('',(139.9,4.4,48.5));
#90915=CARTESIAN_POINT('',(70.05,4.4,48.5));
#90916=CARTESIAN_POINT('',(140.1,4.4,48.35));
#90917=CARTESIAN_POINT('',(140.1,4.4,48.5));
#90918=CARTESIAN_POINT('',(139.9,4.4,48.35));
#90919=CARTESIAN_POINT('',(139.9,4.4,48.35));
#90920=CARTESIAN_POINT('',(139.9,4.4,48.5));
#90921=CARTESIAN_POINT('Origin',(140.1,7.4,48.5));
#90922=CARTESIAN_POINT('',(140.1,7.4,48.5));
#90923=CARTESIAN_POINT('',(140.1,7.7,48.5));
#90924=CARTESIAN_POINT('',(140.1,7.4,48.35));
#90925=CARTESIAN_POINT('',(140.1,7.4,48.5));
#90926=CARTESIAN_POINT('',(140.1,4.4,48.35));
#90927=CARTESIAN_POINT('Origin',(139.9,7.4,48.5));
#90928=CARTESIAN_POINT('',(139.9,7.4,48.5));
#90929=CARTESIAN_POINT('',(69.95,7.4,48.5));
#90930=CARTESIAN_POINT('',(139.9,7.4,48.35));
#90931=CARTESIAN_POINT('',(139.9,7.4,48.5));
#90932=CARTESIAN_POINT('',(140.1,7.4,48.35));
#90933=CARTESIAN_POINT('Origin',(139.9,4.4,48.5));
#90934=CARTESIAN_POINT('',(139.9,6.2,48.5));
#90935=CARTESIAN_POINT('',(139.9,7.4,48.35));
#90936=CARTESIAN_POINT('Origin',(140.,5.9,48.35));
#90937=CARTESIAN_POINT('Origin',(142.1,6.,48.5));
#90938=CARTESIAN_POINT('',(142.1,6.,48.5));
#90939=CARTESIAN_POINT('',(141.9,6.,48.5));
#90940=CARTESIAN_POINT('',(71.05,6.,48.5));
#90941=CARTESIAN_POINT('',(142.1,6.,48.35));
#90942=CARTESIAN_POINT('',(142.1,6.,48.5));
#90943=CARTESIAN_POINT('',(141.9,6.,48.35));
#90944=CARTESIAN_POINT('',(141.9,6.,48.35));
#90945=CARTESIAN_POINT('',(141.9,6.,48.5));
#90946=CARTESIAN_POINT('Origin',(142.1,7.4,48.5));
#90947=CARTESIAN_POINT('',(142.1,7.4,48.5));
#90948=CARTESIAN_POINT('',(142.1,7.7,48.5));
#90949=CARTESIAN_POINT('',(142.1,7.4,48.35));
#90950=CARTESIAN_POINT('',(142.1,7.4,48.5));
#90951=CARTESIAN_POINT('',(142.1,6.,48.35));
#90952=CARTESIAN_POINT('Origin',(141.9,7.4,48.5));
#90953=CARTESIAN_POINT('',(141.9,7.4,48.5));
#90954=CARTESIAN_POINT('',(70.95,7.4,48.5));
#90955=CARTESIAN_POINT('',(141.9,7.4,48.35));
#90956=CARTESIAN_POINT('',(141.9,7.4,48.5));
#90957=CARTESIAN_POINT('',(142.1,7.4,48.35));
#90958=CARTESIAN_POINT('Origin',(141.9,6.,48.5));
#90959=CARTESIAN_POINT('',(141.9,7.,48.5));
#90960=CARTESIAN_POINT('',(141.9,7.4,48.35));
#90961=CARTESIAN_POINT('Origin',(142.,6.7,48.35));
#90962=CARTESIAN_POINT('Origin',(144.1,6.,48.5));
#90963=CARTESIAN_POINT('',(144.1,6.,48.5));
#90964=CARTESIAN_POINT('',(143.9,6.,48.5));
#90965=CARTESIAN_POINT('',(72.05,6.,48.5));
#90966=CARTESIAN_POINT('',(144.1,6.,48.35));
#90967=CARTESIAN_POINT('',(144.1,6.,48.5));
#90968=CARTESIAN_POINT('',(143.9,6.,48.35));
#90969=CARTESIAN_POINT('',(143.9,6.,48.35));
#90970=CARTESIAN_POINT('',(143.9,6.,48.5));
#90971=CARTESIAN_POINT('Origin',(144.1,7.4,48.5));
#90972=CARTESIAN_POINT('',(144.1,7.4,48.5));
#90973=CARTESIAN_POINT('',(144.1,7.7,48.5));
#90974=CARTESIAN_POINT('',(144.1,7.4,48.35));
#90975=CARTESIAN_POINT('',(144.1,7.4,48.5));
#90976=CARTESIAN_POINT('',(144.1,6.,48.35));
#90977=CARTESIAN_POINT('Origin',(143.9,7.4,48.5));
#90978=CARTESIAN_POINT('',(143.9,7.4,48.5));
#90979=CARTESIAN_POINT('',(71.95,7.4,48.5));
#90980=CARTESIAN_POINT('',(143.9,7.4,48.35));
#90981=CARTESIAN_POINT('',(143.9,7.4,48.5));
#90982=CARTESIAN_POINT('',(144.1,7.4,48.35));
#90983=CARTESIAN_POINT('Origin',(143.9,6.,48.5));
#90984=CARTESIAN_POINT('',(143.9,7.,48.5));
#90985=CARTESIAN_POINT('',(143.9,7.4,48.35));
#90986=CARTESIAN_POINT('Origin',(144.,6.7,48.35));
#90987=CARTESIAN_POINT('Origin',(146.1,6.,48.5));
#90988=CARTESIAN_POINT('',(146.1,6.,48.5));
#90989=CARTESIAN_POINT('',(145.9,6.,48.5));
#90990=CARTESIAN_POINT('',(73.05,6.,48.5));
#90991=CARTESIAN_POINT('',(146.1,6.,48.35));
#90992=CARTESIAN_POINT('',(146.1,6.,48.5));
#90993=CARTESIAN_POINT('',(145.9,6.,48.35));
#90994=CARTESIAN_POINT('',(145.9,6.,48.35));
#90995=CARTESIAN_POINT('',(145.9,6.,48.5));
#90996=CARTESIAN_POINT('Origin',(146.1,7.4,48.5));
#90997=CARTESIAN_POINT('',(146.1,7.4,48.5));
#90998=CARTESIAN_POINT('',(146.1,7.7,48.5));
#90999=CARTESIAN_POINT('',(146.1,7.4,48.35));
#91000=CARTESIAN_POINT('',(146.1,7.4,48.5));
#91001=CARTESIAN_POINT('',(146.1,6.,48.35));
#91002=CARTESIAN_POINT('Origin',(145.9,7.4,48.5));
#91003=CARTESIAN_POINT('',(145.9,7.4,48.5));
#91004=CARTESIAN_POINT('',(72.95,7.4,48.5));
#91005=CARTESIAN_POINT('',(145.9,7.4,48.35));
#91006=CARTESIAN_POINT('',(145.9,7.4,48.5));
#91007=CARTESIAN_POINT('',(146.1,7.4,48.35));
#91008=CARTESIAN_POINT('Origin',(145.9,6.,48.5));
#91009=CARTESIAN_POINT('',(145.9,7.,48.5));
#91010=CARTESIAN_POINT('',(145.9,7.4,48.35));
#91011=CARTESIAN_POINT('Origin',(146.,6.7,48.35));
#91012=CARTESIAN_POINT('Origin',(148.1,6.,48.5));
#91013=CARTESIAN_POINT('',(148.1,6.,48.5));
#91014=CARTESIAN_POINT('',(147.9,6.,48.5));
#91015=CARTESIAN_POINT('',(74.05,6.,48.5));
#91016=CARTESIAN_POINT('',(148.1,6.,48.35));
#91017=CARTESIAN_POINT('',(148.1,6.,48.5));
#91018=CARTESIAN_POINT('',(147.9,6.,48.35));
#91019=CARTESIAN_POINT('',(147.9,6.,48.35));
#91020=CARTESIAN_POINT('',(147.9,6.,48.5));
#91021=CARTESIAN_POINT('Origin',(148.1,7.4,48.5));
#91022=CARTESIAN_POINT('',(148.1,7.4,48.5));
#91023=CARTESIAN_POINT('',(148.1,7.7,48.5));
#91024=CARTESIAN_POINT('',(148.1,7.4,48.35));
#91025=CARTESIAN_POINT('',(148.1,7.4,48.5));
#91026=CARTESIAN_POINT('',(148.1,6.,48.35));
#91027=CARTESIAN_POINT('Origin',(147.9,7.4,48.5));
#91028=CARTESIAN_POINT('',(147.9,7.4,48.5));
#91029=CARTESIAN_POINT('',(73.95,7.4,48.5));
#91030=CARTESIAN_POINT('',(147.9,7.4,48.35));
#91031=CARTESIAN_POINT('',(147.9,7.4,48.5));
#91032=CARTESIAN_POINT('',(148.1,7.4,48.35));
#91033=CARTESIAN_POINT('Origin',(147.9,6.,48.5));
#91034=CARTESIAN_POINT('',(147.9,7.,48.5));
#91035=CARTESIAN_POINT('',(147.9,7.4,48.35));
#91036=CARTESIAN_POINT('Origin',(148.,6.7,48.35));
#91037=CARTESIAN_POINT('Origin',(150.1,4.4,48.5));
#91038=CARTESIAN_POINT('',(150.1,4.4,48.5));
#91039=CARTESIAN_POINT('',(149.9,4.4,48.5));
#91040=CARTESIAN_POINT('',(75.05,4.4,48.5));
#91041=CARTESIAN_POINT('',(150.1,4.4,48.35));
#91042=CARTESIAN_POINT('',(150.1,4.4,48.5));
#91043=CARTESIAN_POINT('',(149.9,4.4,48.35));
#91044=CARTESIAN_POINT('',(149.9,4.4,48.35));
#91045=CARTESIAN_POINT('',(149.9,4.4,48.5));
#91046=CARTESIAN_POINT('Origin',(150.1,7.4,48.5));
#91047=CARTESIAN_POINT('',(150.1,7.4,48.5));
#91048=CARTESIAN_POINT('',(150.1,7.7,48.5));
#91049=CARTESIAN_POINT('',(150.1,7.4,48.35));
#91050=CARTESIAN_POINT('',(150.1,7.4,48.5));
#91051=CARTESIAN_POINT('',(150.1,4.4,48.35));
#91052=CARTESIAN_POINT('Origin',(149.9,7.4,48.5));
#91053=CARTESIAN_POINT('',(149.9,7.4,48.5));
#91054=CARTESIAN_POINT('',(74.95,7.4,48.5));
#91055=CARTESIAN_POINT('',(149.9,7.4,48.35));
#91056=CARTESIAN_POINT('',(149.9,7.4,48.5));
#91057=CARTESIAN_POINT('',(150.1,7.4,48.35));
#91058=CARTESIAN_POINT('Origin',(149.9,4.4,48.5));
#91059=CARTESIAN_POINT('',(149.9,6.2,48.5));
#91060=CARTESIAN_POINT('',(149.9,7.4,48.35));
#91061=CARTESIAN_POINT('Origin',(150.,5.9,48.35));
#91062=CARTESIAN_POINT('Origin',(152.1,6.,48.5));
#91063=CARTESIAN_POINT('',(152.1,6.,48.5));
#91064=CARTESIAN_POINT('',(151.9,6.,48.5));
#91065=CARTESIAN_POINT('',(76.05,6.,48.5));
#91066=CARTESIAN_POINT('',(152.1,6.,48.35));
#91067=CARTESIAN_POINT('',(152.1,6.,48.5));
#91068=CARTESIAN_POINT('',(151.9,6.,48.35));
#91069=CARTESIAN_POINT('',(151.9,6.,48.35));
#91070=CARTESIAN_POINT('',(151.9,6.,48.5));
#91071=CARTESIAN_POINT('Origin',(152.1,7.4,48.5));
#91072=CARTESIAN_POINT('',(152.1,7.4,48.5));
#91073=CARTESIAN_POINT('',(152.1,7.7,48.5));
#91074=CARTESIAN_POINT('',(152.1,7.4,48.35));
#91075=CARTESIAN_POINT('',(152.1,7.4,48.5));
#91076=CARTESIAN_POINT('',(152.1,6.,48.35));
#91077=CARTESIAN_POINT('Origin',(151.9,7.4,48.5));
#91078=CARTESIAN_POINT('',(151.9,7.4,48.5));
#91079=CARTESIAN_POINT('',(75.95,7.4,48.5));
#91080=CARTESIAN_POINT('',(151.9,7.4,48.35));
#91081=CARTESIAN_POINT('',(151.9,7.4,48.5));
#91082=CARTESIAN_POINT('',(152.1,7.4,48.35));
#91083=CARTESIAN_POINT('Origin',(151.9,6.,48.5));
#91084=CARTESIAN_POINT('',(151.9,7.,48.5));
#91085=CARTESIAN_POINT('',(151.9,7.4,48.35));
#91086=CARTESIAN_POINT('Origin',(152.,6.7,48.35));
#91087=CARTESIAN_POINT('Origin',(154.1,6.,48.5));
#91088=CARTESIAN_POINT('',(154.1,6.,48.5));
#91089=CARTESIAN_POINT('',(153.9,6.,48.5));
#91090=CARTESIAN_POINT('',(77.05,6.,48.5));
#91091=CARTESIAN_POINT('',(154.1,6.,48.35));
#91092=CARTESIAN_POINT('',(154.1,6.,48.5));
#91093=CARTESIAN_POINT('',(153.9,6.,48.35));
#91094=CARTESIAN_POINT('',(153.9,6.,48.35));
#91095=CARTESIAN_POINT('',(153.9,6.,48.5));
#91096=CARTESIAN_POINT('Origin',(154.1,7.4,48.5));
#91097=CARTESIAN_POINT('',(154.1,7.4,48.5));
#91098=CARTESIAN_POINT('',(154.1,7.7,48.5));
#91099=CARTESIAN_POINT('',(154.1,7.4,48.35));
#91100=CARTESIAN_POINT('',(154.1,7.4,48.5));
#91101=CARTESIAN_POINT('',(154.1,6.,48.35));
#91102=CARTESIAN_POINT('Origin',(153.9,7.4,48.5));
#91103=CARTESIAN_POINT('',(153.9,7.4,48.5));
#91104=CARTESIAN_POINT('',(76.95,7.4,48.5));
#91105=CARTESIAN_POINT('',(153.9,7.4,48.35));
#91106=CARTESIAN_POINT('',(153.9,7.4,48.5));
#91107=CARTESIAN_POINT('',(154.1,7.4,48.35));
#91108=CARTESIAN_POINT('Origin',(153.9,6.,48.5));
#91109=CARTESIAN_POINT('',(153.9,7.,48.5));
#91110=CARTESIAN_POINT('',(153.9,7.4,48.35));
#91111=CARTESIAN_POINT('Origin',(154.,6.7,48.35));
#91112=CARTESIAN_POINT('Origin',(156.1,6.,48.5));
#91113=CARTESIAN_POINT('',(156.1,6.,48.5));
#91114=CARTESIAN_POINT('',(155.9,6.,48.5));
#91115=CARTESIAN_POINT('',(78.05,6.,48.5));
#91116=CARTESIAN_POINT('',(156.1,6.,48.35));
#91117=CARTESIAN_POINT('',(156.1,6.,48.5));
#91118=CARTESIAN_POINT('',(155.9,6.,48.35));
#91119=CARTESIAN_POINT('',(155.9,6.,48.35));
#91120=CARTESIAN_POINT('',(155.9,6.,48.5));
#91121=CARTESIAN_POINT('Origin',(156.1,7.4,48.5));
#91122=CARTESIAN_POINT('',(156.1,7.4,48.5));
#91123=CARTESIAN_POINT('',(156.1,7.7,48.5));
#91124=CARTESIAN_POINT('',(156.1,7.4,48.35));
#91125=CARTESIAN_POINT('',(156.1,7.4,48.5));
#91126=CARTESIAN_POINT('',(156.1,6.,48.35));
#91127=CARTESIAN_POINT('Origin',(155.9,7.4,48.5));
#91128=CARTESIAN_POINT('',(155.9,7.4,48.5));
#91129=CARTESIAN_POINT('',(77.95,7.4,48.5));
#91130=CARTESIAN_POINT('',(155.9,7.4,48.35));
#91131=CARTESIAN_POINT('',(155.9,7.4,48.5));
#91132=CARTESIAN_POINT('',(156.1,7.4,48.35));
#91133=CARTESIAN_POINT('Origin',(155.9,6.,48.5));
#91134=CARTESIAN_POINT('',(155.9,7.,48.5));
#91135=CARTESIAN_POINT('',(155.9,7.4,48.35));
#91136=CARTESIAN_POINT('Origin',(156.,6.7,48.35));
#91137=CARTESIAN_POINT('Origin',(158.1,6.,48.5));
#91138=CARTESIAN_POINT('',(158.1,6.,48.5));
#91139=CARTESIAN_POINT('',(157.9,6.,48.5));
#91140=CARTESIAN_POINT('',(79.05,6.,48.5));
#91141=CARTESIAN_POINT('',(158.1,6.,48.35));
#91142=CARTESIAN_POINT('',(158.1,6.,48.5));
#91143=CARTESIAN_POINT('',(157.9,6.,48.35));
#91144=CARTESIAN_POINT('',(157.9,6.,48.35));
#91145=CARTESIAN_POINT('',(157.9,6.,48.5));
#91146=CARTESIAN_POINT('Origin',(158.1,7.4,48.5));
#91147=CARTESIAN_POINT('',(158.1,7.4,48.5));
#91148=CARTESIAN_POINT('',(158.1,7.7,48.5));
#91149=CARTESIAN_POINT('',(158.1,7.4,48.35));
#91150=CARTESIAN_POINT('',(158.1,7.4,48.5));
#91151=CARTESIAN_POINT('',(158.1,6.,48.35));
#91152=CARTESIAN_POINT('Origin',(157.9,7.4,48.5));
#91153=CARTESIAN_POINT('',(157.9,7.4,48.5));
#91154=CARTESIAN_POINT('',(78.95,7.4,48.5));
#91155=CARTESIAN_POINT('',(157.9,7.4,48.35));
#91156=CARTESIAN_POINT('',(157.9,7.4,48.5));
#91157=CARTESIAN_POINT('',(158.1,7.4,48.35));
#91158=CARTESIAN_POINT('Origin',(157.9,6.,48.5));
#91159=CARTESIAN_POINT('',(157.9,7.,48.5));
#91160=CARTESIAN_POINT('',(157.9,7.4,48.35));
#91161=CARTESIAN_POINT('Origin',(158.,6.7,48.35));
#91162=CARTESIAN_POINT('Origin',(160.1,4.4,48.5));
#91163=CARTESIAN_POINT('',(160.1,4.4,48.5));
#91164=CARTESIAN_POINT('',(159.9,4.4,48.5));
#91165=CARTESIAN_POINT('',(80.05,4.4,48.5));
#91166=CARTESIAN_POINT('',(160.1,4.4,48.35));
#91167=CARTESIAN_POINT('',(160.1,4.4,48.5));
#91168=CARTESIAN_POINT('',(159.9,4.4,48.35));
#91169=CARTESIAN_POINT('',(159.9,4.4,48.35));
#91170=CARTESIAN_POINT('',(159.9,4.4,48.5));
#91171=CARTESIAN_POINT('Origin',(160.1,7.4,48.5));
#91172=CARTESIAN_POINT('',(160.1,7.4,48.5));
#91173=CARTESIAN_POINT('',(160.1,7.7,48.5));
#91174=CARTESIAN_POINT('',(160.1,7.4,48.35));
#91175=CARTESIAN_POINT('',(160.1,7.4,48.5));
#91176=CARTESIAN_POINT('',(160.1,4.4,48.35));
#91177=CARTESIAN_POINT('Origin',(159.9,7.4,48.5));
#91178=CARTESIAN_POINT('',(159.9,7.4,48.5));
#91179=CARTESIAN_POINT('',(79.95,7.4,48.5));
#91180=CARTESIAN_POINT('',(159.9,7.4,48.35));
#91181=CARTESIAN_POINT('',(159.9,7.4,48.5));
#91182=CARTESIAN_POINT('',(160.1,7.4,48.35));
#91183=CARTESIAN_POINT('Origin',(159.9,4.4,48.5));
#91184=CARTESIAN_POINT('',(159.9,6.2,48.5));
#91185=CARTESIAN_POINT('',(159.9,7.4,48.35));
#91186=CARTESIAN_POINT('Origin',(160.,5.9,48.35));
#91187=CARTESIAN_POINT('Origin',(162.1,6.,48.5));
#91188=CARTESIAN_POINT('',(162.1,6.,48.5));
#91189=CARTESIAN_POINT('',(161.9,6.,48.5));
#91190=CARTESIAN_POINT('',(81.05,6.,48.5));
#91191=CARTESIAN_POINT('',(162.1,6.,48.35));
#91192=CARTESIAN_POINT('',(162.1,6.,48.5));
#91193=CARTESIAN_POINT('',(161.9,6.,48.35));
#91194=CARTESIAN_POINT('',(161.9,6.,48.35));
#91195=CARTESIAN_POINT('',(161.9,6.,48.5));
#91196=CARTESIAN_POINT('Origin',(162.1,7.4,48.5));
#91197=CARTESIAN_POINT('',(162.1,7.4,48.5));
#91198=CARTESIAN_POINT('',(162.1,7.7,48.5));
#91199=CARTESIAN_POINT('',(162.1,7.4,48.35));
#91200=CARTESIAN_POINT('',(162.1,7.4,48.5));
#91201=CARTESIAN_POINT('',(162.1,6.,48.35));
#91202=CARTESIAN_POINT('Origin',(161.9,7.4,48.5));
#91203=CARTESIAN_POINT('',(161.9,7.4,48.5));
#91204=CARTESIAN_POINT('',(80.95,7.4,48.5));
#91205=CARTESIAN_POINT('',(161.9,7.4,48.35));
#91206=CARTESIAN_POINT('',(161.9,7.4,48.5));
#91207=CARTESIAN_POINT('',(162.1,7.4,48.35));
#91208=CARTESIAN_POINT('Origin',(161.9,6.,48.5));
#91209=CARTESIAN_POINT('',(161.9,7.,48.5));
#91210=CARTESIAN_POINT('',(161.9,7.4,48.35));
#91211=CARTESIAN_POINT('Origin',(162.,6.7,48.35));
#91212=CARTESIAN_POINT('Origin',(164.1,6.,48.5));
#91213=CARTESIAN_POINT('',(164.1,6.,48.5));
#91214=CARTESIAN_POINT('',(163.9,6.,48.5));
#91215=CARTESIAN_POINT('',(82.05,6.,48.5));
#91216=CARTESIAN_POINT('',(164.1,6.,48.35));
#91217=CARTESIAN_POINT('',(164.1,6.,48.5));
#91218=CARTESIAN_POINT('',(163.9,6.,48.35));
#91219=CARTESIAN_POINT('',(163.9,6.,48.35));
#91220=CARTESIAN_POINT('',(163.9,6.,48.5));
#91221=CARTESIAN_POINT('Origin',(164.1,7.4,48.5));
#91222=CARTESIAN_POINT('',(164.1,7.4,48.5));
#91223=CARTESIAN_POINT('',(164.1,7.7,48.5));
#91224=CARTESIAN_POINT('',(164.1,7.4,48.35));
#91225=CARTESIAN_POINT('',(164.1,7.4,48.5));
#91226=CARTESIAN_POINT('',(164.1,6.,48.35));
#91227=CARTESIAN_POINT('Origin',(163.9,7.4,48.5));
#91228=CARTESIAN_POINT('',(163.9,7.4,48.5));
#91229=CARTESIAN_POINT('',(81.95,7.4,48.5));
#91230=CARTESIAN_POINT('',(163.9,7.4,48.35));
#91231=CARTESIAN_POINT('',(163.9,7.4,48.5));
#91232=CARTESIAN_POINT('',(164.1,7.4,48.35));
#91233=CARTESIAN_POINT('Origin',(163.9,6.,48.5));
#91234=CARTESIAN_POINT('',(163.9,7.,48.5));
#91235=CARTESIAN_POINT('',(163.9,7.4,48.35));
#91236=CARTESIAN_POINT('Origin',(164.,6.7,48.35));
#91237=CARTESIAN_POINT('Origin',(166.1,6.,48.5));
#91238=CARTESIAN_POINT('',(166.1,6.,48.5));
#91239=CARTESIAN_POINT('',(165.9,6.,48.5));
#91240=CARTESIAN_POINT('',(83.05,6.,48.5));
#91241=CARTESIAN_POINT('',(166.1,6.,48.35));
#91242=CARTESIAN_POINT('',(166.1,6.,48.5));
#91243=CARTESIAN_POINT('',(165.9,6.,48.35));
#91244=CARTESIAN_POINT('',(165.9,6.,48.35));
#91245=CARTESIAN_POINT('',(165.9,6.,48.5));
#91246=CARTESIAN_POINT('Origin',(166.1,7.4,48.5));
#91247=CARTESIAN_POINT('',(166.1,7.4,48.5));
#91248=CARTESIAN_POINT('',(166.1,7.7,48.5));
#91249=CARTESIAN_POINT('',(166.1,7.4,48.35));
#91250=CARTESIAN_POINT('',(166.1,7.4,48.5));
#91251=CARTESIAN_POINT('',(166.1,6.,48.35));
#91252=CARTESIAN_POINT('Origin',(165.9,7.4,48.5));
#91253=CARTESIAN_POINT('',(165.9,7.4,48.5));
#91254=CARTESIAN_POINT('',(82.95,7.4,48.5));
#91255=CARTESIAN_POINT('',(165.9,7.4,48.35));
#91256=CARTESIAN_POINT('',(165.9,7.4,48.5));
#91257=CARTESIAN_POINT('',(166.1,7.4,48.35));
#91258=CARTESIAN_POINT('Origin',(165.9,6.,48.5));
#91259=CARTESIAN_POINT('',(165.9,7.,48.5));
#91260=CARTESIAN_POINT('',(165.9,7.4,48.35));
#91261=CARTESIAN_POINT('Origin',(166.,6.7,48.35));
#91262=CARTESIAN_POINT('Origin',(168.1,6.,48.5));
#91263=CARTESIAN_POINT('',(168.1,6.,48.5));
#91264=CARTESIAN_POINT('',(167.9,6.,48.5));
#91265=CARTESIAN_POINT('',(84.05,6.,48.5));
#91266=CARTESIAN_POINT('',(168.1,6.,48.35));
#91267=CARTESIAN_POINT('',(168.1,6.,48.5));
#91268=CARTESIAN_POINT('',(167.9,6.,48.35));
#91269=CARTESIAN_POINT('',(167.9,6.,48.35));
#91270=CARTESIAN_POINT('',(167.9,6.,48.5));
#91271=CARTESIAN_POINT('Origin',(168.1,7.4,48.5));
#91272=CARTESIAN_POINT('',(168.1,7.4,48.5));
#91273=CARTESIAN_POINT('',(168.1,7.7,48.5));
#91274=CARTESIAN_POINT('',(168.1,7.4,48.35));
#91275=CARTESIAN_POINT('',(168.1,7.4,48.5));
#91276=CARTESIAN_POINT('',(168.1,6.,48.35));
#91277=CARTESIAN_POINT('Origin',(167.9,7.4,48.5));
#91278=CARTESIAN_POINT('',(167.9,7.4,48.5));
#91279=CARTESIAN_POINT('',(83.95,7.4,48.5));
#91280=CARTESIAN_POINT('',(167.9,7.4,48.35));
#91281=CARTESIAN_POINT('',(167.9,7.4,48.5));
#91282=CARTESIAN_POINT('',(168.1,7.4,48.35));
#91283=CARTESIAN_POINT('Origin',(167.9,6.,48.5));
#91284=CARTESIAN_POINT('',(167.9,7.,48.5));
#91285=CARTESIAN_POINT('',(167.9,7.4,48.35));
#91286=CARTESIAN_POINT('Origin',(168.,6.7,48.35));
#91287=CARTESIAN_POINT('Origin',(170.1,4.4,48.5));
#91288=CARTESIAN_POINT('',(170.1,4.4,48.5));
#91289=CARTESIAN_POINT('',(169.9,4.4,48.5));
#91290=CARTESIAN_POINT('',(85.05,4.4,48.5));
#91291=CARTESIAN_POINT('',(170.1,4.4,48.35));
#91292=CARTESIAN_POINT('',(170.1,4.4,48.5));
#91293=CARTESIAN_POINT('',(169.9,4.4,48.35));
#91294=CARTESIAN_POINT('',(169.9,4.4,48.35));
#91295=CARTESIAN_POINT('',(169.9,4.4,48.5));
#91296=CARTESIAN_POINT('Origin',(170.1,7.4,48.5));
#91297=CARTESIAN_POINT('',(170.1,7.4,48.5));
#91298=CARTESIAN_POINT('',(170.1,7.7,48.5));
#91299=CARTESIAN_POINT('',(170.1,7.4,48.35));
#91300=CARTESIAN_POINT('',(170.1,7.4,48.5));
#91301=CARTESIAN_POINT('',(170.1,4.4,48.35));
#91302=CARTESIAN_POINT('Origin',(169.9,7.4,48.5));
#91303=CARTESIAN_POINT('',(169.9,7.4,48.5));
#91304=CARTESIAN_POINT('',(84.95,7.4,48.5));
#91305=CARTESIAN_POINT('',(169.9,7.4,48.35));
#91306=CARTESIAN_POINT('',(169.9,7.4,48.5));
#91307=CARTESIAN_POINT('',(170.1,7.4,48.35));
#91308=CARTESIAN_POINT('Origin',(169.9,4.4,48.5));
#91309=CARTESIAN_POINT('',(169.9,6.2,48.5));
#91310=CARTESIAN_POINT('',(169.9,7.4,48.35));
#91311=CARTESIAN_POINT('Origin',(170.,5.9,48.35));
#91312=CARTESIAN_POINT('Origin',(172.1,6.,48.5));
#91313=CARTESIAN_POINT('',(172.1,6.,48.5));
#91314=CARTESIAN_POINT('',(171.9,6.,48.5));
#91315=CARTESIAN_POINT('',(86.05,6.,48.5));
#91316=CARTESIAN_POINT('',(172.1,6.,48.35));
#91317=CARTESIAN_POINT('',(172.1,6.,48.5));
#91318=CARTESIAN_POINT('',(171.9,6.,48.35));
#91319=CARTESIAN_POINT('',(171.9,6.,48.35));
#91320=CARTESIAN_POINT('',(171.9,6.,48.5));
#91321=CARTESIAN_POINT('Origin',(172.1,7.4,48.5));
#91322=CARTESIAN_POINT('',(172.1,7.4,48.5));
#91323=CARTESIAN_POINT('',(172.1,7.7,48.5));
#91324=CARTESIAN_POINT('',(172.1,7.4,48.35));
#91325=CARTESIAN_POINT('',(172.1,7.4,48.5));
#91326=CARTESIAN_POINT('',(172.1,6.,48.35));
#91327=CARTESIAN_POINT('Origin',(171.9,7.4,48.5));
#91328=CARTESIAN_POINT('',(171.9,7.4,48.5));
#91329=CARTESIAN_POINT('',(85.95,7.4,48.5));
#91330=CARTESIAN_POINT('',(171.9,7.4,48.35));
#91331=CARTESIAN_POINT('',(171.9,7.4,48.5));
#91332=CARTESIAN_POINT('',(172.1,7.4,48.35));
#91333=CARTESIAN_POINT('Origin',(171.9,6.,48.5));
#91334=CARTESIAN_POINT('',(171.9,7.,48.5));
#91335=CARTESIAN_POINT('',(171.9,7.4,48.35));
#91336=CARTESIAN_POINT('Origin',(172.,6.7,48.35));
#91337=CARTESIAN_POINT('Origin',(174.1,6.,48.5));
#91338=CARTESIAN_POINT('',(174.1,6.,48.5));
#91339=CARTESIAN_POINT('',(173.9,6.,48.5));
#91340=CARTESIAN_POINT('',(87.05,6.,48.5));
#91341=CARTESIAN_POINT('',(174.1,6.,48.35));
#91342=CARTESIAN_POINT('',(174.1,6.,48.5));
#91343=CARTESIAN_POINT('',(173.9,6.,48.35));
#91344=CARTESIAN_POINT('',(173.9,6.,48.35));
#91345=CARTESIAN_POINT('',(173.9,6.,48.5));
#91346=CARTESIAN_POINT('Origin',(174.1,7.4,48.5));
#91347=CARTESIAN_POINT('',(174.1,7.4,48.5));
#91348=CARTESIAN_POINT('',(174.1,7.7,48.5));
#91349=CARTESIAN_POINT('',(174.1,7.4,48.35));
#91350=CARTESIAN_POINT('',(174.1,7.4,48.5));
#91351=CARTESIAN_POINT('',(174.1,6.,48.35));
#91352=CARTESIAN_POINT('Origin',(173.9,7.4,48.5));
#91353=CARTESIAN_POINT('',(173.9,7.4,48.5));
#91354=CARTESIAN_POINT('',(86.95,7.4,48.5));
#91355=CARTESIAN_POINT('',(173.9,7.4,48.35));
#91356=CARTESIAN_POINT('',(173.9,7.4,48.5));
#91357=CARTESIAN_POINT('',(174.1,7.4,48.35));
#91358=CARTESIAN_POINT('Origin',(173.9,6.,48.5));
#91359=CARTESIAN_POINT('',(173.9,7.,48.5));
#91360=CARTESIAN_POINT('',(173.9,7.4,48.35));
#91361=CARTESIAN_POINT('Origin',(174.,6.7,48.35));
#91362=CARTESIAN_POINT('Origin',(176.1,6.,48.5));
#91363=CARTESIAN_POINT('',(176.1,6.,48.5));
#91364=CARTESIAN_POINT('',(175.9,6.,48.5));
#91365=CARTESIAN_POINT('',(88.05,6.,48.5));
#91366=CARTESIAN_POINT('',(176.1,6.,48.35));
#91367=CARTESIAN_POINT('',(176.1,6.,48.5));
#91368=CARTESIAN_POINT('',(175.9,6.,48.35));
#91369=CARTESIAN_POINT('',(175.9,6.,48.35));
#91370=CARTESIAN_POINT('',(175.9,6.,48.5));
#91371=CARTESIAN_POINT('Origin',(176.1,7.4,48.5));
#91372=CARTESIAN_POINT('',(176.1,7.4,48.5));
#91373=CARTESIAN_POINT('',(176.1,7.7,48.5));
#91374=CARTESIAN_POINT('',(176.1,7.4,48.35));
#91375=CARTESIAN_POINT('',(176.1,7.4,48.5));
#91376=CARTESIAN_POINT('',(176.1,6.,48.35));
#91377=CARTESIAN_POINT('Origin',(175.9,7.4,48.5));
#91378=CARTESIAN_POINT('',(175.9,7.4,48.5));
#91379=CARTESIAN_POINT('',(87.95,7.4,48.5));
#91380=CARTESIAN_POINT('',(175.9,7.4,48.35));
#91381=CARTESIAN_POINT('',(175.9,7.4,48.5));
#91382=CARTESIAN_POINT('',(176.1,7.4,48.35));
#91383=CARTESIAN_POINT('Origin',(175.9,6.,48.5));
#91384=CARTESIAN_POINT('',(175.9,7.,48.5));
#91385=CARTESIAN_POINT('',(175.9,7.4,48.35));
#91386=CARTESIAN_POINT('Origin',(176.,6.7,48.35));
#91387=CARTESIAN_POINT('Origin',(178.1,6.,48.5));
#91388=CARTESIAN_POINT('',(178.1,6.,48.5));
#91389=CARTESIAN_POINT('',(177.9,6.,48.5));
#91390=CARTESIAN_POINT('',(89.05,6.,48.5));
#91391=CARTESIAN_POINT('',(178.1,6.,48.35));
#91392=CARTESIAN_POINT('',(178.1,6.,48.5));
#91393=CARTESIAN_POINT('',(177.9,6.,48.35));
#91394=CARTESIAN_POINT('',(177.9,6.,48.35));
#91395=CARTESIAN_POINT('',(177.9,6.,48.5));
#91396=CARTESIAN_POINT('Origin',(178.1,7.4,48.5));
#91397=CARTESIAN_POINT('',(178.1,7.4,48.5));
#91398=CARTESIAN_POINT('',(178.1,7.7,48.5));
#91399=CARTESIAN_POINT('',(178.1,7.4,48.35));
#91400=CARTESIAN_POINT('',(178.1,7.4,48.5));
#91401=CARTESIAN_POINT('',(178.1,6.,48.35));
#91402=CARTESIAN_POINT('Origin',(177.9,7.4,48.5));
#91403=CARTESIAN_POINT('',(177.9,7.4,48.5));
#91404=CARTESIAN_POINT('',(88.95,7.4,48.5));
#91405=CARTESIAN_POINT('',(177.9,7.4,48.35));
#91406=CARTESIAN_POINT('',(177.9,7.4,48.5));
#91407=CARTESIAN_POINT('',(178.1,7.4,48.35));
#91408=CARTESIAN_POINT('Origin',(177.9,6.,48.5));
#91409=CARTESIAN_POINT('',(177.9,7.,48.5));
#91410=CARTESIAN_POINT('',(177.9,7.4,48.35));
#91411=CARTESIAN_POINT('Origin',(178.,6.7,48.35));
#91412=CARTESIAN_POINT('Origin',(180.1,4.4,48.5));
#91413=CARTESIAN_POINT('',(180.1,4.4,48.5));
#91414=CARTESIAN_POINT('',(179.9,4.4,48.5));
#91415=CARTESIAN_POINT('',(90.05,4.4,48.5));
#91416=CARTESIAN_POINT('',(180.1,4.4,48.35));
#91417=CARTESIAN_POINT('',(180.1,4.4,48.5));
#91418=CARTESIAN_POINT('',(179.9,4.4,48.35));
#91419=CARTESIAN_POINT('',(179.9,4.4,48.35));
#91420=CARTESIAN_POINT('',(179.9,4.4,48.5));
#91421=CARTESIAN_POINT('Origin',(180.1,7.4,48.5));
#91422=CARTESIAN_POINT('',(180.1,7.4,48.5));
#91423=CARTESIAN_POINT('',(180.1,7.7,48.5));
#91424=CARTESIAN_POINT('',(180.1,7.4,48.35));
#91425=CARTESIAN_POINT('',(180.1,7.4,48.5));
#91426=CARTESIAN_POINT('',(180.1,4.4,48.35));
#91427=CARTESIAN_POINT('Origin',(179.9,7.4,48.5));
#91428=CARTESIAN_POINT('',(179.9,7.4,48.5));
#91429=CARTESIAN_POINT('',(89.95,7.4,48.5));
#91430=CARTESIAN_POINT('',(179.9,7.4,48.35));
#91431=CARTESIAN_POINT('',(179.9,7.4,48.5));
#91432=CARTESIAN_POINT('',(180.1,7.4,48.35));
#91433=CARTESIAN_POINT('Origin',(179.9,4.4,48.5));
#91434=CARTESIAN_POINT('',(179.9,6.2,48.5));
#91435=CARTESIAN_POINT('',(179.9,7.4,48.35));
#91436=CARTESIAN_POINT('Origin',(180.,5.9,48.35));
#91437=CARTESIAN_POINT('Origin',(182.1,6.,48.5));
#91438=CARTESIAN_POINT('',(182.1,6.,48.5));
#91439=CARTESIAN_POINT('',(181.9,6.,48.5));
#91440=CARTESIAN_POINT('',(91.05,6.,48.5));
#91441=CARTESIAN_POINT('',(182.1,6.,48.35));
#91442=CARTESIAN_POINT('',(182.1,6.,48.5));
#91443=CARTESIAN_POINT('',(181.9,6.,48.35));
#91444=CARTESIAN_POINT('',(181.9,6.,48.35));
#91445=CARTESIAN_POINT('',(181.9,6.,48.5));
#91446=CARTESIAN_POINT('Origin',(182.1,7.4,48.5));
#91447=CARTESIAN_POINT('',(182.1,7.4,48.5));
#91448=CARTESIAN_POINT('',(182.1,7.7,48.5));
#91449=CARTESIAN_POINT('',(182.1,7.4,48.35));
#91450=CARTESIAN_POINT('',(182.1,7.4,48.5));
#91451=CARTESIAN_POINT('',(182.1,6.,48.35));
#91452=CARTESIAN_POINT('Origin',(181.9,7.4,48.5));
#91453=CARTESIAN_POINT('',(181.9,7.4,48.5));
#91454=CARTESIAN_POINT('',(90.95,7.4,48.5));
#91455=CARTESIAN_POINT('',(181.9,7.4,48.35));
#91456=CARTESIAN_POINT('',(181.9,7.4,48.5));
#91457=CARTESIAN_POINT('',(182.1,7.4,48.35));
#91458=CARTESIAN_POINT('Origin',(181.9,6.,48.5));
#91459=CARTESIAN_POINT('',(181.9,7.,48.5));
#91460=CARTESIAN_POINT('',(181.9,7.4,48.35));
#91461=CARTESIAN_POINT('Origin',(182.,6.7,48.35));
#91462=CARTESIAN_POINT('Origin',(184.1,6.,48.5));
#91463=CARTESIAN_POINT('',(184.1,6.,48.5));
#91464=CARTESIAN_POINT('',(183.9,6.,48.5));
#91465=CARTESIAN_POINT('',(92.05,6.,48.5));
#91466=CARTESIAN_POINT('',(184.1,6.,48.35));
#91467=CARTESIAN_POINT('',(184.1,6.,48.5));
#91468=CARTESIAN_POINT('',(183.9,6.,48.35));
#91469=CARTESIAN_POINT('',(183.9,6.,48.35));
#91470=CARTESIAN_POINT('',(183.9,6.,48.5));
#91471=CARTESIAN_POINT('Origin',(184.1,7.4,48.5));
#91472=CARTESIAN_POINT('',(184.1,7.4,48.5));
#91473=CARTESIAN_POINT('',(184.1,7.7,48.5));
#91474=CARTESIAN_POINT('',(184.1,7.4,48.35));
#91475=CARTESIAN_POINT('',(184.1,7.4,48.5));
#91476=CARTESIAN_POINT('',(184.1,6.,48.35));
#91477=CARTESIAN_POINT('Origin',(183.9,7.4,48.5));
#91478=CARTESIAN_POINT('',(183.9,7.4,48.5));
#91479=CARTESIAN_POINT('',(91.95,7.4,48.5));
#91480=CARTESIAN_POINT('',(183.9,7.4,48.35));
#91481=CARTESIAN_POINT('',(183.9,7.4,48.5));
#91482=CARTESIAN_POINT('',(184.1,7.4,48.35));
#91483=CARTESIAN_POINT('Origin',(183.9,6.,48.5));
#91484=CARTESIAN_POINT('',(183.9,7.,48.5));
#91485=CARTESIAN_POINT('',(183.9,7.4,48.35));
#91486=CARTESIAN_POINT('Origin',(184.,6.7,48.35));
#91487=CARTESIAN_POINT('Origin',(186.1,6.,48.5));
#91488=CARTESIAN_POINT('',(186.1,6.,48.5));
#91489=CARTESIAN_POINT('',(185.9,6.,48.5));
#91490=CARTESIAN_POINT('',(93.05,6.,48.5));
#91491=CARTESIAN_POINT('',(186.1,6.,48.35));
#91492=CARTESIAN_POINT('',(186.1,6.,48.5));
#91493=CARTESIAN_POINT('',(185.9,6.,48.35));
#91494=CARTESIAN_POINT('',(185.9,6.,48.35));
#91495=CARTESIAN_POINT('',(185.9,6.,48.5));
#91496=CARTESIAN_POINT('Origin',(186.1,7.4,48.5));
#91497=CARTESIAN_POINT('',(186.1,7.4,48.5));
#91498=CARTESIAN_POINT('',(186.1,7.7,48.5));
#91499=CARTESIAN_POINT('',(186.1,7.4,48.35));
#91500=CARTESIAN_POINT('',(186.1,7.4,48.5));
#91501=CARTESIAN_POINT('',(186.1,6.,48.35));
#91502=CARTESIAN_POINT('Origin',(185.9,7.4,48.5));
#91503=CARTESIAN_POINT('',(185.9,7.4,48.5));
#91504=CARTESIAN_POINT('',(92.95,7.4,48.5));
#91505=CARTESIAN_POINT('',(185.9,7.4,48.35));
#91506=CARTESIAN_POINT('',(185.9,7.4,48.5));
#91507=CARTESIAN_POINT('',(186.1,7.4,48.35));
#91508=CARTESIAN_POINT('Origin',(185.9,6.,48.5));
#91509=CARTESIAN_POINT('',(185.9,7.,48.5));
#91510=CARTESIAN_POINT('',(185.9,7.4,48.35));
#91511=CARTESIAN_POINT('Origin',(186.,6.7,48.35));
#91512=CARTESIAN_POINT('Origin',(188.1,6.,48.5));
#91513=CARTESIAN_POINT('',(188.1,6.,48.5));
#91514=CARTESIAN_POINT('',(187.9,6.,48.5));
#91515=CARTESIAN_POINT('',(94.05,6.,48.5));
#91516=CARTESIAN_POINT('',(188.1,6.,48.35));
#91517=CARTESIAN_POINT('',(188.1,6.,48.5));
#91518=CARTESIAN_POINT('',(187.9,6.,48.35));
#91519=CARTESIAN_POINT('',(187.9,6.,48.35));
#91520=CARTESIAN_POINT('',(187.9,6.,48.5));
#91521=CARTESIAN_POINT('Origin',(188.1,7.4,48.5));
#91522=CARTESIAN_POINT('',(188.1,7.4,48.5));
#91523=CARTESIAN_POINT('',(188.1,7.7,48.5));
#91524=CARTESIAN_POINT('',(188.1,7.4,48.35));
#91525=CARTESIAN_POINT('',(188.1,7.4,48.5));
#91526=CARTESIAN_POINT('',(188.1,6.,48.35));
#91527=CARTESIAN_POINT('Origin',(187.9,7.4,48.5));
#91528=CARTESIAN_POINT('',(187.9,7.4,48.5));
#91529=CARTESIAN_POINT('',(93.95,7.4,48.5));
#91530=CARTESIAN_POINT('',(187.9,7.4,48.35));
#91531=CARTESIAN_POINT('',(187.9,7.4,48.5));
#91532=CARTESIAN_POINT('',(188.1,7.4,48.35));
#91533=CARTESIAN_POINT('Origin',(187.9,6.,48.5));
#91534=CARTESIAN_POINT('',(187.9,7.,48.5));
#91535=CARTESIAN_POINT('',(187.9,7.4,48.35));
#91536=CARTESIAN_POINT('Origin',(188.,6.7,48.35));
#91537=CARTESIAN_POINT('Origin',(190.1,4.4,48.5));
#91538=CARTESIAN_POINT('',(190.1,4.4,48.5));
#91539=CARTESIAN_POINT('',(189.9,4.4,48.5));
#91540=CARTESIAN_POINT('',(95.05,4.4,48.5));
#91541=CARTESIAN_POINT('',(190.1,4.4,48.35));
#91542=CARTESIAN_POINT('',(190.1,4.4,48.5));
#91543=CARTESIAN_POINT('',(189.9,4.4,48.35));
#91544=CARTESIAN_POINT('',(189.9,4.4,48.35));
#91545=CARTESIAN_POINT('',(189.9,4.4,48.5));
#91546=CARTESIAN_POINT('Origin',(190.1,7.4,48.5));
#91547=CARTESIAN_POINT('',(190.1,7.4,48.5));
#91548=CARTESIAN_POINT('',(190.1,7.7,48.5));
#91549=CARTESIAN_POINT('',(190.1,7.4,48.35));
#91550=CARTESIAN_POINT('',(190.1,7.4,48.5));
#91551=CARTESIAN_POINT('',(190.1,4.4,48.35));
#91552=CARTESIAN_POINT('Origin',(189.9,7.4,48.5));
#91553=CARTESIAN_POINT('',(189.9,7.4,48.5));
#91554=CARTESIAN_POINT('',(94.95,7.4,48.5));
#91555=CARTESIAN_POINT('',(189.9,7.4,48.35));
#91556=CARTESIAN_POINT('',(189.9,7.4,48.5));
#91557=CARTESIAN_POINT('',(190.1,7.4,48.35));
#91558=CARTESIAN_POINT('Origin',(189.9,4.4,48.5));
#91559=CARTESIAN_POINT('',(189.9,6.2,48.5));
#91560=CARTESIAN_POINT('',(189.9,7.4,48.35));
#91561=CARTESIAN_POINT('Origin',(190.,5.9,48.35));
#91562=CARTESIAN_POINT('Origin',(192.1,6.,48.5));
#91563=CARTESIAN_POINT('',(192.1,6.,48.5));
#91564=CARTESIAN_POINT('',(191.9,6.,48.5));
#91565=CARTESIAN_POINT('',(96.05,6.,48.5));
#91566=CARTESIAN_POINT('',(192.1,6.,48.35));
#91567=CARTESIAN_POINT('',(192.1,6.,48.5));
#91568=CARTESIAN_POINT('',(191.9,6.,48.35));
#91569=CARTESIAN_POINT('',(191.9,6.,48.35));
#91570=CARTESIAN_POINT('',(191.9,6.,48.5));
#91571=CARTESIAN_POINT('Origin',(192.1,7.4,48.5));
#91572=CARTESIAN_POINT('',(192.1,7.4,48.5));
#91573=CARTESIAN_POINT('',(192.1,7.7,48.5));
#91574=CARTESIAN_POINT('',(192.1,7.4,48.35));
#91575=CARTESIAN_POINT('',(192.1,7.4,48.5));
#91576=CARTESIAN_POINT('',(192.1,6.,48.35));
#91577=CARTESIAN_POINT('Origin',(191.9,7.4,48.5));
#91578=CARTESIAN_POINT('',(191.9,7.4,48.5));
#91579=CARTESIAN_POINT('',(95.95,7.4,48.5));
#91580=CARTESIAN_POINT('',(191.9,7.4,48.35));
#91581=CARTESIAN_POINT('',(191.9,7.4,48.5));
#91582=CARTESIAN_POINT('',(192.1,7.4,48.35));
#91583=CARTESIAN_POINT('Origin',(191.9,6.,48.5));
#91584=CARTESIAN_POINT('',(191.9,7.,48.5));
#91585=CARTESIAN_POINT('',(191.9,7.4,48.35));
#91586=CARTESIAN_POINT('Origin',(192.,6.7,48.35));
#91587=CARTESIAN_POINT('Origin',(194.1,6.,48.5));
#91588=CARTESIAN_POINT('',(194.1,6.,48.5));
#91589=CARTESIAN_POINT('',(193.9,6.,48.5));
#91590=CARTESIAN_POINT('',(97.05,6.,48.5));
#91591=CARTESIAN_POINT('',(194.1,6.,48.35));
#91592=CARTESIAN_POINT('',(194.1,6.,48.5));
#91593=CARTESIAN_POINT('',(193.9,6.,48.35));
#91594=CARTESIAN_POINT('',(193.9,6.,48.35));
#91595=CARTESIAN_POINT('',(193.9,6.,48.5));
#91596=CARTESIAN_POINT('Origin',(194.1,7.4,48.5));
#91597=CARTESIAN_POINT('',(194.1,7.4,48.5));
#91598=CARTESIAN_POINT('',(194.1,7.7,48.5));
#91599=CARTESIAN_POINT('',(194.1,7.4,48.35));
#91600=CARTESIAN_POINT('',(194.1,7.4,48.5));
#91601=CARTESIAN_POINT('',(194.1,6.,48.35));
#91602=CARTESIAN_POINT('Origin',(193.9,7.4,48.5));
#91603=CARTESIAN_POINT('',(193.9,7.4,48.5));
#91604=CARTESIAN_POINT('',(96.95,7.4,48.5));
#91605=CARTESIAN_POINT('',(193.9,7.4,48.35));
#91606=CARTESIAN_POINT('',(193.9,7.4,48.5));
#91607=CARTESIAN_POINT('',(194.1,7.4,48.35));
#91608=CARTESIAN_POINT('Origin',(193.9,6.,48.5));
#91609=CARTESIAN_POINT('',(193.9,7.,48.5));
#91610=CARTESIAN_POINT('',(193.9,7.4,48.35));
#91611=CARTESIAN_POINT('Origin',(194.,6.7,48.35));
#91612=CARTESIAN_POINT('Origin',(196.1,6.,48.5));
#91613=CARTESIAN_POINT('',(196.1,6.,48.5));
#91614=CARTESIAN_POINT('',(195.9,6.,48.5));
#91615=CARTESIAN_POINT('',(98.05,6.,48.5));
#91616=CARTESIAN_POINT('',(196.1,6.,48.35));
#91617=CARTESIAN_POINT('',(196.1,6.,48.5));
#91618=CARTESIAN_POINT('',(195.9,6.,48.35));
#91619=CARTESIAN_POINT('',(195.9,6.,48.35));
#91620=CARTESIAN_POINT('',(195.9,6.,48.5));
#91621=CARTESIAN_POINT('Origin',(196.1,7.4,48.5));
#91622=CARTESIAN_POINT('',(196.1,7.4,48.5));
#91623=CARTESIAN_POINT('',(196.1,7.7,48.5));
#91624=CARTESIAN_POINT('',(196.1,7.4,48.35));
#91625=CARTESIAN_POINT('',(196.1,7.4,48.5));
#91626=CARTESIAN_POINT('',(196.1,6.,48.35));
#91627=CARTESIAN_POINT('Origin',(195.9,7.4,48.5));
#91628=CARTESIAN_POINT('',(195.9,7.4,48.5));
#91629=CARTESIAN_POINT('',(97.95,7.4,48.5));
#91630=CARTESIAN_POINT('',(195.9,7.4,48.35));
#91631=CARTESIAN_POINT('',(195.9,7.4,48.5));
#91632=CARTESIAN_POINT('',(196.1,7.4,48.35));
#91633=CARTESIAN_POINT('Origin',(195.9,6.,48.5));
#91634=CARTESIAN_POINT('',(195.9,7.,48.5));
#91635=CARTESIAN_POINT('',(195.9,7.4,48.35));
#91636=CARTESIAN_POINT('Origin',(196.,6.7,48.35));
#91637=CARTESIAN_POINT('Origin',(198.1,6.,48.5));
#91638=CARTESIAN_POINT('',(198.1,6.,48.5));
#91639=CARTESIAN_POINT('',(197.9,6.,48.5));
#91640=CARTESIAN_POINT('',(99.05,6.,48.5));
#91641=CARTESIAN_POINT('',(198.1,6.,48.35));
#91642=CARTESIAN_POINT('',(198.1,6.,48.5));
#91643=CARTESIAN_POINT('',(197.9,6.,48.35));
#91644=CARTESIAN_POINT('',(197.9,6.,48.35));
#91645=CARTESIAN_POINT('',(197.9,6.,48.5));
#91646=CARTESIAN_POINT('Origin',(198.1,7.4,48.5));
#91647=CARTESIAN_POINT('',(198.1,7.4,48.5));
#91648=CARTESIAN_POINT('',(198.1,7.7,48.5));
#91649=CARTESIAN_POINT('',(198.1,7.4,48.35));
#91650=CARTESIAN_POINT('',(198.1,7.4,48.5));
#91651=CARTESIAN_POINT('',(198.1,6.,48.35));
#91652=CARTESIAN_POINT('Origin',(197.9,7.4,48.5));
#91653=CARTESIAN_POINT('',(197.9,7.4,48.5));
#91654=CARTESIAN_POINT('',(98.95,7.4,48.5));
#91655=CARTESIAN_POINT('',(197.9,7.4,48.35));
#91656=CARTESIAN_POINT('',(197.9,7.4,48.5));
#91657=CARTESIAN_POINT('',(198.1,7.4,48.35));
#91658=CARTESIAN_POINT('Origin',(197.9,6.,48.5));
#91659=CARTESIAN_POINT('',(197.9,7.,48.5));
#91660=CARTESIAN_POINT('',(197.9,7.4,48.35));
#91661=CARTESIAN_POINT('Origin',(198.,6.7,48.35));
#91662=CARTESIAN_POINT('Origin',(200.1,4.4,48.5));
#91663=CARTESIAN_POINT('',(200.1,4.4,48.5));
#91664=CARTESIAN_POINT('',(199.9,4.4,48.5));
#91665=CARTESIAN_POINT('',(100.05,4.4,48.5));
#91666=CARTESIAN_POINT('',(200.1,4.4,48.35));
#91667=CARTESIAN_POINT('',(200.1,4.4,48.5));
#91668=CARTESIAN_POINT('',(199.9,4.4,48.35));
#91669=CARTESIAN_POINT('',(199.9,4.4,48.35));
#91670=CARTESIAN_POINT('',(199.9,4.4,48.5));
#91671=CARTESIAN_POINT('Origin',(200.1,7.4,48.5));
#91672=CARTESIAN_POINT('',(200.1,7.4,48.5));
#91673=CARTESIAN_POINT('',(200.1,7.7,48.5));
#91674=CARTESIAN_POINT('',(200.1,7.4,48.35));
#91675=CARTESIAN_POINT('',(200.1,7.4,48.5));
#91676=CARTESIAN_POINT('',(200.1,4.4,48.35));
#91677=CARTESIAN_POINT('Origin',(199.9,7.4,48.5));
#91678=CARTESIAN_POINT('',(199.9,7.4,48.5));
#91679=CARTESIAN_POINT('',(99.95,7.4,48.5));
#91680=CARTESIAN_POINT('',(199.9,7.4,48.35));
#91681=CARTESIAN_POINT('',(199.9,7.4,48.5));
#91682=CARTESIAN_POINT('',(200.1,7.4,48.35));
#91683=CARTESIAN_POINT('Origin',(199.9,4.4,48.5));
#91684=CARTESIAN_POINT('',(199.9,6.2,48.5));
#91685=CARTESIAN_POINT('',(199.9,7.4,48.35));
#91686=CARTESIAN_POINT('Origin',(200.,5.9,48.35));
#91687=CARTESIAN_POINT('Origin',(220.,0.,20.5));
#91688=CARTESIAN_POINT('',(220.,0.3,20.5));
#91689=CARTESIAN_POINT('',(219.7,0.,20.5));
#91690=CARTESIAN_POINT('',(219.85,0.150000000000003,20.5));
#91691=CARTESIAN_POINT('',(220.,0.5,20.5));
#91692=CARTESIAN_POINT('',(220.,2.,20.5));
#91693=CARTESIAN_POINT('',(0.,0.5,20.5));
#91694=CARTESIAN_POINT('',(0.,0.5,20.5));
#91695=CARTESIAN_POINT('',(0.,0.3,20.5));
#91696=CARTESIAN_POINT('',(0.,2.,20.5));
#91697=CARTESIAN_POINT('',(0.3,0.,20.5));
#91698=CARTESIAN_POINT('',(55.15,-54.85,20.5));
#91699=CARTESIAN_POINT('',(110.,0.,20.5));
#91700=CARTESIAN_POINT('Origin',(0.,0.,36.5));
#91701=CARTESIAN_POINT('',(219.7,0.,36.5));
#91702=CARTESIAN_POINT('',(220.,0.3,36.5));
#91703=CARTESIAN_POINT('',(164.849999999998,-54.85,36.5));
#91704=CARTESIAN_POINT('',(0.3,0.,36.5));
#91705=CARTESIAN_POINT('',(0.,0.,36.5));
#91706=CARTESIAN_POINT('',(0.,0.3,36.5));
#91707=CARTESIAN_POINT('',(0.15,0.15,36.5));
#91708=CARTESIAN_POINT('',(0.,0.5,36.5));
#91709=CARTESIAN_POINT('',(0.,2.,36.5));
#91710=CARTESIAN_POINT('',(220.,0.5,36.5));
#91711=CARTESIAN_POINT('',(220.,0.5,36.5));
#91712=CARTESIAN_POINT('',(220.,2.,36.5));
#91713=CARTESIAN_POINT('Origin',(110.,0.5,28.5));
#91714=CARTESIAN_POINT('',(0.,0.5,28.5));
#91715=CARTESIAN_POINT('',(220.,0.5,28.5));
#91716=CARTESIAN_POINT('Origin',(0.,4.,28.5));
#91717=CARTESIAN_POINT('',(0.,0.3,47.8757359312881));
#91718=CARTESIAN_POINT('',(0.,0.3,38.5));
#91719=CARTESIAN_POINT('',(0.,0.624264068711927,48.2));
#91720=CARTESIAN_POINT('',(0.,-3.53786796564405,44.037867965644));
#91721=CARTESIAN_POINT('',(0.,7.37573593128807,48.2));
#91722=CARTESIAN_POINT('',(0.,6.,48.2));
#91723=CARTESIAN_POINT('',(0.,7.7,47.8757359312881));
#91724=CARTESIAN_POINT('',(0.,11.537867965644,44.037867965644));
#91725=CARTESIAN_POINT('',(0.,7.7,38.5132486540519));
#91726=CARTESIAN_POINT('',(0.,7.7,18.5));
#91727=CARTESIAN_POINT('',(0.,8.49641016151377,38.0534410329165));
#91728=CARTESIAN_POINT('Origin',(0.,8.,38.1132486540519));
#91729=CARTESIAN_POINT('',(0.,12.6535898384862,40.4535898384862));
#91730=CARTESIAN_POINT('',(0.,7.06867061317363,37.2291352203497));
#91731=CARTESIAN_POINT('',(0.,12.7,40.4267949192431));
#91732=CARTESIAN_POINT('',(0.,12.0081243060696,40.8262495373796));
#91733=CARTESIAN_POINT('',(0.,12.7,31.83));
#91734=CARTESIAN_POINT('',(0.,12.7,22.25));
#91735=CARTESIAN_POINT('',(0.,9.2,31.83));
#91736=CARTESIAN_POINT('',(0.,9.,31.83));
#91737=CARTESIAN_POINT('',(0.,9.2,25.17));
#91738=CARTESIAN_POINT('',(0.,9.2,30.015));
#91739=CARTESIAN_POINT('',(0.,12.7,25.17));
#91740=CARTESIAN_POINT('',(0.,6.75,25.17));
#91741=CARTESIAN_POINT('',(0.,12.7,16.5732050807569));
#91742=CARTESIAN_POINT('',(0.,12.7,22.25));
#91743=CARTESIAN_POINT('',(0.,12.6535898384862,16.5464101615138));
#91744=CARTESIAN_POINT('',(0.,12.0081243060695,16.1737504626203));
#91745=CARTESIAN_POINT('',(0.,8.49641016151378,18.9465589670835));
#91746=CARTESIAN_POINT('',(0.,4.56867061317363,21.2142404526244));
#91747=CARTESIAN_POINT('',(0.,7.7,18.4867513459481));
#91748=CARTESIAN_POINT('Origin',(0.,8.,18.8867513459481));
#91749=CARTESIAN_POINT('',(0.,7.7,9.12426406871192));
#91750=CARTESIAN_POINT('',(0.,7.7,18.5));
#91751=CARTESIAN_POINT('',(0.,7.37573593128808,8.8));
#91752=CARTESIAN_POINT('',(0.,11.537867965644,12.9621320343559));
#91753=CARTESIAN_POINT('',(0.,0.624264068711924,8.8));
#91754=CARTESIAN_POINT('',(0.,2.,8.8));
#91755=CARTESIAN_POINT('',(0.,0.300000000000004,9.12426406871192));
#91756=CARTESIAN_POINT('',(0.,-3.53786796564403,12.962132034356));
#91757=CARTESIAN_POINT('',(0.,0.3,38.5));
#91758=CARTESIAN_POINT('Origin',(219.85,0.15,38.5));
#91759=CARTESIAN_POINT('',(220.,0.300000000000002,47.8757359312881));
#91760=CARTESIAN_POINT('',(220.,0.3,38.5));
#91761=CARTESIAN_POINT('',(219.7,0.,48.));
#91762=CARTESIAN_POINT('',(220.,0.300000000000001,47.8757359312881));
#91763=CARTESIAN_POINT('',(219.7,0.,38.5));
#91764=CARTESIAN_POINT('Origin',(219.85,0.15,38.5));
#91765=CARTESIAN_POINT('',(219.7,0.,9.));
#91766=CARTESIAN_POINT('',(219.7,0.,38.5));
#91767=CARTESIAN_POINT('',(220.,0.3,9.12426406871192));
#91768=CARTESIAN_POINT('',(220.,0.3,9.12426406871192));
#91769=CARTESIAN_POINT('',(220.,0.3,38.5));
#91770=CARTESIAN_POINT('Origin',(0.15,0.15,38.5));
#91771=CARTESIAN_POINT('',(0.3,0.,48.));
#91772=CARTESIAN_POINT('',(0.3,0.,38.5));
#91773=CARTESIAN_POINT('',(0.,0.3,47.8757359312881));
#91774=CARTESIAN_POINT('Origin',(0.,0.,48.5));
#91775=CARTESIAN_POINT('',(0.,0.,48.));
#91776=CARTESIAN_POINT('',(107.65,0.,44.5));
#91777=CARTESIAN_POINT('Origin',(110.,0.,44.5));
#91778=CARTESIAN_POINT('',(32.65,0.,44.5));
#91779=CARTESIAN_POINT('Origin',(35.,0.,44.5));
#91780=CARTESIAN_POINT('',(182.65,0.,44.5));
#91781=CARTESIAN_POINT('Origin',(185.,0.,44.5));
#91782=CARTESIAN_POINT('Origin',(216.,4.5,46.));
#91783=CARTESIAN_POINT('',(215.,4.50000000000002,46.));
#91784=CARTESIAN_POINT('Origin',(216.,4.5,46.));
#91785=CARTESIAN_POINT('',(216.,3.89913938097244,46.));
#91786=CARTESIAN_POINT('',(215.,4.5,46.));
#91787=CARTESIAN_POINT('Origin',(4.,4.5,11.));
#91788=CARTESIAN_POINT('',(3.,4.5,11.));
#91789=CARTESIAN_POINT('Origin',(4.,4.5,11.));
#91790=CARTESIAN_POINT('',(4.,3.89913938097244,11.));
#91791=CARTESIAN_POINT('',(3.,4.5,11.));
#91792=CARTESIAN_POINT('Origin',(4.,8.,11.));
#91793=CARTESIAN_POINT('',(3.,8.,11.));
#91794=CARTESIAN_POINT('Origin',(4.,8.,11.));
#91795=CARTESIAN_POINT('',(3.,8.,11.));
#91796=CARTESIAN_POINT('Origin',(216.,8.,46.));
#91797=CARTESIAN_POINT('',(215.,8.,46.));
#91798=CARTESIAN_POINT('Origin',(216.,8.,46.));
#91799=CARTESIAN_POINT('',(215.,8.,46.));
#91800=CARTESIAN_POINT('Origin',(214.,9.4,28.5));
#91801=CARTESIAN_POINT('',(212.5,9.5,28.5));
#91802=CARTESIAN_POINT('Origin',(214.,9.5,28.5));
#91803=CARTESIAN_POINT('',(212.7,9.3,28.5));
#91804=CARTESIAN_POINT('',(212.6,9.4,28.5));
#91805=CARTESIAN_POINT('Origin',(214.,9.3,28.5));
#91806=CARTESIAN_POINT('Origin',(214.,9.5,28.5));
#91807=CARTESIAN_POINT('',(212.7,4.5,28.5));
#91808=CARTESIAN_POINT('',(212.7,9.5,28.5));
#91809=CARTESIAN_POINT('Origin',(214.,4.5,28.5));
#91810=CARTESIAN_POINT('Origin',(0.,9.5,31.53));
#91811=CARTESIAN_POINT('',(219.7,9.5,25.47));
#91812=CARTESIAN_POINT('',(219.7,9.5,31.53));
#91813=CARTESIAN_POINT('',(219.7,9.5,30.015));
#91814=CARTESIAN_POINT('',(0.3,9.5,25.47));
#91815=CARTESIAN_POINT('',(0.,9.5,25.47));
#91816=CARTESIAN_POINT('',(0.3,9.5,31.53));
#91817=CARTESIAN_POINT('',(0.3,9.5,30.015));
#91818=CARTESIAN_POINT('',(0.,9.5,31.53));
#91819=CARTESIAN_POINT('',(4.5,9.5,28.5));
#91820=CARTESIAN_POINT('Origin',(6.,9.5,28.5));
#91821=CARTESIAN_POINT('Origin',(214.,4.5,28.5));
#91822=CARTESIAN_POINT('',(214.,3.71888119526417,28.5));
#91823=CARTESIAN_POINT('',(212.7,4.5,28.5));
#91824=CARTESIAN_POINT('Origin',(6.,9.4,28.5));
#91825=CARTESIAN_POINT('',(4.7,9.3,28.5));
#91826=CARTESIAN_POINT('',(4.6,9.4,28.5));
#91827=CARTESIAN_POINT('Origin',(6.,9.3,28.5));
#91828=CARTESIAN_POINT('Origin',(6.,9.5,28.5));
#91829=CARTESIAN_POINT('',(4.7,4.5,28.5));
#91830=CARTESIAN_POINT('',(4.7,9.5,28.5));
#91831=CARTESIAN_POINT('Origin',(6.,4.5,28.5));
#91832=CARTESIAN_POINT('Origin',(6.,4.5,28.5));
#91833=CARTESIAN_POINT('',(6.,3.71888119526417,28.5));
#91834=CARTESIAN_POINT('',(4.7,4.5,28.5));
#91835=CARTESIAN_POINT('Origin',(185.,8.,12.5));
#91836=CARTESIAN_POINT('',(182.,8.,12.5));
#91837=CARTESIAN_POINT('Origin',(185.,8.,12.5));
#91838=CARTESIAN_POINT('',(182.,4.8,12.5));
#91839=CARTESIAN_POINT('',(182.,8.,12.5));
#91840=CARTESIAN_POINT('Origin',(185.,4.8,12.5));
#91841=CARTESIAN_POINT('Origin',(185.,4.8,12.5));
#91842=CARTESIAN_POINT('',(182.95,4.8,12.5));
#91843=CARTESIAN_POINT('Origin',(185.,4.8,12.5));
#91844=CARTESIAN_POINT('Origin',(35.,8.,12.5));
#91845=CARTESIAN_POINT('',(32.,8.,12.5));
#91846=CARTESIAN_POINT('Origin',(35.,8.,12.5));
#91847=CARTESIAN_POINT('',(32.,4.8,12.5));
#91848=CARTESIAN_POINT('',(32.,8.,12.5));
#91849=CARTESIAN_POINT('Origin',(35.,4.8,12.5));
#91850=CARTESIAN_POINT('Origin',(35.,4.8,12.5));
#91851=CARTESIAN_POINT('',(32.95,4.8,12.5));
#91852=CARTESIAN_POINT('Origin',(35.,4.8,12.5));
#91853=CARTESIAN_POINT('Origin',(35.,8.,44.5));
#91854=CARTESIAN_POINT('',(32.,8.,44.5));
#91855=CARTESIAN_POINT('Origin',(35.,8.,44.5));
#91856=CARTESIAN_POINT('',(32.,4.8,44.5));
#91857=CARTESIAN_POINT('',(32.,8.,44.5));
#91858=CARTESIAN_POINT('Origin',(35.,4.8,44.5));
#91859=CARTESIAN_POINT('Origin',(35.,4.8,44.5));
#91860=CARTESIAN_POINT('',(32.95,4.8,44.5));
#91861=CARTESIAN_POINT('Origin',(35.,4.8,44.5));
#91862=CARTESIAN_POINT('Origin',(110.,8.,12.5));
#91863=CARTESIAN_POINT('',(107.,8.,12.5));
#91864=CARTESIAN_POINT('Origin',(110.,8.,12.5));
#91865=CARTESIAN_POINT('',(107.,4.8,12.5));
#91866=CARTESIAN_POINT('',(107.,8.,12.5));
#91867=CARTESIAN_POINT('Origin',(110.,4.8,12.5));
#91868=CARTESIAN_POINT('Origin',(110.,4.8,12.5));
#91869=CARTESIAN_POINT('',(107.95,4.8,12.5));
#91870=CARTESIAN_POINT('Origin',(110.,4.8,12.5));
#91871=CARTESIAN_POINT('Origin',(110.,8.,44.5));
#91872=CARTESIAN_POINT('',(107.,8.,44.5));
#91873=CARTESIAN_POINT('Origin',(110.,8.,44.5));
#91874=CARTESIAN_POINT('',(107.,4.8,44.5));
#91875=CARTESIAN_POINT('',(107.,8.,44.5));
#91876=CARTESIAN_POINT('Origin',(110.,4.8,44.5));
#91877=CARTESIAN_POINT('Origin',(110.,4.8,44.5));
#91878=CARTESIAN_POINT('',(107.95,4.8,44.5));
#91879=CARTESIAN_POINT('Origin',(110.,4.8,44.5));
#91880=CARTESIAN_POINT('Origin',(185.,8.,44.5));
#91881=CARTESIAN_POINT('',(182.,8.,44.5));
#91882=CARTESIAN_POINT('Origin',(185.,8.,44.5));
#91883=CARTESIAN_POINT('',(182.,4.8,44.5));
#91884=CARTESIAN_POINT('',(182.,8.,44.5));
#91885=CARTESIAN_POINT('Origin',(185.,4.8,44.5));
#91886=CARTESIAN_POINT('Origin',(185.,4.8,44.5));
#91887=CARTESIAN_POINT('',(182.95,4.8,44.5));
#91888=CARTESIAN_POINT('Origin',(185.,4.8,44.5));
#91889=CARTESIAN_POINT('Origin',(185.,0.15,44.5));
#91890=CARTESIAN_POINT('',(182.95,0.3,44.5));
#91891=CARTESIAN_POINT('',(182.8,0.15,44.5));
#91892=CARTESIAN_POINT('Origin',(185.,0.3,44.5));
#91893=CARTESIAN_POINT('Origin',(0.,0.,48.5));
#91894=CARTESIAN_POINT('',(0.3,0.,9.));
#91895=CARTESIAN_POINT('',(0.3,0.,38.5));
#91896=CARTESIAN_POINT('',(0.,0.,9.));
#91897=CARTESIAN_POINT('',(182.65,0.,12.5));
#91898=CARTESIAN_POINT('Origin',(185.,0.,12.5));
#91899=CARTESIAN_POINT('',(32.65,0.,12.5));
#91900=CARTESIAN_POINT('Origin',(35.,0.,12.5));
#91901=CARTESIAN_POINT('',(107.65,0.,12.5));
#91902=CARTESIAN_POINT('Origin',(110.,0.,12.5));
#91903=CARTESIAN_POINT('Origin',(185.,0.,44.5));
#91904=CARTESIAN_POINT('',(182.95,0.,44.5));
#91905=CARTESIAN_POINT('Origin',(110.,0.15,44.5));
#91906=CARTESIAN_POINT('',(107.95,0.3,44.5));
#91907=CARTESIAN_POINT('',(107.8,0.15,44.5));
#91908=CARTESIAN_POINT('Origin',(110.,0.3,44.5));
#91909=CARTESIAN_POINT('Origin',(110.,0.,44.5));
#91910=CARTESIAN_POINT('',(107.95,0.,44.5));
#91911=CARTESIAN_POINT('Origin',(110.,0.15,12.5));
#91912=CARTESIAN_POINT('',(107.95,0.3,12.5));
#91913=CARTESIAN_POINT('',(107.8,0.15,12.5));
#91914=CARTESIAN_POINT('Origin',(110.,0.3,12.5));
#91915=CARTESIAN_POINT('Origin',(110.,0.,12.5));
#91916=CARTESIAN_POINT('',(107.95,0.,12.5));
#91917=CARTESIAN_POINT('Origin',(35.,0.15,44.5));
#91918=CARTESIAN_POINT('',(32.95,0.3,44.5));
#91919=CARTESIAN_POINT('',(32.8,0.15,44.5));
#91920=CARTESIAN_POINT('Origin',(35.,0.3,44.5));
#91921=CARTESIAN_POINT('Origin',(35.,0.,44.5));
#91922=CARTESIAN_POINT('',(32.95,0.,44.5));
#91923=CARTESIAN_POINT('Origin',(35.,0.15,12.5));
#91924=CARTESIAN_POINT('',(32.95,0.3,12.5));
#91925=CARTESIAN_POINT('',(32.8,0.15,12.5));
#91926=CARTESIAN_POINT('Origin',(35.,0.3,12.5));
#91927=CARTESIAN_POINT('Origin',(35.,0.,12.5));
#91928=CARTESIAN_POINT('',(32.95,0.,12.5));
#91929=CARTESIAN_POINT('Origin',(185.,0.15,12.5));
#91930=CARTESIAN_POINT('',(182.95,0.3,12.5));
#91931=CARTESIAN_POINT('',(182.8,0.15,12.5));
#91932=CARTESIAN_POINT('Origin',(185.,0.3,12.5));
#91933=CARTESIAN_POINT('Origin',(185.,0.,12.5));
#91934=CARTESIAN_POINT('',(182.95,0.,12.5));
#91935=CARTESIAN_POINT('Origin',(219.85,6.99367061317363,37.3590390309174));
#91936=CARTESIAN_POINT('',(219.7,12.6535898384862,40.8));
#91937=CARTESIAN_POINT('',(219.7,8.43301270189222,38.3632486540519));
#91938=CARTESIAN_POINT('',(219.7,6.91867061317363,37.488942841485));
#91939=CARTESIAN_POINT('',(220.,8.49641016151377,38.0534410329165));
#91940=CARTESIAN_POINT('Origin',(219.7,8.,38.1132486540519));
#91941=CARTESIAN_POINT('',(220.,12.6535898384862,40.4535898384862));
#91942=CARTESIAN_POINT('',(220.,7.06867061317363,37.2291352203497));
#91943=CARTESIAN_POINT('',(220.,12.6535898384862,40.4535898384862));
#91944=CARTESIAN_POINT('Origin',(219.85,12.0831243060696,40.9561533479473));
#91945=CARTESIAN_POINT('',(220.,12.7,40.4267949192431));
#91946=CARTESIAN_POINT('',(220.,12.0081243060696,40.8262495373796));
#91947=CARTESIAN_POINT('',(219.7,13.,40.6));
#91948=CARTESIAN_POINT('',(220.,12.7,40.4267949192431));
#91949=CARTESIAN_POINT('',(219.7,12.1581243060696,41.086057158515));
#91950=CARTESIAN_POINT('Origin',(219.85,12.85,22.25));
#91951=CARTESIAN_POINT('',(220.,12.7,31.83));
#91952=CARTESIAN_POINT('',(220.,12.7,22.25));
#91953=CARTESIAN_POINT('',(219.7,13.,31.53));
#91954=CARTESIAN_POINT('',(220.,12.7,31.83));
#91955=CARTESIAN_POINT('',(219.7,13.,22.25));
#91956=CARTESIAN_POINT('Origin',(219.85,6.75,25.32));
#91957=CARTESIAN_POINT('',(220.,9.2,25.17));
#91958=CARTESIAN_POINT('',(220.,12.7,25.17));
#91959=CARTESIAN_POINT('',(220.,6.75,25.17));
#91960=CARTESIAN_POINT('',(219.7,13.,25.47));
#91961=CARTESIAN_POINT('',(220.,12.7,25.17));
#91962=CARTESIAN_POINT('',(219.7,6.75,25.47));
#91963=CARTESIAN_POINT('',(219.7,9.5,25.47));
#91964=CARTESIAN_POINT('Origin',(219.85,12.85,22.25));
#91965=CARTESIAN_POINT('',(220.,12.7,16.5732050807569));
#91966=CARTESIAN_POINT('',(220.,12.7,22.25));
#91967=CARTESIAN_POINT('',(219.7,13.,16.4));
#91968=CARTESIAN_POINT('',(220.,12.7,16.5732050807569));
#91969=CARTESIAN_POINT('',(219.7,13.,22.25));
#91970=CARTESIAN_POINT('Origin',(219.85,12.0831243060695,16.0438466520527));
#91971=CARTESIAN_POINT('',(220.,12.6535898384862,16.5464101615138));
#91972=CARTESIAN_POINT('',(220.,12.0081243060695,16.1737504626203));
#91973=CARTESIAN_POINT('',(219.7,12.6535898384862,16.2));
#91974=CARTESIAN_POINT('',(220.,12.6535898384862,16.5464101615138));
#91975=CARTESIAN_POINT('',(219.7,12.1581243060695,15.913942841485));
#91976=CARTESIAN_POINT('Origin',(219.85,4.49367061317363,21.0843366420567));
#91977=CARTESIAN_POINT('',(220.,8.49641016151378,18.9465589670835));
#91978=CARTESIAN_POINT('',(220.,4.56867061317363,21.2142404526244));
#91979=CARTESIAN_POINT('',(219.7,8.43301270189222,18.6367513459481));
#91980=CARTESIAN_POINT('Origin',(219.7,8.,18.8867513459481));
#91981=CARTESIAN_POINT('',(219.7,4.41867061317363,20.954432831489));
#91982=CARTESIAN_POINT('Origin',(219.85,9.35,30.015));
#91983=CARTESIAN_POINT('',(220.,9.2,31.83));
#91984=CARTESIAN_POINT('',(220.,9.2,30.015));
#91985=CARTESIAN_POINT('',(219.7,9.5,31.53));
#91986=CARTESIAN_POINT('Origin',(219.85,9.,31.68));
#91987=CARTESIAN_POINT('',(220.,9.,31.83));
#91988=CARTESIAN_POINT('',(219.7,9.,31.53));
#91989=CARTESIAN_POINT('Origin',(0.,8.,38.1132486540519));
#91990=CARTESIAN_POINT('',(0.3,8.43301270189222,38.3632486540519));
#91991=CARTESIAN_POINT('',(0.,8.43301270189222,38.3632486540519));
#91992=CARTESIAN_POINT('Origin',(0.300000000000001,8.,38.1132486540519));
#91993=CARTESIAN_POINT('',(0.3,8.,38.6132486540519));
#91994=CARTESIAN_POINT('Origin',(0.3,8.,38.1132486540519));
#91995=CARTESIAN_POINT('',(219.7,8.,38.6132486540519));
#91996=CARTESIAN_POINT('',(0.,8.,38.6132486540519));
#91997=CARTESIAN_POINT('',(220.,7.7,38.5132486540519));
#91998=CARTESIAN_POINT('Origin',(219.7,8.,38.1132486540519));
#91999=CARTESIAN_POINT('Origin',(220.,8.,38.1132486540519));
#92000=CARTESIAN_POINT('Origin',(0.,13.,41.));
#92001=CARTESIAN_POINT('',(0.3,12.6535898384862,40.8));
#92002=CARTESIAN_POINT('',(0.,12.6535898384862,40.8));
#92003=CARTESIAN_POINT('',(0.3,6.91867061317363,37.488942841485));
#92004=CARTESIAN_POINT('Origin',(0.,12.8267949192431,40.7));
#92005=CARTESIAN_POINT('',(0.3,13.,40.6));
#92006=CARTESIAN_POINT('',(0.,13.,40.6));
#92007=CARTESIAN_POINT('',(0.3,12.1581243060696,41.086057158515));
#92008=CARTESIAN_POINT('Origin',(0.,13.,16.));
#92009=CARTESIAN_POINT('',(0.3,13.,31.53));
#92010=CARTESIAN_POINT('',(0.,13.,31.53));
#92011=CARTESIAN_POINT('',(0.3,13.,22.25));
#92012=CARTESIAN_POINT('Origin',(0.,14.,31.53));
#92013=CARTESIAN_POINT('',(0.3,9.,31.53));
#92014=CARTESIAN_POINT('Origin',(0.,9.5,25.47));
#92015=CARTESIAN_POINT('',(0.3,13.,25.47));
#92016=CARTESIAN_POINT('',(0.,13.,25.47));
#92017=CARTESIAN_POINT('',(0.3,6.75,25.47));
#92018=CARTESIAN_POINT('Origin',(219.85,7.85,18.5));
#92019=CARTESIAN_POINT('',(219.7,8.,9.));
#92020=CARTESIAN_POINT('',(219.7,8.,18.3867513459481));
#92021=CARTESIAN_POINT('',(219.7,8.,18.5));
#92022=CARTESIAN_POINT('',(220.,7.7,18.4867513459481));
#92023=CARTESIAN_POINT('Origin',(219.7,8.,18.8867513459481));
#92024=CARTESIAN_POINT('',(220.,7.7,9.12426406871192));
#92025=CARTESIAN_POINT('',(220.,7.7,18.5));
#92026=CARTESIAN_POINT('',(220.,7.7,9.12426406871192));
#92027=CARTESIAN_POINT('Origin',(219.85,11.643933982822,12.856066017178));
#92028=CARTESIAN_POINT('',(220.,7.37573593128808,8.8));
#92029=CARTESIAN_POINT('',(220.,11.537867965644,12.9621320343559));
#92030=CARTESIAN_POINT('',(219.7,7.5,8.5));
#92031=CARTESIAN_POINT('',(220.,7.37573593128808,8.8));
#92032=CARTESIAN_POINT('',(219.7,11.75,12.75));
#92033=CARTESIAN_POINT('Origin',(219.85,2.,8.65));
#92034=CARTESIAN_POINT('',(220.,0.624264068711924,8.8));
#92035=CARTESIAN_POINT('',(220.,2.,8.8));
#92036=CARTESIAN_POINT('',(219.7,0.5,8.5));
#92037=CARTESIAN_POINT('',(220.,0.624264068711924,8.8));
#92038=CARTESIAN_POINT('',(219.7,2.,8.5));
#92039=CARTESIAN_POINT('Origin',(219.85,-3.64393398282202,12.856066017178));
#92040=CARTESIAN_POINT('',(220.,-3.53786796564403,12.962132034356));
#92041=CARTESIAN_POINT('',(219.7,-3.75,12.75));
#92042=CARTESIAN_POINT('Origin',(219.85,-3.64393398282203,44.1439339828219));
#92043=CARTESIAN_POINT('',(220.,0.624264068711926,48.2));
#92044=CARTESIAN_POINT('',(220.,-3.53786796564405,44.037867965644));
#92045=CARTESIAN_POINT('',(219.7,0.5,48.5));
#92046=CARTESIAN_POINT('',(220.,0.624264068711926,48.2));
#92047=CARTESIAN_POINT('',(219.7,-3.75000000000001,44.2499999999999));
#92048=CARTESIAN_POINT('Origin',(219.85,6.,48.35));
#92049=CARTESIAN_POINT('',(220.,7.37573593128807,48.2));
#92050=CARTESIAN_POINT('',(220.,6.,48.2));
#92051=CARTESIAN_POINT('',(219.7,7.5,48.5));
#92052=CARTESIAN_POINT('',(220.,7.37573593128807,48.2));
#92053=CARTESIAN_POINT('',(219.7,6.,48.5));
#92054=CARTESIAN_POINT('Origin',(219.85,11.643933982822,44.143933982822));
#92055=CARTESIAN_POINT('',(220.,7.7,47.8757359312881));
#92056=CARTESIAN_POINT('',(220.,11.537867965644,44.037867965644));
#92057=CARTESIAN_POINT('',(219.7,8.,48.));
#92058=CARTESIAN_POINT('',(220.,7.7,47.8757359312881));
#92059=CARTESIAN_POINT('',(219.7,11.75,44.25));
#92060=CARTESIAN_POINT('Origin',(219.85,7.85,18.5));
#92061=CARTESIAN_POINT('',(220.,7.7,18.5));
#92062=CARTESIAN_POINT('',(219.7,8.,18.5));
#92063=CARTESIAN_POINT('Origin',(0.,8.,8.5));
#92064=CARTESIAN_POINT('',(0.3,8.,9.));
#92065=CARTESIAN_POINT('',(0.,8.,9.));
#92066=CARTESIAN_POINT('',(0.3,8.,18.3867513459481));
#92067=CARTESIAN_POINT('',(0.3,8.,18.5));
#92068=CARTESIAN_POINT('',(0.,8.,18.3867513459481));
#92069=CARTESIAN_POINT('Origin',(0.,7.75,8.75));
#92070=CARTESIAN_POINT('',(0.3,7.5,8.5));
#92071=CARTESIAN_POINT('',(0.,7.5,8.5));
#92072=CARTESIAN_POINT('',(0.3,11.75,12.75));
#92073=CARTESIAN_POINT('Origin',(0.,0.,8.5));
#92074=CARTESIAN_POINT('',(0.3,0.5,8.5));
#92075=CARTESIAN_POINT('',(0.,0.5,8.5));
#92076=CARTESIAN_POINT('',(0.3,2.,8.5));
#92077=CARTESIAN_POINT('Origin',(0.,0.25,8.75));
#92078=CARTESIAN_POINT('',(0.3,-3.75,12.75));
#92079=CARTESIAN_POINT('Origin',(0.,0.25,48.25));
#92080=CARTESIAN_POINT('',(0.3,0.5,48.5));
#92081=CARTESIAN_POINT('',(0.,0.5,48.5));
#92082=CARTESIAN_POINT('',(0.3,-3.75000000000001,44.2499999999999));
#92083=CARTESIAN_POINT('Origin',(0.,8.,48.5));
#92084=CARTESIAN_POINT('',(0.3,7.5,48.5));
#92085=CARTESIAN_POINT('',(0.,7.5,48.5));
#92086=CARTESIAN_POINT('',(0.3,6.,48.5));
#92087=CARTESIAN_POINT('Origin',(0.,7.75,48.25));
#92088=CARTESIAN_POINT('',(0.3,8.,48.));
#92089=CARTESIAN_POINT('',(0.,8.,48.));
#92090=CARTESIAN_POINT('',(0.3,11.75,44.25));
#92091=CARTESIAN_POINT('Origin',(0.,8.,8.5));
#92092=CARTESIAN_POINT('',(0.3,8.,18.5));
#92093=CARTESIAN_POINT('Origin',(0.15,4.49367061317363,21.0843366420567));
#92094=CARTESIAN_POINT('',(0.3,12.6535898384862,16.2));
#92095=CARTESIAN_POINT('',(0.3,8.43301270189222,18.6367513459481));
#92096=CARTESIAN_POINT('',(0.3,4.41867061317363,20.954432831489));
#92097=CARTESIAN_POINT('Origin',(0.300000000000001,8.,18.8867513459481));
#92098=CARTESIAN_POINT('',(0.,12.6535898384862,16.5464101615138));
#92099=CARTESIAN_POINT('Origin',(0.15,12.0831243060695,16.0438466520527));
#92100=CARTESIAN_POINT('',(0.3,13.,16.4));
#92101=CARTESIAN_POINT('',(0.,12.7,16.5732050807569));
#92102=CARTESIAN_POINT('',(0.3,12.1581243060695,15.913942841485));
#92103=CARTESIAN_POINT('Origin',(0.15,12.85,22.25));
#92104=CARTESIAN_POINT('',(0.,12.7,25.17));
#92105=CARTESIAN_POINT('',(0.3,13.,22.25));
#92106=CARTESIAN_POINT('Origin',(0.15,6.75,25.32));
#92107=CARTESIAN_POINT('',(0.,9.2,25.17));
#92108=CARTESIAN_POINT('Origin',(0.15,9.35,30.015));
#92109=CARTESIAN_POINT('',(0.,9.2,31.83));
#92110=CARTESIAN_POINT('Origin',(0.15,9.,31.68));
#92111=CARTESIAN_POINT('',(0.,12.7,31.83));
#92112=CARTESIAN_POINT('Origin',(0.15,12.85,22.25));
#92113=CARTESIAN_POINT('',(0.,12.7,40.4267949192431));
#92114=CARTESIAN_POINT('Origin',(0.15,12.0831243060696,40.9561533479473));
#92115=CARTESIAN_POINT('',(0.,12.6535898384862,40.4535898384862));
#92116=CARTESIAN_POINT('Origin',(0.15,6.99367061317363,37.3590390309174));
#92117=CARTESIAN_POINT('Origin',(0.15,7.85,18.5));
#92118=CARTESIAN_POINT('',(0.,7.7,47.8757359312881));
#92119=CARTESIAN_POINT('Origin',(0.15,11.643933982822,44.143933982822));
#92120=CARTESIAN_POINT('',(0.,7.37573593128807,48.2));
#92121=CARTESIAN_POINT('Origin',(0.15,6.,48.35));
#92122=CARTESIAN_POINT('',(0.,0.624264068711926,48.2));
#92123=CARTESIAN_POINT('Origin',(0.15,-3.64393398282203,44.1439339828219));
#92124=CARTESIAN_POINT('Origin',(0.15,0.15,38.5));
#92125=CARTESIAN_POINT('',(0.,0.300000000000004,9.12426406871192));
#92126=CARTESIAN_POINT('Origin',(0.15,-3.64393398282202,12.856066017178));
#92127=CARTESIAN_POINT('',(0.,0.624264068711924,8.8));
#92128=CARTESIAN_POINT('Origin',(0.15,2.,8.65));
#92129=CARTESIAN_POINT('',(0.,7.37573593128808,8.8));
#92130=CARTESIAN_POINT('Origin',(0.15,11.643933982822,12.856066017178));
#92131=CARTESIAN_POINT('',(0.,7.7,9.12426406871192));
#92132=CARTESIAN_POINT('Origin',(0.15,7.85,18.5));
#92133=CARTESIAN_POINT('Origin',(0.3,8.,18.8867513459481));
#92134=CARTESIAN_POINT('Origin',(220.,4.,28.5));
#92135=CARTESIAN_POINT('Origin',(220.,8.,18.8867513459481));
#92136=CARTESIAN_POINT('Origin',(0.,13.,16.));
#92137=CARTESIAN_POINT('',(0.,13.,16.4));
#92138=CARTESIAN_POINT('Origin',(0.,8.,18.8867513459481));
#92139=CARTESIAN_POINT('',(0.,8.43301270189222,18.6367513459481));
#92140=CARTESIAN_POINT('Origin',(0.,12.8267949192431,16.3));
#92141=CARTESIAN_POINT('',(0.,12.6535898384862,16.2));
#92142=CARTESIAN_POINT('Origin',(0.,8.,18.8867513459481));
#113946=UNCERTAINTY_MEASURE_WITH_UNIT(LENGTH_MEASURE(0.01),#113985,
'DISTANCE_ACCURACY_VALUE',
'Maximum model space distance between geometric entities at asserted c
onnectivities');
#113964=UNCERTAINTY_MEASURE_WITH_UNIT(LENGTH_MEASURE(0.01),#113985,
'DISTANCE_ACCURACY_VALUE',
'Maximum model space distance between geometric entities at asserted c
onnectivities');
#113966=(
GEOMETRIC_REPRESENTATION_CONTEXT(3)
GLOBAL_UNCERTAINTY_ASSIGNED_CONTEXT((#113946))
GLOBAL_UNIT_ASSIGNED_CONTEXT((#113985,#113987,#113988))
REPRESENTATION_CONTEXT('','3D')
);
#113984=(
GEOMETRIC_REPRESENTATION_CONTEXT(3)
GLOBAL_UNCERTAINTY_ASSIGNED_CONTEXT((#113964))
GLOBAL_UNIT_ASSIGNED_CONTEXT((#113985,#113987,#113988))
REPRESENTATION_CONTEXT('','3D')
);
#113985=(
LENGTH_UNIT()
NAMED_UNIT(*)
SI_UNIT(.MILLI.,.METRE.)
);
#113987=(
NAMED_UNIT(*)
PLANE_ANGLE_UNIT()
SI_UNIT($,.RADIAN.)
);
#113988=(
NAMED_UNIT(*)
SI_UNIT($,.STERADIAN.)
SOLID_ANGLE_UNIT()
);
#113990=SHAPE_DEFINITION_REPRESENTATION(#114009,#114052);
#114009=PRODUCT_DEFINITION_SHAPE('',$,#114072);
#114052=SHAPE_REPRESENTATION('',(#60610),#113966);
#114070=PRODUCT_DEFINITION_CONTEXT('part definition',#114129,'design');
#114072=PRODUCT_DEFINITION('2026-10-05-09-42-27-850',
'Cast Iron Dovetail Base Block LWX40 x 220',#114091,#114070);
#114091=PRODUCT_DEFINITION_FORMATION('',$,#114132);
#114129=APPLICATION_CONTEXT(
'Core Data for Automotive Mechanical Design Process');
#114130=PRODUCT_CONTEXT('part definition',#114129,'mechanical');
#114132=PRODUCT('2026-10-05-09-42-27-850',
'Cast Iron Dovetail Base Block LWX40 x 220',$,(#114130));
#114283=COLOUR_RGB('Dark Blue',0.08,0.2,0.34);
#114284=FILL_AREA_STYLE_COLOUR('',#114283);
#114285=FILL_AREA_STYLE('',(#114284));
#114286=SURFACE_STYLE_FILL_AREA(#114285);
#114287=SURFACE_SIDE_STYLE('',(#114286));
#114288=SURFACE_STYLE_USAGE(.BOTH.,#114287);
#114289=PRESENTATION_STYLE_ASSIGNMENT((#114288));
ENDSEC;
END-ISO-10303-21;
